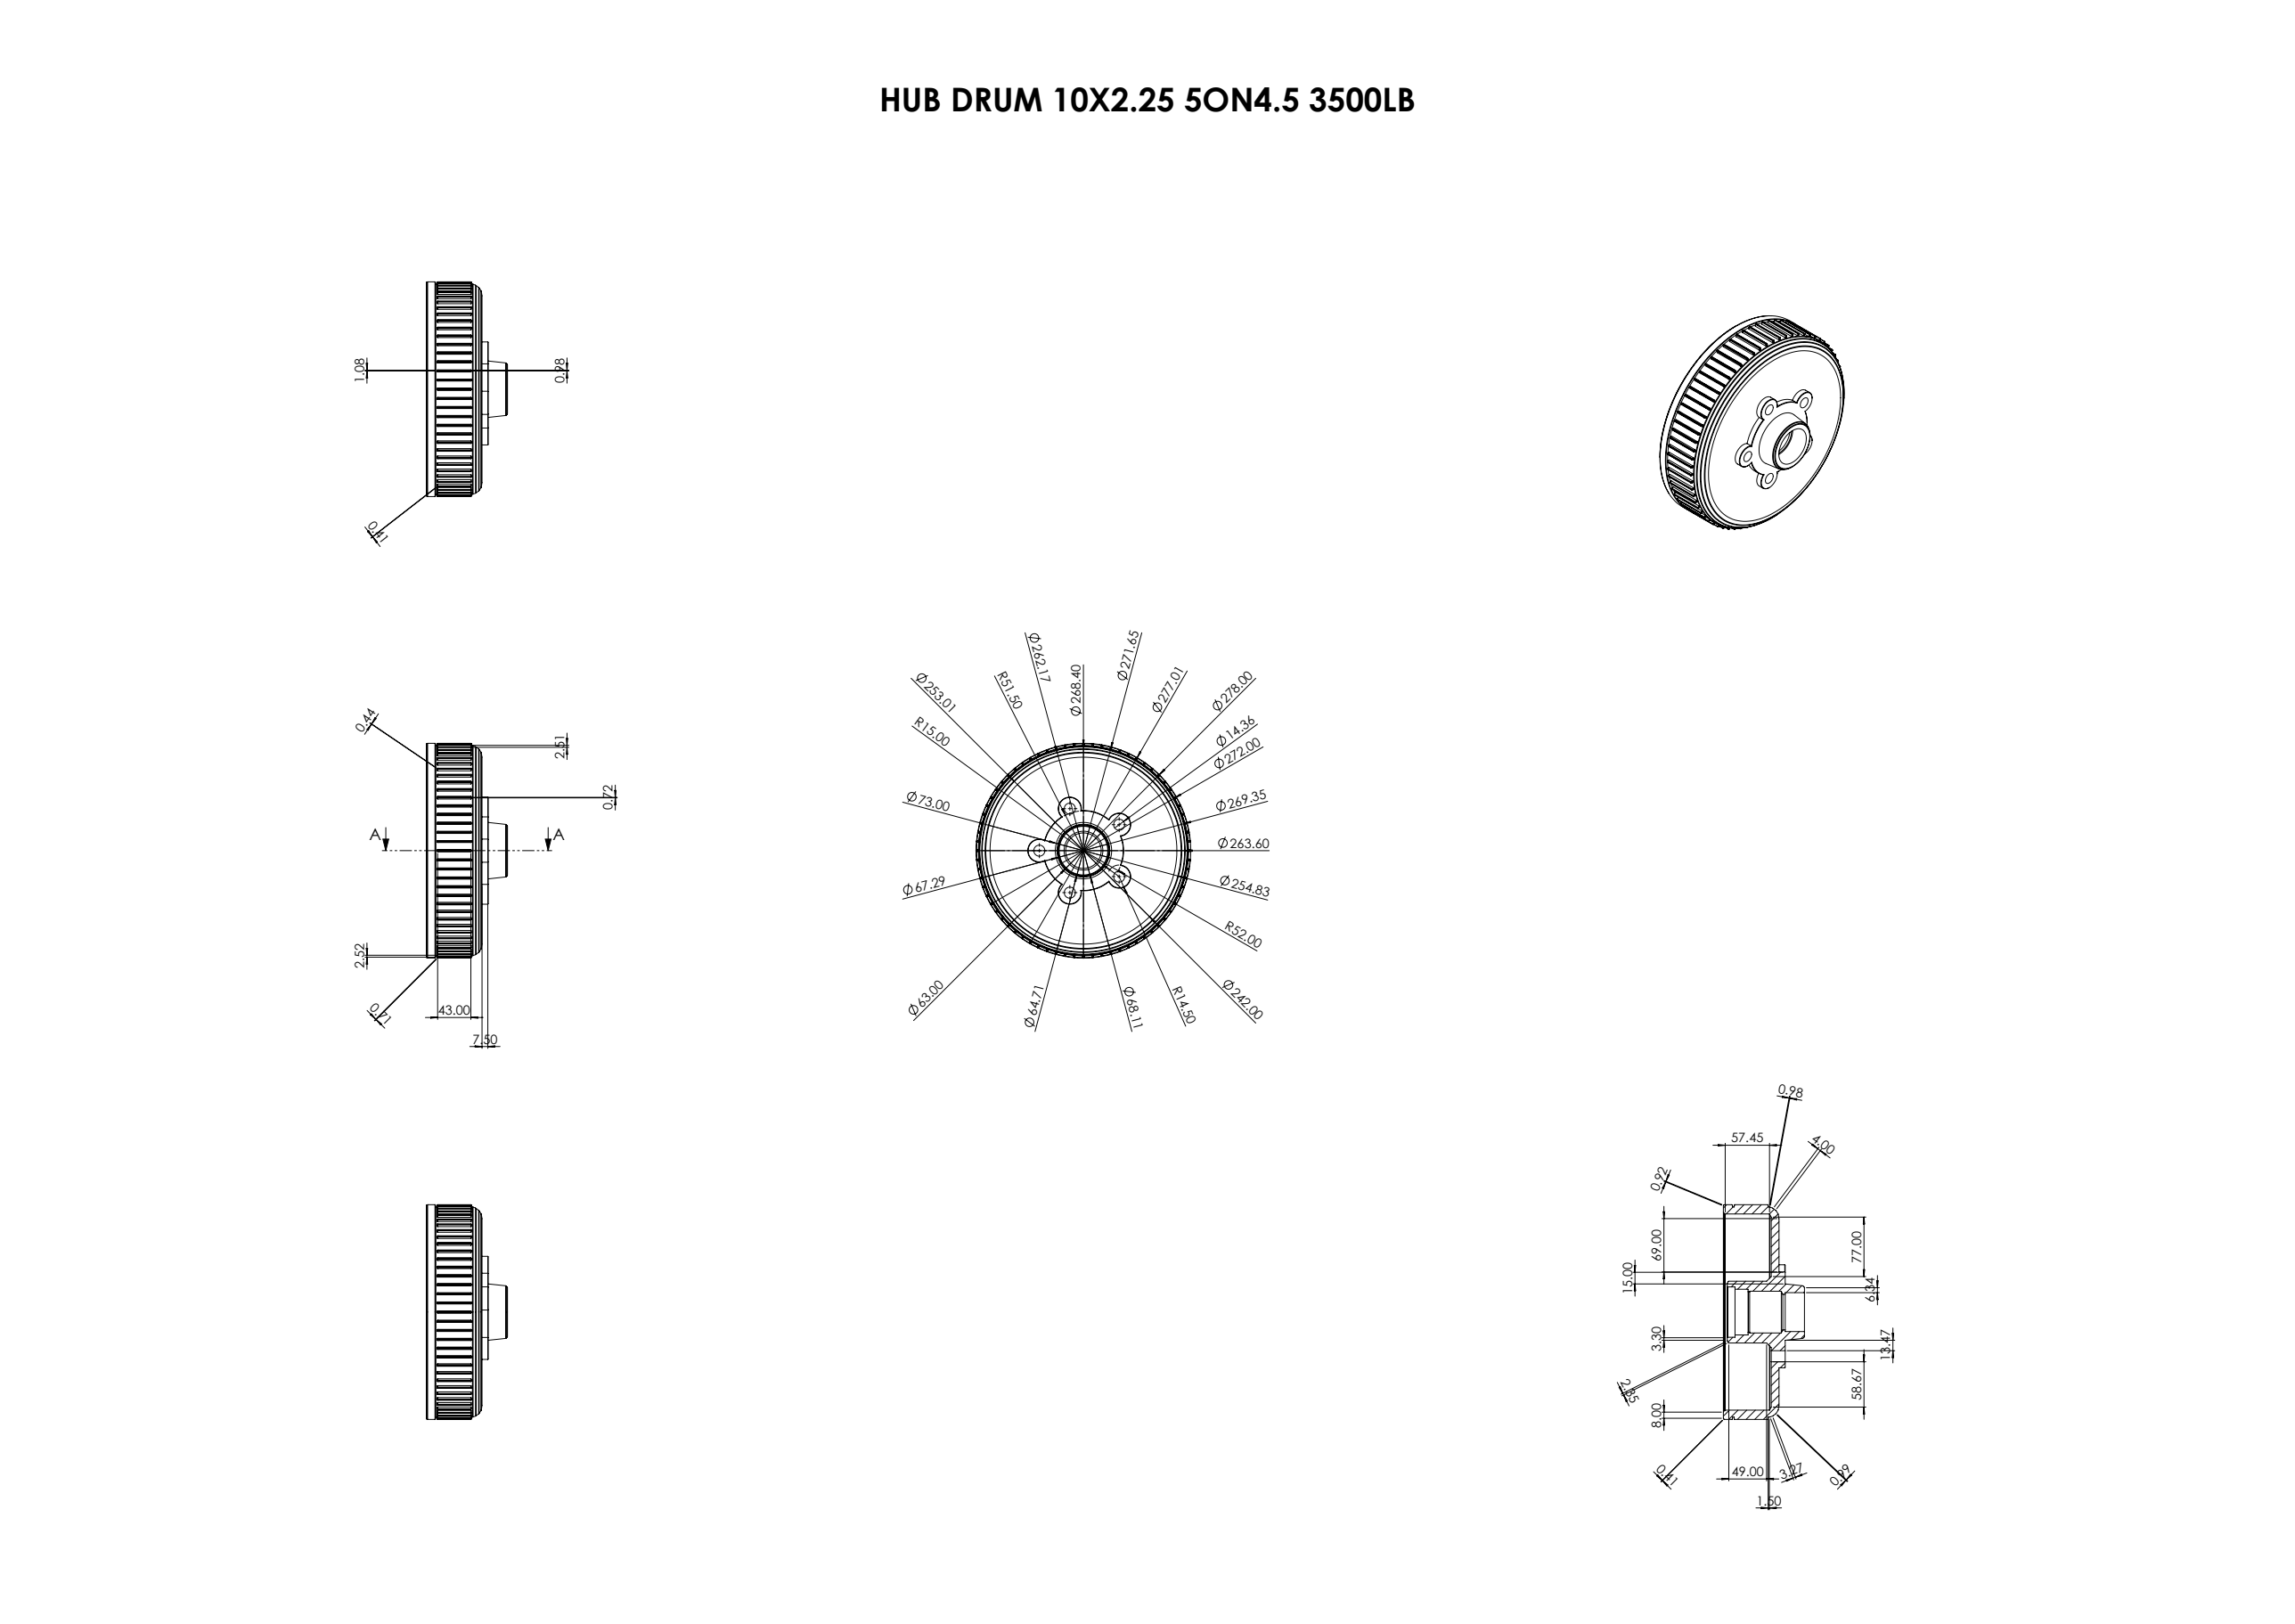
ISO-10303-21;
HEADER;
/* Generated by software containing ST-Developer
 * from STEP Tools, Inc. (www.steptools.com) 
 */

FILE_DESCRIPTION(
/* description */ (''),
/* implementation_level */ '2;1');

FILE_NAME(
/* name */ '01_Hub_Drum_10x2.25_5on4.5_3500lb.step',
/* time_stamp */ '2026-10-25T01:26:34-07:00',
/* author */ (''),
/* organization */ (''),
/* preprocessor_version */ 'ST-DEVELOPER v20.2',
/* originating_system */ 'Autodesk Translation Framework v15.15.0.0',
/* authorisation */ '');

FILE_SCHEMA (('AUTOMOTIVE_DESIGN { 1 0 10303 214 3 1 1 }'));
ENDSEC;

DATA;
#10=MECHANICAL_DESIGN_GEOMETRIC_PRESENTATION_REPRESENTATION('',(#321),#71628);
#295=SHAPE_REPRESENTATION_RELATIONSHIP('SRR','None',#71683,#308);
#308=ADVANCED_BREP_SHAPE_REPRESENTATION('',(#334),#71615);
#321=STYLED_ITEM('',(#71804),#334);
#334=MANIFOLD_SOLID_BREP('Body1',#34208);
#347=B_SPLINE_CURVE_WITH_KNOTS('',3,(#48590,#48591,#48592,#48593),
 .UNSPECIFIED.,.F.,.F.,(4,4),(-0.0954037219784117,0.),.UNSPECIFIED.);
#348=B_SPLINE_CURVE_WITH_KNOTS('',3,(#48596,#48597,#48598,#48599),
 .UNSPECIFIED.,.F.,.F.,(4,4),(-0.0954037219783748,0.),.UNSPECIFIED.);
#349=B_SPLINE_CURVE_WITH_KNOTS('',3,(#48604,#48605,#48606,#48607),
 .UNSPECIFIED.,.F.,.F.,(4,4),(-0.0954037219783863,0.),.UNSPECIFIED.);
#350=B_SPLINE_CURVE_WITH_KNOTS('',3,(#48613,#48614,#48615,#48616),
 .UNSPECIFIED.,.F.,.F.,(4,4),(-0.0954037219782671,0.),.UNSPECIFIED.);
#351=B_SPLINE_CURVE_WITH_KNOTS('',3,(#48622,#48623,#48624,#48625),
 .UNSPECIFIED.,.F.,.F.,(4,4),(-0.0954037219784872,0.),.UNSPECIFIED.);
#352=B_SPLINE_CURVE_WITH_KNOTS('',3,(#48631,#48632,#48633,#48634),
 .UNSPECIFIED.,.F.,.F.,(4,4),(-0.0954037219781768,0.),.UNSPECIFIED.);
#353=B_SPLINE_CURVE_WITH_KNOTS('',3,(#48640,#48641,#48642,#48643),
 .UNSPECIFIED.,.F.,.F.,(4,4),(-0.0954037219782904,0.),.UNSPECIFIED.);
#354=B_SPLINE_CURVE_WITH_KNOTS('',3,(#48650,#48651,#48652,#48653),
 .UNSPECIFIED.,.F.,.F.,(4,4),(-0.0954037219784109,0.),.UNSPECIFIED.);
#355=B_SPLINE_CURVE_WITH_KNOTS('',3,(#48659,#48660,#48661,#48662),
 .UNSPECIFIED.,.F.,.F.,(4,4),(-0.0954037219783438,0.),.UNSPECIFIED.);
#356=B_SPLINE_CURVE_WITH_KNOTS('',3,(#48668,#48669,#48670,#48671),
 .UNSPECIFIED.,.F.,.F.,(4,4),(-0.0954037219783345,0.),.UNSPECIFIED.);
#842=ELLIPSE('',#34430,192.333044482741,136.);
#843=ELLIPSE('',#34431,192.333044482741,136.);
#844=ELLIPSE('',#34435,192.333044482741,136.);
#845=ELLIPSE('',#34436,192.333044482741,136.);
#846=ELLIPSE('',#34438,192.333044482741,136.);
#847=ELLIPSE('',#34440,192.333044482741,136.);
#848=ELLIPSE('',#34441,192.333044482741,136.);
#849=ELLIPSE('',#34443,192.333044482741,136.);
#850=ELLIPSE('',#34444,192.333044482741,136.);
#851=ELLIPSE('',#34446,192.333044482741,136.);
#852=ELLIPSE('',#34447,192.33304448274,136.);
#853=ELLIPSE('',#34449,192.33304448274,136.);
#854=ELLIPSE('',#34450,192.333044482742,136.);
#855=ELLIPSE('',#34452,192.333044482743,136.);
#856=ELLIPSE('',#34453,192.333044482742,136.);
#857=ELLIPSE('',#34455,192.33304448274,136.);
#858=ELLIPSE('',#34456,192.33304448274,136.);
#859=ELLIPSE('',#34458,192.333044482743,136.);
#860=ELLIPSE('',#34459,192.333044482742,136.);
#861=ELLIPSE('',#34461,192.33304448274,136.);
#862=ELLIPSE('',#34462,192.333044482743,136.);
#863=ELLIPSE('',#34464,192.333044482739,136.);
#864=ELLIPSE('',#34465,192.333044482741,136.);
#865=ELLIPSE('',#34467,192.333044482745,136.);
#866=ELLIPSE('',#34468,192.333044482737,136.);
#867=ELLIPSE('',#34470,192.333044482741,136.);
#868=ELLIPSE('',#34471,192.333044482739,136.);
#869=ELLIPSE('',#34473,192.333044482738,136.);
#870=ELLIPSE('',#34474,192.333044482739,136.);
#871=ELLIPSE('',#34476,192.333044482743,136.);
#872=ELLIPSE('',#34477,192.333044482742,136.);
#873=ELLIPSE('',#34479,192.333044482738,136.);
#874=ELLIPSE('',#34480,192.333044482743,136.);
#875=ELLIPSE('',#34482,192.333044482741,136.);
#876=ELLIPSE('',#34483,192.333044482741,136.);
#877=ELLIPSE('',#34485,192.333044482741,136.);
#878=ELLIPSE('',#34486,192.333044482743,136.);
#879=ELLIPSE('',#34488,192.333044482743,136.);
#880=ELLIPSE('',#34489,192.33304448274,136.);
#881=ELLIPSE('',#34491,192.333044482743,136.);
#882=ELLIPSE('',#34492,192.33304448274,136.);
#883=ELLIPSE('',#34494,192.33304448274,136.);
#884=ELLIPSE('',#34495,192.33304448274,136.);
#885=ELLIPSE('',#34497,192.33304448274,136.);
#886=ELLIPSE('',#34498,192.333044482738,136.);
#887=ELLIPSE('',#34500,192.333044482741,136.);
#888=ELLIPSE('',#34501,192.333044482741,136.);
#889=ELLIPSE('',#34503,192.33304448274,136.);
#890=ELLIPSE('',#34504,192.33304448274,136.);
#891=ELLIPSE('',#34506,192.333044482742,136.);
#892=ELLIPSE('',#34507,192.333044482741,136.);
#893=ELLIPSE('',#34509,192.33304448274,136.);
#894=ELLIPSE('',#34510,192.333044482743,136.);
#895=ELLIPSE('',#34512,192.33304448274,136.);
#896=ELLIPSE('',#34513,192.33304448274,136.);
#897=ELLIPSE('',#34515,192.333044482739,136.);
#898=ELLIPSE('',#34516,192.33304448274,136.);
#899=ELLIPSE('',#34518,192.33304448274,136.);
#900=ELLIPSE('',#34519,192.33304448274,136.);
#901=ELLIPSE('',#34521,192.333044482739,136.);
#902=ELLIPSE('',#34522,192.333044482741,136.);
#903=ELLIPSE('',#34524,192.333044482743,136.);
#904=ELLIPSE('',#34525,192.333044482743,136.);
#905=ELLIPSE('',#34527,192.333044482741,136.);
#906=ELLIPSE('',#34528,192.333044482742,136.);
#907=ELLIPSE('',#34530,192.333044482741,136.);
#908=ELLIPSE('',#34531,192.333044482741,136.);
#909=ELLIPSE('',#34533,192.333044482742,136.);
#910=ELLIPSE('',#34534,192.333044482742,136.);
#911=ELLIPSE('',#34536,192.333044482742,136.);
#912=ELLIPSE('',#34537,192.333044482741,136.);
#913=ELLIPSE('',#34539,192.333044482741,136.);
#914=ELLIPSE('',#34540,192.333044482742,136.);
#915=ELLIPSE('',#34542,192.333044482741,136.);
#916=ELLIPSE('',#34543,192.33304448274,136.);
#917=ELLIPSE('',#34545,192.333044482742,136.);
#918=ELLIPSE('',#34546,192.333044482741,136.);
#919=ELLIPSE('',#34548,192.333044482741,136.);
#920=ELLIPSE('',#34549,192.33304448274,136.);
#921=ELLIPSE('',#34551,192.33304448274,136.);
#922=ELLIPSE('',#34552,192.333044482741,136.);
#923=ELLIPSE('',#34554,192.333044482743,136.);
#924=ELLIPSE('',#34555,192.333044482741,136.);
#925=ELLIPSE('',#34557,192.33304448274,136.);
#926=ELLIPSE('',#34558,192.33304448274,136.);
#927=ELLIPSE('',#34560,192.333044482742,136.);
#928=ELLIPSE('',#34561,192.333044482742,136.);
#929=ELLIPSE('',#34563,192.333044482742,136.);
#930=ELLIPSE('',#34564,192.333044482743,136.);
#931=ELLIPSE('',#34566,192.33304448274,136.);
#932=ELLIPSE('',#34567,192.333044482741,136.);
#933=ELLIPSE('',#34569,192.333044482745,136.);
#934=ELLIPSE('',#34570,192.33304448274,136.);
#935=ELLIPSE('',#34572,192.333044482743,136.);
#936=ELLIPSE('',#34573,192.333044482741,136.);
#937=ELLIPSE('',#34575,192.33304448274,136.);
#938=ELLIPSE('',#34576,192.33304448274,136.);
#939=ELLIPSE('',#34578,192.333044482743,136.);
#940=ELLIPSE('',#34579,192.333044482742,136.);
#941=ELLIPSE('',#34581,192.33304448274,136.);
#942=ELLIPSE('',#34582,192.333044482742,136.);
#943=ELLIPSE('',#34584,192.333044482741,136.);
#944=ELLIPSE('',#34585,192.333044482741,136.);
#945=ELLIPSE('',#34587,192.333044482741,136.);
#946=ELLIPSE('',#34588,192.333044482743,136.);
#947=ELLIPSE('',#34590,192.333044482741,136.);
#948=ELLIPSE('',#34591,192.33304448274,136.);
#949=ELLIPSE('',#34593,192.333044482743,136.);
#950=ELLIPSE('',#34594,192.33304448274,136.);
#951=ELLIPSE('',#34596,192.33304448274,136.);
#952=ELLIPSE('',#34597,192.33304448274,136.);
#953=ELLIPSE('',#34599,192.33304448274,136.);
#954=ELLIPSE('',#34600,192.333044482738,136.);
#955=ELLIPSE('',#34602,192.333044482741,136.);
#956=ELLIPSE('',#34603,192.333044482741,136.);
#957=ELLIPSE('',#34605,192.333044482738,136.);
#958=ELLIPSE('',#34606,192.333044482743,136.);
#959=ELLIPSE('',#34608,192.333044482742,136.);
#960=ELLIPSE('',#34609,192.333044482741,136.);
#961=ELLIPSE('',#34611,192.33304448274,136.);
#962=ELLIPSE('',#34612,192.333044482741,136.);
#963=ELLIPSE('',#34614,192.333044482739,136.);
#964=ELLIPSE('',#34615,192.33304448274,136.);
#965=ELLIPSE('',#34617,192.333044482741,136.);
#966=ELLIPSE('',#34618,192.333044482741,136.);
#967=ELLIPSE('',#34620,192.333044482739,136.);
#968=ELLIPSE('',#34621,192.333044482738,136.);
#969=ELLIPSE('',#34623,192.333044482741,136.);
#970=ELLIPSE('',#34624,192.333044482743,136.);
#971=ELLIPSE('',#34626,192.333044482743,136.);
#972=ELLIPSE('',#34627,192.333044482743,136.);
#973=ELLIPSE('',#34629,192.333044482741,136.);
#974=ELLIPSE('',#34630,192.333044482741,136.);
#975=ELLIPSE('',#34632,192.333044482741,136.);
#976=ELLIPSE('',#34633,192.333044482741,136.);
#977=ELLIPSE('',#34635,192.333044482742,136.);
#978=ELLIPSE('',#34636,192.333044482743,136.);
#979=ELLIPSE('',#34638,192.33304448274,136.);
#980=ELLIPSE('',#34639,192.333044482739,136.);
#981=ELLIPSE('',#34641,192.333044482742,136.);
#982=ELLIPSE('',#34642,192.333044482741,136.);
#983=ELLIPSE('',#34644,192.33304448274,136.);
#984=ELLIPSE('',#34645,192.33304448274,136.);
#985=ELLIPSE('',#34647,192.333044482741,136.);
#986=ELLIPSE('',#34648,192.333044482741,136.);
#987=ELLIPSE('',#34650,192.333044482741,136.);
#988=ELLIPSE('',#34651,192.33304448274,136.);
#989=ELLIPSE('',#34653,192.333044482741,136.);
#990=ELLIPSE('',#34654,192.333044482741,136.);
#991=ELLIPSE('',#34656,192.333044482741,136.);
#992=ELLIPSE('',#34657,192.33304448274,136.);
#993=ELLIPSE('',#34659,192.33304448274,136.);
#994=ELLIPSE('',#34660,192.333044482742,136.);
#995=ELLIPSE('',#34662,192.333044482743,136.);
#996=ELLIPSE('',#34663,192.333044482742,136.);
#997=ELLIPSE('',#34665,192.33304448274,136.);
#998=ELLIPSE('',#34666,192.333044482741,136.);
#999=ELLIPSE('',#34668,192.333044482742,136.);
#1000=ELLIPSE('',#34669,192.333044482742,136.);
#1001=ELLIPSE('',#34671,192.33304448274,136.);
#1002=ELLIPSE('',#34672,192.333044482745,136.);
#1003=ELLIPSE('',#34674,192.333044482739,136.);
#1004=ELLIPSE('',#34675,192.333044482741,136.);
#1005=ELLIPSE('',#34677,192.333044482745,136.);
#1006=ELLIPSE('',#34678,192.333044482739,136.);
#1007=ELLIPSE('',#34680,192.333044482741,136.);
#1008=ELLIPSE('',#34681,192.333044482741,136.);
#1009=ELLIPSE('',#34683,192.333044482738,136.);
#1010=ELLIPSE('',#34684,192.33304448274,136.);
#1011=ELLIPSE('',#34686,192.333044482743,136.);
#1012=ELLIPSE('',#34687,192.333044482742,136.);
#1013=ELLIPSE('',#34689,192.33304448274,136.);
#1014=ELLIPSE('',#34690,192.333044482742,136.);
#1015=ELLIPSE('',#34692,192.333044482741,136.);
#1016=ELLIPSE('',#34693,192.333044482741,136.);
#1017=ELLIPSE('',#34695,192.333044482741,136.);
#1018=ELLIPSE('',#34696,192.333044482743,136.);
#1019=ELLIPSE('',#34698,192.333044482743,136.);
#1020=ELLIPSE('',#34699,192.33304448274,136.);
#1021=ELLIPSE('',#34701,192.333044482743,136.);
#1022=ELLIPSE('',#34702,192.333044482738,136.);
#1023=ELLIPSE('',#34704,192.33304448274,136.);
#1024=ELLIPSE('',#34705,192.33304448274,136.);
#1025=ELLIPSE('',#34707,192.33304448274,136.);
#1026=ELLIPSE('',#34708,192.333044482738,136.);
#1027=ELLIPSE('',#34710,192.333044482741,136.);
#1028=ELLIPSE('',#34711,192.333044482741,136.);
#1029=ELLIPSE('',#34713,192.333044482738,136.);
#1030=ELLIPSE('',#34714,192.333044482743,136.);
#1031=ELLIPSE('',#34716,192.333044482742,136.);
#1032=ELLIPSE('',#34717,192.333044482741,136.);
#1033=ELLIPSE('',#34719,192.33304448274,136.);
#1034=ELLIPSE('',#34720,192.333044482744,136.);
#1035=ELLIPSE('',#34722,192.33304448274,136.);
#1036=ELLIPSE('',#34723,192.33304448274,136.);
#1037=ELLIPSE('',#34725,192.333044482741,136.);
#1038=ELLIPSE('',#34726,192.333044482741,136.);
#1039=ELLIPSE('',#34728,192.33304448274,136.);
#1040=ELLIPSE('',#34729,192.33304448274,136.);
#1041=ELLIPSE('',#34731,192.333044482741,136.);
#1042=ELLIPSE('',#34732,192.333044482741,136.);
#1043=ELLIPSE('',#34734,192.333044482742,136.);
#1044=ELLIPSE('',#34735,192.333044482741,136.);
#1045=ELLIPSE('',#34737,192.333044482741,136.);
#1046=ELLIPSE('',#34738,192.333044482741,136.);
#1047=ELLIPSE('',#34740,192.33304448274,136.);
#1048=ELLIPSE('',#34741,192.333044482742,136.);
#1049=ELLIPSE('',#34743,192.333044482742,136.);
#1050=ELLIPSE('',#34744,192.333044482743,136.);
#1051=ELLIPSE('',#34746,192.333044482742,136.);
#1052=ELLIPSE('',#34747,192.333044482741,136.);
#1053=ELLIPSE('',#34749,192.333044482741,136.);
#1054=ELLIPSE('',#34750,192.333044482742,136.);
#1055=ELLIPSE('',#34752,192.333044482741,136.);
#1056=ELLIPSE('',#34753,192.33304448274,136.);
#1057=ELLIPSE('',#34755,192.333044482741,136.);
#1058=ELLIPSE('',#34756,192.333044482741,136.);
#1059=ELLIPSE('',#34758,192.333044482741,136.);
#1060=ELLIPSE('',#34759,192.33304448274,136.);
#1061=ELLIPSE('',#34761,192.333044482741,136.);
#1062=ELLIPSE('',#34762,192.333044482741,136.);
#1063=ELLIPSE('',#34764,192.333044482741,136.);
#1064=ELLIPSE('',#34765,192.333044482741,136.);
#1065=ELLIPSE('',#34767,192.33304448274,136.);
#1066=ELLIPSE('',#34768,192.333044482742,136.);
#1067=ELLIPSE('',#34770,192.333044482742,136.);
#1068=ELLIPSE('',#34771,192.333044482741,136.);
#1069=ELLIPSE('',#34773,192.33304448274,136.);
#1070=ELLIPSE('',#34774,192.33304448274,136.);
#1071=ELLIPSE('',#34776,192.333044482742,136.);
#1072=ELLIPSE('',#34777,192.333044482742,136.);
#1073=ELLIPSE('',#34779,192.33304448274,136.);
#1074=ELLIPSE('',#34780,192.333044482742,136.);
#1075=ELLIPSE('',#34782,192.333044482741,136.);
#1076=ELLIPSE('',#34783,192.333044482741,136.);
#1077=ELLIPSE('',#34785,192.333044482743,136.);
#1078=ELLIPSE('',#34786,192.33304448274,136.);
#1079=ELLIPSE('',#34788,192.333044482743,136.);
#1080=ELLIPSE('',#34789,192.333044482742,136.);
#1081=ELLIPSE('',#34791,192.33304448274,136.);
#1082=ELLIPSE('',#34792,192.333044482739,136.);
#1083=ELLIPSE('',#34794,192.333044482741,136.);
#1084=ELLIPSE('',#34795,192.333044482741,136.);
#1085=ELLIPSE('',#34797,192.333044482738,136.);
#1086=ELLIPSE('',#34798,192.333044482743,136.);
#1087=ELLIPSE('',#34800,192.333044482741,136.);
#1088=ELLIPSE('',#34801,192.333044482741,136.);
#1089=ELLIPSE('',#34803,192.333044482741,136.);
#1090=ELLIPSE('',#34804,192.333044482743,136.);
#1091=ELLIPSE('',#34806,192.333044482741,136.);
#1092=ELLIPSE('',#34807,192.33304448274,136.);
#1093=ELLIPSE('',#34809,192.333044482743,136.);
#1094=ELLIPSE('',#34810,192.33304448274,136.);
#1095=ELLIPSE('',#34812,192.33304448274,136.);
#1096=ELLIPSE('',#34813,192.33304448274,136.);
#1097=ELLIPSE('',#34815,192.33304448274,136.);
#1098=ELLIPSE('',#34816,192.333044482738,136.);
#1099=ELLIPSE('',#34818,192.333044482738,136.);
#1100=ELLIPSE('',#34819,192.333044482743,136.);
#1101=ELLIPSE('',#34821,192.333044482738,136.);
#1102=ELLIPSE('',#34822,192.333044482743,136.);
#1103=ELLIPSE('',#34824,192.33304448274,136.);
#1104=ELLIPSE('',#34825,192.33304448274,136.);
#1105=ELLIPSE('',#34827,192.33304448274,136.);
#1106=ELLIPSE('',#34828,192.333044482744,136.);
#1107=ELLIPSE('',#34830,192.33304448274,136.);
#1108=ELLIPSE('',#34831,192.33304448274,136.);
#1109=ELLIPSE('',#34833,192.333044482741,136.);
#1110=ELLIPSE('',#34834,192.333044482741,136.);
#1111=ELLIPSE('',#34836,192.33304448274,136.);
#1112=ELLIPSE('',#34837,192.33304448274,136.);
#1113=ELLIPSE('',#34839,192.333044482741,136.);
#1114=ELLIPSE('',#34840,192.333044482743,136.);
#1115=ELLIPSE('',#34842,192.333044482743,136.);
#1116=ELLIPSE('',#34843,192.33304448274,136.);
#1117=ELLIPSE('',#34845,192.333044482742,136.);
#1118=ELLIPSE('',#34846,192.333044482742,136.);
#1119=ELLIPSE('',#34848,192.333044482741,136.);
#1120=ELLIPSE('',#34849,192.333044482741,136.);
#1121=ELLIPSE('',#34851,192.333044482742,136.);
#1122=ELLIPSE('',#34852,192.333044482743,136.);
#1123=ELLIPSE('',#34854,192.333044482742,136.);
#1124=ELLIPSE('',#34855,192.333044482741,136.);
#1125=ELLIPSE('',#34857,192.333044482741,136.);
#1126=ELLIPSE('',#34858,192.333044482742,136.);
#1127=ELLIPSE('',#34860,192.333044482741,136.);
#1128=ELLIPSE('',#34861,192.33304448274,136.);
#1129=ELLIPSE('',#34863,192.333044482741,136.);
#1130=FACE_BOUND('',#5239,.T.);
#1131=FACE_BOUND('',#5243,.T.);
#1132=FACE_BOUND('',#5247,.T.);
#1133=FACE_BOUND('',#5259,.T.);
#1134=FACE_BOUND('',#5260,.T.);
#1135=FACE_BOUND('',#5261,.T.);
#1136=FACE_BOUND('',#5262,.T.);
#1137=FACE_BOUND('',#5263,.T.);
#1138=FACE_BOUND('',#5264,.T.);
#1139=FACE_BOUND('',#5265,.T.);
#1140=FACE_BOUND('',#5266,.T.);
#1141=FACE_BOUND('',#5267,.T.);
#1142=FACE_BOUND('',#5268,.T.);
#1143=FACE_BOUND('',#5269,.T.);
#1144=FACE_BOUND('',#5270,.T.);
#1145=FACE_BOUND('',#5271,.T.);
#1146=FACE_BOUND('',#5272,.T.);
#1147=FACE_BOUND('',#5273,.T.);
#1148=FACE_BOUND('',#5274,.T.);
#1149=FACE_BOUND('',#5275,.T.);
#1150=FACE_BOUND('',#5276,.T.);
#1151=FACE_BOUND('',#5277,.T.);
#1152=FACE_BOUND('',#5278,.T.);
#1153=FACE_BOUND('',#5279,.T.);
#1154=FACE_BOUND('',#5280,.T.);
#1155=FACE_BOUND('',#5281,.T.);
#1156=FACE_BOUND('',#5282,.T.);
#1157=FACE_BOUND('',#5283,.T.);
#1158=FACE_BOUND('',#5284,.T.);
#1159=FACE_BOUND('',#5285,.T.);
#1160=FACE_BOUND('',#5286,.T.);
#1161=FACE_BOUND('',#5287,.T.);
#1162=FACE_BOUND('',#5288,.T.);
#1163=FACE_BOUND('',#5289,.T.);
#1164=FACE_BOUND('',#5290,.T.);
#1165=FACE_BOUND('',#5291,.T.);
#1166=FACE_BOUND('',#5292,.T.);
#1167=FACE_BOUND('',#5293,.T.);
#1168=FACE_BOUND('',#5294,.T.);
#1169=FACE_BOUND('',#5295,.T.);
#1170=FACE_BOUND('',#5296,.T.);
#1171=FACE_BOUND('',#5297,.T.);
#1172=FACE_BOUND('',#5298,.T.);
#1173=FACE_BOUND('',#5299,.T.);
#1174=FACE_BOUND('',#5300,.T.);
#1175=FACE_BOUND('',#5301,.T.);
#1176=FACE_BOUND('',#5302,.T.);
#1177=FACE_BOUND('',#5303,.T.);
#1178=FACE_BOUND('',#5304,.T.);
#1179=FACE_BOUND('',#5305,.T.);
#1180=FACE_BOUND('',#5306,.T.);
#1181=FACE_BOUND('',#5307,.T.);
#1182=FACE_BOUND('',#5308,.T.);
#1183=FACE_BOUND('',#5309,.T.);
#1184=FACE_BOUND('',#5310,.T.);
#1185=FACE_BOUND('',#5311,.T.);
#1186=FACE_BOUND('',#5312,.T.);
#1187=FACE_BOUND('',#5313,.T.);
#1188=FACE_BOUND('',#5314,.T.);
#1189=FACE_BOUND('',#5315,.T.);
#1190=FACE_BOUND('',#5316,.T.);
#1191=FACE_BOUND('',#5317,.T.);
#1192=FACE_BOUND('',#5318,.T.);
#1193=FACE_BOUND('',#5319,.T.);
#1194=FACE_BOUND('',#5320,.T.);
#1195=FACE_BOUND('',#5321,.T.);
#1196=FACE_BOUND('',#5322,.T.);
#1197=FACE_BOUND('',#5323,.T.);
#1198=FACE_BOUND('',#5324,.T.);
#1199=FACE_BOUND('',#5325,.T.);
#1200=FACE_BOUND('',#5326,.T.);
#1201=FACE_BOUND('',#5327,.T.);
#1202=FACE_BOUND('',#5328,.T.);
#1203=FACE_BOUND('',#5329,.T.);
#1204=FACE_BOUND('',#5347,.T.);
#1205=FACE_BOUND('',#5348,.T.);
#1206=FACE_BOUND('',#5349,.T.);
#1207=FACE_BOUND('',#5350,.T.);
#1208=FACE_BOUND('',#5351,.T.);
#1209=FACE_BOUND('',#5352,.T.);
#1210=FACE_BOUND('',#6399,.T.);
#1211=FACE_BOUND('',#6559,.T.);
#1212=FACE_BOUND('',#6562,.T.);
#1213=FACE_BOUND('',#6565,.T.);
#1214=FACE_BOUND('',#6568,.T.);
#1215=FACE_BOUND('',#6573,.T.);
#1216=FACE_BOUND('',#6574,.T.);
#1217=FACE_BOUND('',#6575,.T.);
#1218=FACE_BOUND('',#6576,.T.);
#1219=FACE_BOUND('',#6577,.T.);
#1220=FACE_BOUND('',#6578,.T.);
#1335=PLANE('',#34379);
#1336=PLANE('',#34387);
#1337=PLANE('',#34396);
#1338=PLANE('',#34906);
#1339=PLANE('',#34912);
#1340=PLANE('',#34913);
#1341=PLANE('',#34914);
#1342=PLANE('',#34915);
#1343=PLANE('',#34916);
#1344=PLANE('',#34917);
#1345=PLANE('',#34918);
#1346=PLANE('',#34919);
#1347=PLANE('',#34920);
#1348=PLANE('',#34921);
#1349=PLANE('',#34922);
#1350=PLANE('',#34923);
#1351=PLANE('',#34924);
#1352=PLANE('',#34925);
#1353=PLANE('',#34926);
#1354=PLANE('',#34927);
#1355=PLANE('',#34928);
#1356=PLANE('',#34929);
#1357=PLANE('',#34930);
#1358=PLANE('',#34931);
#1359=PLANE('',#34932);
#1360=PLANE('',#34933);
#1361=PLANE('',#34934);
#1362=PLANE('',#34935);
#1363=PLANE('',#34936);
#1364=PLANE('',#34937);
#1365=PLANE('',#34938);
#1366=PLANE('',#34939);
#1367=PLANE('',#34940);
#1368=PLANE('',#34941);
#1369=PLANE('',#34942);
#1370=PLANE('',#34943);
#1371=PLANE('',#34944);
#1372=PLANE('',#34945);
#1373=PLANE('',#34946);
#1374=PLANE('',#34947);
#1375=PLANE('',#34948);
#1376=PLANE('',#34949);
#1377=PLANE('',#34950);
#1378=PLANE('',#34951);
#1379=PLANE('',#34952);
#1380=PLANE('',#34953);
#1381=PLANE('',#34954);
#1382=PLANE('',#34955);
#1383=PLANE('',#34956);
#1384=PLANE('',#34957);
#1385=PLANE('',#34958);
#1386=PLANE('',#34959);
#1387=PLANE('',#34960);
#1388=PLANE('',#34961);
#1389=PLANE('',#34962);
#1390=PLANE('',#34963);
#1391=PLANE('',#34964);
#1392=PLANE('',#34965);
#1393=PLANE('',#34966);
#1394=PLANE('',#34967);
#1395=PLANE('',#34968);
#1396=PLANE('',#34969);
#1397=PLANE('',#34970);
#1398=PLANE('',#34971);
#1399=PLANE('',#34972);
#1400=PLANE('',#34973);
#1401=PLANE('',#34974);
#1402=PLANE('',#34975);
#1403=PLANE('',#34976);
#1404=PLANE('',#34977);
#1405=PLANE('',#34978);
#1406=PLANE('',#34979);
#1407=PLANE('',#34980);
#1408=PLANE('',#34981);
#1409=PLANE('',#34982);
#1410=PLANE('',#34983);
#1411=PLANE('',#34984);
#1412=PLANE('',#34985);
#1413=PLANE('',#34986);
#1414=PLANE('',#34987);
#1415=PLANE('',#34988);
#1416=PLANE('',#34989);
#1417=PLANE('',#34990);
#1418=PLANE('',#34991);
#1419=PLANE('',#34992);
#1420=PLANE('',#34993);
#1421=PLANE('',#34994);
#1422=PLANE('',#34995);
#1423=PLANE('',#34996);
#1424=PLANE('',#34997);
#1425=PLANE('',#34998);
#1426=PLANE('',#34999);
#1427=PLANE('',#35000);
#1428=PLANE('',#35001);
#1429=PLANE('',#35002);
#1430=PLANE('',#35003);
#1431=PLANE('',#35004);
#1432=PLANE('',#35005);
#1433=PLANE('',#35006);
#1434=PLANE('',#35007);
#1435=PLANE('',#35008);
#1436=PLANE('',#35009);
#1437=PLANE('',#35010);
#1438=PLANE('',#35011);
#1439=PLANE('',#35012);
#1440=PLANE('',#35013);
#1441=PLANE('',#35014);
#1442=PLANE('',#35015);
#1443=PLANE('',#35016);
#1444=PLANE('',#35017);
#1445=PLANE('',#35018);
#1446=PLANE('',#35019);
#1447=PLANE('',#35020);
#1448=PLANE('',#35021);
#1449=PLANE('',#35022);
#1450=PLANE('',#35023);
#1451=PLANE('',#35024);
#1452=PLANE('',#35025);
#1453=PLANE('',#35026);
#1454=PLANE('',#35027);
#1455=PLANE('',#35028);
#1456=PLANE('',#35029);
#1457=PLANE('',#35030);
#1458=PLANE('',#35031);
#1459=PLANE('',#35032);
#1460=PLANE('',#35033);
#1461=PLANE('',#35034);
#1462=PLANE('',#35035);
#1463=PLANE('',#35036);
#1464=PLANE('',#35037);
#1465=PLANE('',#35038);
#1466=PLANE('',#35039);
#1467=PLANE('',#35040);
#1468=PLANE('',#35041);
#1469=PLANE('',#35042);
#1470=PLANE('',#35043);
#1471=PLANE('',#35044);
#1472=PLANE('',#35045);
#1473=PLANE('',#35046);
#1474=PLANE('',#35047);
#1475=PLANE('',#35048);
#1476=PLANE('',#35049);
#1477=PLANE('',#35050);
#1478=PLANE('',#35051);
#1479=PLANE('',#35052);
#1480=PLANE('',#35053);
#1481=PLANE('',#35054);
#1482=PLANE('',#35055);
#1483=PLANE('',#35056);
#1484=PLANE('',#35057);
#1485=PLANE('',#35058);
#1486=PLANE('',#35059);
#1487=PLANE('',#35060);
#1488=PLANE('',#35061);
#1489=PLANE('',#35062);
#1490=PLANE('',#35063);
#1491=PLANE('',#35064);
#1492=PLANE('',#35065);
#1493=PLANE('',#35066);
#1494=PLANE('',#35067);
#1495=PLANE('',#35068);
#1496=PLANE('',#35069);
#1497=PLANE('',#35070);
#1498=PLANE('',#35071);
#1499=PLANE('',#35072);
#1500=PLANE('',#35073);
#1501=PLANE('',#35074);
#1502=PLANE('',#35075);
#1503=PLANE('',#35076);
#1504=PLANE('',#35077);
#1505=PLANE('',#35078);
#1506=PLANE('',#35079);
#1507=PLANE('',#35080);
#1508=PLANE('',#35081);
#1509=PLANE('',#35082);
#1510=PLANE('',#35083);
#1511=PLANE('',#35084);
#1512=PLANE('',#35085);
#1513=PLANE('',#35086);
#1514=PLANE('',#35087);
#1515=PLANE('',#35088);
#1516=PLANE('',#35089);
#1517=PLANE('',#35090);
#1518=PLANE('',#35091);
#1519=PLANE('',#35092);
#1520=PLANE('',#35093);
#1521=PLANE('',#35094);
#1522=PLANE('',#35095);
#1523=PLANE('',#35096);
#1524=PLANE('',#35097);
#1525=PLANE('',#35098);
#1526=PLANE('',#35099);
#1527=PLANE('',#35100);
#1528=PLANE('',#35101);
#1529=PLANE('',#35102);
#1530=PLANE('',#35103);
#1531=PLANE('',#35104);
#1532=PLANE('',#35105);
#1533=PLANE('',#35106);
#1534=PLANE('',#35107);
#1535=PLANE('',#35108);
#1536=PLANE('',#35109);
#1537=PLANE('',#35110);
#1538=PLANE('',#35111);
#1539=PLANE('',#35112);
#1540=PLANE('',#35113);
#1541=PLANE('',#35114);
#1542=PLANE('',#35115);
#1543=PLANE('',#35116);
#1544=PLANE('',#35117);
#1545=PLANE('',#35118);
#1546=PLANE('',#35119);
#1547=PLANE('',#35120);
#1548=PLANE('',#35121);
#1549=PLANE('',#35122);
#1550=PLANE('',#35123);
#1551=PLANE('',#35124);
#1552=PLANE('',#35125);
#1553=PLANE('',#35126);
#1554=PLANE('',#35127);
#1555=PLANE('',#35128);
#1556=PLANE('',#35129);
#1557=PLANE('',#35130);
#1558=PLANE('',#35131);
#1559=PLANE('',#35132);
#1560=PLANE('',#35133);
#1561=PLANE('',#35134);
#1562=PLANE('',#35135);
#1563=PLANE('',#35136);
#1564=PLANE('',#35137);
#1565=PLANE('',#35138);
#1566=PLANE('',#35139);
#1567=PLANE('',#35140);
#1568=PLANE('',#35141);
#1569=PLANE('',#35142);
#1570=PLANE('',#35143);
#1571=PLANE('',#35144);
#1572=PLANE('',#35145);
#1573=PLANE('',#35146);
#1574=PLANE('',#35147);
#1575=PLANE('',#35148);
#1576=PLANE('',#35149);
#1577=PLANE('',#35150);
#1578=PLANE('',#35151);
#1579=PLANE('',#35152);
#1580=PLANE('',#35153);
#1581=PLANE('',#35154);
#1582=PLANE('',#35155);
#1583=PLANE('',#35156);
#1584=PLANE('',#35157);
#1585=PLANE('',#35158);
#1586=PLANE('',#35159);
#1587=PLANE('',#35160);
#1588=PLANE('',#35161);
#1589=PLANE('',#35162);
#1590=PLANE('',#35163);
#1591=PLANE('',#35164);
#1592=PLANE('',#35165);
#1593=PLANE('',#35166);
#1594=PLANE('',#35167);
#1595=PLANE('',#35168);
#1596=PLANE('',#35169);
#1597=PLANE('',#35170);
#1598=PLANE('',#35171);
#1599=PLANE('',#35172);
#1600=PLANE('',#35173);
#1601=PLANE('',#35174);
#1602=PLANE('',#35175);
#1603=PLANE('',#35176);
#1604=PLANE('',#35177);
#1605=PLANE('',#35178);
#1606=PLANE('',#35179);
#1607=PLANE('',#35180);
#1608=PLANE('',#35181);
#1609=PLANE('',#35182);
#1610=PLANE('',#35183);
#1611=PLANE('',#35184);
#1612=PLANE('',#35185);
#1613=PLANE('',#35186);
#1614=PLANE('',#35187);
#1615=PLANE('',#35188);
#1616=PLANE('',#35189);
#1617=PLANE('',#35190);
#1618=PLANE('',#35191);
#1619=PLANE('',#35192);
#1620=PLANE('',#35193);
#1621=PLANE('',#35194);
#1622=PLANE('',#35195);
#1623=PLANE('',#35196);
#1624=PLANE('',#35197);
#1625=PLANE('',#35198);
#1626=PLANE('',#35199);
#1627=PLANE('',#35200);
#1628=PLANE('',#35201);
#1629=PLANE('',#35202);
#1630=PLANE('',#35203);
#1631=PLANE('',#35204);
#1632=PLANE('',#35205);
#1633=PLANE('',#35206);
#1634=PLANE('',#35207);
#1635=PLANE('',#35208);
#1636=PLANE('',#35209);
#1637=PLANE('',#35210);
#1638=PLANE('',#35211);
#1639=PLANE('',#35212);
#1640=PLANE('',#35213);
#1641=PLANE('',#35214);
#1642=PLANE('',#35215);
#1643=PLANE('',#35216);
#1644=PLANE('',#35217);
#1645=PLANE('',#35218);
#1646=PLANE('',#35219);
#1647=PLANE('',#35220);
#1648=PLANE('',#35221);
#1649=PLANE('',#35222);
#1650=PLANE('',#35223);
#1651=PLANE('',#35224);
#1652=PLANE('',#35225);
#1653=PLANE('',#35226);
#1654=PLANE('',#35227);
#1655=PLANE('',#35228);
#1656=PLANE('',#35229);
#1657=PLANE('',#35230);
#1658=PLANE('',#35231);
#1659=PLANE('',#35232);
#1660=PLANE('',#35233);
#1661=PLANE('',#35234);
#1662=PLANE('',#35235);
#1663=PLANE('',#35236);
#1664=PLANE('',#35237);
#1665=PLANE('',#35238);
#1666=PLANE('',#35239);
#1667=PLANE('',#35240);
#1668=PLANE('',#35241);
#1669=PLANE('',#35242);
#1670=PLANE('',#35243);
#1671=PLANE('',#35244);
#1672=PLANE('',#35245);
#1673=PLANE('',#35246);
#1674=PLANE('',#35247);
#1675=PLANE('',#35248);
#1676=PLANE('',#35249);
#1677=PLANE('',#35250);
#1678=PLANE('',#35251);
#1679=PLANE('',#35252);
#1680=PLANE('',#35253);
#1681=PLANE('',#35254);
#1682=PLANE('',#35255);
#1683=PLANE('',#35256);
#1684=PLANE('',#35257);
#1685=PLANE('',#35258);
#1686=PLANE('',#35259);
#1687=PLANE('',#35260);
#1688=PLANE('',#35261);
#1689=PLANE('',#35262);
#1690=PLANE('',#35263);
#1691=PLANE('',#35264);
#1692=PLANE('',#35265);
#1693=PLANE('',#35266);
#1694=PLANE('',#35267);
#1695=PLANE('',#35268);
#1696=PLANE('',#35269);
#1697=PLANE('',#35270);
#1698=PLANE('',#35271);
#1699=PLANE('',#35272);
#1700=PLANE('',#35273);
#1701=PLANE('',#35274);
#1702=PLANE('',#35275);
#1703=PLANE('',#35276);
#1704=PLANE('',#35277);
#1705=PLANE('',#35278);
#1706=PLANE('',#35279);
#1707=PLANE('',#35280);
#1708=PLANE('',#35281);
#1709=PLANE('',#35282);
#1710=PLANE('',#35283);
#1711=PLANE('',#35284);
#1712=PLANE('',#35285);
#1713=PLANE('',#35286);
#1714=PLANE('',#35287);
#1715=PLANE('',#35288);
#1716=PLANE('',#35289);
#1717=PLANE('',#35290);
#1718=PLANE('',#35291);
#1719=PLANE('',#35292);
#1720=PLANE('',#35293);
#1721=PLANE('',#35294);
#1722=PLANE('',#35295);
#1723=PLANE('',#35296);
#1724=PLANE('',#35297);
#1725=PLANE('',#35298);
#1726=PLANE('',#35299);
#1727=PLANE('',#35300);
#1728=PLANE('',#35301);
#1729=PLANE('',#35302);
#1730=PLANE('',#35303);
#1731=PLANE('',#35304);
#1732=PLANE('',#35305);
#1733=PLANE('',#35306);
#1734=PLANE('',#35307);
#1735=PLANE('',#35308);
#1736=PLANE('',#35309);
#1737=PLANE('',#35310);
#1738=PLANE('',#35311);
#1739=PLANE('',#35312);
#1740=PLANE('',#35313);
#1741=PLANE('',#35314);
#1742=PLANE('',#35315);
#1743=PLANE('',#35316);
#1744=PLANE('',#35317);
#1745=PLANE('',#35318);
#1746=PLANE('',#35319);
#1747=PLANE('',#35320);
#1748=PLANE('',#35321);
#1749=PLANE('',#35322);
#1750=PLANE('',#35323);
#1751=PLANE('',#35324);
#1752=PLANE('',#35325);
#1753=PLANE('',#35326);
#1754=PLANE('',#35327);
#1755=PLANE('',#35328);
#1756=PLANE('',#35329);
#1757=PLANE('',#35330);
#1758=PLANE('',#35331);
#1759=PLANE('',#35332);
#1760=PLANE('',#35333);
#1761=PLANE('',#35334);
#1762=PLANE('',#35335);
#1763=PLANE('',#35336);
#1764=PLANE('',#35337);
#1765=PLANE('',#35338);
#1766=PLANE('',#35339);
#1767=PLANE('',#35340);
#1768=PLANE('',#35341);
#1769=PLANE('',#35342);
#1770=PLANE('',#35343);
#1771=PLANE('',#35344);
#1772=PLANE('',#35345);
#1773=PLANE('',#35346);
#1774=PLANE('',#35347);
#1775=PLANE('',#35348);
#1776=PLANE('',#35349);
#1777=PLANE('',#35350);
#1778=PLANE('',#35351);
#1779=PLANE('',#35352);
#1780=PLANE('',#35353);
#1781=PLANE('',#35354);
#1782=PLANE('',#35355);
#1783=PLANE('',#35356);
#1784=PLANE('',#35357);
#1785=PLANE('',#35358);
#1786=PLANE('',#35359);
#1787=PLANE('',#35360);
#1788=PLANE('',#35361);
#1789=PLANE('',#35362);
#1790=PLANE('',#35363);
#1791=PLANE('',#35364);
#1792=PLANE('',#35365);
#1793=PLANE('',#35366);
#1794=PLANE('',#35367);
#1795=PLANE('',#35368);
#1796=PLANE('',#35369);
#1797=PLANE('',#35370);
#1798=PLANE('',#35371);
#1799=PLANE('',#35372);
#1800=PLANE('',#35373);
#1801=PLANE('',#35374);
#1802=PLANE('',#35375);
#1803=PLANE('',#35376);
#1804=PLANE('',#35377);
#1805=PLANE('',#35378);
#1806=PLANE('',#35379);
#1807=PLANE('',#35380);
#1808=PLANE('',#35381);
#1809=PLANE('',#35382);
#1810=PLANE('',#35383);
#1811=PLANE('',#35384);
#1812=PLANE('',#35385);
#1813=PLANE('',#35386);
#1814=PLANE('',#35387);
#1815=PLANE('',#35388);
#1816=PLANE('',#35389);
#1817=PLANE('',#35390);
#1818=PLANE('',#35391);
#1819=PLANE('',#35392);
#1820=PLANE('',#35393);
#1821=PLANE('',#35394);
#1822=PLANE('',#35395);
#1823=PLANE('',#35396);
#1824=PLANE('',#35397);
#1825=PLANE('',#35398);
#1826=PLANE('',#35399);
#1827=PLANE('',#35400);
#1828=PLANE('',#35401);
#1829=PLANE('',#35402);
#1830=PLANE('',#35403);
#1831=PLANE('',#35404);
#1832=PLANE('',#35405);
#1833=PLANE('',#35406);
#1834=PLANE('',#35407);
#1835=PLANE('',#35408);
#1836=PLANE('',#35409);
#1837=PLANE('',#35410);
#1838=PLANE('',#35411);
#1839=PLANE('',#35412);
#1840=PLANE('',#35413);
#1841=PLANE('',#35414);
#1842=PLANE('',#35415);
#1843=PLANE('',#35416);
#1844=PLANE('',#35417);
#1845=PLANE('',#35418);
#1846=PLANE('',#35419);
#1847=PLANE('',#35420);
#1848=PLANE('',#35421);
#1849=PLANE('',#35422);
#1850=PLANE('',#35423);
#1851=PLANE('',#35424);
#1852=PLANE('',#35425);
#1853=PLANE('',#35426);
#1854=PLANE('',#35427);
#1855=PLANE('',#35428);
#1856=PLANE('',#35429);
#1857=PLANE('',#35430);
#1858=PLANE('',#35431);
#1859=PLANE('',#35432);
#1860=PLANE('',#35433);
#1861=PLANE('',#35434);
#1862=PLANE('',#35435);
#1863=PLANE('',#35436);
#1864=PLANE('',#35437);
#1865=PLANE('',#35438);
#1866=PLANE('',#35439);
#1867=PLANE('',#35440);
#1868=PLANE('',#35441);
#1869=PLANE('',#35442);
#1870=PLANE('',#35443);
#1871=PLANE('',#35444);
#1872=PLANE('',#35445);
#1873=PLANE('',#35446);
#1874=PLANE('',#35447);
#1875=PLANE('',#35448);
#1876=PLANE('',#35449);
#1877=PLANE('',#35450);
#1878=PLANE('',#35451);
#1879=PLANE('',#35452);
#1880=PLANE('',#35453);
#1881=PLANE('',#35454);
#1882=PLANE('',#35455);
#1883=PLANE('',#35456);
#1884=PLANE('',#35457);
#1885=PLANE('',#35458);
#1886=PLANE('',#35459);
#1887=PLANE('',#35460);
#1888=PLANE('',#35461);
#1889=PLANE('',#35462);
#1890=PLANE('',#35463);
#1891=PLANE('',#35464);
#1892=PLANE('',#35465);
#1893=PLANE('',#35466);
#1894=PLANE('',#35467);
#1895=PLANE('',#35468);
#1896=PLANE('',#35469);
#1897=PLANE('',#35470);
#1898=PLANE('',#35471);
#1899=PLANE('',#35472);
#1900=PLANE('',#35473);
#1901=PLANE('',#35474);
#1902=PLANE('',#35475);
#1903=PLANE('',#35476);
#1904=PLANE('',#35477);
#1905=PLANE('',#35478);
#1906=PLANE('',#35479);
#1907=PLANE('',#35480);
#1908=PLANE('',#35481);
#1909=PLANE('',#35482);
#1910=PLANE('',#35483);
#1911=PLANE('',#35484);
#1912=PLANE('',#35485);
#1913=PLANE('',#35486);
#1914=PLANE('',#35487);
#1915=PLANE('',#35488);
#1916=PLANE('',#35489);
#1917=PLANE('',#35490);
#1918=PLANE('',#35491);
#1919=PLANE('',#35492);
#1920=PLANE('',#35493);
#1921=PLANE('',#35494);
#1922=PLANE('',#35495);
#1923=PLANE('',#35496);
#1924=PLANE('',#35497);
#1925=PLANE('',#35498);
#1926=PLANE('',#35499);
#1927=PLANE('',#35500);
#1928=PLANE('',#35501);
#1929=PLANE('',#35502);
#1930=PLANE('',#35503);
#1931=PLANE('',#35504);
#1932=PLANE('',#35505);
#1933=PLANE('',#35506);
#1934=PLANE('',#35507);
#1935=PLANE('',#35508);
#1936=PLANE('',#35509);
#1937=PLANE('',#35510);
#1938=PLANE('',#35511);
#1939=PLANE('',#35512);
#1940=PLANE('',#35513);
#1941=PLANE('',#35514);
#1942=PLANE('',#35515);
#1943=PLANE('',#35516);
#1944=PLANE('',#35517);
#1945=PLANE('',#35518);
#1946=PLANE('',#35519);
#1947=PLANE('',#35520);
#1948=PLANE('',#35521);
#1949=PLANE('',#35522);
#1950=PLANE('',#35523);
#1951=PLANE('',#35524);
#1952=PLANE('',#35525);
#1953=PLANE('',#35526);
#1954=PLANE('',#35527);
#1955=PLANE('',#35528);
#1956=PLANE('',#35529);
#1957=PLANE('',#35530);
#1958=PLANE('',#35531);
#1959=PLANE('',#35532);
#1960=PLANE('',#35533);
#1961=PLANE('',#35534);
#1962=PLANE('',#35535);
#1963=PLANE('',#35536);
#1964=PLANE('',#35537);
#1965=PLANE('',#35538);
#1966=PLANE('',#35539);
#1967=PLANE('',#35540);
#1968=PLANE('',#35541);
#1969=PLANE('',#35542);
#1970=PLANE('',#35543);
#1971=PLANE('',#35544);
#1972=PLANE('',#35545);
#1973=PLANE('',#35546);
#1974=PLANE('',#35547);
#1975=PLANE('',#35548);
#1976=PLANE('',#35549);
#1977=PLANE('',#35550);
#1978=PLANE('',#35551);
#1979=PLANE('',#35552);
#1980=PLANE('',#35553);
#1981=PLANE('',#35554);
#1982=PLANE('',#35555);
#1983=PLANE('',#35556);
#1984=PLANE('',#35557);
#1985=PLANE('',#35558);
#1986=PLANE('',#35559);
#1987=PLANE('',#35560);
#1988=PLANE('',#35561);
#1989=PLANE('',#35562);
#1990=PLANE('',#35563);
#1991=PLANE('',#35564);
#1992=PLANE('',#35565);
#1993=PLANE('',#35566);
#1994=PLANE('',#35567);
#1995=PLANE('',#35568);
#1996=PLANE('',#35569);
#1997=PLANE('',#35570);
#1998=PLANE('',#35571);
#1999=PLANE('',#35572);
#2000=PLANE('',#35573);
#2001=PLANE('',#35574);
#2002=PLANE('',#35575);
#2003=PLANE('',#35576);
#2004=PLANE('',#35577);
#2005=PLANE('',#35578);
#2006=PLANE('',#35579);
#2007=PLANE('',#35580);
#2008=PLANE('',#35581);
#2009=PLANE('',#35582);
#2010=PLANE('',#35583);
#2011=PLANE('',#35584);
#2012=PLANE('',#35585);
#2013=PLANE('',#35586);
#2014=PLANE('',#35587);
#2015=PLANE('',#35588);
#2016=PLANE('',#35589);
#2017=PLANE('',#35590);
#2018=PLANE('',#35591);
#2019=PLANE('',#35592);
#2020=PLANE('',#35593);
#2021=PLANE('',#35594);
#2022=PLANE('',#35595);
#2023=PLANE('',#35596);
#2024=PLANE('',#35597);
#2025=PLANE('',#35598);
#2026=PLANE('',#35599);
#2027=PLANE('',#35600);
#2028=PLANE('',#35601);
#2029=PLANE('',#35602);
#2030=PLANE('',#35603);
#2031=PLANE('',#35604);
#2032=PLANE('',#35605);
#2033=PLANE('',#35606);
#2034=PLANE('',#35607);
#2035=PLANE('',#35608);
#2036=PLANE('',#35609);
#2037=PLANE('',#35610);
#2038=PLANE('',#35611);
#2039=PLANE('',#35612);
#2040=PLANE('',#35613);
#2041=PLANE('',#35614);
#2042=PLANE('',#35615);
#2043=PLANE('',#35616);
#2044=PLANE('',#35617);
#2045=PLANE('',#35618);
#2046=PLANE('',#35619);
#2047=PLANE('',#35620);
#2048=PLANE('',#35621);
#2049=PLANE('',#35622);
#2050=PLANE('',#35623);
#2051=PLANE('',#35624);
#2052=PLANE('',#35625);
#2053=PLANE('',#35626);
#2054=PLANE('',#35627);
#2055=PLANE('',#35628);
#2056=PLANE('',#35629);
#2057=PLANE('',#35630);
#2058=PLANE('',#35631);
#2059=PLANE('',#35632);
#2060=PLANE('',#35633);
#2061=PLANE('',#35634);
#2062=PLANE('',#35635);
#2063=PLANE('',#35636);
#2064=PLANE('',#35637);
#2065=PLANE('',#35638);
#2066=PLANE('',#35639);
#2067=PLANE('',#35640);
#2068=PLANE('',#35641);
#2069=PLANE('',#35642);
#2070=PLANE('',#35643);
#2071=PLANE('',#35644);
#2072=PLANE('',#35645);
#2073=PLANE('',#35646);
#2074=PLANE('',#35647);
#2075=PLANE('',#35648);
#2076=PLANE('',#35649);
#2077=PLANE('',#35650);
#2078=PLANE('',#35651);
#2079=PLANE('',#35652);
#2080=PLANE('',#35653);
#2081=PLANE('',#35654);
#2082=PLANE('',#35655);
#2083=PLANE('',#35656);
#2084=PLANE('',#35657);
#2085=PLANE('',#35658);
#2086=PLANE('',#35659);
#2087=PLANE('',#35660);
#2088=PLANE('',#35661);
#2089=PLANE('',#35662);
#2090=PLANE('',#35663);
#2091=PLANE('',#35664);
#2092=PLANE('',#35665);
#2093=PLANE('',#35666);
#2094=PLANE('',#35667);
#2095=PLANE('',#35668);
#2096=PLANE('',#35669);
#2097=PLANE('',#35670);
#2098=PLANE('',#35671);
#2099=PLANE('',#35672);
#2100=PLANE('',#35673);
#2101=PLANE('',#35674);
#2102=PLANE('',#35675);
#2103=PLANE('',#35676);
#2104=PLANE('',#35677);
#2105=PLANE('',#35678);
#2106=PLANE('',#35679);
#2107=PLANE('',#35680);
#2108=PLANE('',#35681);
#2109=PLANE('',#35682);
#2110=PLANE('',#35683);
#2111=PLANE('',#35684);
#2112=PLANE('',#35685);
#2113=PLANE('',#35686);
#2114=PLANE('',#35687);
#2115=PLANE('',#35688);
#2116=PLANE('',#35689);
#2117=PLANE('',#35690);
#2118=PLANE('',#35691);
#2119=PLANE('',#35692);
#2120=PLANE('',#35693);
#2121=PLANE('',#35694);
#2122=PLANE('',#35695);
#2123=PLANE('',#35696);
#2124=PLANE('',#35697);
#2125=PLANE('',#35698);
#2126=PLANE('',#35699);
#2127=PLANE('',#35700);
#2128=PLANE('',#35701);
#2129=PLANE('',#35702);
#2130=PLANE('',#35703);
#2131=PLANE('',#35704);
#2132=PLANE('',#35705);
#2133=PLANE('',#35706);
#2134=PLANE('',#35707);
#2135=PLANE('',#35708);
#2136=PLANE('',#35709);
#2137=PLANE('',#35710);
#2138=PLANE('',#35711);
#2139=PLANE('',#35712);
#2140=PLANE('',#35713);
#2141=PLANE('',#35714);
#2142=PLANE('',#35715);
#2143=PLANE('',#35716);
#2144=PLANE('',#35717);
#2145=PLANE('',#35718);
#2146=PLANE('',#35719);
#2147=PLANE('',#35720);
#2148=PLANE('',#35721);
#2149=PLANE('',#35722);
#2150=PLANE('',#35723);
#2151=PLANE('',#35724);
#2152=PLANE('',#35725);
#2153=PLANE('',#35726);
#2154=PLANE('',#35727);
#2155=PLANE('',#35728);
#2156=PLANE('',#35729);
#2157=PLANE('',#35730);
#2158=PLANE('',#35731);
#2159=PLANE('',#35732);
#2160=PLANE('',#35733);
#2161=PLANE('',#35734);
#2162=PLANE('',#35735);
#2163=PLANE('',#35736);
#2164=PLANE('',#35737);
#2165=PLANE('',#35738);
#2166=PLANE('',#35739);
#2167=PLANE('',#35740);
#2168=PLANE('',#35741);
#2169=PLANE('',#35742);
#2170=PLANE('',#35743);
#2171=PLANE('',#35744);
#2172=PLANE('',#35745);
#2173=PLANE('',#35746);
#2174=PLANE('',#35747);
#2175=PLANE('',#35748);
#2176=PLANE('',#35749);
#2177=PLANE('',#35750);
#2178=PLANE('',#35751);
#2179=PLANE('',#35752);
#2180=PLANE('',#35753);
#2181=PLANE('',#35754);
#2182=PLANE('',#35755);
#2183=PLANE('',#35756);
#2184=PLANE('',#35757);
#2185=PLANE('',#35758);
#2186=PLANE('',#35759);
#2187=PLANE('',#35760);
#2188=PLANE('',#35761);
#2189=PLANE('',#35762);
#2190=PLANE('',#35763);
#2191=PLANE('',#35764);
#2192=PLANE('',#35765);
#2193=PLANE('',#35766);
#2194=PLANE('',#35767);
#2195=PLANE('',#35768);
#2196=PLANE('',#35769);
#2197=PLANE('',#35770);
#2198=PLANE('',#35771);
#2199=PLANE('',#35772);
#2200=PLANE('',#35773);
#2201=PLANE('',#35774);
#2202=PLANE('',#35775);
#2203=PLANE('',#35776);
#2204=PLANE('',#35777);
#2205=PLANE('',#35778);
#2206=PLANE('',#35779);
#2207=PLANE('',#35780);
#2208=PLANE('',#35781);
#2209=PLANE('',#35782);
#2210=PLANE('',#35783);
#2211=PLANE('',#35784);
#2212=PLANE('',#35785);
#2213=PLANE('',#35786);
#2214=PLANE('',#35787);
#2215=PLANE('',#35788);
#2216=PLANE('',#35789);
#2217=PLANE('',#35790);
#2218=PLANE('',#35791);
#2219=PLANE('',#35792);
#2220=PLANE('',#35793);
#2221=PLANE('',#35794);
#2222=PLANE('',#35795);
#2223=PLANE('',#35796);
#2224=PLANE('',#35797);
#2225=PLANE('',#35798);
#2226=PLANE('',#35799);
#2227=PLANE('',#35800);
#2228=PLANE('',#35801);
#2229=PLANE('',#35802);
#2230=PLANE('',#35803);
#2231=PLANE('',#35804);
#2232=PLANE('',#35805);
#2233=PLANE('',#35806);
#2234=PLANE('',#35807);
#2235=PLANE('',#35808);
#2236=PLANE('',#35809);
#2237=PLANE('',#35810);
#2238=PLANE('',#35811);
#2239=PLANE('',#35812);
#2240=PLANE('',#35813);
#2241=PLANE('',#35814);
#2242=PLANE('',#35815);
#2243=PLANE('',#35816);
#2244=PLANE('',#35817);
#2245=PLANE('',#35818);
#2246=PLANE('',#35819);
#2247=PLANE('',#35820);
#2248=PLANE('',#35821);
#2249=PLANE('',#35822);
#2250=PLANE('',#35823);
#2251=PLANE('',#35824);
#2252=PLANE('',#35825);
#2253=PLANE('',#35826);
#2254=PLANE('',#35827);
#2255=PLANE('',#35828);
#2256=PLANE('',#35829);
#2257=PLANE('',#35830);
#2258=PLANE('',#35831);
#2259=PLANE('',#35832);
#2260=PLANE('',#35833);
#2261=PLANE('',#35834);
#2262=PLANE('',#35835);
#2263=PLANE('',#35836);
#2264=PLANE('',#35837);
#2265=PLANE('',#35838);
#2266=PLANE('',#35839);
#2267=PLANE('',#35840);
#2268=PLANE('',#35841);
#2269=PLANE('',#35842);
#2270=PLANE('',#35843);
#2271=PLANE('',#35844);
#2272=PLANE('',#35845);
#2273=PLANE('',#35846);
#2274=PLANE('',#35847);
#2275=PLANE('',#35848);
#2276=PLANE('',#35849);
#2277=PLANE('',#35850);
#2278=PLANE('',#35851);
#2279=PLANE('',#35852);
#2280=PLANE('',#35853);
#2281=PLANE('',#35854);
#2282=PLANE('',#35855);
#2283=PLANE('',#35856);
#2284=PLANE('',#35857);
#2285=PLANE('',#35858);
#2286=PLANE('',#35859);
#2287=PLANE('',#35860);
#2288=PLANE('',#35861);
#2289=PLANE('',#35862);
#2290=PLANE('',#35863);
#2291=PLANE('',#35864);
#2292=PLANE('',#35865);
#2293=PLANE('',#35866);
#2294=PLANE('',#35867);
#2295=PLANE('',#35868);
#2296=PLANE('',#35869);
#2297=PLANE('',#35870);
#2298=PLANE('',#35871);
#2299=PLANE('',#35872);
#2300=PLANE('',#35873);
#2301=PLANE('',#35874);
#2302=PLANE('',#35875);
#2303=PLANE('',#35876);
#2304=PLANE('',#35877);
#2305=PLANE('',#35878);
#2306=PLANE('',#35879);
#2307=PLANE('',#35880);
#2308=PLANE('',#35881);
#2309=PLANE('',#35882);
#2310=PLANE('',#35883);
#2311=PLANE('',#35884);
#2312=PLANE('',#35885);
#2313=PLANE('',#35886);
#2314=PLANE('',#35887);
#2315=PLANE('',#35888);
#2316=PLANE('',#35889);
#2317=PLANE('',#35890);
#2318=PLANE('',#35891);
#2319=PLANE('',#35892);
#2320=PLANE('',#35893);
#2321=PLANE('',#35894);
#2322=PLANE('',#35895);
#2323=PLANE('',#35896);
#2324=PLANE('',#35897);
#2325=PLANE('',#35898);
#2326=PLANE('',#35899);
#2327=PLANE('',#35900);
#2328=PLANE('',#35901);
#2329=PLANE('',#35902);
#2330=PLANE('',#35903);
#2331=PLANE('',#35904);
#2332=PLANE('',#35905);
#2333=PLANE('',#35906);
#2334=PLANE('',#35907);
#2335=PLANE('',#35908);
#2336=PLANE('',#35909);
#2337=PLANE('',#35910);
#2338=PLANE('',#35911);
#2339=PLANE('',#35912);
#2340=PLANE('',#35913);
#2341=PLANE('',#35914);
#2342=PLANE('',#35915);
#2343=PLANE('',#35916);
#2344=PLANE('',#35917);
#2345=PLANE('',#35918);
#2346=PLANE('',#35919);
#2347=PLANE('',#35930);
#2348=PLANE('',#35931);
#2349=PLANE('',#35932);
#2350=PLANE('',#35933);
#2351=PLANE('',#35934);
#2352=PLANE('',#35935);
#2353=PLANE('',#35936);
#2354=PLANE('',#35937);
#2355=PLANE('',#35938);
#2356=PLANE('',#35939);
#2357=PLANE('',#35940);
#2358=PLANE('',#35941);
#2359=PLANE('',#35942);
#2360=PLANE('',#35943);
#2361=PLANE('',#35944);
#2362=PLANE('',#35945);
#2363=PLANE('',#35946);
#2364=PLANE('',#35947);
#2365=PLANE('',#35948);
#2366=PLANE('',#35949);
#2367=PLANE('',#35950);
#2368=PLANE('',#35951);
#2369=PLANE('',#35952);
#2370=PLANE('',#35953);
#2371=PLANE('',#35954);
#2372=PLANE('',#35955);
#2373=PLANE('',#35956);
#2374=PLANE('',#35957);
#2375=PLANE('',#35958);
#2376=PLANE('',#35959);
#2377=PLANE('',#35971);
#2378=PLANE('',#35978);
#2379=PLANE('',#35979);
#2380=PLANE('',#35980);
#2381=PLANE('',#35981);
#2382=PLANE('',#35982);
#2383=PLANE('',#35983);
#2384=PLANE('',#35984);
#2385=PLANE('',#35985);
#2386=PLANE('',#35986);
#2387=PLANE('',#35987);
#2388=PLANE('',#35988);
#2389=PLANE('',#35989);
#2390=PLANE('',#35990);
#2391=PLANE('',#35991);
#2392=PLANE('',#35992);
#2393=PLANE('',#35993);
#2394=PLANE('',#35994);
#2395=PLANE('',#35995);
#2396=PLANE('',#35996);
#2397=PLANE('',#35997);
#2398=PLANE('',#35998);
#2399=PLANE('',#35999);
#2400=PLANE('',#36000);
#2401=PLANE('',#36001);
#2402=PLANE('',#36002);
#2403=PLANE('',#36003);
#2404=PLANE('',#36004);
#2405=PLANE('',#36005);
#2406=PLANE('',#36006);
#2407=PLANE('',#36007);
#2408=PLANE('',#36008);
#2409=PLANE('',#36009);
#2410=PLANE('',#36010);
#2411=PLANE('',#36011);
#2412=PLANE('',#36012);
#2413=PLANE('',#36013);
#2414=PLANE('',#36014);
#2415=PLANE('',#36015);
#2416=PLANE('',#36016);
#2417=PLANE('',#36017);
#2418=PLANE('',#36018);
#2419=PLANE('',#36019);
#2420=PLANE('',#36020);
#2421=PLANE('',#36021);
#2422=PLANE('',#36022);
#2423=PLANE('',#36023);
#2424=PLANE('',#36024);
#2425=PLANE('',#36025);
#2426=PLANE('',#36026);
#2427=PLANE('',#36027);
#2428=PLANE('',#36028);
#2429=PLANE('',#36029);
#2430=PLANE('',#36030);
#2431=PLANE('',#36031);
#2432=PLANE('',#36032);
#2433=PLANE('',#36033);
#2434=PLANE('',#36034);
#2435=PLANE('',#36035);
#2436=PLANE('',#36036);
#2437=PLANE('',#36037);
#2438=PLANE('',#36038);
#2439=PLANE('',#36039);
#2440=PLANE('',#36040);
#2441=PLANE('',#36041);
#2442=PLANE('',#36042);
#2443=PLANE('',#36043);
#2444=PLANE('',#36044);
#2445=PLANE('',#36045);
#2446=PLANE('',#36046);
#2447=PLANE('',#36047);
#2448=PLANE('',#36048);
#2449=PLANE('',#36049);
#2450=PLANE('',#36050);
#2451=PLANE('',#36051);
#2452=PLANE('',#36052);
#2453=PLANE('',#36053);
#2454=PLANE('',#36054);
#2455=PLANE('',#36055);
#2456=PLANE('',#36056);
#2457=PLANE('',#36057);
#2458=PLANE('',#36058);
#2459=PLANE('',#36059);
#2460=PLANE('',#36060);
#2461=PLANE('',#36061);
#2462=PLANE('',#36062);
#2463=PLANE('',#36063);
#2464=PLANE('',#36064);
#2465=PLANE('',#36065);
#2466=PLANE('',#36066);
#2467=PLANE('',#36067);
#2468=PLANE('',#36068);
#2469=PLANE('',#36069);
#2470=PLANE('',#36070);
#2471=PLANE('',#36071);
#2472=PLANE('',#36072);
#2473=PLANE('',#36073);
#2474=PLANE('',#36074);
#2475=PLANE('',#36075);
#2476=PLANE('',#36076);
#2477=PLANE('',#36077);
#2478=PLANE('',#36078);
#2479=PLANE('',#36079);
#2480=PLANE('',#36080);
#2481=PLANE('',#36081);
#2482=PLANE('',#36082);
#2483=PLANE('',#36083);
#2484=PLANE('',#36084);
#2485=PLANE('',#36085);
#2486=PLANE('',#36086);
#2487=PLANE('',#36087);
#2488=PLANE('',#36088);
#2489=PLANE('',#36089);
#2490=PLANE('',#36090);
#2491=PLANE('',#36091);
#2492=PLANE('',#36092);
#2493=PLANE('',#36093);
#2494=PLANE('',#36094);
#2495=PLANE('',#36095);
#2496=PLANE('',#36096);
#2497=PLANE('',#36097);
#2498=PLANE('',#36098);
#2499=PLANE('',#36099);
#2500=PLANE('',#36100);
#2501=PLANE('',#36101);
#2502=PLANE('',#36102);
#2503=PLANE('',#36103);
#2504=PLANE('',#36104);
#2505=PLANE('',#36105);
#2506=PLANE('',#36106);
#2507=PLANE('',#36107);
#2508=PLANE('',#36108);
#2509=PLANE('',#36109);
#2510=PLANE('',#36110);
#2511=PLANE('',#36111);
#2512=PLANE('',#36112);
#2513=PLANE('',#36113);
#2514=PLANE('',#36114);
#2515=PLANE('',#36115);
#2516=PLANE('',#36116);
#2517=PLANE('',#36117);
#2518=PLANE('',#36118);
#2519=PLANE('',#36119);
#2520=PLANE('',#36120);
#2521=PLANE('',#36121);
#2522=PLANE('',#36145);
#2523=PLANE('',#36148);
#2524=PLANE('',#36151);
#2525=PLANE('',#36154);
#2526=PLANE('',#36161);
#2992=CYLINDRICAL_SURFACE('',#34375,40.);
#2993=CYLINDRICAL_SURFACE('',#34385,26.);
#2994=CYLINDRICAL_SURFACE('',#34428,136.);
#2995=CYLINDRICAL_SURFACE('',#34894,15.);
#2996=CYLINDRICAL_SURFACE('',#34896,52.);
#2997=CYLINDRICAL_SURFACE('',#34898,15.);
#2998=CYLINDRICAL_SURFACE('',#34900,52.);
#2999=CYLINDRICAL_SURFACE('',#34902,15.);
#3000=CYLINDRICAL_SURFACE('',#34904,52.);
#3001=CYLINDRICAL_SURFACE('',#35928,127.);
#3002=CYLINDRICAL_SURFACE('',#35965,139.);
#3003=CYLINDRICAL_SURFACE('',#36122,7.18);
#3004=CYLINDRICAL_SURFACE('',#36124,7.18);
#3005=CYLINDRICAL_SURFACE('',#36126,7.18);
#3006=CYLINDRICAL_SURFACE('',#36128,7.18);
#3007=CYLINDRICAL_SURFACE('',#36130,7.18);
#3008=CYLINDRICAL_SURFACE('',#36135,23.);
#3009=CYLINDRICAL_SURFACE('',#36137,15.);
#3010=CYLINDRICAL_SURFACE('',#36139,52.);
#3011=CYLINDRICAL_SURFACE('',#36141,15.);
#3012=CYLINDRICAL_SURFACE('',#36143,52.);
#3013=CYLINDRICAL_SURFACE('',#36146,25.16);
#3014=CYLINDRICAL_SURFACE('',#36149,27.);
#3015=CYLINDRICAL_SURFACE('',#36152,29.58);
#3016=CYLINDRICAL_SURFACE('',#36156,32.6);
#3139=FACE_OUTER_BOUND('',#5234,.T.);
#3140=FACE_OUTER_BOUND('',#5235,.T.);
#3141=FACE_OUTER_BOUND('',#5236,.T.);
#3142=FACE_OUTER_BOUND('',#5237,.T.);
#3143=FACE_OUTER_BOUND('',#5238,.T.);
#3144=FACE_OUTER_BOUND('',#5240,.T.);
#3145=FACE_OUTER_BOUND('',#5241,.T.);
#3146=FACE_OUTER_BOUND('',#5242,.T.);
#3147=FACE_OUTER_BOUND('',#5244,.T.);
#3148=FACE_OUTER_BOUND('',#5245,.T.);
#3149=FACE_OUTER_BOUND('',#5246,.T.);
#3150=FACE_OUTER_BOUND('',#5248,.T.);
#3151=FACE_OUTER_BOUND('',#5249,.T.);
#3152=FACE_OUTER_BOUND('',#5250,.T.);
#3153=FACE_OUTER_BOUND('',#5251,.T.);
#3154=FACE_OUTER_BOUND('',#5252,.T.);
#3155=FACE_OUTER_BOUND('',#5253,.T.);
#3156=FACE_OUTER_BOUND('',#5254,.T.);
#3157=FACE_OUTER_BOUND('',#5255,.T.);
#3158=FACE_OUTER_BOUND('',#5256,.T.);
#3159=FACE_OUTER_BOUND('',#5257,.T.);
#3160=FACE_OUTER_BOUND('',#5258,.T.);
#3161=FACE_OUTER_BOUND('',#5330,.T.);
#3162=FACE_OUTER_BOUND('',#5331,.T.);
#3163=FACE_OUTER_BOUND('',#5332,.T.);
#3164=FACE_OUTER_BOUND('',#5333,.T.);
#3165=FACE_OUTER_BOUND('',#5334,.T.);
#3166=FACE_OUTER_BOUND('',#5335,.T.);
#3167=FACE_OUTER_BOUND('',#5336,.T.);
#3168=FACE_OUTER_BOUND('',#5337,.T.);
#3169=FACE_OUTER_BOUND('',#5338,.T.);
#3170=FACE_OUTER_BOUND('',#5339,.T.);
#3171=FACE_OUTER_BOUND('',#5340,.T.);
#3172=FACE_OUTER_BOUND('',#5341,.T.);
#3173=FACE_OUTER_BOUND('',#5342,.T.);
#3174=FACE_OUTER_BOUND('',#5343,.T.);
#3175=FACE_OUTER_BOUND('',#5344,.T.);
#3176=FACE_OUTER_BOUND('',#5345,.T.);
#3177=FACE_OUTER_BOUND('',#5346,.T.);
#3178=FACE_OUTER_BOUND('',#5353,.T.);
#3179=FACE_OUTER_BOUND('',#5354,.T.);
#3180=FACE_OUTER_BOUND('',#5355,.T.);
#3181=FACE_OUTER_BOUND('',#5356,.T.);
#3182=FACE_OUTER_BOUND('',#5357,.T.);
#3183=FACE_OUTER_BOUND('',#5358,.T.);
#3184=FACE_OUTER_BOUND('',#5359,.T.);
#3185=FACE_OUTER_BOUND('',#5360,.T.);
#3186=FACE_OUTER_BOUND('',#5361,.T.);
#3187=FACE_OUTER_BOUND('',#5362,.T.);
#3188=FACE_OUTER_BOUND('',#5363,.T.);
#3189=FACE_OUTER_BOUND('',#5364,.T.);
#3190=FACE_OUTER_BOUND('',#5365,.T.);
#3191=FACE_OUTER_BOUND('',#5366,.T.);
#3192=FACE_OUTER_BOUND('',#5367,.T.);
#3193=FACE_OUTER_BOUND('',#5368,.T.);
#3194=FACE_OUTER_BOUND('',#5369,.T.);
#3195=FACE_OUTER_BOUND('',#5370,.T.);
#3196=FACE_OUTER_BOUND('',#5371,.T.);
#3197=FACE_OUTER_BOUND('',#5372,.T.);
#3198=FACE_OUTER_BOUND('',#5373,.T.);
#3199=FACE_OUTER_BOUND('',#5374,.T.);
#3200=FACE_OUTER_BOUND('',#5375,.T.);
#3201=FACE_OUTER_BOUND('',#5376,.T.);
#3202=FACE_OUTER_BOUND('',#5377,.T.);
#3203=FACE_OUTER_BOUND('',#5378,.T.);
#3204=FACE_OUTER_BOUND('',#5379,.T.);
#3205=FACE_OUTER_BOUND('',#5380,.T.);
#3206=FACE_OUTER_BOUND('',#5381,.T.);
#3207=FACE_OUTER_BOUND('',#5382,.T.);
#3208=FACE_OUTER_BOUND('',#5383,.T.);
#3209=FACE_OUTER_BOUND('',#5384,.T.);
#3210=FACE_OUTER_BOUND('',#5385,.T.);
#3211=FACE_OUTER_BOUND('',#5386,.T.);
#3212=FACE_OUTER_BOUND('',#5387,.T.);
#3213=FACE_OUTER_BOUND('',#5388,.T.);
#3214=FACE_OUTER_BOUND('',#5389,.T.);
#3215=FACE_OUTER_BOUND('',#5390,.T.);
#3216=FACE_OUTER_BOUND('',#5391,.T.);
#3217=FACE_OUTER_BOUND('',#5392,.T.);
#3218=FACE_OUTER_BOUND('',#5393,.T.);
#3219=FACE_OUTER_BOUND('',#5394,.T.);
#3220=FACE_OUTER_BOUND('',#5395,.T.);
#3221=FACE_OUTER_BOUND('',#5396,.T.);
#3222=FACE_OUTER_BOUND('',#5397,.T.);
#3223=FACE_OUTER_BOUND('',#5398,.T.);
#3224=FACE_OUTER_BOUND('',#5399,.T.);
#3225=FACE_OUTER_BOUND('',#5400,.T.);
#3226=FACE_OUTER_BOUND('',#5401,.T.);
#3227=FACE_OUTER_BOUND('',#5402,.T.);
#3228=FACE_OUTER_BOUND('',#5403,.T.);
#3229=FACE_OUTER_BOUND('',#5404,.T.);
#3230=FACE_OUTER_BOUND('',#5405,.T.);
#3231=FACE_OUTER_BOUND('',#5406,.T.);
#3232=FACE_OUTER_BOUND('',#5407,.T.);
#3233=FACE_OUTER_BOUND('',#5408,.T.);
#3234=FACE_OUTER_BOUND('',#5409,.T.);
#3235=FACE_OUTER_BOUND('',#5410,.T.);
#3236=FACE_OUTER_BOUND('',#5411,.T.);
#3237=FACE_OUTER_BOUND('',#5412,.T.);
#3238=FACE_OUTER_BOUND('',#5413,.T.);
#3239=FACE_OUTER_BOUND('',#5414,.T.);
#3240=FACE_OUTER_BOUND('',#5415,.T.);
#3241=FACE_OUTER_BOUND('',#5416,.T.);
#3242=FACE_OUTER_BOUND('',#5417,.T.);
#3243=FACE_OUTER_BOUND('',#5418,.T.);
#3244=FACE_OUTER_BOUND('',#5419,.T.);
#3245=FACE_OUTER_BOUND('',#5420,.T.);
#3246=FACE_OUTER_BOUND('',#5421,.T.);
#3247=FACE_OUTER_BOUND('',#5422,.T.);
#3248=FACE_OUTER_BOUND('',#5423,.T.);
#3249=FACE_OUTER_BOUND('',#5424,.T.);
#3250=FACE_OUTER_BOUND('',#5425,.T.);
#3251=FACE_OUTER_BOUND('',#5426,.T.);
#3252=FACE_OUTER_BOUND('',#5427,.T.);
#3253=FACE_OUTER_BOUND('',#5428,.T.);
#3254=FACE_OUTER_BOUND('',#5429,.T.);
#3255=FACE_OUTER_BOUND('',#5430,.T.);
#3256=FACE_OUTER_BOUND('',#5431,.T.);
#3257=FACE_OUTER_BOUND('',#5432,.T.);
#3258=FACE_OUTER_BOUND('',#5433,.T.);
#3259=FACE_OUTER_BOUND('',#5434,.T.);
#3260=FACE_OUTER_BOUND('',#5435,.T.);
#3261=FACE_OUTER_BOUND('',#5436,.T.);
#3262=FACE_OUTER_BOUND('',#5437,.T.);
#3263=FACE_OUTER_BOUND('',#5438,.T.);
#3264=FACE_OUTER_BOUND('',#5439,.T.);
#3265=FACE_OUTER_BOUND('',#5440,.T.);
#3266=FACE_OUTER_BOUND('',#5441,.T.);
#3267=FACE_OUTER_BOUND('',#5442,.T.);
#3268=FACE_OUTER_BOUND('',#5443,.T.);
#3269=FACE_OUTER_BOUND('',#5444,.T.);
#3270=FACE_OUTER_BOUND('',#5445,.T.);
#3271=FACE_OUTER_BOUND('',#5446,.T.);
#3272=FACE_OUTER_BOUND('',#5447,.T.);
#3273=FACE_OUTER_BOUND('',#5448,.T.);
#3274=FACE_OUTER_BOUND('',#5449,.T.);
#3275=FACE_OUTER_BOUND('',#5450,.T.);
#3276=FACE_OUTER_BOUND('',#5451,.T.);
#3277=FACE_OUTER_BOUND('',#5452,.T.);
#3278=FACE_OUTER_BOUND('',#5453,.T.);
#3279=FACE_OUTER_BOUND('',#5454,.T.);
#3280=FACE_OUTER_BOUND('',#5455,.T.);
#3281=FACE_OUTER_BOUND('',#5456,.T.);
#3282=FACE_OUTER_BOUND('',#5457,.T.);
#3283=FACE_OUTER_BOUND('',#5458,.T.);
#3284=FACE_OUTER_BOUND('',#5459,.T.);
#3285=FACE_OUTER_BOUND('',#5460,.T.);
#3286=FACE_OUTER_BOUND('',#5461,.T.);
#3287=FACE_OUTER_BOUND('',#5462,.T.);
#3288=FACE_OUTER_BOUND('',#5463,.T.);
#3289=FACE_OUTER_BOUND('',#5464,.T.);
#3290=FACE_OUTER_BOUND('',#5465,.T.);
#3291=FACE_OUTER_BOUND('',#5466,.T.);
#3292=FACE_OUTER_BOUND('',#5467,.T.);
#3293=FACE_OUTER_BOUND('',#5468,.T.);
#3294=FACE_OUTER_BOUND('',#5469,.T.);
#3295=FACE_OUTER_BOUND('',#5470,.T.);
#3296=FACE_OUTER_BOUND('',#5471,.T.);
#3297=FACE_OUTER_BOUND('',#5472,.T.);
#3298=FACE_OUTER_BOUND('',#5473,.T.);
#3299=FACE_OUTER_BOUND('',#5474,.T.);
#3300=FACE_OUTER_BOUND('',#5475,.T.);
#3301=FACE_OUTER_BOUND('',#5476,.T.);
#3302=FACE_OUTER_BOUND('',#5477,.T.);
#3303=FACE_OUTER_BOUND('',#5478,.T.);
#3304=FACE_OUTER_BOUND('',#5479,.T.);
#3305=FACE_OUTER_BOUND('',#5480,.T.);
#3306=FACE_OUTER_BOUND('',#5481,.T.);
#3307=FACE_OUTER_BOUND('',#5482,.T.);
#3308=FACE_OUTER_BOUND('',#5483,.T.);
#3309=FACE_OUTER_BOUND('',#5484,.T.);
#3310=FACE_OUTER_BOUND('',#5485,.T.);
#3311=FACE_OUTER_BOUND('',#5486,.T.);
#3312=FACE_OUTER_BOUND('',#5487,.T.);
#3313=FACE_OUTER_BOUND('',#5488,.T.);
#3314=FACE_OUTER_BOUND('',#5489,.T.);
#3315=FACE_OUTER_BOUND('',#5490,.T.);
#3316=FACE_OUTER_BOUND('',#5491,.T.);
#3317=FACE_OUTER_BOUND('',#5492,.T.);
#3318=FACE_OUTER_BOUND('',#5493,.T.);
#3319=FACE_OUTER_BOUND('',#5494,.T.);
#3320=FACE_OUTER_BOUND('',#5495,.T.);
#3321=FACE_OUTER_BOUND('',#5496,.T.);
#3322=FACE_OUTER_BOUND('',#5497,.T.);
#3323=FACE_OUTER_BOUND('',#5498,.T.);
#3324=FACE_OUTER_BOUND('',#5499,.T.);
#3325=FACE_OUTER_BOUND('',#5500,.T.);
#3326=FACE_OUTER_BOUND('',#5501,.T.);
#3327=FACE_OUTER_BOUND('',#5502,.T.);
#3328=FACE_OUTER_BOUND('',#5503,.T.);
#3329=FACE_OUTER_BOUND('',#5504,.T.);
#3330=FACE_OUTER_BOUND('',#5505,.T.);
#3331=FACE_OUTER_BOUND('',#5506,.T.);
#3332=FACE_OUTER_BOUND('',#5507,.T.);
#3333=FACE_OUTER_BOUND('',#5508,.T.);
#3334=FACE_OUTER_BOUND('',#5509,.T.);
#3335=FACE_OUTER_BOUND('',#5510,.T.);
#3336=FACE_OUTER_BOUND('',#5511,.T.);
#3337=FACE_OUTER_BOUND('',#5512,.T.);
#3338=FACE_OUTER_BOUND('',#5513,.T.);
#3339=FACE_OUTER_BOUND('',#5514,.T.);
#3340=FACE_OUTER_BOUND('',#5515,.T.);
#3341=FACE_OUTER_BOUND('',#5516,.T.);
#3342=FACE_OUTER_BOUND('',#5517,.T.);
#3343=FACE_OUTER_BOUND('',#5518,.T.);
#3344=FACE_OUTER_BOUND('',#5519,.T.);
#3345=FACE_OUTER_BOUND('',#5520,.T.);
#3346=FACE_OUTER_BOUND('',#5521,.T.);
#3347=FACE_OUTER_BOUND('',#5522,.T.);
#3348=FACE_OUTER_BOUND('',#5523,.T.);
#3349=FACE_OUTER_BOUND('',#5524,.T.);
#3350=FACE_OUTER_BOUND('',#5525,.T.);
#3351=FACE_OUTER_BOUND('',#5526,.T.);
#3352=FACE_OUTER_BOUND('',#5527,.T.);
#3353=FACE_OUTER_BOUND('',#5528,.T.);
#3354=FACE_OUTER_BOUND('',#5529,.T.);
#3355=FACE_OUTER_BOUND('',#5530,.T.);
#3356=FACE_OUTER_BOUND('',#5531,.T.);
#3357=FACE_OUTER_BOUND('',#5532,.T.);
#3358=FACE_OUTER_BOUND('',#5533,.T.);
#3359=FACE_OUTER_BOUND('',#5534,.T.);
#3360=FACE_OUTER_BOUND('',#5535,.T.);
#3361=FACE_OUTER_BOUND('',#5536,.T.);
#3362=FACE_OUTER_BOUND('',#5537,.T.);
#3363=FACE_OUTER_BOUND('',#5538,.T.);
#3364=FACE_OUTER_BOUND('',#5539,.T.);
#3365=FACE_OUTER_BOUND('',#5540,.T.);
#3366=FACE_OUTER_BOUND('',#5541,.T.);
#3367=FACE_OUTER_BOUND('',#5542,.T.);
#3368=FACE_OUTER_BOUND('',#5543,.T.);
#3369=FACE_OUTER_BOUND('',#5544,.T.);
#3370=FACE_OUTER_BOUND('',#5545,.T.);
#3371=FACE_OUTER_BOUND('',#5546,.T.);
#3372=FACE_OUTER_BOUND('',#5547,.T.);
#3373=FACE_OUTER_BOUND('',#5548,.T.);
#3374=FACE_OUTER_BOUND('',#5549,.T.);
#3375=FACE_OUTER_BOUND('',#5550,.T.);
#3376=FACE_OUTER_BOUND('',#5551,.T.);
#3377=FACE_OUTER_BOUND('',#5552,.T.);
#3378=FACE_OUTER_BOUND('',#5553,.T.);
#3379=FACE_OUTER_BOUND('',#5554,.T.);
#3380=FACE_OUTER_BOUND('',#5555,.T.);
#3381=FACE_OUTER_BOUND('',#5556,.T.);
#3382=FACE_OUTER_BOUND('',#5557,.T.);
#3383=FACE_OUTER_BOUND('',#5558,.T.);
#3384=FACE_OUTER_BOUND('',#5559,.T.);
#3385=FACE_OUTER_BOUND('',#5560,.T.);
#3386=FACE_OUTER_BOUND('',#5561,.T.);
#3387=FACE_OUTER_BOUND('',#5562,.T.);
#3388=FACE_OUTER_BOUND('',#5563,.T.);
#3389=FACE_OUTER_BOUND('',#5564,.T.);
#3390=FACE_OUTER_BOUND('',#5565,.T.);
#3391=FACE_OUTER_BOUND('',#5566,.T.);
#3392=FACE_OUTER_BOUND('',#5567,.T.);
#3393=FACE_OUTER_BOUND('',#5568,.T.);
#3394=FACE_OUTER_BOUND('',#5569,.T.);
#3395=FACE_OUTER_BOUND('',#5570,.T.);
#3396=FACE_OUTER_BOUND('',#5571,.T.);
#3397=FACE_OUTER_BOUND('',#5572,.T.);
#3398=FACE_OUTER_BOUND('',#5573,.T.);
#3399=FACE_OUTER_BOUND('',#5574,.T.);
#3400=FACE_OUTER_BOUND('',#5575,.T.);
#3401=FACE_OUTER_BOUND('',#5576,.T.);
#3402=FACE_OUTER_BOUND('',#5577,.T.);
#3403=FACE_OUTER_BOUND('',#5578,.T.);
#3404=FACE_OUTER_BOUND('',#5579,.T.);
#3405=FACE_OUTER_BOUND('',#5580,.T.);
#3406=FACE_OUTER_BOUND('',#5581,.T.);
#3407=FACE_OUTER_BOUND('',#5582,.T.);
#3408=FACE_OUTER_BOUND('',#5583,.T.);
#3409=FACE_OUTER_BOUND('',#5584,.T.);
#3410=FACE_OUTER_BOUND('',#5585,.T.);
#3411=FACE_OUTER_BOUND('',#5586,.T.);
#3412=FACE_OUTER_BOUND('',#5587,.T.);
#3413=FACE_OUTER_BOUND('',#5588,.T.);
#3414=FACE_OUTER_BOUND('',#5589,.T.);
#3415=FACE_OUTER_BOUND('',#5590,.T.);
#3416=FACE_OUTER_BOUND('',#5591,.T.);
#3417=FACE_OUTER_BOUND('',#5592,.T.);
#3418=FACE_OUTER_BOUND('',#5593,.T.);
#3419=FACE_OUTER_BOUND('',#5594,.T.);
#3420=FACE_OUTER_BOUND('',#5595,.T.);
#3421=FACE_OUTER_BOUND('',#5596,.T.);
#3422=FACE_OUTER_BOUND('',#5597,.T.);
#3423=FACE_OUTER_BOUND('',#5598,.T.);
#3424=FACE_OUTER_BOUND('',#5599,.T.);
#3425=FACE_OUTER_BOUND('',#5600,.T.);
#3426=FACE_OUTER_BOUND('',#5601,.T.);
#3427=FACE_OUTER_BOUND('',#5602,.T.);
#3428=FACE_OUTER_BOUND('',#5603,.T.);
#3429=FACE_OUTER_BOUND('',#5604,.T.);
#3430=FACE_OUTER_BOUND('',#5605,.T.);
#3431=FACE_OUTER_BOUND('',#5606,.T.);
#3432=FACE_OUTER_BOUND('',#5607,.T.);
#3433=FACE_OUTER_BOUND('',#5608,.T.);
#3434=FACE_OUTER_BOUND('',#5609,.T.);
#3435=FACE_OUTER_BOUND('',#5610,.T.);
#3436=FACE_OUTER_BOUND('',#5611,.T.);
#3437=FACE_OUTER_BOUND('',#5612,.T.);
#3438=FACE_OUTER_BOUND('',#5613,.T.);
#3439=FACE_OUTER_BOUND('',#5614,.T.);
#3440=FACE_OUTER_BOUND('',#5615,.T.);
#3441=FACE_OUTER_BOUND('',#5616,.T.);
#3442=FACE_OUTER_BOUND('',#5617,.T.);
#3443=FACE_OUTER_BOUND('',#5618,.T.);
#3444=FACE_OUTER_BOUND('',#5619,.T.);
#3445=FACE_OUTER_BOUND('',#5620,.T.);
#3446=FACE_OUTER_BOUND('',#5621,.T.);
#3447=FACE_OUTER_BOUND('',#5622,.T.);
#3448=FACE_OUTER_BOUND('',#5623,.T.);
#3449=FACE_OUTER_BOUND('',#5624,.T.);
#3450=FACE_OUTER_BOUND('',#5625,.T.);
#3451=FACE_OUTER_BOUND('',#5626,.T.);
#3452=FACE_OUTER_BOUND('',#5627,.T.);
#3453=FACE_OUTER_BOUND('',#5628,.T.);
#3454=FACE_OUTER_BOUND('',#5629,.T.);
#3455=FACE_OUTER_BOUND('',#5630,.T.);
#3456=FACE_OUTER_BOUND('',#5631,.T.);
#3457=FACE_OUTER_BOUND('',#5632,.T.);
#3458=FACE_OUTER_BOUND('',#5633,.T.);
#3459=FACE_OUTER_BOUND('',#5634,.T.);
#3460=FACE_OUTER_BOUND('',#5635,.T.);
#3461=FACE_OUTER_BOUND('',#5636,.T.);
#3462=FACE_OUTER_BOUND('',#5637,.T.);
#3463=FACE_OUTER_BOUND('',#5638,.T.);
#3464=FACE_OUTER_BOUND('',#5639,.T.);
#3465=FACE_OUTER_BOUND('',#5640,.T.);
#3466=FACE_OUTER_BOUND('',#5641,.T.);
#3467=FACE_OUTER_BOUND('',#5642,.T.);
#3468=FACE_OUTER_BOUND('',#5643,.T.);
#3469=FACE_OUTER_BOUND('',#5644,.T.);
#3470=FACE_OUTER_BOUND('',#5645,.T.);
#3471=FACE_OUTER_BOUND('',#5646,.T.);
#3472=FACE_OUTER_BOUND('',#5647,.T.);
#3473=FACE_OUTER_BOUND('',#5648,.T.);
#3474=FACE_OUTER_BOUND('',#5649,.T.);
#3475=FACE_OUTER_BOUND('',#5650,.T.);
#3476=FACE_OUTER_BOUND('',#5651,.T.);
#3477=FACE_OUTER_BOUND('',#5652,.T.);
#3478=FACE_OUTER_BOUND('',#5653,.T.);
#3479=FACE_OUTER_BOUND('',#5654,.T.);
#3480=FACE_OUTER_BOUND('',#5655,.T.);
#3481=FACE_OUTER_BOUND('',#5656,.T.);
#3482=FACE_OUTER_BOUND('',#5657,.T.);
#3483=FACE_OUTER_BOUND('',#5658,.T.);
#3484=FACE_OUTER_BOUND('',#5659,.T.);
#3485=FACE_OUTER_BOUND('',#5660,.T.);
#3486=FACE_OUTER_BOUND('',#5661,.T.);
#3487=FACE_OUTER_BOUND('',#5662,.T.);
#3488=FACE_OUTER_BOUND('',#5663,.T.);
#3489=FACE_OUTER_BOUND('',#5664,.T.);
#3490=FACE_OUTER_BOUND('',#5665,.T.);
#3491=FACE_OUTER_BOUND('',#5666,.T.);
#3492=FACE_OUTER_BOUND('',#5667,.T.);
#3493=FACE_OUTER_BOUND('',#5668,.T.);
#3494=FACE_OUTER_BOUND('',#5669,.T.);
#3495=FACE_OUTER_BOUND('',#5670,.T.);
#3496=FACE_OUTER_BOUND('',#5671,.T.);
#3497=FACE_OUTER_BOUND('',#5672,.T.);
#3498=FACE_OUTER_BOUND('',#5673,.T.);
#3499=FACE_OUTER_BOUND('',#5674,.T.);
#3500=FACE_OUTER_BOUND('',#5675,.T.);
#3501=FACE_OUTER_BOUND('',#5676,.T.);
#3502=FACE_OUTER_BOUND('',#5677,.T.);
#3503=FACE_OUTER_BOUND('',#5678,.T.);
#3504=FACE_OUTER_BOUND('',#5679,.T.);
#3505=FACE_OUTER_BOUND('',#5680,.T.);
#3506=FACE_OUTER_BOUND('',#5681,.T.);
#3507=FACE_OUTER_BOUND('',#5682,.T.);
#3508=FACE_OUTER_BOUND('',#5683,.T.);
#3509=FACE_OUTER_BOUND('',#5684,.T.);
#3510=FACE_OUTER_BOUND('',#5685,.T.);
#3511=FACE_OUTER_BOUND('',#5686,.T.);
#3512=FACE_OUTER_BOUND('',#5687,.T.);
#3513=FACE_OUTER_BOUND('',#5688,.T.);
#3514=FACE_OUTER_BOUND('',#5689,.T.);
#3515=FACE_OUTER_BOUND('',#5690,.T.);
#3516=FACE_OUTER_BOUND('',#5691,.T.);
#3517=FACE_OUTER_BOUND('',#5692,.T.);
#3518=FACE_OUTER_BOUND('',#5693,.T.);
#3519=FACE_OUTER_BOUND('',#5694,.T.);
#3520=FACE_OUTER_BOUND('',#5695,.T.);
#3521=FACE_OUTER_BOUND('',#5696,.T.);
#3522=FACE_OUTER_BOUND('',#5697,.T.);
#3523=FACE_OUTER_BOUND('',#5698,.T.);
#3524=FACE_OUTER_BOUND('',#5699,.T.);
#3525=FACE_OUTER_BOUND('',#5700,.T.);
#3526=FACE_OUTER_BOUND('',#5701,.T.);
#3527=FACE_OUTER_BOUND('',#5702,.T.);
#3528=FACE_OUTER_BOUND('',#5703,.T.);
#3529=FACE_OUTER_BOUND('',#5704,.T.);
#3530=FACE_OUTER_BOUND('',#5705,.T.);
#3531=FACE_OUTER_BOUND('',#5706,.T.);
#3532=FACE_OUTER_BOUND('',#5707,.T.);
#3533=FACE_OUTER_BOUND('',#5708,.T.);
#3534=FACE_OUTER_BOUND('',#5709,.T.);
#3535=FACE_OUTER_BOUND('',#5710,.T.);
#3536=FACE_OUTER_BOUND('',#5711,.T.);
#3537=FACE_OUTER_BOUND('',#5712,.T.);
#3538=FACE_OUTER_BOUND('',#5713,.T.);
#3539=FACE_OUTER_BOUND('',#5714,.T.);
#3540=FACE_OUTER_BOUND('',#5715,.T.);
#3541=FACE_OUTER_BOUND('',#5716,.T.);
#3542=FACE_OUTER_BOUND('',#5717,.T.);
#3543=FACE_OUTER_BOUND('',#5718,.T.);
#3544=FACE_OUTER_BOUND('',#5719,.T.);
#3545=FACE_OUTER_BOUND('',#5720,.T.);
#3546=FACE_OUTER_BOUND('',#5721,.T.);
#3547=FACE_OUTER_BOUND('',#5722,.T.);
#3548=FACE_OUTER_BOUND('',#5723,.T.);
#3549=FACE_OUTER_BOUND('',#5724,.T.);
#3550=FACE_OUTER_BOUND('',#5725,.T.);
#3551=FACE_OUTER_BOUND('',#5726,.T.);
#3552=FACE_OUTER_BOUND('',#5727,.T.);
#3553=FACE_OUTER_BOUND('',#5728,.T.);
#3554=FACE_OUTER_BOUND('',#5729,.T.);
#3555=FACE_OUTER_BOUND('',#5730,.T.);
#3556=FACE_OUTER_BOUND('',#5731,.T.);
#3557=FACE_OUTER_BOUND('',#5732,.T.);
#3558=FACE_OUTER_BOUND('',#5733,.T.);
#3559=FACE_OUTER_BOUND('',#5734,.T.);
#3560=FACE_OUTER_BOUND('',#5735,.T.);
#3561=FACE_OUTER_BOUND('',#5736,.T.);
#3562=FACE_OUTER_BOUND('',#5737,.T.);
#3563=FACE_OUTER_BOUND('',#5738,.T.);
#3564=FACE_OUTER_BOUND('',#5739,.T.);
#3565=FACE_OUTER_BOUND('',#5740,.T.);
#3566=FACE_OUTER_BOUND('',#5741,.T.);
#3567=FACE_OUTER_BOUND('',#5742,.T.);
#3568=FACE_OUTER_BOUND('',#5743,.T.);
#3569=FACE_OUTER_BOUND('',#5744,.T.);
#3570=FACE_OUTER_BOUND('',#5745,.T.);
#3571=FACE_OUTER_BOUND('',#5746,.T.);
#3572=FACE_OUTER_BOUND('',#5747,.T.);
#3573=FACE_OUTER_BOUND('',#5748,.T.);
#3574=FACE_OUTER_BOUND('',#5749,.T.);
#3575=FACE_OUTER_BOUND('',#5750,.T.);
#3576=FACE_OUTER_BOUND('',#5751,.T.);
#3577=FACE_OUTER_BOUND('',#5752,.T.);
#3578=FACE_OUTER_BOUND('',#5753,.T.);
#3579=FACE_OUTER_BOUND('',#5754,.T.);
#3580=FACE_OUTER_BOUND('',#5755,.T.);
#3581=FACE_OUTER_BOUND('',#5756,.T.);
#3582=FACE_OUTER_BOUND('',#5757,.T.);
#3583=FACE_OUTER_BOUND('',#5758,.T.);
#3584=FACE_OUTER_BOUND('',#5759,.T.);
#3585=FACE_OUTER_BOUND('',#5760,.T.);
#3586=FACE_OUTER_BOUND('',#5761,.T.);
#3587=FACE_OUTER_BOUND('',#5762,.T.);
#3588=FACE_OUTER_BOUND('',#5763,.T.);
#3589=FACE_OUTER_BOUND('',#5764,.T.);
#3590=FACE_OUTER_BOUND('',#5765,.T.);
#3591=FACE_OUTER_BOUND('',#5766,.T.);
#3592=FACE_OUTER_BOUND('',#5767,.T.);
#3593=FACE_OUTER_BOUND('',#5768,.T.);
#3594=FACE_OUTER_BOUND('',#5769,.T.);
#3595=FACE_OUTER_BOUND('',#5770,.T.);
#3596=FACE_OUTER_BOUND('',#5771,.T.);
#3597=FACE_OUTER_BOUND('',#5772,.T.);
#3598=FACE_OUTER_BOUND('',#5773,.T.);
#3599=FACE_OUTER_BOUND('',#5774,.T.);
#3600=FACE_OUTER_BOUND('',#5775,.T.);
#3601=FACE_OUTER_BOUND('',#5776,.T.);
#3602=FACE_OUTER_BOUND('',#5777,.T.);
#3603=FACE_OUTER_BOUND('',#5778,.T.);
#3604=FACE_OUTER_BOUND('',#5779,.T.);
#3605=FACE_OUTER_BOUND('',#5780,.T.);
#3606=FACE_OUTER_BOUND('',#5781,.T.);
#3607=FACE_OUTER_BOUND('',#5782,.T.);
#3608=FACE_OUTER_BOUND('',#5783,.T.);
#3609=FACE_OUTER_BOUND('',#5784,.T.);
#3610=FACE_OUTER_BOUND('',#5785,.T.);
#3611=FACE_OUTER_BOUND('',#5786,.T.);
#3612=FACE_OUTER_BOUND('',#5787,.T.);
#3613=FACE_OUTER_BOUND('',#5788,.T.);
#3614=FACE_OUTER_BOUND('',#5789,.T.);
#3615=FACE_OUTER_BOUND('',#5790,.T.);
#3616=FACE_OUTER_BOUND('',#5791,.T.);
#3617=FACE_OUTER_BOUND('',#5792,.T.);
#3618=FACE_OUTER_BOUND('',#5793,.T.);
#3619=FACE_OUTER_BOUND('',#5794,.T.);
#3620=FACE_OUTER_BOUND('',#5795,.T.);
#3621=FACE_OUTER_BOUND('',#5796,.T.);
#3622=FACE_OUTER_BOUND('',#5797,.T.);
#3623=FACE_OUTER_BOUND('',#5798,.T.);
#3624=FACE_OUTER_BOUND('',#5799,.T.);
#3625=FACE_OUTER_BOUND('',#5800,.T.);
#3626=FACE_OUTER_BOUND('',#5801,.T.);
#3627=FACE_OUTER_BOUND('',#5802,.T.);
#3628=FACE_OUTER_BOUND('',#5803,.T.);
#3629=FACE_OUTER_BOUND('',#5804,.T.);
#3630=FACE_OUTER_BOUND('',#5805,.T.);
#3631=FACE_OUTER_BOUND('',#5806,.T.);
#3632=FACE_OUTER_BOUND('',#5807,.T.);
#3633=FACE_OUTER_BOUND('',#5808,.T.);
#3634=FACE_OUTER_BOUND('',#5809,.T.);
#3635=FACE_OUTER_BOUND('',#5810,.T.);
#3636=FACE_OUTER_BOUND('',#5811,.T.);
#3637=FACE_OUTER_BOUND('',#5812,.T.);
#3638=FACE_OUTER_BOUND('',#5813,.T.);
#3639=FACE_OUTER_BOUND('',#5814,.T.);
#3640=FACE_OUTER_BOUND('',#5815,.T.);
#3641=FACE_OUTER_BOUND('',#5816,.T.);
#3642=FACE_OUTER_BOUND('',#5817,.T.);
#3643=FACE_OUTER_BOUND('',#5818,.T.);
#3644=FACE_OUTER_BOUND('',#5819,.T.);
#3645=FACE_OUTER_BOUND('',#5820,.T.);
#3646=FACE_OUTER_BOUND('',#5821,.T.);
#3647=FACE_OUTER_BOUND('',#5822,.T.);
#3648=FACE_OUTER_BOUND('',#5823,.T.);
#3649=FACE_OUTER_BOUND('',#5824,.T.);
#3650=FACE_OUTER_BOUND('',#5825,.T.);
#3651=FACE_OUTER_BOUND('',#5826,.T.);
#3652=FACE_OUTER_BOUND('',#5827,.T.);
#3653=FACE_OUTER_BOUND('',#5828,.T.);
#3654=FACE_OUTER_BOUND('',#5829,.T.);
#3655=FACE_OUTER_BOUND('',#5830,.T.);
#3656=FACE_OUTER_BOUND('',#5831,.T.);
#3657=FACE_OUTER_BOUND('',#5832,.T.);
#3658=FACE_OUTER_BOUND('',#5833,.T.);
#3659=FACE_OUTER_BOUND('',#5834,.T.);
#3660=FACE_OUTER_BOUND('',#5835,.T.);
#3661=FACE_OUTER_BOUND('',#5836,.T.);
#3662=FACE_OUTER_BOUND('',#5837,.T.);
#3663=FACE_OUTER_BOUND('',#5838,.T.);
#3664=FACE_OUTER_BOUND('',#5839,.T.);
#3665=FACE_OUTER_BOUND('',#5840,.T.);
#3666=FACE_OUTER_BOUND('',#5841,.T.);
#3667=FACE_OUTER_BOUND('',#5842,.T.);
#3668=FACE_OUTER_BOUND('',#5843,.T.);
#3669=FACE_OUTER_BOUND('',#5844,.T.);
#3670=FACE_OUTER_BOUND('',#5845,.T.);
#3671=FACE_OUTER_BOUND('',#5846,.T.);
#3672=FACE_OUTER_BOUND('',#5847,.T.);
#3673=FACE_OUTER_BOUND('',#5848,.T.);
#3674=FACE_OUTER_BOUND('',#5849,.T.);
#3675=FACE_OUTER_BOUND('',#5850,.T.);
#3676=FACE_OUTER_BOUND('',#5851,.T.);
#3677=FACE_OUTER_BOUND('',#5852,.T.);
#3678=FACE_OUTER_BOUND('',#5853,.T.);
#3679=FACE_OUTER_BOUND('',#5854,.T.);
#3680=FACE_OUTER_BOUND('',#5855,.T.);
#3681=FACE_OUTER_BOUND('',#5856,.T.);
#3682=FACE_OUTER_BOUND('',#5857,.T.);
#3683=FACE_OUTER_BOUND('',#5858,.T.);
#3684=FACE_OUTER_BOUND('',#5859,.T.);
#3685=FACE_OUTER_BOUND('',#5860,.T.);
#3686=FACE_OUTER_BOUND('',#5861,.T.);
#3687=FACE_OUTER_BOUND('',#5862,.T.);
#3688=FACE_OUTER_BOUND('',#5863,.T.);
#3689=FACE_OUTER_BOUND('',#5864,.T.);
#3690=FACE_OUTER_BOUND('',#5865,.T.);
#3691=FACE_OUTER_BOUND('',#5866,.T.);
#3692=FACE_OUTER_BOUND('',#5867,.T.);
#3693=FACE_OUTER_BOUND('',#5868,.T.);
#3694=FACE_OUTER_BOUND('',#5869,.T.);
#3695=FACE_OUTER_BOUND('',#5870,.T.);
#3696=FACE_OUTER_BOUND('',#5871,.T.);
#3697=FACE_OUTER_BOUND('',#5872,.T.);
#3698=FACE_OUTER_BOUND('',#5873,.T.);
#3699=FACE_OUTER_BOUND('',#5874,.T.);
#3700=FACE_OUTER_BOUND('',#5875,.T.);
#3701=FACE_OUTER_BOUND('',#5876,.T.);
#3702=FACE_OUTER_BOUND('',#5877,.T.);
#3703=FACE_OUTER_BOUND('',#5878,.T.);
#3704=FACE_OUTER_BOUND('',#5879,.T.);
#3705=FACE_OUTER_BOUND('',#5880,.T.);
#3706=FACE_OUTER_BOUND('',#5881,.T.);
#3707=FACE_OUTER_BOUND('',#5882,.T.);
#3708=FACE_OUTER_BOUND('',#5883,.T.);
#3709=FACE_OUTER_BOUND('',#5884,.T.);
#3710=FACE_OUTER_BOUND('',#5885,.T.);
#3711=FACE_OUTER_BOUND('',#5886,.T.);
#3712=FACE_OUTER_BOUND('',#5887,.T.);
#3713=FACE_OUTER_BOUND('',#5888,.T.);
#3714=FACE_OUTER_BOUND('',#5889,.T.);
#3715=FACE_OUTER_BOUND('',#5890,.T.);
#3716=FACE_OUTER_BOUND('',#5891,.T.);
#3717=FACE_OUTER_BOUND('',#5892,.T.);
#3718=FACE_OUTER_BOUND('',#5893,.T.);
#3719=FACE_OUTER_BOUND('',#5894,.T.);
#3720=FACE_OUTER_BOUND('',#5895,.T.);
#3721=FACE_OUTER_BOUND('',#5896,.T.);
#3722=FACE_OUTER_BOUND('',#5897,.T.);
#3723=FACE_OUTER_BOUND('',#5898,.T.);
#3724=FACE_OUTER_BOUND('',#5899,.T.);
#3725=FACE_OUTER_BOUND('',#5900,.T.);
#3726=FACE_OUTER_BOUND('',#5901,.T.);
#3727=FACE_OUTER_BOUND('',#5902,.T.);
#3728=FACE_OUTER_BOUND('',#5903,.T.);
#3729=FACE_OUTER_BOUND('',#5904,.T.);
#3730=FACE_OUTER_BOUND('',#5905,.T.);
#3731=FACE_OUTER_BOUND('',#5906,.T.);
#3732=FACE_OUTER_BOUND('',#5907,.T.);
#3733=FACE_OUTER_BOUND('',#5908,.T.);
#3734=FACE_OUTER_BOUND('',#5909,.T.);
#3735=FACE_OUTER_BOUND('',#5910,.T.);
#3736=FACE_OUTER_BOUND('',#5911,.T.);
#3737=FACE_OUTER_BOUND('',#5912,.T.);
#3738=FACE_OUTER_BOUND('',#5913,.T.);
#3739=FACE_OUTER_BOUND('',#5914,.T.);
#3740=FACE_OUTER_BOUND('',#5915,.T.);
#3741=FACE_OUTER_BOUND('',#5916,.T.);
#3742=FACE_OUTER_BOUND('',#5917,.T.);
#3743=FACE_OUTER_BOUND('',#5918,.T.);
#3744=FACE_OUTER_BOUND('',#5919,.T.);
#3745=FACE_OUTER_BOUND('',#5920,.T.);
#3746=FACE_OUTER_BOUND('',#5921,.T.);
#3747=FACE_OUTER_BOUND('',#5922,.T.);
#3748=FACE_OUTER_BOUND('',#5923,.T.);
#3749=FACE_OUTER_BOUND('',#5924,.T.);
#3750=FACE_OUTER_BOUND('',#5925,.T.);
#3751=FACE_OUTER_BOUND('',#5926,.T.);
#3752=FACE_OUTER_BOUND('',#5927,.T.);
#3753=FACE_OUTER_BOUND('',#5928,.T.);
#3754=FACE_OUTER_BOUND('',#5929,.T.);
#3755=FACE_OUTER_BOUND('',#5930,.T.);
#3756=FACE_OUTER_BOUND('',#5931,.T.);
#3757=FACE_OUTER_BOUND('',#5932,.T.);
#3758=FACE_OUTER_BOUND('',#5933,.T.);
#3759=FACE_OUTER_BOUND('',#5934,.T.);
#3760=FACE_OUTER_BOUND('',#5935,.T.);
#3761=FACE_OUTER_BOUND('',#5936,.T.);
#3762=FACE_OUTER_BOUND('',#5937,.T.);
#3763=FACE_OUTER_BOUND('',#5938,.T.);
#3764=FACE_OUTER_BOUND('',#5939,.T.);
#3765=FACE_OUTER_BOUND('',#5940,.T.);
#3766=FACE_OUTER_BOUND('',#5941,.T.);
#3767=FACE_OUTER_BOUND('',#5942,.T.);
#3768=FACE_OUTER_BOUND('',#5943,.T.);
#3769=FACE_OUTER_BOUND('',#5944,.T.);
#3770=FACE_OUTER_BOUND('',#5945,.T.);
#3771=FACE_OUTER_BOUND('',#5946,.T.);
#3772=FACE_OUTER_BOUND('',#5947,.T.);
#3773=FACE_OUTER_BOUND('',#5948,.T.);
#3774=FACE_OUTER_BOUND('',#5949,.T.);
#3775=FACE_OUTER_BOUND('',#5950,.T.);
#3776=FACE_OUTER_BOUND('',#5951,.T.);
#3777=FACE_OUTER_BOUND('',#5952,.T.);
#3778=FACE_OUTER_BOUND('',#5953,.T.);
#3779=FACE_OUTER_BOUND('',#5954,.T.);
#3780=FACE_OUTER_BOUND('',#5955,.T.);
#3781=FACE_OUTER_BOUND('',#5956,.T.);
#3782=FACE_OUTER_BOUND('',#5957,.T.);
#3783=FACE_OUTER_BOUND('',#5958,.T.);
#3784=FACE_OUTER_BOUND('',#5959,.T.);
#3785=FACE_OUTER_BOUND('',#5960,.T.);
#3786=FACE_OUTER_BOUND('',#5961,.T.);
#3787=FACE_OUTER_BOUND('',#5962,.T.);
#3788=FACE_OUTER_BOUND('',#5963,.T.);
#3789=FACE_OUTER_BOUND('',#5964,.T.);
#3790=FACE_OUTER_BOUND('',#5965,.T.);
#3791=FACE_OUTER_BOUND('',#5966,.T.);
#3792=FACE_OUTER_BOUND('',#5967,.T.);
#3793=FACE_OUTER_BOUND('',#5968,.T.);
#3794=FACE_OUTER_BOUND('',#5969,.T.);
#3795=FACE_OUTER_BOUND('',#5970,.T.);
#3796=FACE_OUTER_BOUND('',#5971,.T.);
#3797=FACE_OUTER_BOUND('',#5972,.T.);
#3798=FACE_OUTER_BOUND('',#5973,.T.);
#3799=FACE_OUTER_BOUND('',#5974,.T.);
#3800=FACE_OUTER_BOUND('',#5975,.T.);
#3801=FACE_OUTER_BOUND('',#5976,.T.);
#3802=FACE_OUTER_BOUND('',#5977,.T.);
#3803=FACE_OUTER_BOUND('',#5978,.T.);
#3804=FACE_OUTER_BOUND('',#5979,.T.);
#3805=FACE_OUTER_BOUND('',#5980,.T.);
#3806=FACE_OUTER_BOUND('',#5981,.T.);
#3807=FACE_OUTER_BOUND('',#5982,.T.);
#3808=FACE_OUTER_BOUND('',#5983,.T.);
#3809=FACE_OUTER_BOUND('',#5984,.T.);
#3810=FACE_OUTER_BOUND('',#5985,.T.);
#3811=FACE_OUTER_BOUND('',#5986,.T.);
#3812=FACE_OUTER_BOUND('',#5987,.T.);
#3813=FACE_OUTER_BOUND('',#5988,.T.);
#3814=FACE_OUTER_BOUND('',#5989,.T.);
#3815=FACE_OUTER_BOUND('',#5990,.T.);
#3816=FACE_OUTER_BOUND('',#5991,.T.);
#3817=FACE_OUTER_BOUND('',#5992,.T.);
#3818=FACE_OUTER_BOUND('',#5993,.T.);
#3819=FACE_OUTER_BOUND('',#5994,.T.);
#3820=FACE_OUTER_BOUND('',#5995,.T.);
#3821=FACE_OUTER_BOUND('',#5996,.T.);
#3822=FACE_OUTER_BOUND('',#5997,.T.);
#3823=FACE_OUTER_BOUND('',#5998,.T.);
#3824=FACE_OUTER_BOUND('',#5999,.T.);
#3825=FACE_OUTER_BOUND('',#6000,.T.);
#3826=FACE_OUTER_BOUND('',#6001,.T.);
#3827=FACE_OUTER_BOUND('',#6002,.T.);
#3828=FACE_OUTER_BOUND('',#6003,.T.);
#3829=FACE_OUTER_BOUND('',#6004,.T.);
#3830=FACE_OUTER_BOUND('',#6005,.T.);
#3831=FACE_OUTER_BOUND('',#6006,.T.);
#3832=FACE_OUTER_BOUND('',#6007,.T.);
#3833=FACE_OUTER_BOUND('',#6008,.T.);
#3834=FACE_OUTER_BOUND('',#6009,.T.);
#3835=FACE_OUTER_BOUND('',#6010,.T.);
#3836=FACE_OUTER_BOUND('',#6011,.T.);
#3837=FACE_OUTER_BOUND('',#6012,.T.);
#3838=FACE_OUTER_BOUND('',#6013,.T.);
#3839=FACE_OUTER_BOUND('',#6014,.T.);
#3840=FACE_OUTER_BOUND('',#6015,.T.);
#3841=FACE_OUTER_BOUND('',#6016,.T.);
#3842=FACE_OUTER_BOUND('',#6017,.T.);
#3843=FACE_OUTER_BOUND('',#6018,.T.);
#3844=FACE_OUTER_BOUND('',#6019,.T.);
#3845=FACE_OUTER_BOUND('',#6020,.T.);
#3846=FACE_OUTER_BOUND('',#6021,.T.);
#3847=FACE_OUTER_BOUND('',#6022,.T.);
#3848=FACE_OUTER_BOUND('',#6023,.T.);
#3849=FACE_OUTER_BOUND('',#6024,.T.);
#3850=FACE_OUTER_BOUND('',#6025,.T.);
#3851=FACE_OUTER_BOUND('',#6026,.T.);
#3852=FACE_OUTER_BOUND('',#6027,.T.);
#3853=FACE_OUTER_BOUND('',#6028,.T.);
#3854=FACE_OUTER_BOUND('',#6029,.T.);
#3855=FACE_OUTER_BOUND('',#6030,.T.);
#3856=FACE_OUTER_BOUND('',#6031,.T.);
#3857=FACE_OUTER_BOUND('',#6032,.T.);
#3858=FACE_OUTER_BOUND('',#6033,.T.);
#3859=FACE_OUTER_BOUND('',#6034,.T.);
#3860=FACE_OUTER_BOUND('',#6035,.T.);
#3861=FACE_OUTER_BOUND('',#6036,.T.);
#3862=FACE_OUTER_BOUND('',#6037,.T.);
#3863=FACE_OUTER_BOUND('',#6038,.T.);
#3864=FACE_OUTER_BOUND('',#6039,.T.);
#3865=FACE_OUTER_BOUND('',#6040,.T.);
#3866=FACE_OUTER_BOUND('',#6041,.T.);
#3867=FACE_OUTER_BOUND('',#6042,.T.);
#3868=FACE_OUTER_BOUND('',#6043,.T.);
#3869=FACE_OUTER_BOUND('',#6044,.T.);
#3870=FACE_OUTER_BOUND('',#6045,.T.);
#3871=FACE_OUTER_BOUND('',#6046,.T.);
#3872=FACE_OUTER_BOUND('',#6047,.T.);
#3873=FACE_OUTER_BOUND('',#6048,.T.);
#3874=FACE_OUTER_BOUND('',#6049,.T.);
#3875=FACE_OUTER_BOUND('',#6050,.T.);
#3876=FACE_OUTER_BOUND('',#6051,.T.);
#3877=FACE_OUTER_BOUND('',#6052,.T.);
#3878=FACE_OUTER_BOUND('',#6053,.T.);
#3879=FACE_OUTER_BOUND('',#6054,.T.);
#3880=FACE_OUTER_BOUND('',#6055,.T.);
#3881=FACE_OUTER_BOUND('',#6056,.T.);
#3882=FACE_OUTER_BOUND('',#6057,.T.);
#3883=FACE_OUTER_BOUND('',#6058,.T.);
#3884=FACE_OUTER_BOUND('',#6059,.T.);
#3885=FACE_OUTER_BOUND('',#6060,.T.);
#3886=FACE_OUTER_BOUND('',#6061,.T.);
#3887=FACE_OUTER_BOUND('',#6062,.T.);
#3888=FACE_OUTER_BOUND('',#6063,.T.);
#3889=FACE_OUTER_BOUND('',#6064,.T.);
#3890=FACE_OUTER_BOUND('',#6065,.T.);
#3891=FACE_OUTER_BOUND('',#6066,.T.);
#3892=FACE_OUTER_BOUND('',#6067,.T.);
#3893=FACE_OUTER_BOUND('',#6068,.T.);
#3894=FACE_OUTER_BOUND('',#6069,.T.);
#3895=FACE_OUTER_BOUND('',#6070,.T.);
#3896=FACE_OUTER_BOUND('',#6071,.T.);
#3897=FACE_OUTER_BOUND('',#6072,.T.);
#3898=FACE_OUTER_BOUND('',#6073,.T.);
#3899=FACE_OUTER_BOUND('',#6074,.T.);
#3900=FACE_OUTER_BOUND('',#6075,.T.);
#3901=FACE_OUTER_BOUND('',#6076,.T.);
#3902=FACE_OUTER_BOUND('',#6077,.T.);
#3903=FACE_OUTER_BOUND('',#6078,.T.);
#3904=FACE_OUTER_BOUND('',#6079,.T.);
#3905=FACE_OUTER_BOUND('',#6080,.T.);
#3906=FACE_OUTER_BOUND('',#6081,.T.);
#3907=FACE_OUTER_BOUND('',#6082,.T.);
#3908=FACE_OUTER_BOUND('',#6083,.T.);
#3909=FACE_OUTER_BOUND('',#6084,.T.);
#3910=FACE_OUTER_BOUND('',#6085,.T.);
#3911=FACE_OUTER_BOUND('',#6086,.T.);
#3912=FACE_OUTER_BOUND('',#6087,.T.);
#3913=FACE_OUTER_BOUND('',#6088,.T.);
#3914=FACE_OUTER_BOUND('',#6089,.T.);
#3915=FACE_OUTER_BOUND('',#6090,.T.);
#3916=FACE_OUTER_BOUND('',#6091,.T.);
#3917=FACE_OUTER_BOUND('',#6092,.T.);
#3918=FACE_OUTER_BOUND('',#6093,.T.);
#3919=FACE_OUTER_BOUND('',#6094,.T.);
#3920=FACE_OUTER_BOUND('',#6095,.T.);
#3921=FACE_OUTER_BOUND('',#6096,.T.);
#3922=FACE_OUTER_BOUND('',#6097,.T.);
#3923=FACE_OUTER_BOUND('',#6098,.T.);
#3924=FACE_OUTER_BOUND('',#6099,.T.);
#3925=FACE_OUTER_BOUND('',#6100,.T.);
#3926=FACE_OUTER_BOUND('',#6101,.T.);
#3927=FACE_OUTER_BOUND('',#6102,.T.);
#3928=FACE_OUTER_BOUND('',#6103,.T.);
#3929=FACE_OUTER_BOUND('',#6104,.T.);
#3930=FACE_OUTER_BOUND('',#6105,.T.);
#3931=FACE_OUTER_BOUND('',#6106,.T.);
#3932=FACE_OUTER_BOUND('',#6107,.T.);
#3933=FACE_OUTER_BOUND('',#6108,.T.);
#3934=FACE_OUTER_BOUND('',#6109,.T.);
#3935=FACE_OUTER_BOUND('',#6110,.T.);
#3936=FACE_OUTER_BOUND('',#6111,.T.);
#3937=FACE_OUTER_BOUND('',#6112,.T.);
#3938=FACE_OUTER_BOUND('',#6113,.T.);
#3939=FACE_OUTER_BOUND('',#6114,.T.);
#3940=FACE_OUTER_BOUND('',#6115,.T.);
#3941=FACE_OUTER_BOUND('',#6116,.T.);
#3942=FACE_OUTER_BOUND('',#6117,.T.);
#3943=FACE_OUTER_BOUND('',#6118,.T.);
#3944=FACE_OUTER_BOUND('',#6119,.T.);
#3945=FACE_OUTER_BOUND('',#6120,.T.);
#3946=FACE_OUTER_BOUND('',#6121,.T.);
#3947=FACE_OUTER_BOUND('',#6122,.T.);
#3948=FACE_OUTER_BOUND('',#6123,.T.);
#3949=FACE_OUTER_BOUND('',#6124,.T.);
#3950=FACE_OUTER_BOUND('',#6125,.T.);
#3951=FACE_OUTER_BOUND('',#6126,.T.);
#3952=FACE_OUTER_BOUND('',#6127,.T.);
#3953=FACE_OUTER_BOUND('',#6128,.T.);
#3954=FACE_OUTER_BOUND('',#6129,.T.);
#3955=FACE_OUTER_BOUND('',#6130,.T.);
#3956=FACE_OUTER_BOUND('',#6131,.T.);
#3957=FACE_OUTER_BOUND('',#6132,.T.);
#3958=FACE_OUTER_BOUND('',#6133,.T.);
#3959=FACE_OUTER_BOUND('',#6134,.T.);
#3960=FACE_OUTER_BOUND('',#6135,.T.);
#3961=FACE_OUTER_BOUND('',#6136,.T.);
#3962=FACE_OUTER_BOUND('',#6137,.T.);
#3963=FACE_OUTER_BOUND('',#6138,.T.);
#3964=FACE_OUTER_BOUND('',#6139,.T.);
#3965=FACE_OUTER_BOUND('',#6140,.T.);
#3966=FACE_OUTER_BOUND('',#6141,.T.);
#3967=FACE_OUTER_BOUND('',#6142,.T.);
#3968=FACE_OUTER_BOUND('',#6143,.T.);
#3969=FACE_OUTER_BOUND('',#6144,.T.);
#3970=FACE_OUTER_BOUND('',#6145,.T.);
#3971=FACE_OUTER_BOUND('',#6146,.T.);
#3972=FACE_OUTER_BOUND('',#6147,.T.);
#3973=FACE_OUTER_BOUND('',#6148,.T.);
#3974=FACE_OUTER_BOUND('',#6149,.T.);
#3975=FACE_OUTER_BOUND('',#6150,.T.);
#3976=FACE_OUTER_BOUND('',#6151,.T.);
#3977=FACE_OUTER_BOUND('',#6152,.T.);
#3978=FACE_OUTER_BOUND('',#6153,.T.);
#3979=FACE_OUTER_BOUND('',#6154,.T.);
#3980=FACE_OUTER_BOUND('',#6155,.T.);
#3981=FACE_OUTER_BOUND('',#6156,.T.);
#3982=FACE_OUTER_BOUND('',#6157,.T.);
#3983=FACE_OUTER_BOUND('',#6158,.T.);
#3984=FACE_OUTER_BOUND('',#6159,.T.);
#3985=FACE_OUTER_BOUND('',#6160,.T.);
#3986=FACE_OUTER_BOUND('',#6161,.T.);
#3987=FACE_OUTER_BOUND('',#6162,.T.);
#3988=FACE_OUTER_BOUND('',#6163,.T.);
#3989=FACE_OUTER_BOUND('',#6164,.T.);
#3990=FACE_OUTER_BOUND('',#6165,.T.);
#3991=FACE_OUTER_BOUND('',#6166,.T.);
#3992=FACE_OUTER_BOUND('',#6167,.T.);
#3993=FACE_OUTER_BOUND('',#6168,.T.);
#3994=FACE_OUTER_BOUND('',#6169,.T.);
#3995=FACE_OUTER_BOUND('',#6170,.T.);
#3996=FACE_OUTER_BOUND('',#6171,.T.);
#3997=FACE_OUTER_BOUND('',#6172,.T.);
#3998=FACE_OUTER_BOUND('',#6173,.T.);
#3999=FACE_OUTER_BOUND('',#6174,.T.);
#4000=FACE_OUTER_BOUND('',#6175,.T.);
#4001=FACE_OUTER_BOUND('',#6176,.T.);
#4002=FACE_OUTER_BOUND('',#6177,.T.);
#4003=FACE_OUTER_BOUND('',#6178,.T.);
#4004=FACE_OUTER_BOUND('',#6179,.T.);
#4005=FACE_OUTER_BOUND('',#6180,.T.);
#4006=FACE_OUTER_BOUND('',#6181,.T.);
#4007=FACE_OUTER_BOUND('',#6182,.T.);
#4008=FACE_OUTER_BOUND('',#6183,.T.);
#4009=FACE_OUTER_BOUND('',#6184,.T.);
#4010=FACE_OUTER_BOUND('',#6185,.T.);
#4011=FACE_OUTER_BOUND('',#6186,.T.);
#4012=FACE_OUTER_BOUND('',#6187,.T.);
#4013=FACE_OUTER_BOUND('',#6188,.T.);
#4014=FACE_OUTER_BOUND('',#6189,.T.);
#4015=FACE_OUTER_BOUND('',#6190,.T.);
#4016=FACE_OUTER_BOUND('',#6191,.T.);
#4017=FACE_OUTER_BOUND('',#6192,.T.);
#4018=FACE_OUTER_BOUND('',#6193,.T.);
#4019=FACE_OUTER_BOUND('',#6194,.T.);
#4020=FACE_OUTER_BOUND('',#6195,.T.);
#4021=FACE_OUTER_BOUND('',#6196,.T.);
#4022=FACE_OUTER_BOUND('',#6197,.T.);
#4023=FACE_OUTER_BOUND('',#6198,.T.);
#4024=FACE_OUTER_BOUND('',#6199,.T.);
#4025=FACE_OUTER_BOUND('',#6200,.T.);
#4026=FACE_OUTER_BOUND('',#6201,.T.);
#4027=FACE_OUTER_BOUND('',#6202,.T.);
#4028=FACE_OUTER_BOUND('',#6203,.T.);
#4029=FACE_OUTER_BOUND('',#6204,.T.);
#4030=FACE_OUTER_BOUND('',#6205,.T.);
#4031=FACE_OUTER_BOUND('',#6206,.T.);
#4032=FACE_OUTER_BOUND('',#6207,.T.);
#4033=FACE_OUTER_BOUND('',#6208,.T.);
#4034=FACE_OUTER_BOUND('',#6209,.T.);
#4035=FACE_OUTER_BOUND('',#6210,.T.);
#4036=FACE_OUTER_BOUND('',#6211,.T.);
#4037=FACE_OUTER_BOUND('',#6212,.T.);
#4038=FACE_OUTER_BOUND('',#6213,.T.);
#4039=FACE_OUTER_BOUND('',#6214,.T.);
#4040=FACE_OUTER_BOUND('',#6215,.T.);
#4041=FACE_OUTER_BOUND('',#6216,.T.);
#4042=FACE_OUTER_BOUND('',#6217,.T.);
#4043=FACE_OUTER_BOUND('',#6218,.T.);
#4044=FACE_OUTER_BOUND('',#6219,.T.);
#4045=FACE_OUTER_BOUND('',#6220,.T.);
#4046=FACE_OUTER_BOUND('',#6221,.T.);
#4047=FACE_OUTER_BOUND('',#6222,.T.);
#4048=FACE_OUTER_BOUND('',#6223,.T.);
#4049=FACE_OUTER_BOUND('',#6224,.T.);
#4050=FACE_OUTER_BOUND('',#6225,.T.);
#4051=FACE_OUTER_BOUND('',#6226,.T.);
#4052=FACE_OUTER_BOUND('',#6227,.T.);
#4053=FACE_OUTER_BOUND('',#6228,.T.);
#4054=FACE_OUTER_BOUND('',#6229,.T.);
#4055=FACE_OUTER_BOUND('',#6230,.T.);
#4056=FACE_OUTER_BOUND('',#6231,.T.);
#4057=FACE_OUTER_BOUND('',#6232,.T.);
#4058=FACE_OUTER_BOUND('',#6233,.T.);
#4059=FACE_OUTER_BOUND('',#6234,.T.);
#4060=FACE_OUTER_BOUND('',#6235,.T.);
#4061=FACE_OUTER_BOUND('',#6236,.T.);
#4062=FACE_OUTER_BOUND('',#6237,.T.);
#4063=FACE_OUTER_BOUND('',#6238,.T.);
#4064=FACE_OUTER_BOUND('',#6239,.T.);
#4065=FACE_OUTER_BOUND('',#6240,.T.);
#4066=FACE_OUTER_BOUND('',#6241,.T.);
#4067=FACE_OUTER_BOUND('',#6242,.T.);
#4068=FACE_OUTER_BOUND('',#6243,.T.);
#4069=FACE_OUTER_BOUND('',#6244,.T.);
#4070=FACE_OUTER_BOUND('',#6245,.T.);
#4071=FACE_OUTER_BOUND('',#6246,.T.);
#4072=FACE_OUTER_BOUND('',#6247,.T.);
#4073=FACE_OUTER_BOUND('',#6248,.T.);
#4074=FACE_OUTER_BOUND('',#6249,.T.);
#4075=FACE_OUTER_BOUND('',#6250,.T.);
#4076=FACE_OUTER_BOUND('',#6251,.T.);
#4077=FACE_OUTER_BOUND('',#6252,.T.);
#4078=FACE_OUTER_BOUND('',#6253,.T.);
#4079=FACE_OUTER_BOUND('',#6254,.T.);
#4080=FACE_OUTER_BOUND('',#6255,.T.);
#4081=FACE_OUTER_BOUND('',#6256,.T.);
#4082=FACE_OUTER_BOUND('',#6257,.T.);
#4083=FACE_OUTER_BOUND('',#6258,.T.);
#4084=FACE_OUTER_BOUND('',#6259,.T.);
#4085=FACE_OUTER_BOUND('',#6260,.T.);
#4086=FACE_OUTER_BOUND('',#6261,.T.);
#4087=FACE_OUTER_BOUND('',#6262,.T.);
#4088=FACE_OUTER_BOUND('',#6263,.T.);
#4089=FACE_OUTER_BOUND('',#6264,.T.);
#4090=FACE_OUTER_BOUND('',#6265,.T.);
#4091=FACE_OUTER_BOUND('',#6266,.T.);
#4092=FACE_OUTER_BOUND('',#6267,.T.);
#4093=FACE_OUTER_BOUND('',#6268,.T.);
#4094=FACE_OUTER_BOUND('',#6269,.T.);
#4095=FACE_OUTER_BOUND('',#6270,.T.);
#4096=FACE_OUTER_BOUND('',#6271,.T.);
#4097=FACE_OUTER_BOUND('',#6272,.T.);
#4098=FACE_OUTER_BOUND('',#6273,.T.);
#4099=FACE_OUTER_BOUND('',#6274,.T.);
#4100=FACE_OUTER_BOUND('',#6275,.T.);
#4101=FACE_OUTER_BOUND('',#6276,.T.);
#4102=FACE_OUTER_BOUND('',#6277,.T.);
#4103=FACE_OUTER_BOUND('',#6278,.T.);
#4104=FACE_OUTER_BOUND('',#6279,.T.);
#4105=FACE_OUTER_BOUND('',#6280,.T.);
#4106=FACE_OUTER_BOUND('',#6281,.T.);
#4107=FACE_OUTER_BOUND('',#6282,.T.);
#4108=FACE_OUTER_BOUND('',#6283,.T.);
#4109=FACE_OUTER_BOUND('',#6284,.T.);
#4110=FACE_OUTER_BOUND('',#6285,.T.);
#4111=FACE_OUTER_BOUND('',#6286,.T.);
#4112=FACE_OUTER_BOUND('',#6287,.T.);
#4113=FACE_OUTER_BOUND('',#6288,.T.);
#4114=FACE_OUTER_BOUND('',#6289,.T.);
#4115=FACE_OUTER_BOUND('',#6290,.T.);
#4116=FACE_OUTER_BOUND('',#6291,.T.);
#4117=FACE_OUTER_BOUND('',#6292,.T.);
#4118=FACE_OUTER_BOUND('',#6293,.T.);
#4119=FACE_OUTER_BOUND('',#6294,.T.);
#4120=FACE_OUTER_BOUND('',#6295,.T.);
#4121=FACE_OUTER_BOUND('',#6296,.T.);
#4122=FACE_OUTER_BOUND('',#6297,.T.);
#4123=FACE_OUTER_BOUND('',#6298,.T.);
#4124=FACE_OUTER_BOUND('',#6299,.T.);
#4125=FACE_OUTER_BOUND('',#6300,.T.);
#4126=FACE_OUTER_BOUND('',#6301,.T.);
#4127=FACE_OUTER_BOUND('',#6302,.T.);
#4128=FACE_OUTER_BOUND('',#6303,.T.);
#4129=FACE_OUTER_BOUND('',#6304,.T.);
#4130=FACE_OUTER_BOUND('',#6305,.T.);
#4131=FACE_OUTER_BOUND('',#6306,.T.);
#4132=FACE_OUTER_BOUND('',#6307,.T.);
#4133=FACE_OUTER_BOUND('',#6308,.T.);
#4134=FACE_OUTER_BOUND('',#6309,.T.);
#4135=FACE_OUTER_BOUND('',#6310,.T.);
#4136=FACE_OUTER_BOUND('',#6311,.T.);
#4137=FACE_OUTER_BOUND('',#6312,.T.);
#4138=FACE_OUTER_BOUND('',#6313,.T.);
#4139=FACE_OUTER_BOUND('',#6314,.T.);
#4140=FACE_OUTER_BOUND('',#6315,.T.);
#4141=FACE_OUTER_BOUND('',#6316,.T.);
#4142=FACE_OUTER_BOUND('',#6317,.T.);
#4143=FACE_OUTER_BOUND('',#6318,.T.);
#4144=FACE_OUTER_BOUND('',#6319,.T.);
#4145=FACE_OUTER_BOUND('',#6320,.T.);
#4146=FACE_OUTER_BOUND('',#6321,.T.);
#4147=FACE_OUTER_BOUND('',#6322,.T.);
#4148=FACE_OUTER_BOUND('',#6323,.T.);
#4149=FACE_OUTER_BOUND('',#6324,.T.);
#4150=FACE_OUTER_BOUND('',#6325,.T.);
#4151=FACE_OUTER_BOUND('',#6326,.T.);
#4152=FACE_OUTER_BOUND('',#6327,.T.);
#4153=FACE_OUTER_BOUND('',#6328,.T.);
#4154=FACE_OUTER_BOUND('',#6329,.T.);
#4155=FACE_OUTER_BOUND('',#6330,.T.);
#4156=FACE_OUTER_BOUND('',#6331,.T.);
#4157=FACE_OUTER_BOUND('',#6332,.T.);
#4158=FACE_OUTER_BOUND('',#6333,.T.);
#4159=FACE_OUTER_BOUND('',#6334,.T.);
#4160=FACE_OUTER_BOUND('',#6335,.T.);
#4161=FACE_OUTER_BOUND('',#6336,.T.);
#4162=FACE_OUTER_BOUND('',#6337,.T.);
#4163=FACE_OUTER_BOUND('',#6338,.T.);
#4164=FACE_OUTER_BOUND('',#6339,.T.);
#4165=FACE_OUTER_BOUND('',#6340,.T.);
#4166=FACE_OUTER_BOUND('',#6341,.T.);
#4167=FACE_OUTER_BOUND('',#6342,.T.);
#4168=FACE_OUTER_BOUND('',#6343,.T.);
#4169=FACE_OUTER_BOUND('',#6344,.T.);
#4170=FACE_OUTER_BOUND('',#6345,.T.);
#4171=FACE_OUTER_BOUND('',#6346,.T.);
#4172=FACE_OUTER_BOUND('',#6347,.T.);
#4173=FACE_OUTER_BOUND('',#6348,.T.);
#4174=FACE_OUTER_BOUND('',#6349,.T.);
#4175=FACE_OUTER_BOUND('',#6350,.T.);
#4176=FACE_OUTER_BOUND('',#6351,.T.);
#4177=FACE_OUTER_BOUND('',#6352,.T.);
#4178=FACE_OUTER_BOUND('',#6353,.T.);
#4179=FACE_OUTER_BOUND('',#6354,.T.);
#4180=FACE_OUTER_BOUND('',#6355,.T.);
#4181=FACE_OUTER_BOUND('',#6356,.T.);
#4182=FACE_OUTER_BOUND('',#6357,.T.);
#4183=FACE_OUTER_BOUND('',#6358,.T.);
#4184=FACE_OUTER_BOUND('',#6359,.T.);
#4185=FACE_OUTER_BOUND('',#6360,.T.);
#4186=FACE_OUTER_BOUND('',#6361,.T.);
#4187=FACE_OUTER_BOUND('',#6362,.T.);
#4188=FACE_OUTER_BOUND('',#6363,.T.);
#4189=FACE_OUTER_BOUND('',#6364,.T.);
#4190=FACE_OUTER_BOUND('',#6365,.T.);
#4191=FACE_OUTER_BOUND('',#6366,.T.);
#4192=FACE_OUTER_BOUND('',#6367,.T.);
#4193=FACE_OUTER_BOUND('',#6368,.T.);
#4194=FACE_OUTER_BOUND('',#6369,.T.);
#4195=FACE_OUTER_BOUND('',#6370,.T.);
#4196=FACE_OUTER_BOUND('',#6371,.T.);
#4197=FACE_OUTER_BOUND('',#6372,.T.);
#4198=FACE_OUTER_BOUND('',#6373,.T.);
#4199=FACE_OUTER_BOUND('',#6374,.T.);
#4200=FACE_OUTER_BOUND('',#6375,.T.);
#4201=FACE_OUTER_BOUND('',#6376,.T.);
#4202=FACE_OUTER_BOUND('',#6377,.T.);
#4203=FACE_OUTER_BOUND('',#6378,.T.);
#4204=FACE_OUTER_BOUND('',#6379,.T.);
#4205=FACE_OUTER_BOUND('',#6380,.T.);
#4206=FACE_OUTER_BOUND('',#6381,.T.);
#4207=FACE_OUTER_BOUND('',#6382,.T.);
#4208=FACE_OUTER_BOUND('',#6383,.T.);
#4209=FACE_OUTER_BOUND('',#6384,.T.);
#4210=FACE_OUTER_BOUND('',#6385,.T.);
#4211=FACE_OUTER_BOUND('',#6386,.T.);
#4212=FACE_OUTER_BOUND('',#6387,.T.);
#4213=FACE_OUTER_BOUND('',#6388,.T.);
#4214=FACE_OUTER_BOUND('',#6389,.T.);
#4215=FACE_OUTER_BOUND('',#6390,.T.);
#4216=FACE_OUTER_BOUND('',#6391,.T.);
#4217=FACE_OUTER_BOUND('',#6392,.T.);
#4218=FACE_OUTER_BOUND('',#6393,.T.);
#4219=FACE_OUTER_BOUND('',#6394,.T.);
#4220=FACE_OUTER_BOUND('',#6395,.T.);
#4221=FACE_OUTER_BOUND('',#6396,.T.);
#4222=FACE_OUTER_BOUND('',#6397,.T.);
#4223=FACE_OUTER_BOUND('',#6398,.T.);
#4224=FACE_OUTER_BOUND('',#6400,.T.);
#4225=FACE_OUTER_BOUND('',#6401,.T.);
#4226=FACE_OUTER_BOUND('',#6402,.T.);
#4227=FACE_OUTER_BOUND('',#6403,.T.);
#4228=FACE_OUTER_BOUND('',#6404,.T.);
#4229=FACE_OUTER_BOUND('',#6405,.T.);
#4230=FACE_OUTER_BOUND('',#6406,.T.);
#4231=FACE_OUTER_BOUND('',#6407,.T.);
#4232=FACE_OUTER_BOUND('',#6408,.T.);
#4233=FACE_OUTER_BOUND('',#6409,.T.);
#4234=FACE_OUTER_BOUND('',#6410,.T.);
#4235=FACE_OUTER_BOUND('',#6411,.T.);
#4236=FACE_OUTER_BOUND('',#6412,.T.);
#4237=FACE_OUTER_BOUND('',#6413,.T.);
#4238=FACE_OUTER_BOUND('',#6414,.T.);
#4239=FACE_OUTER_BOUND('',#6415,.T.);
#4240=FACE_OUTER_BOUND('',#6416,.T.);
#4241=FACE_OUTER_BOUND('',#6417,.T.);
#4242=FACE_OUTER_BOUND('',#6418,.T.);
#4243=FACE_OUTER_BOUND('',#6419,.T.);
#4244=FACE_OUTER_BOUND('',#6420,.T.);
#4245=FACE_OUTER_BOUND('',#6421,.T.);
#4246=FACE_OUTER_BOUND('',#6422,.T.);
#4247=FACE_OUTER_BOUND('',#6423,.T.);
#4248=FACE_OUTER_BOUND('',#6424,.T.);
#4249=FACE_OUTER_BOUND('',#6425,.T.);
#4250=FACE_OUTER_BOUND('',#6426,.T.);
#4251=FACE_OUTER_BOUND('',#6427,.T.);
#4252=FACE_OUTER_BOUND('',#6428,.T.);
#4253=FACE_OUTER_BOUND('',#6429,.T.);
#4254=FACE_OUTER_BOUND('',#6430,.T.);
#4255=FACE_OUTER_BOUND('',#6431,.T.);
#4256=FACE_OUTER_BOUND('',#6432,.T.);
#4257=FACE_OUTER_BOUND('',#6433,.T.);
#4258=FACE_OUTER_BOUND('',#6434,.T.);
#4259=FACE_OUTER_BOUND('',#6435,.T.);
#4260=FACE_OUTER_BOUND('',#6436,.T.);
#4261=FACE_OUTER_BOUND('',#6437,.T.);
#4262=FACE_OUTER_BOUND('',#6438,.T.);
#4263=FACE_OUTER_BOUND('',#6439,.T.);
#4264=FACE_OUTER_BOUND('',#6440,.T.);
#4265=FACE_OUTER_BOUND('',#6441,.T.);
#4266=FACE_OUTER_BOUND('',#6442,.T.);
#4267=FACE_OUTER_BOUND('',#6443,.T.);
#4268=FACE_OUTER_BOUND('',#6444,.T.);
#4269=FACE_OUTER_BOUND('',#6445,.T.);
#4270=FACE_OUTER_BOUND('',#6446,.T.);
#4271=FACE_OUTER_BOUND('',#6447,.T.);
#4272=FACE_OUTER_BOUND('',#6448,.T.);
#4273=FACE_OUTER_BOUND('',#6449,.T.);
#4274=FACE_OUTER_BOUND('',#6450,.T.);
#4275=FACE_OUTER_BOUND('',#6451,.T.);
#4276=FACE_OUTER_BOUND('',#6452,.T.);
#4277=FACE_OUTER_BOUND('',#6453,.T.);
#4278=FACE_OUTER_BOUND('',#6454,.T.);
#4279=FACE_OUTER_BOUND('',#6455,.T.);
#4280=FACE_OUTER_BOUND('',#6456,.T.);
#4281=FACE_OUTER_BOUND('',#6457,.T.);
#4282=FACE_OUTER_BOUND('',#6458,.T.);
#4283=FACE_OUTER_BOUND('',#6459,.T.);
#4284=FACE_OUTER_BOUND('',#6460,.T.);
#4285=FACE_OUTER_BOUND('',#6461,.T.);
#4286=FACE_OUTER_BOUND('',#6462,.T.);
#4287=FACE_OUTER_BOUND('',#6463,.T.);
#4288=FACE_OUTER_BOUND('',#6464,.T.);
#4289=FACE_OUTER_BOUND('',#6465,.T.);
#4290=FACE_OUTER_BOUND('',#6466,.T.);
#4291=FACE_OUTER_BOUND('',#6467,.T.);
#4292=FACE_OUTER_BOUND('',#6468,.T.);
#4293=FACE_OUTER_BOUND('',#6469,.T.);
#4294=FACE_OUTER_BOUND('',#6470,.T.);
#4295=FACE_OUTER_BOUND('',#6471,.T.);
#4296=FACE_OUTER_BOUND('',#6472,.T.);
#4297=FACE_OUTER_BOUND('',#6473,.T.);
#4298=FACE_OUTER_BOUND('',#6474,.T.);
#4299=FACE_OUTER_BOUND('',#6475,.T.);
#4300=FACE_OUTER_BOUND('',#6476,.T.);
#4301=FACE_OUTER_BOUND('',#6477,.T.);
#4302=FACE_OUTER_BOUND('',#6478,.T.);
#4303=FACE_OUTER_BOUND('',#6479,.T.);
#4304=FACE_OUTER_BOUND('',#6480,.T.);
#4305=FACE_OUTER_BOUND('',#6481,.T.);
#4306=FACE_OUTER_BOUND('',#6482,.T.);
#4307=FACE_OUTER_BOUND('',#6483,.T.);
#4308=FACE_OUTER_BOUND('',#6484,.T.);
#4309=FACE_OUTER_BOUND('',#6485,.T.);
#4310=FACE_OUTER_BOUND('',#6486,.T.);
#4311=FACE_OUTER_BOUND('',#6487,.T.);
#4312=FACE_OUTER_BOUND('',#6488,.T.);
#4313=FACE_OUTER_BOUND('',#6489,.T.);
#4314=FACE_OUTER_BOUND('',#6490,.T.);
#4315=FACE_OUTER_BOUND('',#6491,.T.);
#4316=FACE_OUTER_BOUND('',#6492,.T.);
#4317=FACE_OUTER_BOUND('',#6493,.T.);
#4318=FACE_OUTER_BOUND('',#6494,.T.);
#4319=FACE_OUTER_BOUND('',#6495,.T.);
#4320=FACE_OUTER_BOUND('',#6496,.T.);
#4321=FACE_OUTER_BOUND('',#6497,.T.);
#4322=FACE_OUTER_BOUND('',#6498,.T.);
#4323=FACE_OUTER_BOUND('',#6499,.T.);
#4324=FACE_OUTER_BOUND('',#6500,.T.);
#4325=FACE_OUTER_BOUND('',#6501,.T.);
#4326=FACE_OUTER_BOUND('',#6502,.T.);
#4327=FACE_OUTER_BOUND('',#6503,.T.);
#4328=FACE_OUTER_BOUND('',#6504,.T.);
#4329=FACE_OUTER_BOUND('',#6505,.T.);
#4330=FACE_OUTER_BOUND('',#6506,.T.);
#4331=FACE_OUTER_BOUND('',#6507,.T.);
#4332=FACE_OUTER_BOUND('',#6508,.T.);
#4333=FACE_OUTER_BOUND('',#6509,.T.);
#4334=FACE_OUTER_BOUND('',#6510,.T.);
#4335=FACE_OUTER_BOUND('',#6511,.T.);
#4336=FACE_OUTER_BOUND('',#6512,.T.);
#4337=FACE_OUTER_BOUND('',#6513,.T.);
#4338=FACE_OUTER_BOUND('',#6514,.T.);
#4339=FACE_OUTER_BOUND('',#6515,.T.);
#4340=FACE_OUTER_BOUND('',#6516,.T.);
#4341=FACE_OUTER_BOUND('',#6517,.T.);
#4342=FACE_OUTER_BOUND('',#6518,.T.);
#4343=FACE_OUTER_BOUND('',#6519,.T.);
#4344=FACE_OUTER_BOUND('',#6520,.T.);
#4345=FACE_OUTER_BOUND('',#6521,.T.);
#4346=FACE_OUTER_BOUND('',#6522,.T.);
#4347=FACE_OUTER_BOUND('',#6523,.T.);
#4348=FACE_OUTER_BOUND('',#6524,.T.);
#4349=FACE_OUTER_BOUND('',#6525,.T.);
#4350=FACE_OUTER_BOUND('',#6526,.T.);
#4351=FACE_OUTER_BOUND('',#6527,.T.);
#4352=FACE_OUTER_BOUND('',#6528,.T.);
#4353=FACE_OUTER_BOUND('',#6529,.T.);
#4354=FACE_OUTER_BOUND('',#6530,.T.);
#4355=FACE_OUTER_BOUND('',#6531,.T.);
#4356=FACE_OUTER_BOUND('',#6532,.T.);
#4357=FACE_OUTER_BOUND('',#6533,.T.);
#4358=FACE_OUTER_BOUND('',#6534,.T.);
#4359=FACE_OUTER_BOUND('',#6535,.T.);
#4360=FACE_OUTER_BOUND('',#6536,.T.);
#4361=FACE_OUTER_BOUND('',#6537,.T.);
#4362=FACE_OUTER_BOUND('',#6538,.T.);
#4363=FACE_OUTER_BOUND('',#6539,.T.);
#4364=FACE_OUTER_BOUND('',#6540,.T.);
#4365=FACE_OUTER_BOUND('',#6541,.T.);
#4366=FACE_OUTER_BOUND('',#6542,.T.);
#4367=FACE_OUTER_BOUND('',#6543,.T.);
#4368=FACE_OUTER_BOUND('',#6544,.T.);
#4369=FACE_OUTER_BOUND('',#6545,.T.);
#4370=FACE_OUTER_BOUND('',#6546,.T.);
#4371=FACE_OUTER_BOUND('',#6547,.T.);
#4372=FACE_OUTER_BOUND('',#6548,.T.);
#4373=FACE_OUTER_BOUND('',#6549,.T.);
#4374=FACE_OUTER_BOUND('',#6550,.T.);
#4375=FACE_OUTER_BOUND('',#6551,.T.);
#4376=FACE_OUTER_BOUND('',#6552,.T.);
#4377=FACE_OUTER_BOUND('',#6553,.T.);
#4378=FACE_OUTER_BOUND('',#6554,.T.);
#4379=FACE_OUTER_BOUND('',#6555,.T.);
#4380=FACE_OUTER_BOUND('',#6556,.T.);
#4381=FACE_OUTER_BOUND('',#6557,.T.);
#4382=FACE_OUTER_BOUND('',#6558,.T.);
#4383=FACE_OUTER_BOUND('',#6560,.T.);
#4384=FACE_OUTER_BOUND('',#6561,.T.);
#4385=FACE_OUTER_BOUND('',#6563,.T.);
#4386=FACE_OUTER_BOUND('',#6564,.T.);
#4387=FACE_OUTER_BOUND('',#6566,.T.);
#4388=FACE_OUTER_BOUND('',#6567,.T.);
#4389=FACE_OUTER_BOUND('',#6569,.T.);
#4390=FACE_OUTER_BOUND('',#6570,.T.);
#4391=FACE_OUTER_BOUND('',#6571,.T.);
#4392=FACE_OUTER_BOUND('',#6572,.T.);
#4393=FACE_OUTER_BOUND('',#6579,.T.);
#4394=FACE_OUTER_BOUND('',#6580,.T.);
#5234=EDGE_LOOP('',(#22278,#22279,#22280,#22281,#22282,#22283));
#5235=EDGE_LOOP('',(#22284,#22285,#22286,#22287,#22288,#22289));
#5236=EDGE_LOOP('',(#22290,#22291,#22292,#22293,#22294));
#5237=EDGE_LOOP('',(#22295,#22296,#22297,#22298,#22299));
#5238=EDGE_LOOP('',(#22300));
#5239=EDGE_LOOP('',(#22301));
#5240=EDGE_LOOP('',(#22302,#22303,#22304,#22305,#22306));
#5241=EDGE_LOOP('',(#22307,#22308,#22309,#22310,#22311));
#5242=EDGE_LOOP('',(#22312));
#5243=EDGE_LOOP('',(#22313));
#5244=EDGE_LOOP('',(#22314,#22315,#22316,#22317,#22318));
#5245=EDGE_LOOP('',(#22319,#22320,#22321,#22322,#22323,#22324));
#5246=EDGE_LOOP('',(#22325));
#5247=EDGE_LOOP('',(#22326));
#5248=EDGE_LOOP('',(#22327,#22328,#22329,#22330,#22331,#22332));
#5249=EDGE_LOOP('',(#22333,#22334,#22335,#22336,#22337));
#5250=EDGE_LOOP('',(#22338,#22339,#22340,#22341,#22342,#22343));
#5251=EDGE_LOOP('',(#22344,#22345,#22346,#22347,#22348,#22349));
#5252=EDGE_LOOP('',(#22350,#22351,#22352,#22353,#22354));
#5253=EDGE_LOOP('',(#22355,#22356,#22357,#22358,#22359,#22360));
#5254=EDGE_LOOP('',(#22361,#22362,#22363,#22364,#22365,#22366));
#5255=EDGE_LOOP('',(#22367,#22368,#22369,#22370,#22371,#22372));
#5256=EDGE_LOOP('',(#22373,#22374,#22375,#22376,#22377,#22378));
#5257=EDGE_LOOP('',(#22379,#22380,#22381,#22382,#22383,#22384));
#5258=EDGE_LOOP('',(#22385,#22386,#22387,#22388,#22389,#22390,#22391,#22392,
#22393,#22394,#22395,#22396,#22397,#22398,#22399,#22400,#22401));
#5259=EDGE_LOOP('',(#22402,#22403,#22404,#22405,#22406,#22407,#22408,#22409));
#5260=EDGE_LOOP('',(#22410,#22411,#22412,#22413,#22414,#22415,#22416,#22417));
#5261=EDGE_LOOP('',(#22418,#22419,#22420,#22421,#22422,#22423,#22424,#22425));
#5262=EDGE_LOOP('',(#22426,#22427,#22428,#22429,#22430,#22431,#22432,#22433));
#5263=EDGE_LOOP('',(#22434,#22435,#22436,#22437,#22438,#22439,#22440,#22441));
#5264=EDGE_LOOP('',(#22442,#22443,#22444,#22445,#22446,#22447,#22448,#22449));
#5265=EDGE_LOOP('',(#22450,#22451,#22452,#22453,#22454,#22455,#22456,#22457));
#5266=EDGE_LOOP('',(#22458,#22459,#22460,#22461,#22462,#22463,#22464,#22465));
#5267=EDGE_LOOP('',(#22466,#22467,#22468,#22469,#22470,#22471,#22472,#22473));
#5268=EDGE_LOOP('',(#22474,#22475,#22476,#22477,#22478,#22479,#22480,#22481));
#5269=EDGE_LOOP('',(#22482,#22483,#22484,#22485,#22486,#22487,#22488,#22489));
#5270=EDGE_LOOP('',(#22490,#22491,#22492,#22493,#22494,#22495,#22496,#22497));
#5271=EDGE_LOOP('',(#22498,#22499,#22500,#22501,#22502,#22503,#22504,#22505));
#5272=EDGE_LOOP('',(#22506,#22507,#22508,#22509,#22510,#22511,#22512,#22513));
#5273=EDGE_LOOP('',(#22514,#22515,#22516,#22517,#22518,#22519,#22520,#22521));
#5274=EDGE_LOOP('',(#22522,#22523,#22524,#22525,#22526,#22527,#22528,#22529));
#5275=EDGE_LOOP('',(#22530,#22531,#22532,#22533,#22534,#22535,#22536,#22537));
#5276=EDGE_LOOP('',(#22538,#22539,#22540,#22541,#22542,#22543,#22544,#22545));
#5277=EDGE_LOOP('',(#22546,#22547,#22548,#22549,#22550,#22551,#22552,#22553));
#5278=EDGE_LOOP('',(#22554,#22555,#22556,#22557,#22558,#22559,#22560,#22561));
#5279=EDGE_LOOP('',(#22562,#22563,#22564,#22565,#22566,#22567,#22568,#22569));
#5280=EDGE_LOOP('',(#22570,#22571,#22572,#22573,#22574,#22575,#22576,#22577));
#5281=EDGE_LOOP('',(#22578,#22579,#22580,#22581,#22582,#22583,#22584,#22585));
#5282=EDGE_LOOP('',(#22586,#22587,#22588,#22589,#22590,#22591,#22592,#22593));
#5283=EDGE_LOOP('',(#22594,#22595,#22596,#22597,#22598,#22599,#22600,#22601));
#5284=EDGE_LOOP('',(#22602,#22603,#22604,#22605,#22606,#22607,#22608,#22609));
#5285=EDGE_LOOP('',(#22610,#22611,#22612,#22613,#22614,#22615,#22616,#22617));
#5286=EDGE_LOOP('',(#22618,#22619,#22620,#22621,#22622,#22623,#22624,#22625));
#5287=EDGE_LOOP('',(#22626,#22627,#22628,#22629,#22630,#22631,#22632,#22633));
#5288=EDGE_LOOP('',(#22634,#22635,#22636,#22637,#22638,#22639,#22640,#22641));
#5289=EDGE_LOOP('',(#22642,#22643,#22644,#22645,#22646,#22647,#22648,#22649));
#5290=EDGE_LOOP('',(#22650,#22651,#22652,#22653,#22654,#22655,#22656,#22657));
#5291=EDGE_LOOP('',(#22658,#22659,#22660,#22661,#22662,#22663,#22664,#22665));
#5292=EDGE_LOOP('',(#22666,#22667,#22668,#22669,#22670,#22671,#22672,#22673));
#5293=EDGE_LOOP('',(#22674,#22675,#22676,#22677,#22678,#22679,#22680,#22681));
#5294=EDGE_LOOP('',(#22682,#22683,#22684,#22685,#22686,#22687,#22688,#22689));
#5295=EDGE_LOOP('',(#22690,#22691,#22692,#22693,#22694,#22695,#22696,#22697));
#5296=EDGE_LOOP('',(#22698,#22699,#22700,#22701,#22702,#22703,#22704,#22705));
#5297=EDGE_LOOP('',(#22706,#22707,#22708,#22709,#22710,#22711,#22712,#22713));
#5298=EDGE_LOOP('',(#22714,#22715,#22716,#22717,#22718,#22719,#22720,#22721));
#5299=EDGE_LOOP('',(#22722,#22723,#22724,#22725,#22726,#22727,#22728,#22729));
#5300=EDGE_LOOP('',(#22730,#22731,#22732,#22733,#22734,#22735,#22736,#22737));
#5301=EDGE_LOOP('',(#22738,#22739,#22740,#22741,#22742,#22743,#22744,#22745));
#5302=EDGE_LOOP('',(#22746,#22747,#22748,#22749,#22750,#22751,#22752,#22753));
#5303=EDGE_LOOP('',(#22754,#22755,#22756,#22757,#22758,#22759,#22760,#22761));
#5304=EDGE_LOOP('',(#22762,#22763,#22764,#22765,#22766,#22767,#22768,#22769));
#5305=EDGE_LOOP('',(#22770,#22771,#22772,#22773,#22774,#22775,#22776,#22777));
#5306=EDGE_LOOP('',(#22778,#22779,#22780,#22781,#22782,#22783,#22784,#22785));
#5307=EDGE_LOOP('',(#22786,#22787,#22788,#22789,#22790,#22791,#22792,#22793));
#5308=EDGE_LOOP('',(#22794,#22795,#22796,#22797,#22798,#22799,#22800,#22801));
#5309=EDGE_LOOP('',(#22802,#22803,#22804,#22805,#22806,#22807,#22808,#22809));
#5310=EDGE_LOOP('',(#22810,#22811,#22812,#22813,#22814,#22815,#22816,#22817));
#5311=EDGE_LOOP('',(#22818,#22819,#22820,#22821,#22822,#22823,#22824,#22825));
#5312=EDGE_LOOP('',(#22826,#22827,#22828,#22829,#22830,#22831,#22832,#22833));
#5313=EDGE_LOOP('',(#22834,#22835,#22836,#22837,#22838,#22839,#22840,#22841));
#5314=EDGE_LOOP('',(#22842,#22843,#22844,#22845,#22846,#22847,#22848,#22849));
#5315=EDGE_LOOP('',(#22850,#22851,#22852,#22853,#22854,#22855,#22856,#22857));
#5316=EDGE_LOOP('',(#22858,#22859,#22860,#22861,#22862,#22863,#22864,#22865));
#5317=EDGE_LOOP('',(#22866,#22867,#22868,#22869,#22870,#22871,#22872,#22873));
#5318=EDGE_LOOP('',(#22874,#22875,#22876,#22877,#22878,#22879,#22880,#22881));
#5319=EDGE_LOOP('',(#22882,#22883,#22884,#22885,#22886,#22887,#22888,#22889));
#5320=EDGE_LOOP('',(#22890,#22891,#22892,#22893,#22894,#22895,#22896,#22897));
#5321=EDGE_LOOP('',(#22898,#22899,#22900,#22901,#22902,#22903,#22904,#22905));
#5322=EDGE_LOOP('',(#22906,#22907,#22908,#22909,#22910,#22911,#22912,#22913));
#5323=EDGE_LOOP('',(#22914,#22915,#22916,#22917,#22918,#22919,#22920,#22921));
#5324=EDGE_LOOP('',(#22922,#22923,#22924,#22925,#22926,#22927,#22928,#22929));
#5325=EDGE_LOOP('',(#22930,#22931,#22932,#22933,#22934,#22935,#22936,#22937));
#5326=EDGE_LOOP('',(#22938,#22939,#22940,#22941,#22942,#22943,#22944,#22945));
#5327=EDGE_LOOP('',(#22946,#22947,#22948,#22949,#22950,#22951,#22952,#22953));
#5328=EDGE_LOOP('',(#22954,#22955,#22956,#22957,#22958,#22959,#22960,#22961));
#5329=EDGE_LOOP('',(#22962,#22963,#22964,#22965,#22966,#22967,#22968,#22969));
#5330=EDGE_LOOP('',(#22970,#22971,#22972,#22973));
#5331=EDGE_LOOP('',(#22974,#22975,#22976,#22977));
#5332=EDGE_LOOP('',(#22978,#22979,#22980,#22981));
#5333=EDGE_LOOP('',(#22982,#22983,#22984,#22985));
#5334=EDGE_LOOP('',(#22986,#22987,#22988,#22989));
#5335=EDGE_LOOP('',(#22990,#22991,#22992,#22993));
#5336=EDGE_LOOP('',(#22994,#22995,#22996,#22997));
#5337=EDGE_LOOP('',(#22998,#22999,#23000,#23001));
#5338=EDGE_LOOP('',(#23002,#23003,#23004,#23005));
#5339=EDGE_LOOP('',(#23006,#23007,#23008,#23009));
#5340=EDGE_LOOP('',(#23010,#23011,#23012,#23013));
#5341=EDGE_LOOP('',(#23014,#23015,#23016,#23017));
#5342=EDGE_LOOP('',(#23018,#23019,#23020,#23021));
#5343=EDGE_LOOP('',(#23022,#23023,#23024,#23025));
#5344=EDGE_LOOP('',(#23026,#23027,#23028,#23029));
#5345=EDGE_LOOP('',(#23030,#23031,#23032,#23033));
#5346=EDGE_LOOP('',(#23034,#23035,#23036,#23037,#23038,#23039,#23040,#23041,
#23042,#23043));
#5347=EDGE_LOOP('',(#23044));
#5348=EDGE_LOOP('',(#23045));
#5349=EDGE_LOOP('',(#23046));
#5350=EDGE_LOOP('',(#23047));
#5351=EDGE_LOOP('',(#23048));
#5352=EDGE_LOOP('',(#23049));
#5353=EDGE_LOOP('',(#23050,#23051,#23052,#23053,#23054));
#5354=EDGE_LOOP('',(#23055,#23056,#23057,#23058));
#5355=EDGE_LOOP('',(#23059,#23060,#23061,#23062,#23063));
#5356=EDGE_LOOP('',(#23064,#23065,#23066,#23067,#23068));
#5357=EDGE_LOOP('',(#23069,#23070,#23071));
#5358=EDGE_LOOP('',(#23072,#23073,#23074));
#5359=EDGE_LOOP('',(#23075,#23076,#23077,#23078));
#5360=EDGE_LOOP('',(#23079,#23080,#23081));
#5361=EDGE_LOOP('',(#23082,#23083,#23084,#23085));
#5362=EDGE_LOOP('',(#23086,#23087,#23088,#23089));
#5363=EDGE_LOOP('',(#23090,#23091,#23092,#23093));
#5364=EDGE_LOOP('',(#23094,#23095,#23096,#23097));
#5365=EDGE_LOOP('',(#23098,#23099,#23100,#23101));
#5366=EDGE_LOOP('',(#23102,#23103,#23104,#23105));
#5367=EDGE_LOOP('',(#23106,#23107,#23108));
#5368=EDGE_LOOP('',(#23109,#23110,#23111));
#5369=EDGE_LOOP('',(#23112,#23113,#23114));
#5370=EDGE_LOOP('',(#23115,#23116,#23117,#23118));
#5371=EDGE_LOOP('',(#23119,#23120,#23121));
#5372=EDGE_LOOP('',(#23122,#23123,#23124,#23125));
#5373=EDGE_LOOP('',(#23126,#23127,#23128,#23129));
#5374=EDGE_LOOP('',(#23130,#23131,#23132,#23133));
#5375=EDGE_LOOP('',(#23134,#23135,#23136,#23137));
#5376=EDGE_LOOP('',(#23138,#23139,#23140,#23141));
#5377=EDGE_LOOP('',(#23142,#23143,#23144,#23145));
#5378=EDGE_LOOP('',(#23146,#23147,#23148,#23149));
#5379=EDGE_LOOP('',(#23150,#23151,#23152,#23153));
#5380=EDGE_LOOP('',(#23154,#23155,#23156,#23157));
#5381=EDGE_LOOP('',(#23158,#23159,#23160,#23161));
#5382=EDGE_LOOP('',(#23162,#23163,#23164));
#5383=EDGE_LOOP('',(#23165,#23166,#23167,#23168,#23169));
#5384=EDGE_LOOP('',(#23170,#23171,#23172,#23173));
#5385=EDGE_LOOP('',(#23174,#23175,#23176));
#5386=EDGE_LOOP('',(#23177,#23178,#23179,#23180,#23181));
#5387=EDGE_LOOP('',(#23182,#23183,#23184,#23185));
#5388=EDGE_LOOP('',(#23186,#23187,#23188,#23189));
#5389=EDGE_LOOP('',(#23190,#23191,#23192,#23193,#23194));
#5390=EDGE_LOOP('',(#23195,#23196,#23197,#23198));
#5391=EDGE_LOOP('',(#23199,#23200,#23201,#23202,#23203,#23204));
#5392=EDGE_LOOP('',(#23205,#23206,#23207,#23208,#23209));
#5393=EDGE_LOOP('',(#23210,#23211,#23212,#23213));
#5394=EDGE_LOOP('',(#23214,#23215,#23216,#23217));
#5395=EDGE_LOOP('',(#23218,#23219,#23220));
#5396=EDGE_LOOP('',(#23221,#23222,#23223));
#5397=EDGE_LOOP('',(#23224,#23225,#23226));
#5398=EDGE_LOOP('',(#23227,#23228,#23229,#23230));
#5399=EDGE_LOOP('',(#23231,#23232,#23233));
#5400=EDGE_LOOP('',(#23234,#23235,#23236,#23237));
#5401=EDGE_LOOP('',(#23238,#23239,#23240,#23241));
#5402=EDGE_LOOP('',(#23242,#23243,#23244,#23245));
#5403=EDGE_LOOP('',(#23246,#23247,#23248,#23249));
#5404=EDGE_LOOP('',(#23250,#23251,#23252,#23253));
#5405=EDGE_LOOP('',(#23254,#23255,#23256,#23257));
#5406=EDGE_LOOP('',(#23258,#23259,#23260,#23261));
#5407=EDGE_LOOP('',(#23262,#23263,#23264,#23265));
#5408=EDGE_LOOP('',(#23266,#23267,#23268,#23269));
#5409=EDGE_LOOP('',(#23270,#23271,#23272,#23273));
#5410=EDGE_LOOP('',(#23274,#23275,#23276));
#5411=EDGE_LOOP('',(#23277,#23278,#23279));
#5412=EDGE_LOOP('',(#23280,#23281,#23282));
#5413=EDGE_LOOP('',(#23283,#23284,#23285,#23286));
#5414=EDGE_LOOP('',(#23287,#23288,#23289));
#5415=EDGE_LOOP('',(#23290,#23291,#23292,#23293));
#5416=EDGE_LOOP('',(#23294,#23295,#23296,#23297));
#5417=EDGE_LOOP('',(#23298,#23299,#23300,#23301));
#5418=EDGE_LOOP('',(#23302,#23303,#23304,#23305));
#5419=EDGE_LOOP('',(#23306,#23307,#23308,#23309));
#5420=EDGE_LOOP('',(#23310,#23311,#23312,#23313));
#5421=EDGE_LOOP('',(#23314,#23315,#23316,#23317));
#5422=EDGE_LOOP('',(#23318,#23319,#23320,#23321));
#5423=EDGE_LOOP('',(#23322,#23323,#23324,#23325));
#5424=EDGE_LOOP('',(#23326,#23327,#23328,#23329));
#5425=EDGE_LOOP('',(#23330,#23331,#23332,#23333,#23334));
#5426=EDGE_LOOP('',(#23335,#23336,#23337,#23338));
#5427=EDGE_LOOP('',(#23339,#23340,#23341,#23342,#23343));
#5428=EDGE_LOOP('',(#23344,#23345,#23346,#23347,#23348));
#5429=EDGE_LOOP('',(#23349,#23350,#23351));
#5430=EDGE_LOOP('',(#23352,#23353,#23354));
#5431=EDGE_LOOP('',(#23355,#23356,#23357,#23358));
#5432=EDGE_LOOP('',(#23359,#23360,#23361));
#5433=EDGE_LOOP('',(#23362,#23363,#23364,#23365));
#5434=EDGE_LOOP('',(#23366,#23367,#23368,#23369));
#5435=EDGE_LOOP('',(#23370,#23371,#23372,#23373));
#5436=EDGE_LOOP('',(#23374,#23375,#23376,#23377));
#5437=EDGE_LOOP('',(#23378,#23379,#23380,#23381));
#5438=EDGE_LOOP('',(#23382,#23383,#23384,#23385));
#5439=EDGE_LOOP('',(#23386,#23387,#23388));
#5440=EDGE_LOOP('',(#23389,#23390,#23391));
#5441=EDGE_LOOP('',(#23392,#23393,#23394));
#5442=EDGE_LOOP('',(#23395,#23396,#23397,#23398));
#5443=EDGE_LOOP('',(#23399,#23400,#23401));
#5444=EDGE_LOOP('',(#23402,#23403,#23404,#23405));
#5445=EDGE_LOOP('',(#23406,#23407,#23408,#23409));
#5446=EDGE_LOOP('',(#23410,#23411,#23412,#23413));
#5447=EDGE_LOOP('',(#23414,#23415,#23416,#23417));
#5448=EDGE_LOOP('',(#23418,#23419,#23420,#23421));
#5449=EDGE_LOOP('',(#23422,#23423,#23424,#23425));
#5450=EDGE_LOOP('',(#23426,#23427,#23428,#23429));
#5451=EDGE_LOOP('',(#23430,#23431,#23432,#23433));
#5452=EDGE_LOOP('',(#23434,#23435,#23436,#23437));
#5453=EDGE_LOOP('',(#23438,#23439,#23440,#23441));
#5454=EDGE_LOOP('',(#23442,#23443,#23444));
#5455=EDGE_LOOP('',(#23445,#23446,#23447,#23448,#23449));
#5456=EDGE_LOOP('',(#23450,#23451,#23452,#23453));
#5457=EDGE_LOOP('',(#23454,#23455,#23456));
#5458=EDGE_LOOP('',(#23457,#23458,#23459,#23460,#23461));
#5459=EDGE_LOOP('',(#23462,#23463,#23464,#23465));
#5460=EDGE_LOOP('',(#23466,#23467,#23468,#23469));
#5461=EDGE_LOOP('',(#23470,#23471,#23472,#23473,#23474));
#5462=EDGE_LOOP('',(#23475,#23476,#23477,#23478));
#5463=EDGE_LOOP('',(#23479,#23480,#23481,#23482,#23483,#23484));
#5464=EDGE_LOOP('',(#23485,#23486,#23487,#23488,#23489));
#5465=EDGE_LOOP('',(#23490,#23491,#23492,#23493));
#5466=EDGE_LOOP('',(#23494,#23495,#23496,#23497));
#5467=EDGE_LOOP('',(#23498,#23499,#23500));
#5468=EDGE_LOOP('',(#23501,#23502,#23503));
#5469=EDGE_LOOP('',(#23504,#23505,#23506));
#5470=EDGE_LOOP('',(#23507,#23508,#23509,#23510));
#5471=EDGE_LOOP('',(#23511,#23512,#23513));
#5472=EDGE_LOOP('',(#23514,#23515,#23516,#23517));
#5473=EDGE_LOOP('',(#23518,#23519,#23520,#23521));
#5474=EDGE_LOOP('',(#23522,#23523,#23524,#23525));
#5475=EDGE_LOOP('',(#23526,#23527,#23528,#23529));
#5476=EDGE_LOOP('',(#23530,#23531,#23532,#23533));
#5477=EDGE_LOOP('',(#23534,#23535,#23536,#23537));
#5478=EDGE_LOOP('',(#23538,#23539,#23540,#23541));
#5479=EDGE_LOOP('',(#23542,#23543,#23544,#23545));
#5480=EDGE_LOOP('',(#23546,#23547,#23548,#23549));
#5481=EDGE_LOOP('',(#23550,#23551,#23552,#23553));
#5482=EDGE_LOOP('',(#23554,#23555,#23556));
#5483=EDGE_LOOP('',(#23557,#23558,#23559));
#5484=EDGE_LOOP('',(#23560,#23561,#23562));
#5485=EDGE_LOOP('',(#23563,#23564,#23565,#23566));
#5486=EDGE_LOOP('',(#23567,#23568,#23569));
#5487=EDGE_LOOP('',(#23570,#23571,#23572,#23573));
#5488=EDGE_LOOP('',(#23574,#23575,#23576,#23577));
#5489=EDGE_LOOP('',(#23578,#23579,#23580,#23581));
#5490=EDGE_LOOP('',(#23582,#23583,#23584,#23585));
#5491=EDGE_LOOP('',(#23586,#23587,#23588,#23589));
#5492=EDGE_LOOP('',(#23590,#23591,#23592,#23593));
#5493=EDGE_LOOP('',(#23594,#23595,#23596,#23597));
#5494=EDGE_LOOP('',(#23598,#23599,#23600,#23601));
#5495=EDGE_LOOP('',(#23602,#23603,#23604,#23605));
#5496=EDGE_LOOP('',(#23606,#23607,#23608,#23609));
#5497=EDGE_LOOP('',(#23610,#23611,#23612,#23613,#23614));
#5498=EDGE_LOOP('',(#23615,#23616,#23617,#23618));
#5499=EDGE_LOOP('',(#23619,#23620,#23621,#23622,#23623));
#5500=EDGE_LOOP('',(#23624,#23625,#23626,#23627,#23628));
#5501=EDGE_LOOP('',(#23629,#23630,#23631));
#5502=EDGE_LOOP('',(#23632,#23633,#23634));
#5503=EDGE_LOOP('',(#23635,#23636,#23637,#23638));
#5504=EDGE_LOOP('',(#23639,#23640,#23641));
#5505=EDGE_LOOP('',(#23642,#23643,#23644,#23645));
#5506=EDGE_LOOP('',(#23646,#23647,#23648,#23649));
#5507=EDGE_LOOP('',(#23650,#23651,#23652,#23653));
#5508=EDGE_LOOP('',(#23654,#23655,#23656,#23657));
#5509=EDGE_LOOP('',(#23658,#23659,#23660,#23661));
#5510=EDGE_LOOP('',(#23662,#23663,#23664,#23665));
#5511=EDGE_LOOP('',(#23666,#23667,#23668));
#5512=EDGE_LOOP('',(#23669,#23670,#23671));
#5513=EDGE_LOOP('',(#23672,#23673,#23674));
#5514=EDGE_LOOP('',(#23675,#23676,#23677,#23678));
#5515=EDGE_LOOP('',(#23679,#23680,#23681));
#5516=EDGE_LOOP('',(#23682,#23683,#23684,#23685));
#5517=EDGE_LOOP('',(#23686,#23687,#23688,#23689));
#5518=EDGE_LOOP('',(#23690,#23691,#23692,#23693));
#5519=EDGE_LOOP('',(#23694,#23695,#23696,#23697));
#5520=EDGE_LOOP('',(#23698,#23699,#23700,#23701));
#5521=EDGE_LOOP('',(#23702,#23703,#23704,#23705));
#5522=EDGE_LOOP('',(#23706,#23707,#23708,#23709));
#5523=EDGE_LOOP('',(#23710,#23711,#23712,#23713));
#5524=EDGE_LOOP('',(#23714,#23715,#23716,#23717));
#5525=EDGE_LOOP('',(#23718,#23719,#23720,#23721));
#5526=EDGE_LOOP('',(#23722,#23723,#23724));
#5527=EDGE_LOOP('',(#23725,#23726,#23727,#23728,#23729));
#5528=EDGE_LOOP('',(#23730,#23731,#23732,#23733));
#5529=EDGE_LOOP('',(#23734,#23735,#23736));
#5530=EDGE_LOOP('',(#23737,#23738,#23739,#23740,#23741));
#5531=EDGE_LOOP('',(#23742,#23743,#23744,#23745));
#5532=EDGE_LOOP('',(#23746,#23747,#23748,#23749));
#5533=EDGE_LOOP('',(#23750,#23751,#23752,#23753,#23754));
#5534=EDGE_LOOP('',(#23755,#23756,#23757,#23758));
#5535=EDGE_LOOP('',(#23759,#23760,#23761,#23762,#23763,#23764));
#5536=EDGE_LOOP('',(#23765,#23766,#23767,#23768,#23769));
#5537=EDGE_LOOP('',(#23770,#23771,#23772,#23773));
#5538=EDGE_LOOP('',(#23774,#23775,#23776,#23777));
#5539=EDGE_LOOP('',(#23778,#23779,#23780));
#5540=EDGE_LOOP('',(#23781,#23782,#23783));
#5541=EDGE_LOOP('',(#23784,#23785,#23786));
#5542=EDGE_LOOP('',(#23787,#23788,#23789,#23790));
#5543=EDGE_LOOP('',(#23791,#23792,#23793));
#5544=EDGE_LOOP('',(#23794,#23795,#23796,#23797));
#5545=EDGE_LOOP('',(#23798,#23799,#23800,#23801));
#5546=EDGE_LOOP('',(#23802,#23803,#23804,#23805));
#5547=EDGE_LOOP('',(#23806,#23807,#23808,#23809));
#5548=EDGE_LOOP('',(#23810,#23811,#23812,#23813));
#5549=EDGE_LOOP('',(#23814,#23815,#23816,#23817));
#5550=EDGE_LOOP('',(#23818,#23819,#23820,#23821));
#5551=EDGE_LOOP('',(#23822,#23823,#23824,#23825));
#5552=EDGE_LOOP('',(#23826,#23827,#23828,#23829));
#5553=EDGE_LOOP('',(#23830,#23831,#23832,#23833));
#5554=EDGE_LOOP('',(#23834,#23835,#23836));
#5555=EDGE_LOOP('',(#23837,#23838,#23839));
#5556=EDGE_LOOP('',(#23840,#23841,#23842));
#5557=EDGE_LOOP('',(#23843,#23844,#23845,#23846));
#5558=EDGE_LOOP('',(#23847,#23848,#23849));
#5559=EDGE_LOOP('',(#23850,#23851,#23852,#23853));
#5560=EDGE_LOOP('',(#23854,#23855,#23856,#23857));
#5561=EDGE_LOOP('',(#23858,#23859,#23860,#23861));
#5562=EDGE_LOOP('',(#23862,#23863,#23864,#23865));
#5563=EDGE_LOOP('',(#23866,#23867,#23868,#23869));
#5564=EDGE_LOOP('',(#23870,#23871,#23872,#23873));
#5565=EDGE_LOOP('',(#23874,#23875,#23876,#23877));
#5566=EDGE_LOOP('',(#23878,#23879,#23880,#23881));
#5567=EDGE_LOOP('',(#23882,#23883,#23884,#23885));
#5568=EDGE_LOOP('',(#23886,#23887,#23888,#23889));
#5569=EDGE_LOOP('',(#23890,#23891,#23892,#23893,#23894));
#5570=EDGE_LOOP('',(#23895,#23896,#23897,#23898));
#5571=EDGE_LOOP('',(#23899,#23900,#23901,#23902,#23903));
#5572=EDGE_LOOP('',(#23904,#23905,#23906,#23907,#23908));
#5573=EDGE_LOOP('',(#23909,#23910,#23911));
#5574=EDGE_LOOP('',(#23912,#23913,#23914));
#5575=EDGE_LOOP('',(#23915,#23916,#23917,#23918));
#5576=EDGE_LOOP('',(#23919,#23920,#23921));
#5577=EDGE_LOOP('',(#23922,#23923,#23924,#23925));
#5578=EDGE_LOOP('',(#23926,#23927,#23928,#23929));
#5579=EDGE_LOOP('',(#23930,#23931,#23932,#23933));
#5580=EDGE_LOOP('',(#23934,#23935,#23936,#23937));
#5581=EDGE_LOOP('',(#23938,#23939,#23940,#23941));
#5582=EDGE_LOOP('',(#23942,#23943,#23944,#23945));
#5583=EDGE_LOOP('',(#23946,#23947,#23948));
#5584=EDGE_LOOP('',(#23949,#23950,#23951));
#5585=EDGE_LOOP('',(#23952,#23953,#23954));
#5586=EDGE_LOOP('',(#23955,#23956,#23957,#23958));
#5587=EDGE_LOOP('',(#23959,#23960,#23961));
#5588=EDGE_LOOP('',(#23962,#23963,#23964,#23965));
#5589=EDGE_LOOP('',(#23966,#23967,#23968,#23969));
#5590=EDGE_LOOP('',(#23970,#23971,#23972,#23973));
#5591=EDGE_LOOP('',(#23974,#23975,#23976,#23977));
#5592=EDGE_LOOP('',(#23978,#23979,#23980,#23981));
#5593=EDGE_LOOP('',(#23982,#23983,#23984,#23985));
#5594=EDGE_LOOP('',(#23986,#23987,#23988,#23989));
#5595=EDGE_LOOP('',(#23990,#23991,#23992,#23993));
#5596=EDGE_LOOP('',(#23994,#23995,#23996,#23997));
#5597=EDGE_LOOP('',(#23998,#23999,#24000,#24001));
#5598=EDGE_LOOP('',(#24002,#24003,#24004));
#5599=EDGE_LOOP('',(#24005,#24006,#24007,#24008,#24009));
#5600=EDGE_LOOP('',(#24010,#24011,#24012,#24013));
#5601=EDGE_LOOP('',(#24014,#24015,#24016));
#5602=EDGE_LOOP('',(#24017,#24018,#24019,#24020,#24021));
#5603=EDGE_LOOP('',(#24022,#24023,#24024,#24025));
#5604=EDGE_LOOP('',(#24026,#24027,#24028,#24029));
#5605=EDGE_LOOP('',(#24030,#24031,#24032,#24033,#24034));
#5606=EDGE_LOOP('',(#24035,#24036,#24037,#24038));
#5607=EDGE_LOOP('',(#24039,#24040,#24041,#24042,#24043,#24044));
#5608=EDGE_LOOP('',(#24045,#24046,#24047,#24048,#24049));
#5609=EDGE_LOOP('',(#24050,#24051,#24052,#24053));
#5610=EDGE_LOOP('',(#24054,#24055,#24056,#24057));
#5611=EDGE_LOOP('',(#24058,#24059,#24060));
#5612=EDGE_LOOP('',(#24061,#24062,#24063));
#5613=EDGE_LOOP('',(#24064,#24065,#24066));
#5614=EDGE_LOOP('',(#24067,#24068,#24069,#24070));
#5615=EDGE_LOOP('',(#24071,#24072,#24073));
#5616=EDGE_LOOP('',(#24074,#24075,#24076,#24077));
#5617=EDGE_LOOP('',(#24078,#24079,#24080,#24081));
#5618=EDGE_LOOP('',(#24082,#24083,#24084,#24085));
#5619=EDGE_LOOP('',(#24086,#24087,#24088,#24089));
#5620=EDGE_LOOP('',(#24090,#24091,#24092,#24093));
#5621=EDGE_LOOP('',(#24094,#24095,#24096,#24097));
#5622=EDGE_LOOP('',(#24098,#24099,#24100,#24101));
#5623=EDGE_LOOP('',(#24102,#24103,#24104,#24105,#24106));
#5624=EDGE_LOOP('',(#24107,#24108,#24109,#24110));
#5625=EDGE_LOOP('',(#24111,#24112,#24113,#24114));
#5626=EDGE_LOOP('',(#24115,#24116,#24117));
#5627=EDGE_LOOP('',(#24118,#24119,#24120));
#5628=EDGE_LOOP('',(#24121,#24122,#24123));
#5629=EDGE_LOOP('',(#24124,#24125,#24126,#24127));
#5630=EDGE_LOOP('',(#24128,#24129,#24130));
#5631=EDGE_LOOP('',(#24131,#24132,#24133,#24134));
#5632=EDGE_LOOP('',(#24135,#24136,#24137,#24138));
#5633=EDGE_LOOP('',(#24139,#24140,#24141,#24142));
#5634=EDGE_LOOP('',(#24143,#24144,#24145,#24146));
#5635=EDGE_LOOP('',(#24147,#24148,#24149,#24150));
#5636=EDGE_LOOP('',(#24151,#24152,#24153,#24154));
#5637=EDGE_LOOP('',(#24155,#24156,#24157,#24158));
#5638=EDGE_LOOP('',(#24159,#24160,#24161,#24162));
#5639=EDGE_LOOP('',(#24163,#24164,#24165,#24166));
#5640=EDGE_LOOP('',(#24167,#24168,#24169,#24170));
#5641=EDGE_LOOP('',(#24171,#24172,#24173,#24174,#24175));
#5642=EDGE_LOOP('',(#24176,#24177,#24178,#24179));
#5643=EDGE_LOOP('',(#24180,#24181,#24182,#24183,#24184));
#5644=EDGE_LOOP('',(#24185,#24186,#24187,#24188,#24189));
#5645=EDGE_LOOP('',(#24190,#24191,#24192));
#5646=EDGE_LOOP('',(#24193,#24194,#24195));
#5647=EDGE_LOOP('',(#24196,#24197,#24198,#24199));
#5648=EDGE_LOOP('',(#24200,#24201,#24202));
#5649=EDGE_LOOP('',(#24203,#24204,#24205,#24206));
#5650=EDGE_LOOP('',(#24207,#24208,#24209,#24210));
#5651=EDGE_LOOP('',(#24211,#24212,#24213,#24214));
#5652=EDGE_LOOP('',(#24215,#24216,#24217,#24218));
#5653=EDGE_LOOP('',(#24219,#24220,#24221,#24222));
#5654=EDGE_LOOP('',(#24223,#24224,#24225,#24226));
#5655=EDGE_LOOP('',(#24227,#24228,#24229));
#5656=EDGE_LOOP('',(#24230,#24231,#24232));
#5657=EDGE_LOOP('',(#24233,#24234,#24235));
#5658=EDGE_LOOP('',(#24236,#24237,#24238,#24239));
#5659=EDGE_LOOP('',(#24240,#24241,#24242));
#5660=EDGE_LOOP('',(#24243,#24244,#24245,#24246));
#5661=EDGE_LOOP('',(#24247,#24248,#24249,#24250));
#5662=EDGE_LOOP('',(#24251,#24252,#24253,#24254));
#5663=EDGE_LOOP('',(#24255,#24256,#24257,#24258));
#5664=EDGE_LOOP('',(#24259,#24260,#24261,#24262));
#5665=EDGE_LOOP('',(#24263,#24264,#24265,#24266));
#5666=EDGE_LOOP('',(#24267,#24268,#24269,#24270));
#5667=EDGE_LOOP('',(#24271,#24272,#24273,#24274));
#5668=EDGE_LOOP('',(#24275,#24276,#24277,#24278));
#5669=EDGE_LOOP('',(#24279,#24280,#24281,#24282));
#5670=EDGE_LOOP('',(#24283,#24284,#24285));
#5671=EDGE_LOOP('',(#24286,#24287,#24288,#24289,#24290));
#5672=EDGE_LOOP('',(#24291,#24292,#24293,#24294));
#5673=EDGE_LOOP('',(#24295,#24296,#24297));
#5674=EDGE_LOOP('',(#24298,#24299,#24300,#24301,#24302));
#5675=EDGE_LOOP('',(#24303,#24304,#24305,#24306));
#5676=EDGE_LOOP('',(#24307,#24308,#24309,#24310));
#5677=EDGE_LOOP('',(#24311,#24312,#24313,#24314,#24315));
#5678=EDGE_LOOP('',(#24316,#24317,#24318,#24319));
#5679=EDGE_LOOP('',(#24320,#24321,#24322,#24323,#24324,#24325));
#5680=EDGE_LOOP('',(#24326,#24327,#24328,#24329,#24330));
#5681=EDGE_LOOP('',(#24331,#24332,#24333,#24334));
#5682=EDGE_LOOP('',(#24335,#24336,#24337,#24338));
#5683=EDGE_LOOP('',(#24339,#24340,#24341));
#5684=EDGE_LOOP('',(#24342,#24343,#24344));
#5685=EDGE_LOOP('',(#24345,#24346,#24347));
#5686=EDGE_LOOP('',(#24348,#24349,#24350,#24351));
#5687=EDGE_LOOP('',(#24352,#24353,#24354));
#5688=EDGE_LOOP('',(#24355,#24356,#24357,#24358));
#5689=EDGE_LOOP('',(#24359,#24360,#24361,#24362));
#5690=EDGE_LOOP('',(#24363,#24364,#24365,#24366));
#5691=EDGE_LOOP('',(#24367,#24368,#24369,#24370));
#5692=EDGE_LOOP('',(#24371,#24372,#24373,#24374));
#5693=EDGE_LOOP('',(#24375,#24376,#24377,#24378));
#5694=EDGE_LOOP('',(#24379,#24380,#24381,#24382));
#5695=EDGE_LOOP('',(#24383,#24384,#24385,#24386));
#5696=EDGE_LOOP('',(#24387,#24388,#24389,#24390));
#5697=EDGE_LOOP('',(#24391,#24392,#24393,#24394));
#5698=EDGE_LOOP('',(#24395,#24396,#24397));
#5699=EDGE_LOOP('',(#24398,#24399,#24400));
#5700=EDGE_LOOP('',(#24401,#24402,#24403));
#5701=EDGE_LOOP('',(#24404,#24405,#24406,#24407));
#5702=EDGE_LOOP('',(#24408,#24409,#24410));
#5703=EDGE_LOOP('',(#24411,#24412,#24413,#24414));
#5704=EDGE_LOOP('',(#24415,#24416,#24417,#24418));
#5705=EDGE_LOOP('',(#24419,#24420,#24421,#24422));
#5706=EDGE_LOOP('',(#24423,#24424,#24425,#24426));
#5707=EDGE_LOOP('',(#24427,#24428,#24429,#24430));
#5708=EDGE_LOOP('',(#24431,#24432,#24433,#24434));
#5709=EDGE_LOOP('',(#24435,#24436,#24437,#24438));
#5710=EDGE_LOOP('',(#24439,#24440,#24441,#24442));
#5711=EDGE_LOOP('',(#24443,#24444,#24445,#24446));
#5712=EDGE_LOOP('',(#24447,#24448,#24449,#24450));
#5713=EDGE_LOOP('',(#24451,#24452,#24453,#24454,#24455));
#5714=EDGE_LOOP('',(#24456,#24457,#24458,#24459));
#5715=EDGE_LOOP('',(#24460,#24461,#24462,#24463,#24464));
#5716=EDGE_LOOP('',(#24465,#24466,#24467,#24468,#24469));
#5717=EDGE_LOOP('',(#24470,#24471,#24472));
#5718=EDGE_LOOP('',(#24473,#24474,#24475));
#5719=EDGE_LOOP('',(#24476,#24477,#24478,#24479));
#5720=EDGE_LOOP('',(#24480,#24481,#24482));
#5721=EDGE_LOOP('',(#24483,#24484,#24485,#24486));
#5722=EDGE_LOOP('',(#24487,#24488,#24489,#24490));
#5723=EDGE_LOOP('',(#24491,#24492,#24493,#24494));
#5724=EDGE_LOOP('',(#24495,#24496,#24497,#24498));
#5725=EDGE_LOOP('',(#24499,#24500,#24501,#24502));
#5726=EDGE_LOOP('',(#24503,#24504,#24505,#24506));
#5727=EDGE_LOOP('',(#24507,#24508,#24509));
#5728=EDGE_LOOP('',(#24510,#24511,#24512));
#5729=EDGE_LOOP('',(#24513,#24514,#24515));
#5730=EDGE_LOOP('',(#24516,#24517,#24518,#24519));
#5731=EDGE_LOOP('',(#24520,#24521,#24522));
#5732=EDGE_LOOP('',(#24523,#24524,#24525,#24526));
#5733=EDGE_LOOP('',(#24527,#24528,#24529,#24530));
#5734=EDGE_LOOP('',(#24531,#24532,#24533,#24534));
#5735=EDGE_LOOP('',(#24535,#24536,#24537,#24538));
#5736=EDGE_LOOP('',(#24539,#24540,#24541,#24542));
#5737=EDGE_LOOP('',(#24543,#24544,#24545,#24546));
#5738=EDGE_LOOP('',(#24547,#24548,#24549,#24550));
#5739=EDGE_LOOP('',(#24551,#24552,#24553,#24554));
#5740=EDGE_LOOP('',(#24555,#24556,#24557,#24558));
#5741=EDGE_LOOP('',(#24559,#24560,#24561,#24562));
#5742=EDGE_LOOP('',(#24563,#24564,#24565));
#5743=EDGE_LOOP('',(#24566,#24567,#24568,#24569,#24570));
#5744=EDGE_LOOP('',(#24571,#24572,#24573,#24574));
#5745=EDGE_LOOP('',(#24575,#24576,#24577));
#5746=EDGE_LOOP('',(#24578,#24579,#24580,#24581,#24582));
#5747=EDGE_LOOP('',(#24583,#24584,#24585,#24586));
#5748=EDGE_LOOP('',(#24587,#24588,#24589,#24590));
#5749=EDGE_LOOP('',(#24591,#24592,#24593,#24594,#24595));
#5750=EDGE_LOOP('',(#24596,#24597,#24598,#24599));
#5751=EDGE_LOOP('',(#24600,#24601,#24602,#24603,#24604,#24605));
#5752=EDGE_LOOP('',(#24606,#24607,#24608,#24609,#24610));
#5753=EDGE_LOOP('',(#24611,#24612,#24613,#24614));
#5754=EDGE_LOOP('',(#24615,#24616,#24617,#24618));
#5755=EDGE_LOOP('',(#24619,#24620,#24621));
#5756=EDGE_LOOP('',(#24622,#24623,#24624));
#5757=EDGE_LOOP('',(#24625,#24626,#24627));
#5758=EDGE_LOOP('',(#24628,#24629,#24630,#24631));
#5759=EDGE_LOOP('',(#24632,#24633,#24634));
#5760=EDGE_LOOP('',(#24635,#24636,#24637,#24638));
#5761=EDGE_LOOP('',(#24639,#24640,#24641,#24642));
#5762=EDGE_LOOP('',(#24643,#24644,#24645,#24646));
#5763=EDGE_LOOP('',(#24647,#24648,#24649,#24650));
#5764=EDGE_LOOP('',(#24651,#24652,#24653,#24654));
#5765=EDGE_LOOP('',(#24655,#24656,#24657,#24658));
#5766=EDGE_LOOP('',(#24659,#24660,#24661,#24662));
#5767=EDGE_LOOP('',(#24663,#24664,#24665,#24666));
#5768=EDGE_LOOP('',(#24667,#24668,#24669,#24670));
#5769=EDGE_LOOP('',(#24671,#24672,#24673,#24674));
#5770=EDGE_LOOP('',(#24675,#24676,#24677));
#5771=EDGE_LOOP('',(#24678,#24679,#24680));
#5772=EDGE_LOOP('',(#24681,#24682,#24683));
#5773=EDGE_LOOP('',(#24684,#24685,#24686,#24687));
#5774=EDGE_LOOP('',(#24688,#24689,#24690));
#5775=EDGE_LOOP('',(#24691,#24692,#24693,#24694));
#5776=EDGE_LOOP('',(#24695,#24696,#24697,#24698));
#5777=EDGE_LOOP('',(#24699,#24700,#24701,#24702));
#5778=EDGE_LOOP('',(#24703,#24704,#24705,#24706));
#5779=EDGE_LOOP('',(#24707,#24708,#24709,#24710));
#5780=EDGE_LOOP('',(#24711,#24712,#24713,#24714));
#5781=EDGE_LOOP('',(#24715,#24716,#24717,#24718));
#5782=EDGE_LOOP('',(#24719,#24720,#24721,#24722));
#5783=EDGE_LOOP('',(#24723,#24724,#24725,#24726));
#5784=EDGE_LOOP('',(#24727,#24728,#24729,#24730));
#5785=EDGE_LOOP('',(#24731,#24732,#24733,#24734,#24735));
#5786=EDGE_LOOP('',(#24736,#24737,#24738,#24739));
#5787=EDGE_LOOP('',(#24740,#24741,#24742,#24743,#24744));
#5788=EDGE_LOOP('',(#24745,#24746,#24747,#24748,#24749));
#5789=EDGE_LOOP('',(#24750,#24751,#24752));
#5790=EDGE_LOOP('',(#24753,#24754,#24755));
#5791=EDGE_LOOP('',(#24756,#24757,#24758,#24759));
#5792=EDGE_LOOP('',(#24760,#24761,#24762));
#5793=EDGE_LOOP('',(#24763,#24764,#24765,#24766));
#5794=EDGE_LOOP('',(#24767,#24768,#24769,#24770));
#5795=EDGE_LOOP('',(#24771,#24772,#24773,#24774));
#5796=EDGE_LOOP('',(#24775,#24776,#24777,#24778));
#5797=EDGE_LOOP('',(#24779,#24780,#24781,#24782));
#5798=EDGE_LOOP('',(#24783,#24784,#24785,#24786));
#5799=EDGE_LOOP('',(#24787,#24788,#24789));
#5800=EDGE_LOOP('',(#24790,#24791,#24792));
#5801=EDGE_LOOP('',(#24793,#24794,#24795));
#5802=EDGE_LOOP('',(#24796,#24797,#24798,#24799));
#5803=EDGE_LOOP('',(#24800,#24801,#24802));
#5804=EDGE_LOOP('',(#24803,#24804,#24805,#24806));
#5805=EDGE_LOOP('',(#24807,#24808,#24809,#24810));
#5806=EDGE_LOOP('',(#24811,#24812,#24813,#24814));
#5807=EDGE_LOOP('',(#24815,#24816,#24817,#24818));
#5808=EDGE_LOOP('',(#24819,#24820,#24821,#24822));
#5809=EDGE_LOOP('',(#24823,#24824,#24825,#24826));
#5810=EDGE_LOOP('',(#24827,#24828,#24829,#24830));
#5811=EDGE_LOOP('',(#24831,#24832,#24833,#24834));
#5812=EDGE_LOOP('',(#24835,#24836,#24837,#24838));
#5813=EDGE_LOOP('',(#24839,#24840,#24841,#24842));
#5814=EDGE_LOOP('',(#24843,#24844,#24845));
#5815=EDGE_LOOP('',(#24846,#24847,#24848,#24849,#24850));
#5816=EDGE_LOOP('',(#24851,#24852,#24853,#24854));
#5817=EDGE_LOOP('',(#24855,#24856,#24857));
#5818=EDGE_LOOP('',(#24858,#24859,#24860,#24861,#24862));
#5819=EDGE_LOOP('',(#24863,#24864,#24865,#24866));
#5820=EDGE_LOOP('',(#24867,#24868,#24869,#24870));
#5821=EDGE_LOOP('',(#24871,#24872,#24873,#24874,#24875));
#5822=EDGE_LOOP('',(#24876,#24877,#24878,#24879));
#5823=EDGE_LOOP('',(#24880,#24881,#24882,#24883,#24884,#24885));
#5824=EDGE_LOOP('',(#24886,#24887,#24888,#24889,#24890));
#5825=EDGE_LOOP('',(#24891,#24892,#24893,#24894));
#5826=EDGE_LOOP('',(#24895,#24896,#24897,#24898));
#5827=EDGE_LOOP('',(#24899,#24900,#24901));
#5828=EDGE_LOOP('',(#24902,#24903,#24904));
#5829=EDGE_LOOP('',(#24905,#24906,#24907));
#5830=EDGE_LOOP('',(#24908,#24909,#24910,#24911));
#5831=EDGE_LOOP('',(#24912,#24913,#24914));
#5832=EDGE_LOOP('',(#24915,#24916,#24917,#24918));
#5833=EDGE_LOOP('',(#24919,#24920,#24921,#24922));
#5834=EDGE_LOOP('',(#24923,#24924,#24925,#24926));
#5835=EDGE_LOOP('',(#24927,#24928,#24929,#24930));
#5836=EDGE_LOOP('',(#24931,#24932,#24933,#24934));
#5837=EDGE_LOOP('',(#24935,#24936,#24937,#24938));
#5838=EDGE_LOOP('',(#24939,#24940,#24941,#24942));
#5839=EDGE_LOOP('',(#24943,#24944,#24945,#24946));
#5840=EDGE_LOOP('',(#24947,#24948,#24949,#24950));
#5841=EDGE_LOOP('',(#24951,#24952,#24953,#24954));
#5842=EDGE_LOOP('',(#24955,#24956,#24957));
#5843=EDGE_LOOP('',(#24958,#24959,#24960));
#5844=EDGE_LOOP('',(#24961,#24962,#24963));
#5845=EDGE_LOOP('',(#24964,#24965,#24966,#24967));
#5846=EDGE_LOOP('',(#24968,#24969,#24970));
#5847=EDGE_LOOP('',(#24971,#24972,#24973,#24974));
#5848=EDGE_LOOP('',(#24975,#24976,#24977,#24978));
#5849=EDGE_LOOP('',(#24979,#24980,#24981,#24982));
#5850=EDGE_LOOP('',(#24983,#24984,#24985,#24986));
#5851=EDGE_LOOP('',(#24987,#24988,#24989,#24990));
#5852=EDGE_LOOP('',(#24991,#24992,#24993,#24994));
#5853=EDGE_LOOP('',(#24995,#24996,#24997,#24998));
#5854=EDGE_LOOP('',(#24999,#25000,#25001,#25002));
#5855=EDGE_LOOP('',(#25003,#25004,#25005,#25006));
#5856=EDGE_LOOP('',(#25007,#25008,#25009,#25010));
#5857=EDGE_LOOP('',(#25011,#25012,#25013,#25014,#25015));
#5858=EDGE_LOOP('',(#25016,#25017,#25018,#25019));
#5859=EDGE_LOOP('',(#25020,#25021,#25022,#25023,#25024));
#5860=EDGE_LOOP('',(#25025,#25026,#25027,#25028,#25029));
#5861=EDGE_LOOP('',(#25030,#25031,#25032));
#5862=EDGE_LOOP('',(#25033,#25034,#25035));
#5863=EDGE_LOOP('',(#25036,#25037,#25038,#25039));
#5864=EDGE_LOOP('',(#25040,#25041,#25042));
#5865=EDGE_LOOP('',(#25043,#25044,#25045,#25046));
#5866=EDGE_LOOP('',(#25047,#25048,#25049,#25050));
#5867=EDGE_LOOP('',(#25051,#25052,#25053,#25054));
#5868=EDGE_LOOP('',(#25055,#25056,#25057,#25058));
#5869=EDGE_LOOP('',(#25059,#25060,#25061,#25062));
#5870=EDGE_LOOP('',(#25063,#25064,#25065,#25066));
#5871=EDGE_LOOP('',(#25067,#25068,#25069));
#5872=EDGE_LOOP('',(#25070,#25071,#25072));
#5873=EDGE_LOOP('',(#25073,#25074,#25075));
#5874=EDGE_LOOP('',(#25076,#25077,#25078,#25079));
#5875=EDGE_LOOP('',(#25080,#25081,#25082));
#5876=EDGE_LOOP('',(#25083,#25084,#25085,#25086));
#5877=EDGE_LOOP('',(#25087,#25088,#25089,#25090));
#5878=EDGE_LOOP('',(#25091,#25092,#25093,#25094));
#5879=EDGE_LOOP('',(#25095,#25096,#25097,#25098));
#5880=EDGE_LOOP('',(#25099,#25100,#25101,#25102));
#5881=EDGE_LOOP('',(#25103,#25104,#25105,#25106));
#5882=EDGE_LOOP('',(#25107,#25108,#25109,#25110));
#5883=EDGE_LOOP('',(#25111,#25112,#25113,#25114));
#5884=EDGE_LOOP('',(#25115,#25116,#25117,#25118));
#5885=EDGE_LOOP('',(#25119,#25120,#25121,#25122));
#5886=EDGE_LOOP('',(#25123,#25124,#25125));
#5887=EDGE_LOOP('',(#25126,#25127,#25128,#25129,#25130));
#5888=EDGE_LOOP('',(#25131,#25132,#25133,#25134));
#5889=EDGE_LOOP('',(#25135,#25136,#25137));
#5890=EDGE_LOOP('',(#25138,#25139,#25140,#25141,#25142));
#5891=EDGE_LOOP('',(#25143,#25144,#25145,#25146));
#5892=EDGE_LOOP('',(#25147,#25148,#25149,#25150));
#5893=EDGE_LOOP('',(#25151,#25152,#25153,#25154,#25155));
#5894=EDGE_LOOP('',(#25156,#25157,#25158,#25159));
#5895=EDGE_LOOP('',(#25160,#25161,#25162,#25163,#25164,#25165));
#5896=EDGE_LOOP('',(#25166,#25167,#25168,#25169,#25170));
#5897=EDGE_LOOP('',(#25171,#25172,#25173,#25174));
#5898=EDGE_LOOP('',(#25175,#25176,#25177,#25178));
#5899=EDGE_LOOP('',(#25179,#25180,#25181));
#5900=EDGE_LOOP('',(#25182,#25183,#25184));
#5901=EDGE_LOOP('',(#25185,#25186,#25187));
#5902=EDGE_LOOP('',(#25188,#25189,#25190,#25191));
#5903=EDGE_LOOP('',(#25192,#25193,#25194));
#5904=EDGE_LOOP('',(#25195,#25196,#25197,#25198));
#5905=EDGE_LOOP('',(#25199,#25200,#25201,#25202));
#5906=EDGE_LOOP('',(#25203,#25204,#25205,#25206));
#5907=EDGE_LOOP('',(#25207,#25208,#25209,#25210));
#5908=EDGE_LOOP('',(#25211,#25212,#25213,#25214));
#5909=EDGE_LOOP('',(#25215,#25216,#25217,#25218));
#5910=EDGE_LOOP('',(#25219,#25220,#25221,#25222));
#5911=EDGE_LOOP('',(#25223,#25224,#25225,#25226));
#5912=EDGE_LOOP('',(#25227,#25228,#25229,#25230));
#5913=EDGE_LOOP('',(#25231,#25232,#25233,#25234));
#5914=EDGE_LOOP('',(#25235,#25236,#25237));
#5915=EDGE_LOOP('',(#25238,#25239,#25240));
#5916=EDGE_LOOP('',(#25241,#25242,#25243));
#5917=EDGE_LOOP('',(#25244,#25245,#25246,#25247));
#5918=EDGE_LOOP('',(#25248,#25249,#25250));
#5919=EDGE_LOOP('',(#25251,#25252,#25253,#25254));
#5920=EDGE_LOOP('',(#25255,#25256,#25257,#25258));
#5921=EDGE_LOOP('',(#25259,#25260,#25261,#25262));
#5922=EDGE_LOOP('',(#25263,#25264,#25265,#25266));
#5923=EDGE_LOOP('',(#25267,#25268,#25269,#25270));
#5924=EDGE_LOOP('',(#25271,#25272,#25273,#25274));
#5925=EDGE_LOOP('',(#25275,#25276,#25277,#25278));
#5926=EDGE_LOOP('',(#25279,#25280,#25281,#25282));
#5927=EDGE_LOOP('',(#25283,#25284,#25285,#25286));
#5928=EDGE_LOOP('',(#25287,#25288,#25289,#25290));
#5929=EDGE_LOOP('',(#25291,#25292,#25293,#25294,#25295));
#5930=EDGE_LOOP('',(#25296,#25297,#25298,#25299));
#5931=EDGE_LOOP('',(#25300,#25301,#25302,#25303,#25304));
#5932=EDGE_LOOP('',(#25305,#25306,#25307,#25308,#25309));
#5933=EDGE_LOOP('',(#25310,#25311,#25312));
#5934=EDGE_LOOP('',(#25313,#25314,#25315));
#5935=EDGE_LOOP('',(#25316,#25317,#25318,#25319));
#5936=EDGE_LOOP('',(#25320,#25321,#25322));
#5937=EDGE_LOOP('',(#25323,#25324,#25325,#25326));
#5938=EDGE_LOOP('',(#25327,#25328,#25329,#25330));
#5939=EDGE_LOOP('',(#25331,#25332,#25333,#25334));
#5940=EDGE_LOOP('',(#25335,#25336,#25337,#25338));
#5941=EDGE_LOOP('',(#25339,#25340,#25341,#25342));
#5942=EDGE_LOOP('',(#25343,#25344,#25345,#25346));
#5943=EDGE_LOOP('',(#25347,#25348,#25349));
#5944=EDGE_LOOP('',(#25350,#25351,#25352));
#5945=EDGE_LOOP('',(#25353,#25354,#25355));
#5946=EDGE_LOOP('',(#25356,#25357,#25358,#25359));
#5947=EDGE_LOOP('',(#25360,#25361,#25362));
#5948=EDGE_LOOP('',(#25363,#25364,#25365,#25366));
#5949=EDGE_LOOP('',(#25367,#25368,#25369,#25370));
#5950=EDGE_LOOP('',(#25371,#25372,#25373,#25374));
#5951=EDGE_LOOP('',(#25375,#25376,#25377,#25378));
#5952=EDGE_LOOP('',(#25379,#25380,#25381,#25382));
#5953=EDGE_LOOP('',(#25383,#25384,#25385,#25386));
#5954=EDGE_LOOP('',(#25387,#25388,#25389,#25390));
#5955=EDGE_LOOP('',(#25391,#25392,#25393,#25394));
#5956=EDGE_LOOP('',(#25395,#25396,#25397,#25398));
#5957=EDGE_LOOP('',(#25399,#25400,#25401,#25402));
#5958=EDGE_LOOP('',(#25403,#25404,#25405));
#5959=EDGE_LOOP('',(#25406,#25407,#25408,#25409,#25410));
#5960=EDGE_LOOP('',(#25411,#25412,#25413,#25414));
#5961=EDGE_LOOP('',(#25415,#25416,#25417));
#5962=EDGE_LOOP('',(#25418,#25419,#25420,#25421,#25422));
#5963=EDGE_LOOP('',(#25423,#25424,#25425,#25426));
#5964=EDGE_LOOP('',(#25427,#25428,#25429,#25430));
#5965=EDGE_LOOP('',(#25431,#25432,#25433,#25434,#25435));
#5966=EDGE_LOOP('',(#25436,#25437,#25438,#25439));
#5967=EDGE_LOOP('',(#25440,#25441,#25442,#25443,#25444,#25445));
#5968=EDGE_LOOP('',(#25446,#25447,#25448,#25449,#25450));
#5969=EDGE_LOOP('',(#25451,#25452,#25453,#25454));
#5970=EDGE_LOOP('',(#25455,#25456,#25457,#25458));
#5971=EDGE_LOOP('',(#25459,#25460,#25461));
#5972=EDGE_LOOP('',(#25462,#25463,#25464));
#5973=EDGE_LOOP('',(#25465,#25466,#25467));
#5974=EDGE_LOOP('',(#25468,#25469,#25470,#25471));
#5975=EDGE_LOOP('',(#25472,#25473,#25474));
#5976=EDGE_LOOP('',(#25475,#25476,#25477,#25478));
#5977=EDGE_LOOP('',(#25479,#25480,#25481,#25482));
#5978=EDGE_LOOP('',(#25483,#25484,#25485,#25486));
#5979=EDGE_LOOP('',(#25487,#25488,#25489,#25490));
#5980=EDGE_LOOP('',(#25491,#25492,#25493,#25494));
#5981=EDGE_LOOP('',(#25495,#25496,#25497,#25498));
#5982=EDGE_LOOP('',(#25499,#25500,#25501,#25502));
#5983=EDGE_LOOP('',(#25503,#25504,#25505,#25506));
#5984=EDGE_LOOP('',(#25507,#25508,#25509,#25510));
#5985=EDGE_LOOP('',(#25511,#25512,#25513,#25514));
#5986=EDGE_LOOP('',(#25515,#25516,#25517));
#5987=EDGE_LOOP('',(#25518,#25519,#25520));
#5988=EDGE_LOOP('',(#25521,#25522,#25523));
#5989=EDGE_LOOP('',(#25524,#25525,#25526,#25527));
#5990=EDGE_LOOP('',(#25528,#25529,#25530));
#5991=EDGE_LOOP('',(#25531,#25532,#25533,#25534));
#5992=EDGE_LOOP('',(#25535,#25536,#25537,#25538));
#5993=EDGE_LOOP('',(#25539,#25540,#25541,#25542));
#5994=EDGE_LOOP('',(#25543,#25544,#25545,#25546));
#5995=EDGE_LOOP('',(#25547,#25548,#25549,#25550));
#5996=EDGE_LOOP('',(#25551,#25552,#25553,#25554));
#5997=EDGE_LOOP('',(#25555,#25556,#25557,#25558));
#5998=EDGE_LOOP('',(#25559,#25560,#25561,#25562));
#5999=EDGE_LOOP('',(#25563,#25564,#25565,#25566));
#6000=EDGE_LOOP('',(#25567,#25568,#25569,#25570));
#6001=EDGE_LOOP('',(#25571,#25572,#25573,#25574,#25575));
#6002=EDGE_LOOP('',(#25576,#25577,#25578,#25579));
#6003=EDGE_LOOP('',(#25580,#25581,#25582,#25583,#25584));
#6004=EDGE_LOOP('',(#25585,#25586,#25587,#25588,#25589));
#6005=EDGE_LOOP('',(#25590,#25591,#25592));
#6006=EDGE_LOOP('',(#25593,#25594,#25595));
#6007=EDGE_LOOP('',(#25596,#25597,#25598,#25599));
#6008=EDGE_LOOP('',(#25600,#25601,#25602));
#6009=EDGE_LOOP('',(#25603,#25604,#25605,#25606));
#6010=EDGE_LOOP('',(#25607,#25608,#25609,#25610));
#6011=EDGE_LOOP('',(#25611,#25612,#25613,#25614));
#6012=EDGE_LOOP('',(#25615,#25616,#25617,#25618));
#6013=EDGE_LOOP('',(#25619,#25620,#25621,#25622));
#6014=EDGE_LOOP('',(#25623,#25624,#25625,#25626));
#6015=EDGE_LOOP('',(#25627,#25628,#25629));
#6016=EDGE_LOOP('',(#25630,#25631,#25632));
#6017=EDGE_LOOP('',(#25633,#25634,#25635));
#6018=EDGE_LOOP('',(#25636,#25637,#25638,#25639));
#6019=EDGE_LOOP('',(#25640,#25641,#25642));
#6020=EDGE_LOOP('',(#25643,#25644,#25645,#25646));
#6021=EDGE_LOOP('',(#25647,#25648,#25649,#25650));
#6022=EDGE_LOOP('',(#25651,#25652,#25653,#25654));
#6023=EDGE_LOOP('',(#25655,#25656,#25657,#25658));
#6024=EDGE_LOOP('',(#25659,#25660,#25661,#25662));
#6025=EDGE_LOOP('',(#25663,#25664,#25665,#25666));
#6026=EDGE_LOOP('',(#25667,#25668,#25669,#25670));
#6027=EDGE_LOOP('',(#25671,#25672,#25673,#25674));
#6028=EDGE_LOOP('',(#25675,#25676,#25677,#25678));
#6029=EDGE_LOOP('',(#25679,#25680,#25681,#25682));
#6030=EDGE_LOOP('',(#25683,#25684,#25685));
#6031=EDGE_LOOP('',(#25686,#25687,#25688,#25689,#25690));
#6032=EDGE_LOOP('',(#25691,#25692,#25693,#25694));
#6033=EDGE_LOOP('',(#25695,#25696,#25697));
#6034=EDGE_LOOP('',(#25698,#25699,#25700,#25701,#25702));
#6035=EDGE_LOOP('',(#25703,#25704,#25705,#25706));
#6036=EDGE_LOOP('',(#25707,#25708,#25709,#25710));
#6037=EDGE_LOOP('',(#25711,#25712,#25713,#25714,#25715));
#6038=EDGE_LOOP('',(#25716,#25717,#25718,#25719));
#6039=EDGE_LOOP('',(#25720,#25721,#25722,#25723,#25724,#25725));
#6040=EDGE_LOOP('',(#25726,#25727,#25728,#25729,#25730));
#6041=EDGE_LOOP('',(#25731,#25732,#25733,#25734));
#6042=EDGE_LOOP('',(#25735,#25736,#25737,#25738));
#6043=EDGE_LOOP('',(#25739,#25740,#25741));
#6044=EDGE_LOOP('',(#25742,#25743,#25744));
#6045=EDGE_LOOP('',(#25745,#25746,#25747));
#6046=EDGE_LOOP('',(#25748,#25749,#25750,#25751));
#6047=EDGE_LOOP('',(#25752,#25753,#25754));
#6048=EDGE_LOOP('',(#25755,#25756,#25757,#25758));
#6049=EDGE_LOOP('',(#25759,#25760,#25761,#25762));
#6050=EDGE_LOOP('',(#25763,#25764,#25765,#25766));
#6051=EDGE_LOOP('',(#25767,#25768,#25769,#25770));
#6052=EDGE_LOOP('',(#25771,#25772,#25773,#25774));
#6053=EDGE_LOOP('',(#25775,#25776,#25777,#25778));
#6054=EDGE_LOOP('',(#25779,#25780,#25781,#25782));
#6055=EDGE_LOOP('',(#25783,#25784,#25785,#25786));
#6056=EDGE_LOOP('',(#25787,#25788,#25789,#25790));
#6057=EDGE_LOOP('',(#25791,#25792,#25793,#25794));
#6058=EDGE_LOOP('',(#25795,#25796,#25797));
#6059=EDGE_LOOP('',(#25798,#25799,#25800));
#6060=EDGE_LOOP('',(#25801,#25802,#25803));
#6061=EDGE_LOOP('',(#25804,#25805,#25806,#25807));
#6062=EDGE_LOOP('',(#25808,#25809,#25810));
#6063=EDGE_LOOP('',(#25811,#25812,#25813,#25814));
#6064=EDGE_LOOP('',(#25815,#25816,#25817,#25818));
#6065=EDGE_LOOP('',(#25819,#25820,#25821,#25822));
#6066=EDGE_LOOP('',(#25823,#25824,#25825,#25826));
#6067=EDGE_LOOP('',(#25827,#25828,#25829,#25830));
#6068=EDGE_LOOP('',(#25831,#25832,#25833,#25834));
#6069=EDGE_LOOP('',(#25835,#25836,#25837,#25838));
#6070=EDGE_LOOP('',(#25839,#25840,#25841,#25842));
#6071=EDGE_LOOP('',(#25843,#25844,#25845,#25846));
#6072=EDGE_LOOP('',(#25847,#25848,#25849,#25850));
#6073=EDGE_LOOP('',(#25851,#25852,#25853,#25854,#25855));
#6074=EDGE_LOOP('',(#25856,#25857,#25858,#25859));
#6075=EDGE_LOOP('',(#25860,#25861,#25862,#25863,#25864));
#6076=EDGE_LOOP('',(#25865,#25866,#25867,#25868,#25869));
#6077=EDGE_LOOP('',(#25870,#25871,#25872));
#6078=EDGE_LOOP('',(#25873,#25874,#25875));
#6079=EDGE_LOOP('',(#25876,#25877,#25878,#25879));
#6080=EDGE_LOOP('',(#25880,#25881,#25882));
#6081=EDGE_LOOP('',(#25883,#25884,#25885,#25886));
#6082=EDGE_LOOP('',(#25887,#25888,#25889,#25890));
#6083=EDGE_LOOP('',(#25891,#25892,#25893,#25894));
#6084=EDGE_LOOP('',(#25895,#25896,#25897,#25898));
#6085=EDGE_LOOP('',(#25899,#25900,#25901,#25902));
#6086=EDGE_LOOP('',(#25903,#25904,#25905,#25906));
#6087=EDGE_LOOP('',(#25907,#25908,#25909));
#6088=EDGE_LOOP('',(#25910,#25911,#25912));
#6089=EDGE_LOOP('',(#25913,#25914,#25915));
#6090=EDGE_LOOP('',(#25916,#25917,#25918,#25919));
#6091=EDGE_LOOP('',(#25920,#25921,#25922));
#6092=EDGE_LOOP('',(#25923,#25924,#25925,#25926));
#6093=EDGE_LOOP('',(#25927,#25928,#25929,#25930));
#6094=EDGE_LOOP('',(#25931,#25932,#25933,#25934));
#6095=EDGE_LOOP('',(#25935,#25936,#25937,#25938));
#6096=EDGE_LOOP('',(#25939,#25940,#25941,#25942));
#6097=EDGE_LOOP('',(#25943,#25944,#25945,#25946));
#6098=EDGE_LOOP('',(#25947,#25948,#25949,#25950));
#6099=EDGE_LOOP('',(#25951,#25952,#25953,#25954));
#6100=EDGE_LOOP('',(#25955,#25956,#25957,#25958));
#6101=EDGE_LOOP('',(#25959,#25960,#25961,#25962));
#6102=EDGE_LOOP('',(#25963,#25964,#25965));
#6103=EDGE_LOOP('',(#25966,#25967,#25968,#25969,#25970));
#6104=EDGE_LOOP('',(#25971,#25972,#25973,#25974));
#6105=EDGE_LOOP('',(#25975,#25976,#25977));
#6106=EDGE_LOOP('',(#25978,#25979,#25980,#25981,#25982));
#6107=EDGE_LOOP('',(#25983,#25984,#25985,#25986));
#6108=EDGE_LOOP('',(#25987,#25988,#25989,#25990));
#6109=EDGE_LOOP('',(#25991,#25992,#25993,#25994,#25995));
#6110=EDGE_LOOP('',(#25996,#25997,#25998,#25999));
#6111=EDGE_LOOP('',(#26000,#26001,#26002,#26003,#26004,#26005));
#6112=EDGE_LOOP('',(#26006,#26007,#26008,#26009,#26010));
#6113=EDGE_LOOP('',(#26011,#26012,#26013,#26014));
#6114=EDGE_LOOP('',(#26015,#26016,#26017,#26018));
#6115=EDGE_LOOP('',(#26019,#26020,#26021));
#6116=EDGE_LOOP('',(#26022,#26023,#26024));
#6117=EDGE_LOOP('',(#26025,#26026,#26027));
#6118=EDGE_LOOP('',(#26028,#26029,#26030,#26031));
#6119=EDGE_LOOP('',(#26032,#26033,#26034));
#6120=EDGE_LOOP('',(#26035,#26036,#26037,#26038));
#6121=EDGE_LOOP('',(#26039,#26040,#26041,#26042));
#6122=EDGE_LOOP('',(#26043,#26044,#26045,#26046));
#6123=EDGE_LOOP('',(#26047,#26048,#26049,#26050));
#6124=EDGE_LOOP('',(#26051,#26052,#26053,#26054));
#6125=EDGE_LOOP('',(#26055,#26056,#26057,#26058));
#6126=EDGE_LOOP('',(#26059,#26060,#26061,#26062));
#6127=EDGE_LOOP('',(#26063,#26064,#26065,#26066));
#6128=EDGE_LOOP('',(#26067,#26068,#26069,#26070));
#6129=EDGE_LOOP('',(#26071,#26072,#26073,#26074));
#6130=EDGE_LOOP('',(#26075,#26076,#26077));
#6131=EDGE_LOOP('',(#26078,#26079,#26080));
#6132=EDGE_LOOP('',(#26081,#26082,#26083));
#6133=EDGE_LOOP('',(#26084,#26085,#26086,#26087));
#6134=EDGE_LOOP('',(#26088,#26089,#26090));
#6135=EDGE_LOOP('',(#26091,#26092,#26093,#26094));
#6136=EDGE_LOOP('',(#26095,#26096,#26097,#26098));
#6137=EDGE_LOOP('',(#26099,#26100,#26101,#26102));
#6138=EDGE_LOOP('',(#26103,#26104,#26105,#26106));
#6139=EDGE_LOOP('',(#26107,#26108,#26109,#26110));
#6140=EDGE_LOOP('',(#26111,#26112,#26113,#26114));
#6141=EDGE_LOOP('',(#26115,#26116,#26117,#26118));
#6142=EDGE_LOOP('',(#26119,#26120,#26121,#26122));
#6143=EDGE_LOOP('',(#26123,#26124,#26125,#26126));
#6144=EDGE_LOOP('',(#26127,#26128,#26129,#26130));
#6145=EDGE_LOOP('',(#26131,#26132,#26133,#26134,#26135));
#6146=EDGE_LOOP('',(#26136,#26137,#26138,#26139));
#6147=EDGE_LOOP('',(#26140,#26141,#26142,#26143,#26144));
#6148=EDGE_LOOP('',(#26145,#26146,#26147,#26148,#26149));
#6149=EDGE_LOOP('',(#26150,#26151,#26152));
#6150=EDGE_LOOP('',(#26153,#26154,#26155));
#6151=EDGE_LOOP('',(#26156,#26157,#26158,#26159));
#6152=EDGE_LOOP('',(#26160,#26161,#26162));
#6153=EDGE_LOOP('',(#26163,#26164,#26165,#26166));
#6154=EDGE_LOOP('',(#26167,#26168,#26169,#26170));
#6155=EDGE_LOOP('',(#26171,#26172,#26173,#26174));
#6156=EDGE_LOOP('',(#26175,#26176,#26177,#26178));
#6157=EDGE_LOOP('',(#26179,#26180,#26181,#26182));
#6158=EDGE_LOOP('',(#26183,#26184,#26185,#26186));
#6159=EDGE_LOOP('',(#26187,#26188,#26189));
#6160=EDGE_LOOP('',(#26190,#26191,#26192));
#6161=EDGE_LOOP('',(#26193,#26194,#26195));
#6162=EDGE_LOOP('',(#26196,#26197,#26198,#26199));
#6163=EDGE_LOOP('',(#26200,#26201,#26202));
#6164=EDGE_LOOP('',(#26203,#26204,#26205,#26206));
#6165=EDGE_LOOP('',(#26207,#26208,#26209,#26210));
#6166=EDGE_LOOP('',(#26211,#26212,#26213,#26214));
#6167=EDGE_LOOP('',(#26215,#26216,#26217,#26218));
#6168=EDGE_LOOP('',(#26219,#26220,#26221,#26222));
#6169=EDGE_LOOP('',(#26223,#26224,#26225,#26226));
#6170=EDGE_LOOP('',(#26227,#26228,#26229,#26230));
#6171=EDGE_LOOP('',(#26231,#26232,#26233,#26234));
#6172=EDGE_LOOP('',(#26235,#26236,#26237,#26238));
#6173=EDGE_LOOP('',(#26239,#26240,#26241,#26242));
#6174=EDGE_LOOP('',(#26243,#26244,#26245));
#6175=EDGE_LOOP('',(#26246,#26247,#26248,#26249,#26250));
#6176=EDGE_LOOP('',(#26251,#26252,#26253,#26254));
#6177=EDGE_LOOP('',(#26255,#26256,#26257));
#6178=EDGE_LOOP('',(#26258,#26259,#26260,#26261,#26262));
#6179=EDGE_LOOP('',(#26263,#26264,#26265,#26266));
#6180=EDGE_LOOP('',(#26267,#26268,#26269,#26270));
#6181=EDGE_LOOP('',(#26271,#26272,#26273,#26274,#26275));
#6182=EDGE_LOOP('',(#26276,#26277,#26278,#26279));
#6183=EDGE_LOOP('',(#26280,#26281,#26282,#26283,#26284,#26285));
#6184=EDGE_LOOP('',(#26286,#26287,#26288,#26289,#26290));
#6185=EDGE_LOOP('',(#26291,#26292,#26293,#26294));
#6186=EDGE_LOOP('',(#26295,#26296,#26297,#26298));
#6187=EDGE_LOOP('',(#26299,#26300,#26301));
#6188=EDGE_LOOP('',(#26302,#26303,#26304));
#6189=EDGE_LOOP('',(#26305,#26306,#26307));
#6190=EDGE_LOOP('',(#26308,#26309,#26310,#26311));
#6191=EDGE_LOOP('',(#26312,#26313,#26314));
#6192=EDGE_LOOP('',(#26315,#26316,#26317,#26318));
#6193=EDGE_LOOP('',(#26319,#26320,#26321,#26322));
#6194=EDGE_LOOP('',(#26323,#26324,#26325,#26326));
#6195=EDGE_LOOP('',(#26327,#26328,#26329,#26330));
#6196=EDGE_LOOP('',(#26331,#26332,#26333,#26334));
#6197=EDGE_LOOP('',(#26335,#26336,#26337,#26338));
#6198=EDGE_LOOP('',(#26339,#26340,#26341,#26342));
#6199=EDGE_LOOP('',(#26343,#26344,#26345,#26346));
#6200=EDGE_LOOP('',(#26347,#26348,#26349,#26350));
#6201=EDGE_LOOP('',(#26351,#26352,#26353,#26354));
#6202=EDGE_LOOP('',(#26355,#26356,#26357));
#6203=EDGE_LOOP('',(#26358,#26359,#26360));
#6204=EDGE_LOOP('',(#26361,#26362,#26363));
#6205=EDGE_LOOP('',(#26364,#26365,#26366,#26367));
#6206=EDGE_LOOP('',(#26368,#26369,#26370));
#6207=EDGE_LOOP('',(#26371,#26372,#26373,#26374));
#6208=EDGE_LOOP('',(#26375,#26376,#26377,#26378));
#6209=EDGE_LOOP('',(#26379,#26380,#26381,#26382));
#6210=EDGE_LOOP('',(#26383,#26384,#26385,#26386));
#6211=EDGE_LOOP('',(#26387,#26388,#26389,#26390));
#6212=EDGE_LOOP('',(#26391,#26392,#26393,#26394));
#6213=EDGE_LOOP('',(#26395,#26396,#26397,#26398));
#6214=EDGE_LOOP('',(#26399,#26400,#26401,#26402));
#6215=EDGE_LOOP('',(#26403,#26404,#26405,#26406));
#6216=EDGE_LOOP('',(#26407,#26408,#26409,#26410));
#6217=EDGE_LOOP('',(#26411,#26412,#26413,#26414,#26415));
#6218=EDGE_LOOP('',(#26416,#26417,#26418,#26419));
#6219=EDGE_LOOP('',(#26420,#26421,#26422,#26423,#26424));
#6220=EDGE_LOOP('',(#26425,#26426,#26427,#26428,#26429));
#6221=EDGE_LOOP('',(#26430,#26431,#26432));
#6222=EDGE_LOOP('',(#26433,#26434,#26435));
#6223=EDGE_LOOP('',(#26436,#26437,#26438,#26439));
#6224=EDGE_LOOP('',(#26440,#26441,#26442));
#6225=EDGE_LOOP('',(#26443,#26444,#26445,#26446));
#6226=EDGE_LOOP('',(#26447,#26448,#26449,#26450));
#6227=EDGE_LOOP('',(#26451,#26452,#26453,#26454));
#6228=EDGE_LOOP('',(#26455,#26456,#26457,#26458));
#6229=EDGE_LOOP('',(#26459,#26460,#26461,#26462));
#6230=EDGE_LOOP('',(#26463,#26464,#26465,#26466));
#6231=EDGE_LOOP('',(#26467,#26468,#26469));
#6232=EDGE_LOOP('',(#26470,#26471,#26472));
#6233=EDGE_LOOP('',(#26473,#26474,#26475));
#6234=EDGE_LOOP('',(#26476,#26477,#26478,#26479));
#6235=EDGE_LOOP('',(#26480,#26481,#26482));
#6236=EDGE_LOOP('',(#26483,#26484,#26485,#26486));
#6237=EDGE_LOOP('',(#26487,#26488,#26489,#26490));
#6238=EDGE_LOOP('',(#26491,#26492,#26493,#26494));
#6239=EDGE_LOOP('',(#26495,#26496,#26497,#26498));
#6240=EDGE_LOOP('',(#26499,#26500,#26501,#26502));
#6241=EDGE_LOOP('',(#26503,#26504,#26505,#26506));
#6242=EDGE_LOOP('',(#26507,#26508,#26509,#26510));
#6243=EDGE_LOOP('',(#26511,#26512,#26513,#26514));
#6244=EDGE_LOOP('',(#26515,#26516,#26517,#26518));
#6245=EDGE_LOOP('',(#26519,#26520,#26521,#26522));
#6246=EDGE_LOOP('',(#26523,#26524,#26525));
#6247=EDGE_LOOP('',(#26526,#26527,#26528,#26529,#26530));
#6248=EDGE_LOOP('',(#26531,#26532,#26533,#26534));
#6249=EDGE_LOOP('',(#26535,#26536,#26537));
#6250=EDGE_LOOP('',(#26538,#26539,#26540,#26541,#26542));
#6251=EDGE_LOOP('',(#26543,#26544,#26545,#26546));
#6252=EDGE_LOOP('',(#26547,#26548,#26549,#26550));
#6253=EDGE_LOOP('',(#26551,#26552,#26553,#26554,#26555));
#6254=EDGE_LOOP('',(#26556,#26557,#26558,#26559));
#6255=EDGE_LOOP('',(#26560,#26561,#26562,#26563,#26564,#26565));
#6256=EDGE_LOOP('',(#26566,#26567,#26568,#26569,#26570));
#6257=EDGE_LOOP('',(#26571,#26572,#26573,#26574));
#6258=EDGE_LOOP('',(#26575,#26576,#26577,#26578));
#6259=EDGE_LOOP('',(#26579,#26580,#26581));
#6260=EDGE_LOOP('',(#26582,#26583,#26584));
#6261=EDGE_LOOP('',(#26585,#26586,#26587));
#6262=EDGE_LOOP('',(#26588,#26589,#26590,#26591));
#6263=EDGE_LOOP('',(#26592,#26593,#26594));
#6264=EDGE_LOOP('',(#26595,#26596,#26597,#26598));
#6265=EDGE_LOOP('',(#26599,#26600,#26601,#26602));
#6266=EDGE_LOOP('',(#26603,#26604,#26605,#26606));
#6267=EDGE_LOOP('',(#26607,#26608,#26609,#26610));
#6268=EDGE_LOOP('',(#26611,#26612,#26613,#26614));
#6269=EDGE_LOOP('',(#26615,#26616,#26617,#26618));
#6270=EDGE_LOOP('',(#26619,#26620,#26621,#26622));
#6271=EDGE_LOOP('',(#26623,#26624,#26625,#26626));
#6272=EDGE_LOOP('',(#26627,#26628,#26629,#26630));
#6273=EDGE_LOOP('',(#26631,#26632,#26633,#26634));
#6274=EDGE_LOOP('',(#26635,#26636,#26637));
#6275=EDGE_LOOP('',(#26638,#26639,#26640));
#6276=EDGE_LOOP('',(#26641,#26642,#26643));
#6277=EDGE_LOOP('',(#26644,#26645,#26646,#26647));
#6278=EDGE_LOOP('',(#26648,#26649,#26650));
#6279=EDGE_LOOP('',(#26651,#26652,#26653,#26654));
#6280=EDGE_LOOP('',(#26655,#26656,#26657,#26658));
#6281=EDGE_LOOP('',(#26659,#26660,#26661,#26662));
#6282=EDGE_LOOP('',(#26663,#26664,#26665,#26666));
#6283=EDGE_LOOP('',(#26667,#26668,#26669,#26670));
#6284=EDGE_LOOP('',(#26671,#26672,#26673,#26674));
#6285=EDGE_LOOP('',(#26675,#26676,#26677,#26678));
#6286=EDGE_LOOP('',(#26679,#26680,#26681,#26682));
#6287=EDGE_LOOP('',(#26683,#26684,#26685,#26686));
#6288=EDGE_LOOP('',(#26687,#26688,#26689,#26690));
#6289=EDGE_LOOP('',(#26691,#26692,#26693,#26694,#26695));
#6290=EDGE_LOOP('',(#26696,#26697,#26698,#26699));
#6291=EDGE_LOOP('',(#26700,#26701,#26702,#26703,#26704));
#6292=EDGE_LOOP('',(#26705,#26706,#26707,#26708,#26709));
#6293=EDGE_LOOP('',(#26710,#26711,#26712));
#6294=EDGE_LOOP('',(#26713,#26714,#26715));
#6295=EDGE_LOOP('',(#26716,#26717,#26718,#26719));
#6296=EDGE_LOOP('',(#26720,#26721,#26722));
#6297=EDGE_LOOP('',(#26723,#26724,#26725,#26726));
#6298=EDGE_LOOP('',(#26727,#26728,#26729,#26730));
#6299=EDGE_LOOP('',(#26731,#26732,#26733,#26734));
#6300=EDGE_LOOP('',(#26735,#26736,#26737,#26738));
#6301=EDGE_LOOP('',(#26739,#26740,#26741,#26742));
#6302=EDGE_LOOP('',(#26743,#26744,#26745,#26746));
#6303=EDGE_LOOP('',(#26747,#26748,#26749));
#6304=EDGE_LOOP('',(#26750,#26751,#26752));
#6305=EDGE_LOOP('',(#26753,#26754,#26755));
#6306=EDGE_LOOP('',(#26756,#26757,#26758,#26759));
#6307=EDGE_LOOP('',(#26760,#26761,#26762));
#6308=EDGE_LOOP('',(#26763,#26764,#26765,#26766));
#6309=EDGE_LOOP('',(#26767,#26768,#26769,#26770));
#6310=EDGE_LOOP('',(#26771,#26772,#26773,#26774));
#6311=EDGE_LOOP('',(#26775,#26776,#26777,#26778));
#6312=EDGE_LOOP('',(#26779,#26780,#26781,#26782));
#6313=EDGE_LOOP('',(#26783,#26784,#26785,#26786));
#6314=EDGE_LOOP('',(#26787,#26788,#26789,#26790));
#6315=EDGE_LOOP('',(#26791,#26792,#26793,#26794));
#6316=EDGE_LOOP('',(#26795,#26796,#26797,#26798));
#6317=EDGE_LOOP('',(#26799,#26800,#26801,#26802));
#6318=EDGE_LOOP('',(#26803,#26804,#26805));
#6319=EDGE_LOOP('',(#26806,#26807,#26808,#26809,#26810));
#6320=EDGE_LOOP('',(#26811,#26812,#26813,#26814));
#6321=EDGE_LOOP('',(#26815,#26816,#26817));
#6322=EDGE_LOOP('',(#26818,#26819,#26820,#26821,#26822));
#6323=EDGE_LOOP('',(#26823,#26824,#26825,#26826));
#6324=EDGE_LOOP('',(#26827,#26828,#26829,#26830));
#6325=EDGE_LOOP('',(#26831,#26832,#26833,#26834,#26835));
#6326=EDGE_LOOP('',(#26836,#26837,#26838,#26839));
#6327=EDGE_LOOP('',(#26840,#26841,#26842,#26843,#26844,#26845));
#6328=EDGE_LOOP('',(#26846,#26847,#26848,#26849,#26850));
#6329=EDGE_LOOP('',(#26851,#26852,#26853,#26854));
#6330=EDGE_LOOP('',(#26855,#26856,#26857,#26858));
#6331=EDGE_LOOP('',(#26859,#26860,#26861));
#6332=EDGE_LOOP('',(#26862,#26863,#26864));
#6333=EDGE_LOOP('',(#26865,#26866,#26867));
#6334=EDGE_LOOP('',(#26868,#26869,#26870,#26871));
#6335=EDGE_LOOP('',(#26872,#26873,#26874));
#6336=EDGE_LOOP('',(#26875,#26876,#26877,#26878));
#6337=EDGE_LOOP('',(#26879,#26880,#26881,#26882));
#6338=EDGE_LOOP('',(#26883,#26884,#26885,#26886));
#6339=EDGE_LOOP('',(#26887,#26888,#26889,#26890));
#6340=EDGE_LOOP('',(#26891,#26892,#26893,#26894));
#6341=EDGE_LOOP('',(#26895,#26896,#26897,#26898));
#6342=EDGE_LOOP('',(#26899,#26900,#26901,#26902));
#6343=EDGE_LOOP('',(#26903,#26904,#26905,#26906));
#6344=EDGE_LOOP('',(#26907,#26908,#26909,#26910));
#6345=EDGE_LOOP('',(#26911,#26912,#26913,#26914));
#6346=EDGE_LOOP('',(#26915,#26916,#26917));
#6347=EDGE_LOOP('',(#26918,#26919,#26920));
#6348=EDGE_LOOP('',(#26921,#26922,#26923));
#6349=EDGE_LOOP('',(#26924,#26925,#26926,#26927));
#6350=EDGE_LOOP('',(#26928,#26929,#26930));
#6351=EDGE_LOOP('',(#26931,#26932,#26933,#26934));
#6352=EDGE_LOOP('',(#26935,#26936,#26937,#26938));
#6353=EDGE_LOOP('',(#26939,#26940,#26941,#26942));
#6354=EDGE_LOOP('',(#26943,#26944,#26945,#26946));
#6355=EDGE_LOOP('',(#26947,#26948,#26949,#26950));
#6356=EDGE_LOOP('',(#26951,#26952,#26953,#26954));
#6357=EDGE_LOOP('',(#26955,#26956,#26957,#26958));
#6358=EDGE_LOOP('',(#26959,#26960,#26961,#26962));
#6359=EDGE_LOOP('',(#26963,#26964,#26965,#26966));
#6360=EDGE_LOOP('',(#26967,#26968,#26969,#26970));
#6361=EDGE_LOOP('',(#26971,#26972,#26973,#26974,#26975,#26976));
#6362=EDGE_LOOP('',(#26977,#26978,#26979,#26980,#26981,#26982));
#6363=EDGE_LOOP('',(#26983,#26984,#26985,#26986,#26987));
#6364=EDGE_LOOP('',(#26988,#26989,#26990));
#6365=EDGE_LOOP('',(#26991,#26992,#26993));
#6366=EDGE_LOOP('',(#26994,#26995,#26996));
#6367=EDGE_LOOP('',(#26997,#26998,#26999,#27000));
#6368=EDGE_LOOP('',(#27001,#27002,#27003));
#6369=EDGE_LOOP('',(#27004,#27005,#27006,#27007));
#6370=EDGE_LOOP('',(#27008,#27009,#27010,#27011));
#6371=EDGE_LOOP('',(#27012,#27013,#27014,#27015));
#6372=EDGE_LOOP('',(#27016,#27017,#27018,#27019));
#6373=EDGE_LOOP('',(#27020,#27021,#27022,#27023));
#6374=EDGE_LOOP('',(#27024,#27025,#27026,#27027));
#6375=EDGE_LOOP('',(#27028,#27029,#27030,#27031));
#6376=EDGE_LOOP('',(#27032,#27033,#27034,#27035));
#6377=EDGE_LOOP('',(#27036,#27037,#27038,#27039));
#6378=EDGE_LOOP('',(#27040,#27041,#27042,#27043));
#6379=EDGE_LOOP('',(#27044,#27045,#27046));
#6380=EDGE_LOOP('',(#27047,#27048,#27049));
#6381=EDGE_LOOP('',(#27050,#27051,#27052));
#6382=EDGE_LOOP('',(#27053,#27054,#27055,#27056));
#6383=EDGE_LOOP('',(#27057,#27058,#27059));
#6384=EDGE_LOOP('',(#27060,#27061,#27062,#27063));
#6385=EDGE_LOOP('',(#27064,#27065,#27066,#27067));
#6386=EDGE_LOOP('',(#27068,#27069,#27070,#27071));
#6387=EDGE_LOOP('',(#27072,#27073,#27074,#27075));
#6388=EDGE_LOOP('',(#27076,#27077,#27078,#27079));
#6389=EDGE_LOOP('',(#27080,#27081,#27082,#27083));
#6390=EDGE_LOOP('',(#27084,#27085,#27086,#27087));
#6391=EDGE_LOOP('',(#27088,#27089,#27090,#27091));
#6392=EDGE_LOOP('',(#27092,#27093,#27094,#27095));
#6393=EDGE_LOOP('',(#27096,#27097,#27098,#27099));
#6394=EDGE_LOOP('',(#27100,#27101,#27102,#27103,#27104,#27105));
#6395=EDGE_LOOP('',(#27106,#27107,#27108,#27109,#27110,#27111));
#6396=EDGE_LOOP('',(#27112,#27113,#27114,#27115,#27116));
#6397=EDGE_LOOP('',(#27117,#27118,#27119,#27120,#27121));
#6398=EDGE_LOOP('',(#27122));
#6399=EDGE_LOOP('',(#27123));
#6400=EDGE_LOOP('',(#27124,#27125,#27126,#27127,#27128));
#6401=EDGE_LOOP('',(#27129,#27130,#27131,#27132));
#6402=EDGE_LOOP('',(#27133,#27134,#27135,#27136));
#6403=EDGE_LOOP('',(#27137,#27138,#27139,#27140));
#6404=EDGE_LOOP('',(#27141,#27142,#27143,#27144));
#6405=EDGE_LOOP('',(#27145,#27146,#27147,#27148));
#6406=EDGE_LOOP('',(#27149,#27150,#27151,#27152));
#6407=EDGE_LOOP('',(#27153,#27154,#27155,#27156));
#6408=EDGE_LOOP('',(#27157,#27158,#27159,#27160));
#6409=EDGE_LOOP('',(#27161,#27162,#27163,#27164));
#6410=EDGE_LOOP('',(#27165,#27166,#27167,#27168));
#6411=EDGE_LOOP('',(#27169,#27170,#27171,#27172));
#6412=EDGE_LOOP('',(#27173,#27174,#27175,#27176));
#6413=EDGE_LOOP('',(#27177,#27178,#27179,#27180));
#6414=EDGE_LOOP('',(#27181,#27182,#27183,#27184));
#6415=EDGE_LOOP('',(#27185,#27186,#27187,#27188));
#6416=EDGE_LOOP('',(#27189,#27190,#27191,#27192));
#6417=EDGE_LOOP('',(#27193,#27194,#27195,#27196));
#6418=EDGE_LOOP('',(#27197,#27198,#27199,#27200));
#6419=EDGE_LOOP('',(#27201,#27202,#27203,#27204));
#6420=EDGE_LOOP('',(#27205,#27206,#27207,#27208));
#6421=EDGE_LOOP('',(#27209,#27210,#27211,#27212));
#6422=EDGE_LOOP('',(#27213,#27214,#27215,#27216));
#6423=EDGE_LOOP('',(#27217,#27218,#27219,#27220));
#6424=EDGE_LOOP('',(#27221,#27222,#27223,#27224));
#6425=EDGE_LOOP('',(#27225,#27226,#27227,#27228));
#6426=EDGE_LOOP('',(#27229,#27230,#27231,#27232));
#6427=EDGE_LOOP('',(#27233,#27234,#27235,#27236));
#6428=EDGE_LOOP('',(#27237,#27238,#27239,#27240));
#6429=EDGE_LOOP('',(#27241,#27242,#27243,#27244));
#6430=EDGE_LOOP('',(#27245,#27246,#27247,#27248));
#6431=EDGE_LOOP('',(#27249,#27250,#27251,#27252));
#6432=EDGE_LOOP('',(#27253,#27254,#27255,#27256));
#6433=EDGE_LOOP('',(#27257,#27258,#27259,#27260));
#6434=EDGE_LOOP('',(#27261,#27262,#27263,#27264));
#6435=EDGE_LOOP('',(#27265,#27266,#27267,#27268));
#6436=EDGE_LOOP('',(#27269,#27270,#27271,#27272));
#6437=EDGE_LOOP('',(#27273,#27274,#27275,#27276));
#6438=EDGE_LOOP('',(#27277,#27278,#27279,#27280));
#6439=EDGE_LOOP('',(#27281,#27282,#27283,#27284));
#6440=EDGE_LOOP('',(#27285,#27286,#27287,#27288));
#6441=EDGE_LOOP('',(#27289,#27290,#27291,#27292));
#6442=EDGE_LOOP('',(#27293,#27294,#27295,#27296));
#6443=EDGE_LOOP('',(#27297,#27298,#27299,#27300));
#6444=EDGE_LOOP('',(#27301,#27302,#27303,#27304));
#6445=EDGE_LOOP('',(#27305,#27306,#27307,#27308));
#6446=EDGE_LOOP('',(#27309,#27310,#27311,#27312));
#6447=EDGE_LOOP('',(#27313,#27314,#27315,#27316));
#6448=EDGE_LOOP('',(#27317,#27318,#27319,#27320));
#6449=EDGE_LOOP('',(#27321,#27322,#27323,#27324));
#6450=EDGE_LOOP('',(#27325,#27326,#27327,#27328));
#6451=EDGE_LOOP('',(#27329,#27330,#27331,#27332));
#6452=EDGE_LOOP('',(#27333,#27334,#27335,#27336));
#6453=EDGE_LOOP('',(#27337,#27338,#27339,#27340));
#6454=EDGE_LOOP('',(#27341,#27342,#27343,#27344));
#6455=EDGE_LOOP('',(#27345,#27346,#27347,#27348));
#6456=EDGE_LOOP('',(#27349,#27350,#27351,#27352));
#6457=EDGE_LOOP('',(#27353,#27354,#27355,#27356));
#6458=EDGE_LOOP('',(#27357,#27358,#27359,#27360));
#6459=EDGE_LOOP('',(#27361,#27362,#27363,#27364));
#6460=EDGE_LOOP('',(#27365,#27366,#27367,#27368));
#6461=EDGE_LOOP('',(#27369,#27370,#27371,#27372));
#6462=EDGE_LOOP('',(#27373,#27374,#27375,#27376));
#6463=EDGE_LOOP('',(#27377,#27378,#27379,#27380));
#6464=EDGE_LOOP('',(#27381,#27382,#27383,#27384));
#6465=EDGE_LOOP('',(#27385,#27386,#27387,#27388));
#6466=EDGE_LOOP('',(#27389,#27390,#27391,#27392));
#6467=EDGE_LOOP('',(#27393,#27394,#27395,#27396));
#6468=EDGE_LOOP('',(#27397,#27398,#27399,#27400));
#6469=EDGE_LOOP('',(#27401,#27402,#27403,#27404));
#6470=EDGE_LOOP('',(#27405,#27406,#27407,#27408));
#6471=EDGE_LOOP('',(#27409,#27410,#27411,#27412));
#6472=EDGE_LOOP('',(#27413,#27414,#27415,#27416));
#6473=EDGE_LOOP('',(#27417,#27418,#27419,#27420));
#6474=EDGE_LOOP('',(#27421,#27422,#27423,#27424));
#6475=EDGE_LOOP('',(#27425,#27426,#27427,#27428));
#6476=EDGE_LOOP('',(#27429,#27430,#27431,#27432));
#6477=EDGE_LOOP('',(#27433,#27434,#27435,#27436));
#6478=EDGE_LOOP('',(#27437,#27438,#27439,#27440));
#6479=EDGE_LOOP('',(#27441,#27442,#27443,#27444));
#6480=EDGE_LOOP('',(#27445,#27446,#27447,#27448));
#6481=EDGE_LOOP('',(#27449,#27450,#27451,#27452));
#6482=EDGE_LOOP('',(#27453,#27454,#27455,#27456));
#6483=EDGE_LOOP('',(#27457,#27458,#27459,#27460));
#6484=EDGE_LOOP('',(#27461,#27462,#27463,#27464));
#6485=EDGE_LOOP('',(#27465,#27466,#27467,#27468));
#6486=EDGE_LOOP('',(#27469,#27470,#27471,#27472));
#6487=EDGE_LOOP('',(#27473,#27474,#27475,#27476));
#6488=EDGE_LOOP('',(#27477,#27478,#27479,#27480));
#6489=EDGE_LOOP('',(#27481,#27482,#27483,#27484));
#6490=EDGE_LOOP('',(#27485,#27486,#27487,#27488));
#6491=EDGE_LOOP('',(#27489,#27490,#27491,#27492));
#6492=EDGE_LOOP('',(#27493,#27494,#27495,#27496));
#6493=EDGE_LOOP('',(#27497,#27498,#27499,#27500));
#6494=EDGE_LOOP('',(#27501,#27502,#27503,#27504));
#6495=EDGE_LOOP('',(#27505,#27506,#27507,#27508));
#6496=EDGE_LOOP('',(#27509,#27510,#27511,#27512));
#6497=EDGE_LOOP('',(#27513,#27514,#27515,#27516));
#6498=EDGE_LOOP('',(#27517,#27518,#27519,#27520));
#6499=EDGE_LOOP('',(#27521,#27522,#27523,#27524));
#6500=EDGE_LOOP('',(#27525,#27526,#27527,#27528));
#6501=EDGE_LOOP('',(#27529,#27530,#27531,#27532));
#6502=EDGE_LOOP('',(#27533,#27534,#27535,#27536));
#6503=EDGE_LOOP('',(#27537,#27538,#27539,#27540));
#6504=EDGE_LOOP('',(#27541,#27542,#27543,#27544));
#6505=EDGE_LOOP('',(#27545,#27546,#27547,#27548));
#6506=EDGE_LOOP('',(#27549,#27550,#27551,#27552));
#6507=EDGE_LOOP('',(#27553,#27554,#27555,#27556));
#6508=EDGE_LOOP('',(#27557,#27558,#27559,#27560));
#6509=EDGE_LOOP('',(#27561,#27562,#27563,#27564));
#6510=EDGE_LOOP('',(#27565,#27566,#27567,#27568,#27569));
#6511=EDGE_LOOP('',(#27570,#27571,#27572,#27573));
#6512=EDGE_LOOP('',(#27574,#27575,#27576,#27577));
#6513=EDGE_LOOP('',(#27578,#27579,#27580,#27581));
#6514=EDGE_LOOP('',(#27582,#27583,#27584,#27585));
#6515=EDGE_LOOP('',(#27586,#27587,#27588,#27589));
#6516=EDGE_LOOP('',(#27590,#27591,#27592,#27593));
#6517=EDGE_LOOP('',(#27594,#27595,#27596,#27597));
#6518=EDGE_LOOP('',(#27598,#27599,#27600,#27601));
#6519=EDGE_LOOP('',(#27602,#27603,#27604,#27605));
#6520=EDGE_LOOP('',(#27606,#27607,#27608,#27609));
#6521=EDGE_LOOP('',(#27610,#27611,#27612,#27613));
#6522=EDGE_LOOP('',(#27614,#27615,#27616,#27617));
#6523=EDGE_LOOP('',(#27618,#27619,#27620,#27621));
#6524=EDGE_LOOP('',(#27622,#27623,#27624,#27625));
#6525=EDGE_LOOP('',(#27626,#27627,#27628,#27629));
#6526=EDGE_LOOP('',(#27630,#27631,#27632,#27633));
#6527=EDGE_LOOP('',(#27634,#27635,#27636,#27637));
#6528=EDGE_LOOP('',(#27638,#27639,#27640,#27641));
#6529=EDGE_LOOP('',(#27642,#27643,#27644,#27645));
#6530=EDGE_LOOP('',(#27646,#27647,#27648,#27649));
#6531=EDGE_LOOP('',(#27650,#27651,#27652,#27653));
#6532=EDGE_LOOP('',(#27654,#27655,#27656,#27657));
#6533=EDGE_LOOP('',(#27658,#27659,#27660,#27661));
#6534=EDGE_LOOP('',(#27662,#27663,#27664,#27665));
#6535=EDGE_LOOP('',(#27666,#27667,#27668,#27669));
#6536=EDGE_LOOP('',(#27670,#27671,#27672,#27673));
#6537=EDGE_LOOP('',(#27674,#27675,#27676,#27677));
#6538=EDGE_LOOP('',(#27678,#27679,#27680,#27681));
#6539=EDGE_LOOP('',(#27682,#27683,#27684,#27685));
#6540=EDGE_LOOP('',(#27686,#27687,#27688,#27689));
#6541=EDGE_LOOP('',(#27690,#27691,#27692,#27693));
#6542=EDGE_LOOP('',(#27694,#27695,#27696,#27697));
#6543=EDGE_LOOP('',(#27698,#27699,#27700,#27701));
#6544=EDGE_LOOP('',(#27702,#27703,#27704,#27705));
#6545=EDGE_LOOP('',(#27706,#27707,#27708,#27709));
#6546=EDGE_LOOP('',(#27710,#27711,#27712,#27713));
#6547=EDGE_LOOP('',(#27714,#27715,#27716,#27717));
#6548=EDGE_LOOP('',(#27718,#27719,#27720,#27721));
#6549=EDGE_LOOP('',(#27722,#27723,#27724,#27725));
#6550=EDGE_LOOP('',(#27726,#27727,#27728,#27729));
#6551=EDGE_LOOP('',(#27730,#27731,#27732,#27733));
#6552=EDGE_LOOP('',(#27734,#27735,#27736,#27737));
#6553=EDGE_LOOP('',(#27738,#27739,#27740,#27741));
#6554=EDGE_LOOP('',(#27742,#27743,#27744,#27745));
#6555=EDGE_LOOP('',(#27746,#27747,#27748,#27749));
#6556=EDGE_LOOP('',(#27750,#27751,#27752,#27753));
#6557=EDGE_LOOP('',(#27754,#27755,#27756,#27757));
#6558=EDGE_LOOP('',(#27758));
#6559=EDGE_LOOP('',(#27759,#27760,#27761,#27762,#27763,#27764,#27765,#27766,
#27767,#27768));
#6560=EDGE_LOOP('',(#27769,#27770,#27771,#27772));
#6561=EDGE_LOOP('',(#27773));
#6562=EDGE_LOOP('',(#27774));
#6563=EDGE_LOOP('',(#27775,#27776,#27777,#27778));
#6564=EDGE_LOOP('',(#27779));
#6565=EDGE_LOOP('',(#27780));
#6566=EDGE_LOOP('',(#27781,#27782,#27783,#27784));
#6567=EDGE_LOOP('',(#27785));
#6568=EDGE_LOOP('',(#27786));
#6569=EDGE_LOOP('',(#27787,#27788,#27789,#27790));
#6570=EDGE_LOOP('',(#27791,#27792,#27793,#27794));
#6571=EDGE_LOOP('',(#27795,#27796,#27797,#27798));
#6572=EDGE_LOOP('',(#27799));
#6573=EDGE_LOOP('',(#27800));
#6574=EDGE_LOOP('',(#27801));
#6575=EDGE_LOOP('',(#27802));
#6576=EDGE_LOOP('',(#27803));
#6577=EDGE_LOOP('',(#27804));
#6578=EDGE_LOOP('',(#27805));
#6579=EDGE_LOOP('',(#27806,#27807,#27808,#27809));
#6580=EDGE_LOOP('',(#27810,#27811,#27812,#27813));
#7534=LINE('',#47311,#10584);
#7535=LINE('',#47317,#10585);
#7536=LINE('',#47324,#10586);
#7537=LINE('',#47327,#10587);
#7538=LINE('',#47336,#10588);
#7539=LINE('',#47343,#10589);
#7540=LINE('',#47351,#10590);
#7541=LINE('',#47357,#10591);
#7542=LINE('',#47366,#10592);
#7543=LINE('',#47372,#10593);
#7544=LINE('',#47380,#10594);
#7545=LINE('',#47386,#10595);
#7546=LINE('',#47393,#10596);
#7547=LINE('',#47396,#10597);
#7548=LINE('',#47402,#10598);
#7549=LINE('',#47408,#10599);
#7550=LINE('',#47414,#10600);
#7551=LINE('',#47420,#10601);
#7552=LINE('',#47426,#10602);
#7553=LINE('',#47432,#10603);
#7554=LINE('',#47438,#10604);
#7555=LINE('',#47445,#10605);
#7556=LINE('',#47451,#10606);
#7557=LINE('',#47459,#10607);
#7558=LINE('',#47467,#10608);
#7559=LINE('',#47475,#10609);
#7560=LINE('',#47483,#10610);
#7561=LINE('',#47491,#10611);
#7562=LINE('',#47499,#10612);
#7563=LINE('',#47507,#10613);
#7564=LINE('',#47515,#10614);
#7565=LINE('',#47523,#10615);
#7566=LINE('',#47531,#10616);
#7567=LINE('',#47539,#10617);
#7568=LINE('',#47547,#10618);
#7569=LINE('',#47555,#10619);
#7570=LINE('',#47563,#10620);
#7571=LINE('',#47571,#10621);
#7572=LINE('',#47579,#10622);
#7573=LINE('',#47587,#10623);
#7574=LINE('',#47595,#10624);
#7575=LINE('',#47603,#10625);
#7576=LINE('',#47611,#10626);
#7577=LINE('',#47619,#10627);
#7578=LINE('',#47627,#10628);
#7579=LINE('',#47635,#10629);
#7580=LINE('',#47643,#10630);
#7581=LINE('',#47651,#10631);
#7582=LINE('',#47659,#10632);
#7583=LINE('',#47667,#10633);
#7584=LINE('',#47675,#10634);
#7585=LINE('',#47683,#10635);
#7586=LINE('',#47691,#10636);
#7587=LINE('',#47699,#10637);
#7588=LINE('',#47707,#10638);
#7589=LINE('',#47715,#10639);
#7590=LINE('',#47723,#10640);
#7591=LINE('',#47731,#10641);
#7592=LINE('',#47739,#10642);
#7593=LINE('',#47747,#10643);
#7594=LINE('',#47755,#10644);
#7595=LINE('',#47763,#10645);
#7596=LINE('',#47771,#10646);
#7597=LINE('',#47779,#10647);
#7598=LINE('',#47787,#10648);
#7599=LINE('',#47795,#10649);
#7600=LINE('',#47803,#10650);
#7601=LINE('',#47811,#10651);
#7602=LINE('',#47819,#10652);
#7603=LINE('',#47827,#10653);
#7604=LINE('',#47835,#10654);
#7605=LINE('',#47843,#10655);
#7606=LINE('',#47851,#10656);
#7607=LINE('',#47859,#10657);
#7608=LINE('',#47867,#10658);
#7609=LINE('',#47875,#10659);
#7610=LINE('',#47883,#10660);
#7611=LINE('',#47891,#10661);
#7612=LINE('',#47899,#10662);
#7613=LINE('',#47907,#10663);
#7614=LINE('',#47915,#10664);
#7615=LINE('',#47923,#10665);
#7616=LINE('',#47931,#10666);
#7617=LINE('',#47939,#10667);
#7618=LINE('',#47947,#10668);
#7619=LINE('',#47955,#10669);
#7620=LINE('',#47963,#10670);
#7621=LINE('',#47971,#10671);
#7622=LINE('',#47979,#10672);
#7623=LINE('',#47987,#10673);
#7624=LINE('',#47995,#10674);
#7625=LINE('',#48003,#10675);
#7626=LINE('',#48011,#10676);
#7627=LINE('',#48019,#10677);
#7628=LINE('',#48027,#10678);
#7629=LINE('',#48035,#10679);
#7630=LINE('',#48043,#10680);
#7631=LINE('',#48051,#10681);
#7632=LINE('',#48059,#10682);
#7633=LINE('',#48067,#10683);
#7634=LINE('',#48075,#10684);
#7635=LINE('',#48083,#10685);
#7636=LINE('',#48091,#10686);
#7637=LINE('',#48099,#10687);
#7638=LINE('',#48107,#10688);
#7639=LINE('',#48115,#10689);
#7640=LINE('',#48123,#10690);
#7641=LINE('',#48131,#10691);
#7642=LINE('',#48139,#10692);
#7643=LINE('',#48147,#10693);
#7644=LINE('',#48155,#10694);
#7645=LINE('',#48163,#10695);
#7646=LINE('',#48171,#10696);
#7647=LINE('',#48179,#10697);
#7648=LINE('',#48187,#10698);
#7649=LINE('',#48195,#10699);
#7650=LINE('',#48203,#10700);
#7651=LINE('',#48211,#10701);
#7652=LINE('',#48219,#10702);
#7653=LINE('',#48227,#10703);
#7654=LINE('',#48235,#10704);
#7655=LINE('',#48243,#10705);
#7656=LINE('',#48251,#10706);
#7657=LINE('',#48259,#10707);
#7658=LINE('',#48267,#10708);
#7659=LINE('',#48275,#10709);
#7660=LINE('',#48283,#10710);
#7661=LINE('',#48291,#10711);
#7662=LINE('',#48299,#10712);
#7663=LINE('',#48307,#10713);
#7664=LINE('',#48315,#10714);
#7665=LINE('',#48323,#10715);
#7666=LINE('',#48331,#10716);
#7667=LINE('',#48339,#10717);
#7668=LINE('',#48347,#10718);
#7669=LINE('',#48355,#10719);
#7670=LINE('',#48363,#10720);
#7671=LINE('',#48371,#10721);
#7672=LINE('',#48379,#10722);
#7673=LINE('',#48387,#10723);
#7674=LINE('',#48395,#10724);
#7675=LINE('',#48403,#10725);
#7676=LINE('',#48411,#10726);
#7677=LINE('',#48419,#10727);
#7678=LINE('',#48427,#10728);
#7679=LINE('',#48435,#10729);
#7680=LINE('',#48443,#10730);
#7681=LINE('',#48451,#10731);
#7682=LINE('',#48459,#10732);
#7683=LINE('',#48467,#10733);
#7684=LINE('',#48475,#10734);
#7685=LINE('',#48483,#10735);
#7686=LINE('',#48491,#10736);
#7687=LINE('',#48499,#10737);
#7688=LINE('',#48507,#10738);
#7689=LINE('',#48515,#10739);
#7690=LINE('',#48523,#10740);
#7691=LINE('',#48531,#10741);
#7692=LINE('',#48539,#10742);
#7693=LINE('',#48547,#10743);
#7694=LINE('',#48555,#10744);
#7695=LINE('',#48563,#10745);
#7696=LINE('',#48571,#10746);
#7697=LINE('',#48579,#10747);
#7698=LINE('',#48677,#10748);
#7699=LINE('',#48680,#10749);
#7700=LINE('',#48683,#10750);
#7701=LINE('',#48687,#10751);
#7702=LINE('',#48691,#10752);
#7703=LINE('',#48695,#10753);
#7704=LINE('',#48699,#10754);
#7705=LINE('',#48715,#10755);
#7706=LINE('',#48716,#10756);
#7707=LINE('',#48718,#10757);
#7708=LINE('',#48719,#10758);
#7709=LINE('',#48722,#10759);
#7710=LINE('',#48723,#10760);
#7711=LINE('',#48726,#10761);
#7712=LINE('',#48728,#10762);
#7713=LINE('',#48729,#10763);
#7714=LINE('',#48732,#10764);
#7715=LINE('',#48734,#10765);
#7716=LINE('',#48735,#10766);
#7717=LINE('',#48738,#10767);
#7718=LINE('',#48739,#10768);
#7719=LINE('',#48742,#10769);
#7720=LINE('',#48743,#10770);
#7721=LINE('',#48745,#10771);
#7722=LINE('',#48746,#10772);
#7723=LINE('',#48750,#10773);
#7724=LINE('',#48752,#10774);
#7725=LINE('',#48753,#10775);
#7726=LINE('',#48755,#10776);
#7727=LINE('',#48756,#10777);
#7728=LINE('',#48758,#10778);
#7729=LINE('',#48759,#10779);
#7730=LINE('',#48761,#10780);
#7731=LINE('',#48762,#10781);
#7732=LINE('',#48764,#10782);
#7733=LINE('',#48770,#10783);
#7734=LINE('',#48772,#10784);
#7735=LINE('',#48773,#10785);
#7736=LINE('',#48777,#10786);
#7737=LINE('',#48779,#10787);
#7738=LINE('',#48780,#10788);
#7739=LINE('',#48784,#10789);
#7740=LINE('',#48786,#10790);
#7741=LINE('',#48787,#10791);
#7742=LINE('',#48789,#10792);
#7743=LINE('',#48790,#10793);
#7744=LINE('',#48794,#10794);
#7745=LINE('',#48796,#10795);
#7746=LINE('',#48797,#10796);
#7747=LINE('',#48799,#10797);
#7748=LINE('',#48800,#10798);
#7749=LINE('',#48802,#10799);
#7750=LINE('',#48803,#10800);
#7751=LINE('',#48805,#10801);
#7752=LINE('',#48806,#10802);
#7753=LINE('',#48808,#10803);
#7754=LINE('',#48809,#10804);
#7755=LINE('',#48811,#10805);
#7756=LINE('',#48812,#10806);
#7757=LINE('',#48814,#10807);
#7758=LINE('',#48815,#10808);
#7759=LINE('',#48817,#10809);
#7760=LINE('',#48818,#10810);
#7761=LINE('',#48825,#10811);
#7762=LINE('',#48827,#10812);
#7763=LINE('',#48828,#10813);
#7764=LINE('',#48832,#10814);
#7765=LINE('',#48833,#10815);
#7766=LINE('',#48835,#10816);
#7767=LINE('',#48836,#10817);
#7768=LINE('',#48838,#10818);
#7769=LINE('',#48839,#10819);
#7770=LINE('',#48843,#10820);
#7771=LINE('',#48845,#10821);
#7772=LINE('',#48846,#10822);
#7773=LINE('',#48850,#10823);
#7774=LINE('',#48851,#10824);
#7775=LINE('',#48853,#10825);
#7776=LINE('',#48854,#10826);
#7777=LINE('',#48856,#10827);
#7778=LINE('',#48857,#10828);
#7779=LINE('',#48859,#10829);
#7780=LINE('',#48860,#10830);
#7781=LINE('',#48863,#10831);
#7782=LINE('',#48864,#10832);
#7783=LINE('',#48865,#10833);
#7784=LINE('',#48867,#10834);
#7785=LINE('',#48870,#10835);
#7786=LINE('',#48871,#10836);
#7787=LINE('',#48873,#10837);
#7788=LINE('',#48874,#10838);
#7789=LINE('',#48880,#10839);
#7790=LINE('',#48882,#10840);
#7791=LINE('',#48883,#10841);
#7792=LINE('',#48887,#10842);
#7793=LINE('',#48889,#10843);
#7794=LINE('',#48890,#10844);
#7795=LINE('',#48894,#10845);
#7796=LINE('',#48896,#10846);
#7797=LINE('',#48897,#10847);
#7798=LINE('',#48899,#10848);
#7799=LINE('',#48900,#10849);
#7800=LINE('',#48904,#10850);
#7801=LINE('',#48906,#10851);
#7802=LINE('',#48907,#10852);
#7803=LINE('',#48909,#10853);
#7804=LINE('',#48910,#10854);
#7805=LINE('',#48912,#10855);
#7806=LINE('',#48913,#10856);
#7807=LINE('',#48915,#10857);
#7808=LINE('',#48916,#10858);
#7809=LINE('',#48918,#10859);
#7810=LINE('',#48919,#10860);
#7811=LINE('',#48921,#10861);
#7812=LINE('',#48922,#10862);
#7813=LINE('',#48924,#10863);
#7814=LINE('',#48925,#10864);
#7815=LINE('',#48927,#10865);
#7816=LINE('',#48928,#10866);
#7817=LINE('',#48935,#10867);
#7818=LINE('',#48937,#10868);
#7819=LINE('',#48938,#10869);
#7820=LINE('',#48942,#10870);
#7821=LINE('',#48944,#10871);
#7822=LINE('',#48945,#10872);
#7823=LINE('',#48949,#10873);
#7824=LINE('',#48951,#10874);
#7825=LINE('',#48952,#10875);
#7826=LINE('',#48954,#10876);
#7827=LINE('',#48955,#10877);
#7828=LINE('',#48959,#10878);
#7829=LINE('',#48961,#10879);
#7830=LINE('',#48962,#10880);
#7831=LINE('',#48964,#10881);
#7832=LINE('',#48965,#10882);
#7833=LINE('',#48967,#10883);
#7834=LINE('',#48968,#10884);
#7835=LINE('',#48970,#10885);
#7836=LINE('',#48971,#10886);
#7837=LINE('',#48973,#10887);
#7838=LINE('',#48974,#10888);
#7839=LINE('',#48976,#10889);
#7840=LINE('',#48977,#10890);
#7841=LINE('',#48979,#10891);
#7842=LINE('',#48980,#10892);
#7843=LINE('',#48982,#10893);
#7844=LINE('',#48983,#10894);
#7845=LINE('',#48990,#10895);
#7846=LINE('',#48991,#10896);
#7847=LINE('',#48993,#10897);
#7848=LINE('',#48994,#10898);
#7849=LINE('',#48997,#10899);
#7850=LINE('',#48998,#10900);
#7851=LINE('',#49001,#10901);
#7852=LINE('',#49003,#10902);
#7853=LINE('',#49004,#10903);
#7854=LINE('',#49007,#10904);
#7855=LINE('',#49009,#10905);
#7856=LINE('',#49010,#10906);
#7857=LINE('',#49013,#10907);
#7858=LINE('',#49014,#10908);
#7859=LINE('',#49017,#10909);
#7860=LINE('',#49018,#10910);
#7861=LINE('',#49020,#10911);
#7862=LINE('',#49021,#10912);
#7863=LINE('',#49025,#10913);
#7864=LINE('',#49027,#10914);
#7865=LINE('',#49028,#10915);
#7866=LINE('',#49030,#10916);
#7867=LINE('',#49031,#10917);
#7868=LINE('',#49033,#10918);
#7869=LINE('',#49034,#10919);
#7870=LINE('',#49036,#10920);
#7871=LINE('',#49037,#10921);
#7872=LINE('',#49039,#10922);
#7873=LINE('',#49045,#10923);
#7874=LINE('',#49047,#10924);
#7875=LINE('',#49048,#10925);
#7876=LINE('',#49052,#10926);
#7877=LINE('',#49054,#10927);
#7878=LINE('',#49055,#10928);
#7879=LINE('',#49059,#10929);
#7880=LINE('',#49061,#10930);
#7881=LINE('',#49062,#10931);
#7882=LINE('',#49064,#10932);
#7883=LINE('',#49065,#10933);
#7884=LINE('',#49069,#10934);
#7885=LINE('',#49071,#10935);
#7886=LINE('',#49072,#10936);
#7887=LINE('',#49074,#10937);
#7888=LINE('',#49075,#10938);
#7889=LINE('',#49077,#10939);
#7890=LINE('',#49078,#10940);
#7891=LINE('',#49080,#10941);
#7892=LINE('',#49081,#10942);
#7893=LINE('',#49083,#10943);
#7894=LINE('',#49084,#10944);
#7895=LINE('',#49086,#10945);
#7896=LINE('',#49087,#10946);
#7897=LINE('',#49089,#10947);
#7898=LINE('',#49090,#10948);
#7899=LINE('',#49092,#10949);
#7900=LINE('',#49093,#10950);
#7901=LINE('',#49100,#10951);
#7902=LINE('',#49102,#10952);
#7903=LINE('',#49103,#10953);
#7904=LINE('',#49107,#10954);
#7905=LINE('',#49108,#10955);
#7906=LINE('',#49110,#10956);
#7907=LINE('',#49111,#10957);
#7908=LINE('',#49113,#10958);
#7909=LINE('',#49114,#10959);
#7910=LINE('',#49118,#10960);
#7911=LINE('',#49120,#10961);
#7912=LINE('',#49121,#10962);
#7913=LINE('',#49125,#10963);
#7914=LINE('',#49126,#10964);
#7915=LINE('',#49128,#10965);
#7916=LINE('',#49129,#10966);
#7917=LINE('',#49131,#10967);
#7918=LINE('',#49132,#10968);
#7919=LINE('',#49134,#10969);
#7920=LINE('',#49135,#10970);
#7921=LINE('',#49138,#10971);
#7922=LINE('',#49139,#10972);
#7923=LINE('',#49140,#10973);
#7924=LINE('',#49142,#10974);
#7925=LINE('',#49145,#10975);
#7926=LINE('',#49146,#10976);
#7927=LINE('',#49148,#10977);
#7928=LINE('',#49149,#10978);
#7929=LINE('',#49155,#10979);
#7930=LINE('',#49157,#10980);
#7931=LINE('',#49158,#10981);
#7932=LINE('',#49162,#10982);
#7933=LINE('',#49164,#10983);
#7934=LINE('',#49165,#10984);
#7935=LINE('',#49169,#10985);
#7936=LINE('',#49171,#10986);
#7937=LINE('',#49172,#10987);
#7938=LINE('',#49174,#10988);
#7939=LINE('',#49175,#10989);
#7940=LINE('',#49179,#10990);
#7941=LINE('',#49181,#10991);
#7942=LINE('',#49182,#10992);
#7943=LINE('',#49184,#10993);
#7944=LINE('',#49185,#10994);
#7945=LINE('',#49187,#10995);
#7946=LINE('',#49188,#10996);
#7947=LINE('',#49190,#10997);
#7948=LINE('',#49191,#10998);
#7949=LINE('',#49193,#10999);
#7950=LINE('',#49194,#11000);
#7951=LINE('',#49196,#11001);
#7952=LINE('',#49197,#11002);
#7953=LINE('',#49199,#11003);
#7954=LINE('',#49200,#11004);
#7955=LINE('',#49202,#11005);
#7956=LINE('',#49203,#11006);
#7957=LINE('',#49210,#11007);
#7958=LINE('',#49212,#11008);
#7959=LINE('',#49213,#11009);
#7960=LINE('',#49217,#11010);
#7961=LINE('',#49219,#11011);
#7962=LINE('',#49220,#11012);
#7963=LINE('',#49224,#11013);
#7964=LINE('',#49226,#11014);
#7965=LINE('',#49227,#11015);
#7966=LINE('',#49229,#11016);
#7967=LINE('',#49230,#11017);
#7968=LINE('',#49234,#11018);
#7969=LINE('',#49236,#11019);
#7970=LINE('',#49237,#11020);
#7971=LINE('',#49239,#11021);
#7972=LINE('',#49240,#11022);
#7973=LINE('',#49242,#11023);
#7974=LINE('',#49243,#11024);
#7975=LINE('',#49245,#11025);
#7976=LINE('',#49246,#11026);
#7977=LINE('',#49248,#11027);
#7978=LINE('',#49249,#11028);
#7979=LINE('',#49251,#11029);
#7980=LINE('',#49252,#11030);
#7981=LINE('',#49254,#11031);
#7982=LINE('',#49255,#11032);
#7983=LINE('',#49257,#11033);
#7984=LINE('',#49258,#11034);
#7985=LINE('',#49265,#11035);
#7986=LINE('',#49266,#11036);
#7987=LINE('',#49268,#11037);
#7988=LINE('',#49269,#11038);
#7989=LINE('',#49272,#11039);
#7990=LINE('',#49273,#11040);
#7991=LINE('',#49276,#11041);
#7992=LINE('',#49278,#11042);
#7993=LINE('',#49279,#11043);
#7994=LINE('',#49282,#11044);
#7995=LINE('',#49284,#11045);
#7996=LINE('',#49285,#11046);
#7997=LINE('',#49288,#11047);
#7998=LINE('',#49289,#11048);
#7999=LINE('',#49292,#11049);
#8000=LINE('',#49293,#11050);
#8001=LINE('',#49295,#11051);
#8002=LINE('',#49296,#11052);
#8003=LINE('',#49300,#11053);
#8004=LINE('',#49302,#11054);
#8005=LINE('',#49303,#11055);
#8006=LINE('',#49305,#11056);
#8007=LINE('',#49306,#11057);
#8008=LINE('',#49308,#11058);
#8009=LINE('',#49309,#11059);
#8010=LINE('',#49311,#11060);
#8011=LINE('',#49312,#11061);
#8012=LINE('',#49314,#11062);
#8013=LINE('',#49320,#11063);
#8014=LINE('',#49322,#11064);
#8015=LINE('',#49323,#11065);
#8016=LINE('',#49327,#11066);
#8017=LINE('',#49329,#11067);
#8018=LINE('',#49330,#11068);
#8019=LINE('',#49334,#11069);
#8020=LINE('',#49336,#11070);
#8021=LINE('',#49337,#11071);
#8022=LINE('',#49339,#11072);
#8023=LINE('',#49340,#11073);
#8024=LINE('',#49344,#11074);
#8025=LINE('',#49346,#11075);
#8026=LINE('',#49347,#11076);
#8027=LINE('',#49349,#11077);
#8028=LINE('',#49350,#11078);
#8029=LINE('',#49352,#11079);
#8030=LINE('',#49353,#11080);
#8031=LINE('',#49355,#11081);
#8032=LINE('',#49356,#11082);
#8033=LINE('',#49358,#11083);
#8034=LINE('',#49359,#11084);
#8035=LINE('',#49361,#11085);
#8036=LINE('',#49362,#11086);
#8037=LINE('',#49364,#11087);
#8038=LINE('',#49365,#11088);
#8039=LINE('',#49367,#11089);
#8040=LINE('',#49368,#11090);
#8041=LINE('',#49375,#11091);
#8042=LINE('',#49377,#11092);
#8043=LINE('',#49378,#11093);
#8044=LINE('',#49382,#11094);
#8045=LINE('',#49383,#11095);
#8046=LINE('',#49385,#11096);
#8047=LINE('',#49386,#11097);
#8048=LINE('',#49388,#11098);
#8049=LINE('',#49389,#11099);
#8050=LINE('',#49393,#11100);
#8051=LINE('',#49395,#11101);
#8052=LINE('',#49396,#11102);
#8053=LINE('',#49400,#11103);
#8054=LINE('',#49401,#11104);
#8055=LINE('',#49403,#11105);
#8056=LINE('',#49404,#11106);
#8057=LINE('',#49406,#11107);
#8058=LINE('',#49407,#11108);
#8059=LINE('',#49409,#11109);
#8060=LINE('',#49410,#11110);
#8061=LINE('',#49413,#11111);
#8062=LINE('',#49414,#11112);
#8063=LINE('',#49415,#11113);
#8064=LINE('',#49417,#11114);
#8065=LINE('',#49420,#11115);
#8066=LINE('',#49421,#11116);
#8067=LINE('',#49423,#11117);
#8068=LINE('',#49424,#11118);
#8069=LINE('',#49430,#11119);
#8070=LINE('',#49432,#11120);
#8071=LINE('',#49433,#11121);
#8072=LINE('',#49437,#11122);
#8073=LINE('',#49439,#11123);
#8074=LINE('',#49440,#11124);
#8075=LINE('',#49444,#11125);
#8076=LINE('',#49446,#11126);
#8077=LINE('',#49447,#11127);
#8078=LINE('',#49449,#11128);
#8079=LINE('',#49450,#11129);
#8080=LINE('',#49454,#11130);
#8081=LINE('',#49456,#11131);
#8082=LINE('',#49457,#11132);
#8083=LINE('',#49459,#11133);
#8084=LINE('',#49460,#11134);
#8085=LINE('',#49462,#11135);
#8086=LINE('',#49463,#11136);
#8087=LINE('',#49465,#11137);
#8088=LINE('',#49466,#11138);
#8089=LINE('',#49468,#11139);
#8090=LINE('',#49469,#11140);
#8091=LINE('',#49471,#11141);
#8092=LINE('',#49472,#11142);
#8093=LINE('',#49474,#11143);
#8094=LINE('',#49475,#11144);
#8095=LINE('',#49477,#11145);
#8096=LINE('',#49478,#11146);
#8097=LINE('',#49485,#11147);
#8098=LINE('',#49487,#11148);
#8099=LINE('',#49488,#11149);
#8100=LINE('',#49492,#11150);
#8101=LINE('',#49494,#11151);
#8102=LINE('',#49495,#11152);
#8103=LINE('',#49499,#11153);
#8104=LINE('',#49501,#11154);
#8105=LINE('',#49502,#11155);
#8106=LINE('',#49504,#11156);
#8107=LINE('',#49505,#11157);
#8108=LINE('',#49509,#11158);
#8109=LINE('',#49511,#11159);
#8110=LINE('',#49512,#11160);
#8111=LINE('',#49514,#11161);
#8112=LINE('',#49515,#11162);
#8113=LINE('',#49517,#11163);
#8114=LINE('',#49518,#11164);
#8115=LINE('',#49520,#11165);
#8116=LINE('',#49521,#11166);
#8117=LINE('',#49523,#11167);
#8118=LINE('',#49524,#11168);
#8119=LINE('',#49526,#11169);
#8120=LINE('',#49527,#11170);
#8121=LINE('',#49529,#11171);
#8122=LINE('',#49530,#11172);
#8123=LINE('',#49532,#11173);
#8124=LINE('',#49533,#11174);
#8125=LINE('',#49540,#11175);
#8126=LINE('',#49541,#11176);
#8127=LINE('',#49543,#11177);
#8128=LINE('',#49544,#11178);
#8129=LINE('',#49547,#11179);
#8130=LINE('',#49548,#11180);
#8131=LINE('',#49551,#11181);
#8132=LINE('',#49553,#11182);
#8133=LINE('',#49554,#11183);
#8134=LINE('',#49557,#11184);
#8135=LINE('',#49559,#11185);
#8136=LINE('',#49560,#11186);
#8137=LINE('',#49563,#11187);
#8138=LINE('',#49564,#11188);
#8139=LINE('',#49567,#11189);
#8140=LINE('',#49568,#11190);
#8141=LINE('',#49570,#11191);
#8142=LINE('',#49571,#11192);
#8143=LINE('',#49575,#11193);
#8144=LINE('',#49577,#11194);
#8145=LINE('',#49578,#11195);
#8146=LINE('',#49580,#11196);
#8147=LINE('',#49581,#11197);
#8148=LINE('',#49583,#11198);
#8149=LINE('',#49584,#11199);
#8150=LINE('',#49586,#11200);
#8151=LINE('',#49587,#11201);
#8152=LINE('',#49589,#11202);
#8153=LINE('',#49595,#11203);
#8154=LINE('',#49597,#11204);
#8155=LINE('',#49598,#11205);
#8156=LINE('',#49602,#11206);
#8157=LINE('',#49604,#11207);
#8158=LINE('',#49605,#11208);
#8159=LINE('',#49609,#11209);
#8160=LINE('',#49611,#11210);
#8161=LINE('',#49612,#11211);
#8162=LINE('',#49614,#11212);
#8163=LINE('',#49615,#11213);
#8164=LINE('',#49619,#11214);
#8165=LINE('',#49621,#11215);
#8166=LINE('',#49622,#11216);
#8167=LINE('',#49624,#11217);
#8168=LINE('',#49625,#11218);
#8169=LINE('',#49627,#11219);
#8170=LINE('',#49628,#11220);
#8171=LINE('',#49630,#11221);
#8172=LINE('',#49631,#11222);
#8173=LINE('',#49633,#11223);
#8174=LINE('',#49634,#11224);
#8175=LINE('',#49636,#11225);
#8176=LINE('',#49637,#11226);
#8177=LINE('',#49639,#11227);
#8178=LINE('',#49640,#11228);
#8179=LINE('',#49642,#11229);
#8180=LINE('',#49643,#11230);
#8181=LINE('',#49650,#11231);
#8182=LINE('',#49652,#11232);
#8183=LINE('',#49653,#11233);
#8184=LINE('',#49657,#11234);
#8185=LINE('',#49658,#11235);
#8186=LINE('',#49660,#11236);
#8187=LINE('',#49661,#11237);
#8188=LINE('',#49663,#11238);
#8189=LINE('',#49664,#11239);
#8190=LINE('',#49668,#11240);
#8191=LINE('',#49670,#11241);
#8192=LINE('',#49671,#11242);
#8193=LINE('',#49675,#11243);
#8194=LINE('',#49676,#11244);
#8195=LINE('',#49678,#11245);
#8196=LINE('',#49679,#11246);
#8197=LINE('',#49681,#11247);
#8198=LINE('',#49682,#11248);
#8199=LINE('',#49684,#11249);
#8200=LINE('',#49685,#11250);
#8201=LINE('',#49688,#11251);
#8202=LINE('',#49689,#11252);
#8203=LINE('',#49690,#11253);
#8204=LINE('',#49692,#11254);
#8205=LINE('',#49695,#11255);
#8206=LINE('',#49696,#11256);
#8207=LINE('',#49698,#11257);
#8208=LINE('',#49699,#11258);
#8209=LINE('',#49705,#11259);
#8210=LINE('',#49707,#11260);
#8211=LINE('',#49708,#11261);
#8212=LINE('',#49712,#11262);
#8213=LINE('',#49714,#11263);
#8214=LINE('',#49715,#11264);
#8215=LINE('',#49719,#11265);
#8216=LINE('',#49721,#11266);
#8217=LINE('',#49722,#11267);
#8218=LINE('',#49724,#11268);
#8219=LINE('',#49725,#11269);
#8220=LINE('',#49729,#11270);
#8221=LINE('',#49731,#11271);
#8222=LINE('',#49732,#11272);
#8223=LINE('',#49734,#11273);
#8224=LINE('',#49735,#11274);
#8225=LINE('',#49737,#11275);
#8226=LINE('',#49738,#11276);
#8227=LINE('',#49740,#11277);
#8228=LINE('',#49741,#11278);
#8229=LINE('',#49743,#11279);
#8230=LINE('',#49744,#11280);
#8231=LINE('',#49746,#11281);
#8232=LINE('',#49747,#11282);
#8233=LINE('',#49749,#11283);
#8234=LINE('',#49750,#11284);
#8235=LINE('',#49752,#11285);
#8236=LINE('',#49753,#11286);
#8237=LINE('',#49760,#11287);
#8238=LINE('',#49762,#11288);
#8239=LINE('',#49763,#11289);
#8240=LINE('',#49767,#11290);
#8241=LINE('',#49769,#11291);
#8242=LINE('',#49770,#11292);
#8243=LINE('',#49774,#11293);
#8244=LINE('',#49776,#11294);
#8245=LINE('',#49777,#11295);
#8246=LINE('',#49779,#11296);
#8247=LINE('',#49780,#11297);
#8248=LINE('',#49784,#11298);
#8249=LINE('',#49786,#11299);
#8250=LINE('',#49787,#11300);
#8251=LINE('',#49789,#11301);
#8252=LINE('',#49790,#11302);
#8253=LINE('',#49792,#11303);
#8254=LINE('',#49793,#11304);
#8255=LINE('',#49795,#11305);
#8256=LINE('',#49796,#11306);
#8257=LINE('',#49798,#11307);
#8258=LINE('',#49799,#11308);
#8259=LINE('',#49801,#11309);
#8260=LINE('',#49802,#11310);
#8261=LINE('',#49804,#11311);
#8262=LINE('',#49805,#11312);
#8263=LINE('',#49807,#11313);
#8264=LINE('',#49808,#11314);
#8265=LINE('',#49815,#11315);
#8266=LINE('',#49816,#11316);
#8267=LINE('',#49818,#11317);
#8268=LINE('',#49819,#11318);
#8269=LINE('',#49822,#11319);
#8270=LINE('',#49823,#11320);
#8271=LINE('',#49826,#11321);
#8272=LINE('',#49828,#11322);
#8273=LINE('',#49829,#11323);
#8274=LINE('',#49832,#11324);
#8275=LINE('',#49834,#11325);
#8276=LINE('',#49835,#11326);
#8277=LINE('',#49838,#11327);
#8278=LINE('',#49839,#11328);
#8279=LINE('',#49842,#11329);
#8280=LINE('',#49843,#11330);
#8281=LINE('',#49845,#11331);
#8282=LINE('',#49846,#11332);
#8283=LINE('',#49850,#11333);
#8284=LINE('',#49852,#11334);
#8285=LINE('',#49853,#11335);
#8286=LINE('',#49855,#11336);
#8287=LINE('',#49856,#11337);
#8288=LINE('',#49858,#11338);
#8289=LINE('',#49859,#11339);
#8290=LINE('',#49861,#11340);
#8291=LINE('',#49862,#11341);
#8292=LINE('',#49864,#11342);
#8293=LINE('',#49870,#11343);
#8294=LINE('',#49872,#11344);
#8295=LINE('',#49873,#11345);
#8296=LINE('',#49877,#11346);
#8297=LINE('',#49879,#11347);
#8298=LINE('',#49880,#11348);
#8299=LINE('',#49884,#11349);
#8300=LINE('',#49886,#11350);
#8301=LINE('',#49887,#11351);
#8302=LINE('',#49889,#11352);
#8303=LINE('',#49890,#11353);
#8304=LINE('',#49894,#11354);
#8305=LINE('',#49896,#11355);
#8306=LINE('',#49897,#11356);
#8307=LINE('',#49899,#11357);
#8308=LINE('',#49900,#11358);
#8309=LINE('',#49902,#11359);
#8310=LINE('',#49903,#11360);
#8311=LINE('',#49905,#11361);
#8312=LINE('',#49906,#11362);
#8313=LINE('',#49908,#11363);
#8314=LINE('',#49909,#11364);
#8315=LINE('',#49911,#11365);
#8316=LINE('',#49912,#11366);
#8317=LINE('',#49914,#11367);
#8318=LINE('',#49915,#11368);
#8319=LINE('',#49917,#11369);
#8320=LINE('',#49918,#11370);
#8321=LINE('',#49925,#11371);
#8322=LINE('',#49927,#11372);
#8323=LINE('',#49928,#11373);
#8324=LINE('',#49932,#11374);
#8325=LINE('',#49933,#11375);
#8326=LINE('',#49935,#11376);
#8327=LINE('',#49936,#11377);
#8328=LINE('',#49938,#11378);
#8329=LINE('',#49939,#11379);
#8330=LINE('',#49943,#11380);
#8331=LINE('',#49945,#11381);
#8332=LINE('',#49946,#11382);
#8333=LINE('',#49950,#11383);
#8334=LINE('',#49951,#11384);
#8335=LINE('',#49953,#11385);
#8336=LINE('',#49954,#11386);
#8337=LINE('',#49956,#11387);
#8338=LINE('',#49957,#11388);
#8339=LINE('',#49959,#11389);
#8340=LINE('',#49960,#11390);
#8341=LINE('',#49963,#11391);
#8342=LINE('',#49964,#11392);
#8343=LINE('',#49965,#11393);
#8344=LINE('',#49967,#11394);
#8345=LINE('',#49970,#11395);
#8346=LINE('',#49971,#11396);
#8347=LINE('',#49973,#11397);
#8348=LINE('',#49974,#11398);
#8349=LINE('',#49980,#11399);
#8350=LINE('',#49982,#11400);
#8351=LINE('',#49983,#11401);
#8352=LINE('',#49987,#11402);
#8353=LINE('',#49989,#11403);
#8354=LINE('',#49990,#11404);
#8355=LINE('',#49994,#11405);
#8356=LINE('',#49996,#11406);
#8357=LINE('',#49997,#11407);
#8358=LINE('',#49999,#11408);
#8359=LINE('',#50000,#11409);
#8360=LINE('',#50004,#11410);
#8361=LINE('',#50006,#11411);
#8362=LINE('',#50007,#11412);
#8363=LINE('',#50009,#11413);
#8364=LINE('',#50010,#11414);
#8365=LINE('',#50012,#11415);
#8366=LINE('',#50013,#11416);
#8367=LINE('',#50015,#11417);
#8368=LINE('',#50016,#11418);
#8369=LINE('',#50018,#11419);
#8370=LINE('',#50019,#11420);
#8371=LINE('',#50021,#11421);
#8372=LINE('',#50022,#11422);
#8373=LINE('',#50024,#11423);
#8374=LINE('',#50025,#11424);
#8375=LINE('',#50027,#11425);
#8376=LINE('',#50028,#11426);
#8377=LINE('',#50035,#11427);
#8378=LINE('',#50037,#11428);
#8379=LINE('',#50038,#11429);
#8380=LINE('',#50042,#11430);
#8381=LINE('',#50044,#11431);
#8382=LINE('',#50045,#11432);
#8383=LINE('',#50049,#11433);
#8384=LINE('',#50051,#11434);
#8385=LINE('',#50052,#11435);
#8386=LINE('',#50054,#11436);
#8387=LINE('',#50055,#11437);
#8388=LINE('',#50059,#11438);
#8389=LINE('',#50061,#11439);
#8390=LINE('',#50062,#11440);
#8391=LINE('',#50064,#11441);
#8392=LINE('',#50065,#11442);
#8393=LINE('',#50067,#11443);
#8394=LINE('',#50068,#11444);
#8395=LINE('',#50070,#11445);
#8396=LINE('',#50071,#11446);
#8397=LINE('',#50073,#11447);
#8398=LINE('',#50074,#11448);
#8399=LINE('',#50076,#11449);
#8400=LINE('',#50077,#11450);
#8401=LINE('',#50079,#11451);
#8402=LINE('',#50080,#11452);
#8403=LINE('',#50082,#11453);
#8404=LINE('',#50083,#11454);
#8405=LINE('',#50090,#11455);
#8406=LINE('',#50091,#11456);
#8407=LINE('',#50093,#11457);
#8408=LINE('',#50094,#11458);
#8409=LINE('',#50097,#11459);
#8410=LINE('',#50098,#11460);
#8411=LINE('',#50101,#11461);
#8412=LINE('',#50103,#11462);
#8413=LINE('',#50104,#11463);
#8414=LINE('',#50107,#11464);
#8415=LINE('',#50109,#11465);
#8416=LINE('',#50110,#11466);
#8417=LINE('',#50113,#11467);
#8418=LINE('',#50114,#11468);
#8419=LINE('',#50117,#11469);
#8420=LINE('',#50118,#11470);
#8421=LINE('',#50120,#11471);
#8422=LINE('',#50121,#11472);
#8423=LINE('',#50125,#11473);
#8424=LINE('',#50127,#11474);
#8425=LINE('',#50128,#11475);
#8426=LINE('',#50130,#11476);
#8427=LINE('',#50131,#11477);
#8428=LINE('',#50133,#11478);
#8429=LINE('',#50134,#11479);
#8430=LINE('',#50136,#11480);
#8431=LINE('',#50137,#11481);
#8432=LINE('',#50139,#11482);
#8433=LINE('',#50145,#11483);
#8434=LINE('',#50147,#11484);
#8435=LINE('',#50148,#11485);
#8436=LINE('',#50152,#11486);
#8437=LINE('',#50154,#11487);
#8438=LINE('',#50155,#11488);
#8439=LINE('',#50159,#11489);
#8440=LINE('',#50161,#11490);
#8441=LINE('',#50162,#11491);
#8442=LINE('',#50164,#11492);
#8443=LINE('',#50165,#11493);
#8444=LINE('',#50169,#11494);
#8445=LINE('',#50171,#11495);
#8446=LINE('',#50172,#11496);
#8447=LINE('',#50174,#11497);
#8448=LINE('',#50175,#11498);
#8449=LINE('',#50177,#11499);
#8450=LINE('',#50178,#11500);
#8451=LINE('',#50180,#11501);
#8452=LINE('',#50181,#11502);
#8453=LINE('',#50183,#11503);
#8454=LINE('',#50184,#11504);
#8455=LINE('',#50186,#11505);
#8456=LINE('',#50187,#11506);
#8457=LINE('',#50189,#11507);
#8458=LINE('',#50190,#11508);
#8459=LINE('',#50192,#11509);
#8460=LINE('',#50193,#11510);
#8461=LINE('',#50200,#11511);
#8462=LINE('',#50202,#11512);
#8463=LINE('',#50203,#11513);
#8464=LINE('',#50207,#11514);
#8465=LINE('',#50208,#11515);
#8466=LINE('',#50210,#11516);
#8467=LINE('',#50211,#11517);
#8468=LINE('',#50213,#11518);
#8469=LINE('',#50214,#11519);
#8470=LINE('',#50218,#11520);
#8471=LINE('',#50220,#11521);
#8472=LINE('',#50221,#11522);
#8473=LINE('',#50225,#11523);
#8474=LINE('',#50226,#11524);
#8475=LINE('',#50228,#11525);
#8476=LINE('',#50229,#11526);
#8477=LINE('',#50231,#11527);
#8478=LINE('',#50232,#11528);
#8479=LINE('',#50234,#11529);
#8480=LINE('',#50235,#11530);
#8481=LINE('',#50238,#11531);
#8482=LINE('',#50239,#11532);
#8483=LINE('',#50240,#11533);
#8484=LINE('',#50242,#11534);
#8485=LINE('',#50245,#11535);
#8486=LINE('',#50246,#11536);
#8487=LINE('',#50248,#11537);
#8488=LINE('',#50249,#11538);
#8489=LINE('',#50255,#11539);
#8490=LINE('',#50257,#11540);
#8491=LINE('',#50258,#11541);
#8492=LINE('',#50262,#11542);
#8493=LINE('',#50264,#11543);
#8494=LINE('',#50265,#11544);
#8495=LINE('',#50269,#11545);
#8496=LINE('',#50271,#11546);
#8497=LINE('',#50272,#11547);
#8498=LINE('',#50274,#11548);
#8499=LINE('',#50275,#11549);
#8500=LINE('',#50279,#11550);
#8501=LINE('',#50281,#11551);
#8502=LINE('',#50282,#11552);
#8503=LINE('',#50284,#11553);
#8504=LINE('',#50285,#11554);
#8505=LINE('',#50287,#11555);
#8506=LINE('',#50288,#11556);
#8507=LINE('',#50290,#11557);
#8508=LINE('',#50291,#11558);
#8509=LINE('',#50293,#11559);
#8510=LINE('',#50294,#11560);
#8511=LINE('',#50296,#11561);
#8512=LINE('',#50297,#11562);
#8513=LINE('',#50299,#11563);
#8514=LINE('',#50300,#11564);
#8515=LINE('',#50302,#11565);
#8516=LINE('',#50303,#11566);
#8517=LINE('',#50310,#11567);
#8518=LINE('',#50312,#11568);
#8519=LINE('',#50313,#11569);
#8520=LINE('',#50317,#11570);
#8521=LINE('',#50319,#11571);
#8522=LINE('',#50320,#11572);
#8523=LINE('',#50324,#11573);
#8524=LINE('',#50326,#11574);
#8525=LINE('',#50327,#11575);
#8526=LINE('',#50329,#11576);
#8527=LINE('',#50330,#11577);
#8528=LINE('',#50334,#11578);
#8529=LINE('',#50336,#11579);
#8530=LINE('',#50337,#11580);
#8531=LINE('',#50339,#11581);
#8532=LINE('',#50340,#11582);
#8533=LINE('',#50342,#11583);
#8534=LINE('',#50343,#11584);
#8535=LINE('',#50345,#11585);
#8536=LINE('',#50346,#11586);
#8537=LINE('',#50348,#11587);
#8538=LINE('',#50349,#11588);
#8539=LINE('',#50351,#11589);
#8540=LINE('',#50352,#11590);
#8541=LINE('',#50354,#11591);
#8542=LINE('',#50355,#11592);
#8543=LINE('',#50357,#11593);
#8544=LINE('',#50358,#11594);
#8545=LINE('',#50365,#11595);
#8546=LINE('',#50366,#11596);
#8547=LINE('',#50368,#11597);
#8548=LINE('',#50369,#11598);
#8549=LINE('',#50372,#11599);
#8550=LINE('',#50373,#11600);
#8551=LINE('',#50376,#11601);
#8552=LINE('',#50378,#11602);
#8553=LINE('',#50379,#11603);
#8554=LINE('',#50382,#11604);
#8555=LINE('',#50384,#11605);
#8556=LINE('',#50385,#11606);
#8557=LINE('',#50388,#11607);
#8558=LINE('',#50389,#11608);
#8559=LINE('',#50392,#11609);
#8560=LINE('',#50393,#11610);
#8561=LINE('',#50395,#11611);
#8562=LINE('',#50396,#11612);
#8563=LINE('',#50400,#11613);
#8564=LINE('',#50402,#11614);
#8565=LINE('',#50403,#11615);
#8566=LINE('',#50405,#11616);
#8567=LINE('',#50406,#11617);
#8568=LINE('',#50408,#11618);
#8569=LINE('',#50409,#11619);
#8570=LINE('',#50411,#11620);
#8571=LINE('',#50412,#11621);
#8572=LINE('',#50414,#11622);
#8573=LINE('',#50420,#11623);
#8574=LINE('',#50422,#11624);
#8575=LINE('',#50423,#11625);
#8576=LINE('',#50427,#11626);
#8577=LINE('',#50429,#11627);
#8578=LINE('',#50430,#11628);
#8579=LINE('',#50434,#11629);
#8580=LINE('',#50436,#11630);
#8581=LINE('',#50437,#11631);
#8582=LINE('',#50439,#11632);
#8583=LINE('',#50440,#11633);
#8584=LINE('',#50444,#11634);
#8585=LINE('',#50446,#11635);
#8586=LINE('',#50447,#11636);
#8587=LINE('',#50449,#11637);
#8588=LINE('',#50450,#11638);
#8589=LINE('',#50452,#11639);
#8590=LINE('',#50453,#11640);
#8591=LINE('',#50455,#11641);
#8592=LINE('',#50456,#11642);
#8593=LINE('',#50458,#11643);
#8594=LINE('',#50459,#11644);
#8595=LINE('',#50461,#11645);
#8596=LINE('',#50462,#11646);
#8597=LINE('',#50464,#11647);
#8598=LINE('',#50465,#11648);
#8599=LINE('',#50467,#11649);
#8600=LINE('',#50468,#11650);
#8601=LINE('',#50475,#11651);
#8602=LINE('',#50477,#11652);
#8603=LINE('',#50478,#11653);
#8604=LINE('',#50482,#11654);
#8605=LINE('',#50483,#11655);
#8606=LINE('',#50485,#11656);
#8607=LINE('',#50486,#11657);
#8608=LINE('',#50488,#11658);
#8609=LINE('',#50489,#11659);
#8610=LINE('',#50493,#11660);
#8611=LINE('',#50495,#11661);
#8612=LINE('',#50496,#11662);
#8613=LINE('',#50500,#11663);
#8614=LINE('',#50501,#11664);
#8615=LINE('',#50503,#11665);
#8616=LINE('',#50504,#11666);
#8617=LINE('',#50506,#11667);
#8618=LINE('',#50507,#11668);
#8619=LINE('',#50509,#11669);
#8620=LINE('',#50510,#11670);
#8621=LINE('',#50513,#11671);
#8622=LINE('',#50514,#11672);
#8623=LINE('',#50515,#11673);
#8624=LINE('',#50517,#11674);
#8625=LINE('',#50520,#11675);
#8626=LINE('',#50521,#11676);
#8627=LINE('',#50523,#11677);
#8628=LINE('',#50524,#11678);
#8629=LINE('',#50530,#11679);
#8630=LINE('',#50532,#11680);
#8631=LINE('',#50533,#11681);
#8632=LINE('',#50537,#11682);
#8633=LINE('',#50539,#11683);
#8634=LINE('',#50540,#11684);
#8635=LINE('',#50544,#11685);
#8636=LINE('',#50546,#11686);
#8637=LINE('',#50547,#11687);
#8638=LINE('',#50549,#11688);
#8639=LINE('',#50550,#11689);
#8640=LINE('',#50554,#11690);
#8641=LINE('',#50556,#11691);
#8642=LINE('',#50557,#11692);
#8643=LINE('',#50559,#11693);
#8644=LINE('',#50560,#11694);
#8645=LINE('',#50562,#11695);
#8646=LINE('',#50563,#11696);
#8647=LINE('',#50565,#11697);
#8648=LINE('',#50566,#11698);
#8649=LINE('',#50568,#11699);
#8650=LINE('',#50569,#11700);
#8651=LINE('',#50571,#11701);
#8652=LINE('',#50572,#11702);
#8653=LINE('',#50574,#11703);
#8654=LINE('',#50575,#11704);
#8655=LINE('',#50577,#11705);
#8656=LINE('',#50578,#11706);
#8657=LINE('',#50585,#11707);
#8658=LINE('',#50587,#11708);
#8659=LINE('',#50588,#11709);
#8660=LINE('',#50592,#11710);
#8661=LINE('',#50594,#11711);
#8662=LINE('',#50595,#11712);
#8663=LINE('',#50599,#11713);
#8664=LINE('',#50601,#11714);
#8665=LINE('',#50602,#11715);
#8666=LINE('',#50604,#11716);
#8667=LINE('',#50605,#11717);
#8668=LINE('',#50609,#11718);
#8669=LINE('',#50611,#11719);
#8670=LINE('',#50612,#11720);
#8671=LINE('',#50614,#11721);
#8672=LINE('',#50615,#11722);
#8673=LINE('',#50617,#11723);
#8674=LINE('',#50618,#11724);
#8675=LINE('',#50620,#11725);
#8676=LINE('',#50621,#11726);
#8677=LINE('',#50623,#11727);
#8678=LINE('',#50624,#11728);
#8679=LINE('',#50626,#11729);
#8680=LINE('',#50627,#11730);
#8681=LINE('',#50629,#11731);
#8682=LINE('',#50630,#11732);
#8683=LINE('',#50632,#11733);
#8684=LINE('',#50633,#11734);
#8685=LINE('',#50640,#11735);
#8686=LINE('',#50641,#11736);
#8687=LINE('',#50643,#11737);
#8688=LINE('',#50644,#11738);
#8689=LINE('',#50647,#11739);
#8690=LINE('',#50648,#11740);
#8691=LINE('',#50651,#11741);
#8692=LINE('',#50653,#11742);
#8693=LINE('',#50654,#11743);
#8694=LINE('',#50657,#11744);
#8695=LINE('',#50659,#11745);
#8696=LINE('',#50660,#11746);
#8697=LINE('',#50663,#11747);
#8698=LINE('',#50664,#11748);
#8699=LINE('',#50667,#11749);
#8700=LINE('',#50668,#11750);
#8701=LINE('',#50670,#11751);
#8702=LINE('',#50671,#11752);
#8703=LINE('',#50675,#11753);
#8704=LINE('',#50677,#11754);
#8705=LINE('',#50678,#11755);
#8706=LINE('',#50680,#11756);
#8707=LINE('',#50681,#11757);
#8708=LINE('',#50683,#11758);
#8709=LINE('',#50684,#11759);
#8710=LINE('',#50686,#11760);
#8711=LINE('',#50687,#11761);
#8712=LINE('',#50689,#11762);
#8713=LINE('',#50695,#11763);
#8714=LINE('',#50697,#11764);
#8715=LINE('',#50698,#11765);
#8716=LINE('',#50702,#11766);
#8717=LINE('',#50704,#11767);
#8718=LINE('',#50705,#11768);
#8719=LINE('',#50709,#11769);
#8720=LINE('',#50711,#11770);
#8721=LINE('',#50712,#11771);
#8722=LINE('',#50714,#11772);
#8723=LINE('',#50715,#11773);
#8724=LINE('',#50719,#11774);
#8725=LINE('',#50721,#11775);
#8726=LINE('',#50722,#11776);
#8727=LINE('',#50724,#11777);
#8728=LINE('',#50725,#11778);
#8729=LINE('',#50727,#11779);
#8730=LINE('',#50728,#11780);
#8731=LINE('',#50730,#11781);
#8732=LINE('',#50731,#11782);
#8733=LINE('',#50733,#11783);
#8734=LINE('',#50734,#11784);
#8735=LINE('',#50736,#11785);
#8736=LINE('',#50737,#11786);
#8737=LINE('',#50739,#11787);
#8738=LINE('',#50740,#11788);
#8739=LINE('',#50742,#11789);
#8740=LINE('',#50743,#11790);
#8741=LINE('',#50750,#11791);
#8742=LINE('',#50752,#11792);
#8743=LINE('',#50753,#11793);
#8744=LINE('',#50757,#11794);
#8745=LINE('',#50758,#11795);
#8746=LINE('',#50760,#11796);
#8747=LINE('',#50761,#11797);
#8748=LINE('',#50763,#11798);
#8749=LINE('',#50764,#11799);
#8750=LINE('',#50768,#11800);
#8751=LINE('',#50770,#11801);
#8752=LINE('',#50771,#11802);
#8753=LINE('',#50775,#11803);
#8754=LINE('',#50776,#11804);
#8755=LINE('',#50778,#11805);
#8756=LINE('',#50779,#11806);
#8757=LINE('',#50781,#11807);
#8758=LINE('',#50782,#11808);
#8759=LINE('',#50784,#11809);
#8760=LINE('',#50785,#11810);
#8761=LINE('',#50788,#11811);
#8762=LINE('',#50789,#11812);
#8763=LINE('',#50790,#11813);
#8764=LINE('',#50792,#11814);
#8765=LINE('',#50795,#11815);
#8766=LINE('',#50796,#11816);
#8767=LINE('',#50798,#11817);
#8768=LINE('',#50799,#11818);
#8769=LINE('',#50805,#11819);
#8770=LINE('',#50807,#11820);
#8771=LINE('',#50808,#11821);
#8772=LINE('',#50812,#11822);
#8773=LINE('',#50814,#11823);
#8774=LINE('',#50815,#11824);
#8775=LINE('',#50819,#11825);
#8776=LINE('',#50821,#11826);
#8777=LINE('',#50822,#11827);
#8778=LINE('',#50824,#11828);
#8779=LINE('',#50825,#11829);
#8780=LINE('',#50829,#11830);
#8781=LINE('',#50831,#11831);
#8782=LINE('',#50832,#11832);
#8783=LINE('',#50834,#11833);
#8784=LINE('',#50835,#11834);
#8785=LINE('',#50837,#11835);
#8786=LINE('',#50838,#11836);
#8787=LINE('',#50840,#11837);
#8788=LINE('',#50841,#11838);
#8789=LINE('',#50843,#11839);
#8790=LINE('',#50844,#11840);
#8791=LINE('',#50846,#11841);
#8792=LINE('',#50847,#11842);
#8793=LINE('',#50849,#11843);
#8794=LINE('',#50850,#11844);
#8795=LINE('',#50852,#11845);
#8796=LINE('',#50853,#11846);
#8797=LINE('',#50860,#11847);
#8798=LINE('',#50862,#11848);
#8799=LINE('',#50863,#11849);
#8800=LINE('',#50867,#11850);
#8801=LINE('',#50869,#11851);
#8802=LINE('',#50870,#11852);
#8803=LINE('',#50874,#11853);
#8804=LINE('',#50876,#11854);
#8805=LINE('',#50877,#11855);
#8806=LINE('',#50879,#11856);
#8807=LINE('',#50880,#11857);
#8808=LINE('',#50884,#11858);
#8809=LINE('',#50886,#11859);
#8810=LINE('',#50887,#11860);
#8811=LINE('',#50889,#11861);
#8812=LINE('',#50890,#11862);
#8813=LINE('',#50892,#11863);
#8814=LINE('',#50893,#11864);
#8815=LINE('',#50895,#11865);
#8816=LINE('',#50896,#11866);
#8817=LINE('',#50898,#11867);
#8818=LINE('',#50899,#11868);
#8819=LINE('',#50901,#11869);
#8820=LINE('',#50902,#11870);
#8821=LINE('',#50904,#11871);
#8822=LINE('',#50905,#11872);
#8823=LINE('',#50907,#11873);
#8824=LINE('',#50908,#11874);
#8825=LINE('',#50915,#11875);
#8826=LINE('',#50916,#11876);
#8827=LINE('',#50918,#11877);
#8828=LINE('',#50919,#11878);
#8829=LINE('',#50922,#11879);
#8830=LINE('',#50923,#11880);
#8831=LINE('',#50926,#11881);
#8832=LINE('',#50928,#11882);
#8833=LINE('',#50929,#11883);
#8834=LINE('',#50932,#11884);
#8835=LINE('',#50934,#11885);
#8836=LINE('',#50935,#11886);
#8837=LINE('',#50938,#11887);
#8838=LINE('',#50939,#11888);
#8839=LINE('',#50942,#11889);
#8840=LINE('',#50943,#11890);
#8841=LINE('',#50945,#11891);
#8842=LINE('',#50946,#11892);
#8843=LINE('',#50950,#11893);
#8844=LINE('',#50952,#11894);
#8845=LINE('',#50953,#11895);
#8846=LINE('',#50955,#11896);
#8847=LINE('',#50956,#11897);
#8848=LINE('',#50958,#11898);
#8849=LINE('',#50959,#11899);
#8850=LINE('',#50961,#11900);
#8851=LINE('',#50962,#11901);
#8852=LINE('',#50964,#11902);
#8853=LINE('',#50970,#11903);
#8854=LINE('',#50972,#11904);
#8855=LINE('',#50973,#11905);
#8856=LINE('',#50977,#11906);
#8857=LINE('',#50979,#11907);
#8858=LINE('',#50980,#11908);
#8859=LINE('',#50984,#11909);
#8860=LINE('',#50986,#11910);
#8861=LINE('',#50987,#11911);
#8862=LINE('',#50989,#11912);
#8863=LINE('',#50990,#11913);
#8864=LINE('',#50994,#11914);
#8865=LINE('',#50996,#11915);
#8866=LINE('',#50997,#11916);
#8867=LINE('',#50999,#11917);
#8868=LINE('',#51000,#11918);
#8869=LINE('',#51002,#11919);
#8870=LINE('',#51003,#11920);
#8871=LINE('',#51005,#11921);
#8872=LINE('',#51006,#11922);
#8873=LINE('',#51008,#11923);
#8874=LINE('',#51009,#11924);
#8875=LINE('',#51011,#11925);
#8876=LINE('',#51012,#11926);
#8877=LINE('',#51014,#11927);
#8878=LINE('',#51015,#11928);
#8879=LINE('',#51017,#11929);
#8880=LINE('',#51018,#11930);
#8881=LINE('',#51025,#11931);
#8882=LINE('',#51027,#11932);
#8883=LINE('',#51028,#11933);
#8884=LINE('',#51032,#11934);
#8885=LINE('',#51033,#11935);
#8886=LINE('',#51035,#11936);
#8887=LINE('',#51036,#11937);
#8888=LINE('',#51038,#11938);
#8889=LINE('',#51039,#11939);
#8890=LINE('',#51043,#11940);
#8891=LINE('',#51045,#11941);
#8892=LINE('',#51046,#11942);
#8893=LINE('',#51050,#11943);
#8894=LINE('',#51051,#11944);
#8895=LINE('',#51053,#11945);
#8896=LINE('',#51054,#11946);
#8897=LINE('',#51056,#11947);
#8898=LINE('',#51057,#11948);
#8899=LINE('',#51059,#11949);
#8900=LINE('',#51060,#11950);
#8901=LINE('',#51063,#11951);
#8902=LINE('',#51064,#11952);
#8903=LINE('',#51065,#11953);
#8904=LINE('',#51067,#11954);
#8905=LINE('',#51070,#11955);
#8906=LINE('',#51071,#11956);
#8907=LINE('',#51073,#11957);
#8908=LINE('',#51074,#11958);
#8909=LINE('',#51080,#11959);
#8910=LINE('',#51082,#11960);
#8911=LINE('',#51083,#11961);
#8912=LINE('',#51087,#11962);
#8913=LINE('',#51089,#11963);
#8914=LINE('',#51090,#11964);
#8915=LINE('',#51094,#11965);
#8916=LINE('',#51096,#11966);
#8917=LINE('',#51097,#11967);
#8918=LINE('',#51099,#11968);
#8919=LINE('',#51100,#11969);
#8920=LINE('',#51104,#11970);
#8921=LINE('',#51106,#11971);
#8922=LINE('',#51107,#11972);
#8923=LINE('',#51109,#11973);
#8924=LINE('',#51110,#11974);
#8925=LINE('',#51112,#11975);
#8926=LINE('',#51113,#11976);
#8927=LINE('',#51115,#11977);
#8928=LINE('',#51116,#11978);
#8929=LINE('',#51118,#11979);
#8930=LINE('',#51119,#11980);
#8931=LINE('',#51121,#11981);
#8932=LINE('',#51122,#11982);
#8933=LINE('',#51124,#11983);
#8934=LINE('',#51125,#11984);
#8935=LINE('',#51127,#11985);
#8936=LINE('',#51128,#11986);
#8937=LINE('',#51135,#11987);
#8938=LINE('',#51137,#11988);
#8939=LINE('',#51138,#11989);
#8940=LINE('',#51142,#11990);
#8941=LINE('',#51144,#11991);
#8942=LINE('',#51145,#11992);
#8943=LINE('',#51149,#11993);
#8944=LINE('',#51151,#11994);
#8945=LINE('',#51152,#11995);
#8946=LINE('',#51154,#11996);
#8947=LINE('',#51155,#11997);
#8948=LINE('',#51159,#11998);
#8949=LINE('',#51161,#11999);
#8950=LINE('',#51162,#12000);
#8951=LINE('',#51164,#12001);
#8952=LINE('',#51165,#12002);
#8953=LINE('',#51167,#12003);
#8954=LINE('',#51168,#12004);
#8955=LINE('',#51170,#12005);
#8956=LINE('',#51171,#12006);
#8957=LINE('',#51173,#12007);
#8958=LINE('',#51174,#12008);
#8959=LINE('',#51176,#12009);
#8960=LINE('',#51177,#12010);
#8961=LINE('',#51179,#12011);
#8962=LINE('',#51180,#12012);
#8963=LINE('',#51182,#12013);
#8964=LINE('',#51183,#12014);
#8965=LINE('',#51190,#12015);
#8966=LINE('',#51191,#12016);
#8967=LINE('',#51193,#12017);
#8968=LINE('',#51194,#12018);
#8969=LINE('',#51197,#12019);
#8970=LINE('',#51198,#12020);
#8971=LINE('',#51201,#12021);
#8972=LINE('',#51203,#12022);
#8973=LINE('',#51204,#12023);
#8974=LINE('',#51207,#12024);
#8975=LINE('',#51209,#12025);
#8976=LINE('',#51210,#12026);
#8977=LINE('',#51213,#12027);
#8978=LINE('',#51214,#12028);
#8979=LINE('',#51217,#12029);
#8980=LINE('',#51218,#12030);
#8981=LINE('',#51220,#12031);
#8982=LINE('',#51221,#12032);
#8983=LINE('',#51225,#12033);
#8984=LINE('',#51227,#12034);
#8985=LINE('',#51228,#12035);
#8986=LINE('',#51230,#12036);
#8987=LINE('',#51231,#12037);
#8988=LINE('',#51233,#12038);
#8989=LINE('',#51234,#12039);
#8990=LINE('',#51236,#12040);
#8991=LINE('',#51237,#12041);
#8992=LINE('',#51239,#12042);
#8993=LINE('',#51245,#12043);
#8994=LINE('',#51247,#12044);
#8995=LINE('',#51248,#12045);
#8996=LINE('',#51252,#12046);
#8997=LINE('',#51254,#12047);
#8998=LINE('',#51255,#12048);
#8999=LINE('',#51259,#12049);
#9000=LINE('',#51261,#12050);
#9001=LINE('',#51262,#12051);
#9002=LINE('',#51264,#12052);
#9003=LINE('',#51265,#12053);
#9004=LINE('',#51269,#12054);
#9005=LINE('',#51271,#12055);
#9006=LINE('',#51272,#12056);
#9007=LINE('',#51274,#12057);
#9008=LINE('',#51275,#12058);
#9009=LINE('',#51277,#12059);
#9010=LINE('',#51278,#12060);
#9011=LINE('',#51280,#12061);
#9012=LINE('',#51281,#12062);
#9013=LINE('',#51283,#12063);
#9014=LINE('',#51284,#12064);
#9015=LINE('',#51286,#12065);
#9016=LINE('',#51287,#12066);
#9017=LINE('',#51289,#12067);
#9018=LINE('',#51290,#12068);
#9019=LINE('',#51292,#12069);
#9020=LINE('',#51293,#12070);
#9021=LINE('',#51300,#12071);
#9022=LINE('',#51302,#12072);
#9023=LINE('',#51303,#12073);
#9024=LINE('',#51307,#12074);
#9025=LINE('',#51308,#12075);
#9026=LINE('',#51310,#12076);
#9027=LINE('',#51311,#12077);
#9028=LINE('',#51313,#12078);
#9029=LINE('',#51314,#12079);
#9030=LINE('',#51318,#12080);
#9031=LINE('',#51320,#12081);
#9032=LINE('',#51321,#12082);
#9033=LINE('',#51325,#12083);
#9034=LINE('',#51326,#12084);
#9035=LINE('',#51328,#12085);
#9036=LINE('',#51329,#12086);
#9037=LINE('',#51331,#12087);
#9038=LINE('',#51332,#12088);
#9039=LINE('',#51334,#12089);
#9040=LINE('',#51335,#12090);
#9041=LINE('',#51338,#12091);
#9042=LINE('',#51339,#12092);
#9043=LINE('',#51340,#12093);
#9044=LINE('',#51342,#12094);
#9045=LINE('',#51345,#12095);
#9046=LINE('',#51346,#12096);
#9047=LINE('',#51348,#12097);
#9048=LINE('',#51349,#12098);
#9049=LINE('',#51355,#12099);
#9050=LINE('',#51357,#12100);
#9051=LINE('',#51358,#12101);
#9052=LINE('',#51362,#12102);
#9053=LINE('',#51364,#12103);
#9054=LINE('',#51365,#12104);
#9055=LINE('',#51369,#12105);
#9056=LINE('',#51371,#12106);
#9057=LINE('',#51372,#12107);
#9058=LINE('',#51374,#12108);
#9059=LINE('',#51375,#12109);
#9060=LINE('',#51379,#12110);
#9061=LINE('',#51381,#12111);
#9062=LINE('',#51382,#12112);
#9063=LINE('',#51384,#12113);
#9064=LINE('',#51385,#12114);
#9065=LINE('',#51387,#12115);
#9066=LINE('',#51388,#12116);
#9067=LINE('',#51390,#12117);
#9068=LINE('',#51391,#12118);
#9069=LINE('',#51393,#12119);
#9070=LINE('',#51394,#12120);
#9071=LINE('',#51396,#12121);
#9072=LINE('',#51397,#12122);
#9073=LINE('',#51399,#12123);
#9074=LINE('',#51400,#12124);
#9075=LINE('',#51402,#12125);
#9076=LINE('',#51403,#12126);
#9077=LINE('',#51410,#12127);
#9078=LINE('',#51412,#12128);
#9079=LINE('',#51413,#12129);
#9080=LINE('',#51417,#12130);
#9081=LINE('',#51419,#12131);
#9082=LINE('',#51420,#12132);
#9083=LINE('',#51424,#12133);
#9084=LINE('',#51426,#12134);
#9085=LINE('',#51427,#12135);
#9086=LINE('',#51429,#12136);
#9087=LINE('',#51430,#12137);
#9088=LINE('',#51434,#12138);
#9089=LINE('',#51436,#12139);
#9090=LINE('',#51437,#12140);
#9091=LINE('',#51439,#12141);
#9092=LINE('',#51440,#12142);
#9093=LINE('',#51442,#12143);
#9094=LINE('',#51443,#12144);
#9095=LINE('',#51445,#12145);
#9096=LINE('',#51446,#12146);
#9097=LINE('',#51448,#12147);
#9098=LINE('',#51449,#12148);
#9099=LINE('',#51451,#12149);
#9100=LINE('',#51452,#12150);
#9101=LINE('',#51454,#12151);
#9102=LINE('',#51455,#12152);
#9103=LINE('',#51457,#12153);
#9104=LINE('',#51458,#12154);
#9105=LINE('',#51465,#12155);
#9106=LINE('',#51466,#12156);
#9107=LINE('',#51468,#12157);
#9108=LINE('',#51469,#12158);
#9109=LINE('',#51472,#12159);
#9110=LINE('',#51473,#12160);
#9111=LINE('',#51476,#12161);
#9112=LINE('',#51478,#12162);
#9113=LINE('',#51479,#12163);
#9114=LINE('',#51482,#12164);
#9115=LINE('',#51484,#12165);
#9116=LINE('',#51485,#12166);
#9117=LINE('',#51488,#12167);
#9118=LINE('',#51489,#12168);
#9119=LINE('',#51492,#12169);
#9120=LINE('',#51493,#12170);
#9121=LINE('',#51495,#12171);
#9122=LINE('',#51496,#12172);
#9123=LINE('',#51500,#12173);
#9124=LINE('',#51502,#12174);
#9125=LINE('',#51503,#12175);
#9126=LINE('',#51505,#12176);
#9127=LINE('',#51506,#12177);
#9128=LINE('',#51508,#12178);
#9129=LINE('',#51509,#12179);
#9130=LINE('',#51511,#12180);
#9131=LINE('',#51512,#12181);
#9132=LINE('',#51514,#12182);
#9133=LINE('',#51520,#12183);
#9134=LINE('',#51522,#12184);
#9135=LINE('',#51523,#12185);
#9136=LINE('',#51527,#12186);
#9137=LINE('',#51529,#12187);
#9138=LINE('',#51530,#12188);
#9139=LINE('',#51534,#12189);
#9140=LINE('',#51536,#12190);
#9141=LINE('',#51537,#12191);
#9142=LINE('',#51539,#12192);
#9143=LINE('',#51540,#12193);
#9144=LINE('',#51544,#12194);
#9145=LINE('',#51546,#12195);
#9146=LINE('',#51547,#12196);
#9147=LINE('',#51549,#12197);
#9148=LINE('',#51550,#12198);
#9149=LINE('',#51552,#12199);
#9150=LINE('',#51553,#12200);
#9151=LINE('',#51555,#12201);
#9152=LINE('',#51556,#12202);
#9153=LINE('',#51558,#12203);
#9154=LINE('',#51559,#12204);
#9155=LINE('',#51561,#12205);
#9156=LINE('',#51562,#12206);
#9157=LINE('',#51564,#12207);
#9158=LINE('',#51565,#12208);
#9159=LINE('',#51567,#12209);
#9160=LINE('',#51568,#12210);
#9161=LINE('',#51575,#12211);
#9162=LINE('',#51577,#12212);
#9163=LINE('',#51578,#12213);
#9164=LINE('',#51582,#12214);
#9165=LINE('',#51583,#12215);
#9166=LINE('',#51585,#12216);
#9167=LINE('',#51586,#12217);
#9168=LINE('',#51588,#12218);
#9169=LINE('',#51589,#12219);
#9170=LINE('',#51593,#12220);
#9171=LINE('',#51595,#12221);
#9172=LINE('',#51596,#12222);
#9173=LINE('',#51600,#12223);
#9174=LINE('',#51601,#12224);
#9175=LINE('',#51603,#12225);
#9176=LINE('',#51604,#12226);
#9177=LINE('',#51606,#12227);
#9178=LINE('',#51607,#12228);
#9179=LINE('',#51609,#12229);
#9180=LINE('',#51610,#12230);
#9181=LINE('',#51613,#12231);
#9182=LINE('',#51614,#12232);
#9183=LINE('',#51615,#12233);
#9184=LINE('',#51617,#12234);
#9185=LINE('',#51620,#12235);
#9186=LINE('',#51621,#12236);
#9187=LINE('',#51623,#12237);
#9188=LINE('',#51624,#12238);
#9189=LINE('',#51630,#12239);
#9190=LINE('',#51632,#12240);
#9191=LINE('',#51633,#12241);
#9192=LINE('',#51637,#12242);
#9193=LINE('',#51639,#12243);
#9194=LINE('',#51640,#12244);
#9195=LINE('',#51644,#12245);
#9196=LINE('',#51646,#12246);
#9197=LINE('',#51647,#12247);
#9198=LINE('',#51649,#12248);
#9199=LINE('',#51650,#12249);
#9200=LINE('',#51654,#12250);
#9201=LINE('',#51656,#12251);
#9202=LINE('',#51657,#12252);
#9203=LINE('',#51659,#12253);
#9204=LINE('',#51660,#12254);
#9205=LINE('',#51662,#12255);
#9206=LINE('',#51663,#12256);
#9207=LINE('',#51665,#12257);
#9208=LINE('',#51666,#12258);
#9209=LINE('',#51668,#12259);
#9210=LINE('',#51669,#12260);
#9211=LINE('',#51671,#12261);
#9212=LINE('',#51672,#12262);
#9213=LINE('',#51674,#12263);
#9214=LINE('',#51675,#12264);
#9215=LINE('',#51677,#12265);
#9216=LINE('',#51678,#12266);
#9217=LINE('',#51685,#12267);
#9218=LINE('',#51687,#12268);
#9219=LINE('',#51688,#12269);
#9220=LINE('',#51692,#12270);
#9221=LINE('',#51694,#12271);
#9222=LINE('',#51695,#12272);
#9223=LINE('',#51699,#12273);
#9224=LINE('',#51701,#12274);
#9225=LINE('',#51702,#12275);
#9226=LINE('',#51704,#12276);
#9227=LINE('',#51705,#12277);
#9228=LINE('',#51709,#12278);
#9229=LINE('',#51711,#12279);
#9230=LINE('',#51712,#12280);
#9231=LINE('',#51714,#12281);
#9232=LINE('',#51715,#12282);
#9233=LINE('',#51717,#12283);
#9234=LINE('',#51718,#12284);
#9235=LINE('',#51720,#12285);
#9236=LINE('',#51721,#12286);
#9237=LINE('',#51723,#12287);
#9238=LINE('',#51724,#12288);
#9239=LINE('',#51726,#12289);
#9240=LINE('',#51727,#12290);
#9241=LINE('',#51729,#12291);
#9242=LINE('',#51730,#12292);
#9243=LINE('',#51732,#12293);
#9244=LINE('',#51733,#12294);
#9245=LINE('',#51740,#12295);
#9246=LINE('',#51741,#12296);
#9247=LINE('',#51743,#12297);
#9248=LINE('',#51744,#12298);
#9249=LINE('',#51747,#12299);
#9250=LINE('',#51748,#12300);
#9251=LINE('',#51751,#12301);
#9252=LINE('',#51753,#12302);
#9253=LINE('',#51754,#12303);
#9254=LINE('',#51757,#12304);
#9255=LINE('',#51759,#12305);
#9256=LINE('',#51760,#12306);
#9257=LINE('',#51763,#12307);
#9258=LINE('',#51764,#12308);
#9259=LINE('',#51767,#12309);
#9260=LINE('',#51768,#12310);
#9261=LINE('',#51770,#12311);
#9262=LINE('',#51771,#12312);
#9263=LINE('',#51775,#12313);
#9264=LINE('',#51777,#12314);
#9265=LINE('',#51778,#12315);
#9266=LINE('',#51780,#12316);
#9267=LINE('',#51781,#12317);
#9268=LINE('',#51783,#12318);
#9269=LINE('',#51784,#12319);
#9270=LINE('',#51786,#12320);
#9271=LINE('',#51787,#12321);
#9272=LINE('',#51789,#12322);
#9273=LINE('',#51795,#12323);
#9274=LINE('',#51797,#12324);
#9275=LINE('',#51798,#12325);
#9276=LINE('',#51802,#12326);
#9277=LINE('',#51804,#12327);
#9278=LINE('',#51805,#12328);
#9279=LINE('',#51809,#12329);
#9280=LINE('',#51811,#12330);
#9281=LINE('',#51812,#12331);
#9282=LINE('',#51814,#12332);
#9283=LINE('',#51815,#12333);
#9284=LINE('',#51819,#12334);
#9285=LINE('',#51821,#12335);
#9286=LINE('',#51822,#12336);
#9287=LINE('',#51824,#12337);
#9288=LINE('',#51825,#12338);
#9289=LINE('',#51827,#12339);
#9290=LINE('',#51828,#12340);
#9291=LINE('',#51830,#12341);
#9292=LINE('',#51831,#12342);
#9293=LINE('',#51833,#12343);
#9294=LINE('',#51834,#12344);
#9295=LINE('',#51836,#12345);
#9296=LINE('',#51837,#12346);
#9297=LINE('',#51839,#12347);
#9298=LINE('',#51840,#12348);
#9299=LINE('',#51842,#12349);
#9300=LINE('',#51843,#12350);
#9301=LINE('',#51850,#12351);
#9302=LINE('',#51852,#12352);
#9303=LINE('',#51853,#12353);
#9304=LINE('',#51857,#12354);
#9305=LINE('',#51858,#12355);
#9306=LINE('',#51860,#12356);
#9307=LINE('',#51861,#12357);
#9308=LINE('',#51863,#12358);
#9309=LINE('',#51864,#12359);
#9310=LINE('',#51868,#12360);
#9311=LINE('',#51870,#12361);
#9312=LINE('',#51871,#12362);
#9313=LINE('',#51875,#12363);
#9314=LINE('',#51876,#12364);
#9315=LINE('',#51878,#12365);
#9316=LINE('',#51879,#12366);
#9317=LINE('',#51881,#12367);
#9318=LINE('',#51882,#12368);
#9319=LINE('',#51884,#12369);
#9320=LINE('',#51885,#12370);
#9321=LINE('',#51888,#12371);
#9322=LINE('',#51889,#12372);
#9323=LINE('',#51890,#12373);
#9324=LINE('',#51892,#12374);
#9325=LINE('',#51895,#12375);
#9326=LINE('',#51896,#12376);
#9327=LINE('',#51898,#12377);
#9328=LINE('',#51899,#12378);
#9329=LINE('',#51905,#12379);
#9330=LINE('',#51907,#12380);
#9331=LINE('',#51908,#12381);
#9332=LINE('',#51912,#12382);
#9333=LINE('',#51914,#12383);
#9334=LINE('',#51915,#12384);
#9335=LINE('',#51919,#12385);
#9336=LINE('',#51921,#12386);
#9337=LINE('',#51922,#12387);
#9338=LINE('',#51924,#12388);
#9339=LINE('',#51925,#12389);
#9340=LINE('',#51929,#12390);
#9341=LINE('',#51931,#12391);
#9342=LINE('',#51932,#12392);
#9343=LINE('',#51934,#12393);
#9344=LINE('',#51935,#12394);
#9345=LINE('',#51937,#12395);
#9346=LINE('',#51938,#12396);
#9347=LINE('',#51940,#12397);
#9348=LINE('',#51941,#12398);
#9349=LINE('',#51943,#12399);
#9350=LINE('',#51944,#12400);
#9351=LINE('',#51946,#12401);
#9352=LINE('',#51947,#12402);
#9353=LINE('',#51949,#12403);
#9354=LINE('',#51950,#12404);
#9355=LINE('',#51952,#12405);
#9356=LINE('',#51953,#12406);
#9357=LINE('',#51960,#12407);
#9358=LINE('',#51962,#12408);
#9359=LINE('',#51963,#12409);
#9360=LINE('',#51967,#12410);
#9361=LINE('',#51969,#12411);
#9362=LINE('',#51970,#12412);
#9363=LINE('',#51974,#12413);
#9364=LINE('',#51976,#12414);
#9365=LINE('',#51977,#12415);
#9366=LINE('',#51979,#12416);
#9367=LINE('',#51980,#12417);
#9368=LINE('',#51984,#12418);
#9369=LINE('',#51986,#12419);
#9370=LINE('',#51987,#12420);
#9371=LINE('',#51989,#12421);
#9372=LINE('',#51990,#12422);
#9373=LINE('',#51992,#12423);
#9374=LINE('',#51993,#12424);
#9375=LINE('',#51995,#12425);
#9376=LINE('',#51996,#12426);
#9377=LINE('',#51998,#12427);
#9378=LINE('',#51999,#12428);
#9379=LINE('',#52001,#12429);
#9380=LINE('',#52002,#12430);
#9381=LINE('',#52004,#12431);
#9382=LINE('',#52005,#12432);
#9383=LINE('',#52007,#12433);
#9384=LINE('',#52008,#12434);
#9385=LINE('',#52015,#12435);
#9386=LINE('',#52016,#12436);
#9387=LINE('',#52018,#12437);
#9388=LINE('',#52019,#12438);
#9389=LINE('',#52022,#12439);
#9390=LINE('',#52023,#12440);
#9391=LINE('',#52026,#12441);
#9392=LINE('',#52028,#12442);
#9393=LINE('',#52029,#12443);
#9394=LINE('',#52032,#12444);
#9395=LINE('',#52034,#12445);
#9396=LINE('',#52035,#12446);
#9397=LINE('',#52038,#12447);
#9398=LINE('',#52039,#12448);
#9399=LINE('',#52042,#12449);
#9400=LINE('',#52043,#12450);
#9401=LINE('',#52045,#12451);
#9402=LINE('',#52046,#12452);
#9403=LINE('',#52050,#12453);
#9404=LINE('',#52052,#12454);
#9405=LINE('',#52053,#12455);
#9406=LINE('',#52055,#12456);
#9407=LINE('',#52056,#12457);
#9408=LINE('',#52058,#12458);
#9409=LINE('',#52059,#12459);
#9410=LINE('',#52061,#12460);
#9411=LINE('',#52062,#12461);
#9412=LINE('',#52064,#12462);
#9413=LINE('',#52070,#12463);
#9414=LINE('',#52072,#12464);
#9415=LINE('',#52073,#12465);
#9416=LINE('',#52077,#12466);
#9417=LINE('',#52079,#12467);
#9418=LINE('',#52080,#12468);
#9419=LINE('',#52084,#12469);
#9420=LINE('',#52086,#12470);
#9421=LINE('',#52087,#12471);
#9422=LINE('',#52089,#12472);
#9423=LINE('',#52090,#12473);
#9424=LINE('',#52094,#12474);
#9425=LINE('',#52096,#12475);
#9426=LINE('',#52097,#12476);
#9427=LINE('',#52099,#12477);
#9428=LINE('',#52100,#12478);
#9429=LINE('',#52102,#12479);
#9430=LINE('',#52103,#12480);
#9431=LINE('',#52105,#12481);
#9432=LINE('',#52106,#12482);
#9433=LINE('',#52108,#12483);
#9434=LINE('',#52109,#12484);
#9435=LINE('',#52111,#12485);
#9436=LINE('',#52112,#12486);
#9437=LINE('',#52114,#12487);
#9438=LINE('',#52115,#12488);
#9439=LINE('',#52117,#12489);
#9440=LINE('',#52118,#12490);
#9441=LINE('',#52125,#12491);
#9442=LINE('',#52127,#12492);
#9443=LINE('',#52128,#12493);
#9444=LINE('',#52132,#12494);
#9445=LINE('',#52133,#12495);
#9446=LINE('',#52135,#12496);
#9447=LINE('',#52136,#12497);
#9448=LINE('',#52138,#12498);
#9449=LINE('',#52139,#12499);
#9450=LINE('',#52143,#12500);
#9451=LINE('',#52145,#12501);
#9452=LINE('',#52146,#12502);
#9453=LINE('',#52150,#12503);
#9454=LINE('',#52151,#12504);
#9455=LINE('',#52153,#12505);
#9456=LINE('',#52154,#12506);
#9457=LINE('',#52156,#12507);
#9458=LINE('',#52157,#12508);
#9459=LINE('',#52159,#12509);
#9460=LINE('',#52160,#12510);
#9461=LINE('',#52163,#12511);
#9462=LINE('',#52164,#12512);
#9463=LINE('',#52165,#12513);
#9464=LINE('',#52167,#12514);
#9465=LINE('',#52170,#12515);
#9466=LINE('',#52171,#12516);
#9467=LINE('',#52173,#12517);
#9468=LINE('',#52174,#12518);
#9469=LINE('',#52180,#12519);
#9470=LINE('',#52182,#12520);
#9471=LINE('',#52183,#12521);
#9472=LINE('',#52187,#12522);
#9473=LINE('',#52189,#12523);
#9474=LINE('',#52190,#12524);
#9475=LINE('',#52194,#12525);
#9476=LINE('',#52196,#12526);
#9477=LINE('',#52197,#12527);
#9478=LINE('',#52199,#12528);
#9479=LINE('',#52200,#12529);
#9480=LINE('',#52204,#12530);
#9481=LINE('',#52206,#12531);
#9482=LINE('',#52207,#12532);
#9483=LINE('',#52209,#12533);
#9484=LINE('',#52210,#12534);
#9485=LINE('',#52212,#12535);
#9486=LINE('',#52213,#12536);
#9487=LINE('',#52215,#12537);
#9488=LINE('',#52216,#12538);
#9489=LINE('',#52218,#12539);
#9490=LINE('',#52219,#12540);
#9491=LINE('',#52221,#12541);
#9492=LINE('',#52222,#12542);
#9493=LINE('',#52224,#12543);
#9494=LINE('',#52225,#12544);
#9495=LINE('',#52227,#12545);
#9496=LINE('',#52228,#12546);
#9497=LINE('',#52235,#12547);
#9498=LINE('',#52237,#12548);
#9499=LINE('',#52238,#12549);
#9500=LINE('',#52242,#12550);
#9501=LINE('',#52244,#12551);
#9502=LINE('',#52245,#12552);
#9503=LINE('',#52249,#12553);
#9504=LINE('',#52251,#12554);
#9505=LINE('',#52252,#12555);
#9506=LINE('',#52254,#12556);
#9507=LINE('',#52255,#12557);
#9508=LINE('',#52259,#12558);
#9509=LINE('',#52261,#12559);
#9510=LINE('',#52262,#12560);
#9511=LINE('',#52264,#12561);
#9512=LINE('',#52265,#12562);
#9513=LINE('',#52267,#12563);
#9514=LINE('',#52268,#12564);
#9515=LINE('',#52270,#12565);
#9516=LINE('',#52271,#12566);
#9517=LINE('',#52273,#12567);
#9518=LINE('',#52274,#12568);
#9519=LINE('',#52276,#12569);
#9520=LINE('',#52277,#12570);
#9521=LINE('',#52279,#12571);
#9522=LINE('',#52280,#12572);
#9523=LINE('',#52282,#12573);
#9524=LINE('',#52283,#12574);
#9525=LINE('',#52290,#12575);
#9526=LINE('',#52291,#12576);
#9527=LINE('',#52293,#12577);
#9528=LINE('',#52294,#12578);
#9529=LINE('',#52297,#12579);
#9530=LINE('',#52298,#12580);
#9531=LINE('',#52301,#12581);
#9532=LINE('',#52303,#12582);
#9533=LINE('',#52304,#12583);
#9534=LINE('',#52307,#12584);
#9535=LINE('',#52309,#12585);
#9536=LINE('',#52310,#12586);
#9537=LINE('',#52313,#12587);
#9538=LINE('',#52314,#12588);
#9539=LINE('',#52317,#12589);
#9540=LINE('',#52318,#12590);
#9541=LINE('',#52320,#12591);
#9542=LINE('',#52321,#12592);
#9543=LINE('',#52325,#12593);
#9544=LINE('',#52327,#12594);
#9545=LINE('',#52328,#12595);
#9546=LINE('',#52330,#12596);
#9547=LINE('',#52331,#12597);
#9548=LINE('',#52333,#12598);
#9549=LINE('',#52334,#12599);
#9550=LINE('',#52336,#12600);
#9551=LINE('',#52337,#12601);
#9552=LINE('',#52339,#12602);
#9553=LINE('',#52345,#12603);
#9554=LINE('',#52347,#12604);
#9555=LINE('',#52348,#12605);
#9556=LINE('',#52352,#12606);
#9557=LINE('',#52354,#12607);
#9558=LINE('',#52355,#12608);
#9559=LINE('',#52359,#12609);
#9560=LINE('',#52361,#12610);
#9561=LINE('',#52362,#12611);
#9562=LINE('',#52364,#12612);
#9563=LINE('',#52365,#12613);
#9564=LINE('',#52369,#12614);
#9565=LINE('',#52371,#12615);
#9566=LINE('',#52372,#12616);
#9567=LINE('',#52374,#12617);
#9568=LINE('',#52375,#12618);
#9569=LINE('',#52377,#12619);
#9570=LINE('',#52378,#12620);
#9571=LINE('',#52380,#12621);
#9572=LINE('',#52381,#12622);
#9573=LINE('',#52383,#12623);
#9574=LINE('',#52384,#12624);
#9575=LINE('',#52386,#12625);
#9576=LINE('',#52387,#12626);
#9577=LINE('',#52389,#12627);
#9578=LINE('',#52390,#12628);
#9579=LINE('',#52392,#12629);
#9580=LINE('',#52393,#12630);
#9581=LINE('',#52400,#12631);
#9582=LINE('',#52402,#12632);
#9583=LINE('',#52403,#12633);
#9584=LINE('',#52407,#12634);
#9585=LINE('',#52408,#12635);
#9586=LINE('',#52410,#12636);
#9587=LINE('',#52411,#12637);
#9588=LINE('',#52413,#12638);
#9589=LINE('',#52414,#12639);
#9590=LINE('',#52418,#12640);
#9591=LINE('',#52420,#12641);
#9592=LINE('',#52421,#12642);
#9593=LINE('',#52425,#12643);
#9594=LINE('',#52426,#12644);
#9595=LINE('',#52428,#12645);
#9596=LINE('',#52429,#12646);
#9597=LINE('',#52431,#12647);
#9598=LINE('',#52432,#12648);
#9599=LINE('',#52434,#12649);
#9600=LINE('',#52435,#12650);
#9601=LINE('',#52438,#12651);
#9602=LINE('',#52439,#12652);
#9603=LINE('',#52440,#12653);
#9604=LINE('',#52442,#12654);
#9605=LINE('',#52445,#12655);
#9606=LINE('',#52446,#12656);
#9607=LINE('',#52448,#12657);
#9608=LINE('',#52449,#12658);
#9609=LINE('',#52455,#12659);
#9610=LINE('',#52457,#12660);
#9611=LINE('',#52458,#12661);
#9612=LINE('',#52462,#12662);
#9613=LINE('',#52464,#12663);
#9614=LINE('',#52465,#12664);
#9615=LINE('',#52469,#12665);
#9616=LINE('',#52471,#12666);
#9617=LINE('',#52472,#12667);
#9618=LINE('',#52474,#12668);
#9619=LINE('',#52475,#12669);
#9620=LINE('',#52479,#12670);
#9621=LINE('',#52481,#12671);
#9622=LINE('',#52482,#12672);
#9623=LINE('',#52484,#12673);
#9624=LINE('',#52485,#12674);
#9625=LINE('',#52487,#12675);
#9626=LINE('',#52488,#12676);
#9627=LINE('',#52490,#12677);
#9628=LINE('',#52491,#12678);
#9629=LINE('',#52493,#12679);
#9630=LINE('',#52494,#12680);
#9631=LINE('',#52496,#12681);
#9632=LINE('',#52497,#12682);
#9633=LINE('',#52499,#12683);
#9634=LINE('',#52500,#12684);
#9635=LINE('',#52502,#12685);
#9636=LINE('',#52503,#12686);
#9637=LINE('',#52510,#12687);
#9638=LINE('',#52512,#12688);
#9639=LINE('',#52513,#12689);
#9640=LINE('',#52517,#12690);
#9641=LINE('',#52519,#12691);
#9642=LINE('',#52520,#12692);
#9643=LINE('',#52524,#12693);
#9644=LINE('',#52526,#12694);
#9645=LINE('',#52527,#12695);
#9646=LINE('',#52529,#12696);
#9647=LINE('',#52530,#12697);
#9648=LINE('',#52534,#12698);
#9649=LINE('',#52536,#12699);
#9650=LINE('',#52537,#12700);
#9651=LINE('',#52539,#12701);
#9652=LINE('',#52540,#12702);
#9653=LINE('',#52542,#12703);
#9654=LINE('',#52543,#12704);
#9655=LINE('',#52545,#12705);
#9656=LINE('',#52546,#12706);
#9657=LINE('',#52548,#12707);
#9658=LINE('',#52549,#12708);
#9659=LINE('',#52551,#12709);
#9660=LINE('',#52552,#12710);
#9661=LINE('',#52554,#12711);
#9662=LINE('',#52555,#12712);
#9663=LINE('',#52557,#12713);
#9664=LINE('',#52558,#12714);
#9665=LINE('',#52568,#12715);
#9666=LINE('',#52574,#12716);
#9667=LINE('',#52581,#12717);
#9668=LINE('',#52585,#12718);
#9669=LINE('',#52587,#12719);
#9670=LINE('',#52588,#12720);
#9671=LINE('',#52592,#12721);
#9672=LINE('',#52594,#12722);
#9673=LINE('',#52595,#12723);
#9674=LINE('',#52599,#12724);
#9675=LINE('',#52601,#12725);
#9676=LINE('',#52602,#12726);
#9677=LINE('',#52604,#12727);
#9678=LINE('',#52605,#12728);
#9679=LINE('',#52609,#12729);
#9680=LINE('',#52611,#12730);
#9681=LINE('',#52612,#12731);
#9682=LINE('',#52614,#12732);
#9683=LINE('',#52615,#12733);
#9684=LINE('',#52617,#12734);
#9685=LINE('',#52618,#12735);
#9686=LINE('',#52620,#12736);
#9687=LINE('',#52621,#12737);
#9688=LINE('',#52623,#12738);
#9689=LINE('',#52624,#12739);
#9690=LINE('',#52626,#12740);
#9691=LINE('',#52627,#12741);
#9692=LINE('',#52629,#12742);
#9693=LINE('',#52630,#12743);
#9694=LINE('',#52632,#12744);
#9695=LINE('',#52633,#12745);
#9696=LINE('',#52640,#12746);
#9697=LINE('',#52642,#12747);
#9698=LINE('',#52643,#12748);
#9699=LINE('',#52647,#12749);
#9700=LINE('',#52649,#12750);
#9701=LINE('',#52650,#12751);
#9702=LINE('',#52654,#12752);
#9703=LINE('',#52656,#12753);
#9704=LINE('',#52657,#12754);
#9705=LINE('',#52659,#12755);
#9706=LINE('',#52660,#12756);
#9707=LINE('',#52664,#12757);
#9708=LINE('',#52666,#12758);
#9709=LINE('',#52667,#12759);
#9710=LINE('',#52669,#12760);
#9711=LINE('',#52670,#12761);
#9712=LINE('',#52672,#12762);
#9713=LINE('',#52673,#12763);
#9714=LINE('',#52675,#12764);
#9715=LINE('',#52676,#12765);
#9716=LINE('',#52678,#12766);
#9717=LINE('',#52679,#12767);
#9718=LINE('',#52681,#12768);
#9719=LINE('',#52682,#12769);
#9720=LINE('',#52684,#12770);
#9721=LINE('',#52685,#12771);
#9722=LINE('',#52687,#12772);
#9723=LINE('',#52688,#12773);
#9724=LINE('',#52698,#12774);
#9725=LINE('',#52704,#12775);
#9726=LINE('',#52709,#12776);
#9727=LINE('',#52713,#12777);
#9728=LINE('',#52720,#12778);
#9729=LINE('',#52723,#12779);
#9730=LINE('',#52726,#12780);
#9731=LINE('',#52873,#12781);
#9732=LINE('',#52877,#12782);
#9733=LINE('',#52881,#12783);
#9734=LINE('',#52885,#12784);
#9735=LINE('',#52889,#12785);
#9736=LINE('',#52895,#12786);
#9737=LINE('',#52899,#12787);
#9738=LINE('',#52903,#12788);
#9739=LINE('',#52907,#12789);
#9740=LINE('',#52911,#12790);
#9741=LINE('',#52918,#12791);
#9742=LINE('',#52923,#12792);
#9743=LINE('',#52928,#12793);
#9744=LINE('',#52935,#12794);
#9745=LINE('',#52938,#12795);
#9746=LINE('',#52942,#12796);
#9747=LINE('',#52948,#12797);
#9748=LINE('',#52951,#12798);
#10584=VECTOR('',#37671,39.77639320225);
#10585=VECTOR('',#37678,38.5);
#10586=VECTOR('',#37687,40.);
#10587=VECTOR('',#37690,36.97360679775);
#10588=VECTOR('',#37701,26.25);
#10589=VECTOR('',#37710,26.);
#10590=VECTOR('',#37719,31.9267766952966);
#10591=VECTOR('',#37726,33.);
#10592=VECTOR('',#37737,33.8502380998955);
#10593=VECTOR('',#37744,35.25);
#10594=VECTOR('',#37753,126.961414092626);
#10595=VECTOR('',#37760,129.25);
#10596=VECTOR('',#37769,124.);
#10597=VECTOR('',#37772,131.441987426416);
#10598=VECTOR('',#37779,133.);
#10599=VECTOR('',#37786,134.437780860397);
#10600=VECTOR('',#37793,135.25);
#10601=VECTOR('',#37800,135.912219139603);
#10602=VECTOR('',#37807,136.);
#10603=VECTOR('',#37812,10.);
#10604=VECTOR('',#37817,136.);
#10605=VECTOR('',#37824,10.);
#10606=VECTOR('',#37829,10.);
#10607=VECTOR('',#37836,10.);
#10608=VECTOR('',#37843,10.);
#10609=VECTOR('',#37850,10.);
#10610=VECTOR('',#37857,10.);
#10611=VECTOR('',#37864,10.);
#10612=VECTOR('',#37871,10.);
#10613=VECTOR('',#37878,10.);
#10614=VECTOR('',#37885,10.);
#10615=VECTOR('',#37892,10.);
#10616=VECTOR('',#37899,10.);
#10617=VECTOR('',#37906,10.);
#10618=VECTOR('',#37913,10.);
#10619=VECTOR('',#37920,10.);
#10620=VECTOR('',#37927,10.);
#10621=VECTOR('',#37934,10.);
#10622=VECTOR('',#37941,10.);
#10623=VECTOR('',#37948,10.);
#10624=VECTOR('',#37955,10.);
#10625=VECTOR('',#37962,10.);
#10626=VECTOR('',#37969,10.);
#10627=VECTOR('',#37976,10.);
#10628=VECTOR('',#37983,10.);
#10629=VECTOR('',#37990,10.);
#10630=VECTOR('',#37997,10.);
#10631=VECTOR('',#38004,10.);
#10632=VECTOR('',#38011,10.);
#10633=VECTOR('',#38018,10.);
#10634=VECTOR('',#38025,10.);
#10635=VECTOR('',#38032,10.);
#10636=VECTOR('',#38039,10.);
#10637=VECTOR('',#38046,10.);
#10638=VECTOR('',#38053,10.);
#10639=VECTOR('',#38060,10.);
#10640=VECTOR('',#38067,10.);
#10641=VECTOR('',#38074,10.);
#10642=VECTOR('',#38081,10.);
#10643=VECTOR('',#38088,10.);
#10644=VECTOR('',#38095,10.);
#10645=VECTOR('',#38102,10.);
#10646=VECTOR('',#38109,10.);
#10647=VECTOR('',#38116,10.);
#10648=VECTOR('',#38123,10.);
#10649=VECTOR('',#38130,10.);
#10650=VECTOR('',#38137,10.);
#10651=VECTOR('',#38144,10.);
#10652=VECTOR('',#38151,10.);
#10653=VECTOR('',#38158,10.);
#10654=VECTOR('',#38165,10.);
#10655=VECTOR('',#38172,10.);
#10656=VECTOR('',#38179,10.);
#10657=VECTOR('',#38186,10.);
#10658=VECTOR('',#38193,10.);
#10659=VECTOR('',#38200,10.);
#10660=VECTOR('',#38207,10.);
#10661=VECTOR('',#38214,10.);
#10662=VECTOR('',#38221,10.);
#10663=VECTOR('',#38228,10.);
#10664=VECTOR('',#38235,10.);
#10665=VECTOR('',#38242,10.);
#10666=VECTOR('',#38249,10.);
#10667=VECTOR('',#38256,10.);
#10668=VECTOR('',#38263,10.);
#10669=VECTOR('',#38270,10.);
#10670=VECTOR('',#38277,10.);
#10671=VECTOR('',#38284,10.);
#10672=VECTOR('',#38291,10.);
#10673=VECTOR('',#38298,10.);
#10674=VECTOR('',#38305,10.);
#10675=VECTOR('',#38312,10.);
#10676=VECTOR('',#38319,10.);
#10677=VECTOR('',#38326,10.);
#10678=VECTOR('',#38333,10.);
#10679=VECTOR('',#38340,10.);
#10680=VECTOR('',#38347,10.);
#10681=VECTOR('',#38354,10.);
#10682=VECTOR('',#38361,10.);
#10683=VECTOR('',#38368,10.);
#10684=VECTOR('',#38375,10.);
#10685=VECTOR('',#38382,10.);
#10686=VECTOR('',#38389,10.);
#10687=VECTOR('',#38396,10.);
#10688=VECTOR('',#38403,10.);
#10689=VECTOR('',#38410,10.);
#10690=VECTOR('',#38417,10.);
#10691=VECTOR('',#38424,10.);
#10692=VECTOR('',#38431,10.);
#10693=VECTOR('',#38438,10.);
#10694=VECTOR('',#38445,10.);
#10695=VECTOR('',#38452,10.);
#10696=VECTOR('',#38459,10.);
#10697=VECTOR('',#38466,10.);
#10698=VECTOR('',#38473,10.);
#10699=VECTOR('',#38480,10.);
#10700=VECTOR('',#38487,10.);
#10701=VECTOR('',#38494,10.);
#10702=VECTOR('',#38501,10.);
#10703=VECTOR('',#38508,10.);
#10704=VECTOR('',#38515,10.);
#10705=VECTOR('',#38522,10.);
#10706=VECTOR('',#38529,10.);
#10707=VECTOR('',#38536,10.);
#10708=VECTOR('',#38543,10.);
#10709=VECTOR('',#38550,10.);
#10710=VECTOR('',#38557,10.);
#10711=VECTOR('',#38564,10.);
#10712=VECTOR('',#38571,10.);
#10713=VECTOR('',#38578,10.);
#10714=VECTOR('',#38585,10.);
#10715=VECTOR('',#38592,10.);
#10716=VECTOR('',#38599,10.);
#10717=VECTOR('',#38606,10.);
#10718=VECTOR('',#38613,10.);
#10719=VECTOR('',#38620,10.);
#10720=VECTOR('',#38627,10.);
#10721=VECTOR('',#38634,10.);
#10722=VECTOR('',#38641,10.);
#10723=VECTOR('',#38648,10.);
#10724=VECTOR('',#38655,10.);
#10725=VECTOR('',#38662,10.);
#10726=VECTOR('',#38669,10.);
#10727=VECTOR('',#38676,10.);
#10728=VECTOR('',#38683,10.);
#10729=VECTOR('',#38690,10.);
#10730=VECTOR('',#38697,10.);
#10731=VECTOR('',#38704,10.);
#10732=VECTOR('',#38711,10.);
#10733=VECTOR('',#38718,10.);
#10734=VECTOR('',#38725,10.);
#10735=VECTOR('',#38732,10.);
#10736=VECTOR('',#38739,10.);
#10737=VECTOR('',#38746,10.);
#10738=VECTOR('',#38753,10.);
#10739=VECTOR('',#38760,10.);
#10740=VECTOR('',#38767,10.);
#10741=VECTOR('',#38774,10.);
#10742=VECTOR('',#38781,10.);
#10743=VECTOR('',#38788,10.);
#10744=VECTOR('',#38795,10.);
#10745=VECTOR('',#38802,10.);
#10746=VECTOR('',#38809,10.);
#10747=VECTOR('',#38816,10.);
#10748=VECTOR('',#38885,10.);
#10749=VECTOR('',#38888,10.);
#10750=VECTOR('',#38891,10.);
#10751=VECTOR('',#38896,10.);
#10752=VECTOR('',#38901,10.);
#10753=VECTOR('',#38906,10.);
#10754=VECTOR('',#38911,10.);
#10755=VECTOR('',#38928,10.);
#10756=VECTOR('',#38929,10.);
#10757=VECTOR('',#38930,10.);
#10758=VECTOR('',#38931,10.);
#10759=VECTOR('',#38934,10.);
#10760=VECTOR('',#38935,10.);
#10761=VECTOR('',#38938,10.);
#10762=VECTOR('',#38939,10.);
#10763=VECTOR('',#38940,10.);
#10764=VECTOR('',#38943,10.);
#10765=VECTOR('',#38944,10.);
#10766=VECTOR('',#38945,10.);
#10767=VECTOR('',#38948,10.);
#10768=VECTOR('',#38949,10.);
#10769=VECTOR('',#38952,10.);
#10770=VECTOR('',#38953,10.);
#10771=VECTOR('',#38956,10.);
#10772=VECTOR('',#38957,10.);
#10773=VECTOR('',#38960,10.);
#10774=VECTOR('',#38961,10.);
#10775=VECTOR('',#38962,10.);
#10776=VECTOR('',#38965,10.);
#10777=VECTOR('',#38966,10.);
#10778=VECTOR('',#38969,10.);
#10779=VECTOR('',#38970,10.);
#10780=VECTOR('',#38973,10.);
#10781=VECTOR('',#38974,10.);
#10782=VECTOR('',#38977,10.);
#10783=VECTOR('',#38984,10.);
#10784=VECTOR('',#38985,10.);
#10785=VECTOR('',#38986,10.);
#10786=VECTOR('',#38989,10.);
#10787=VECTOR('',#38990,10.);
#10788=VECTOR('',#38991,10.);
#10789=VECTOR('',#38994,10.);
#10790=VECTOR('',#38995,10.);
#10791=VECTOR('',#38996,10.);
#10792=VECTOR('',#38999,10.);
#10793=VECTOR('',#39000,10.);
#10794=VECTOR('',#39003,10.);
#10795=VECTOR('',#39004,10.);
#10796=VECTOR('',#39005,10.);
#10797=VECTOR('',#39008,10.);
#10798=VECTOR('',#39009,10.);
#10799=VECTOR('',#39012,10.);
#10800=VECTOR('',#39013,10.);
#10801=VECTOR('',#39016,10.);
#10802=VECTOR('',#39017,10.);
#10803=VECTOR('',#39020,10.);
#10804=VECTOR('',#39021,10.);
#10805=VECTOR('',#39024,10.);
#10806=VECTOR('',#39025,10.);
#10807=VECTOR('',#39028,10.);
#10808=VECTOR('',#39029,10.);
#10809=VECTOR('',#39032,10.);
#10810=VECTOR('',#39033,10.);
#10811=VECTOR('',#39042,10.);
#10812=VECTOR('',#39043,10.);
#10813=VECTOR('',#39044,10.);
#10814=VECTOR('',#39047,10.);
#10815=VECTOR('',#39048,10.);
#10816=VECTOR('',#39049,10.);
#10817=VECTOR('',#39050,10.);
#10818=VECTOR('',#39053,10.);
#10819=VECTOR('',#39054,10.);
#10820=VECTOR('',#39057,10.);
#10821=VECTOR('',#39058,10.);
#10822=VECTOR('',#39059,10.);
#10823=VECTOR('',#39062,10.);
#10824=VECTOR('',#39063,10.);
#10825=VECTOR('',#39064,10.);
#10826=VECTOR('',#39065,10.);
#10827=VECTOR('',#39068,10.);
#10828=VECTOR('',#39069,10.);
#10829=VECTOR('',#39072,10.);
#10830=VECTOR('',#39073,10.);
#10831=VECTOR('',#39076,10.);
#10832=VECTOR('',#39077,10.);
#10833=VECTOR('',#39078,10.);
#10834=VECTOR('',#39081,10.);
#10835=VECTOR('',#39084,10.);
#10836=VECTOR('',#39085,10.);
#10837=VECTOR('',#39088,10.);
#10838=VECTOR('',#39089,10.);
#10839=VECTOR('',#39096,10.);
#10840=VECTOR('',#39097,10.);
#10841=VECTOR('',#39098,10.);
#10842=VECTOR('',#39101,10.);
#10843=VECTOR('',#39102,10.);
#10844=VECTOR('',#39103,10.);
#10845=VECTOR('',#39106,10.);
#10846=VECTOR('',#39107,10.);
#10847=VECTOR('',#39108,10.);
#10848=VECTOR('',#39111,10.);
#10849=VECTOR('',#39112,10.);
#10850=VECTOR('',#39115,10.);
#10851=VECTOR('',#39116,10.);
#10852=VECTOR('',#39117,10.);
#10853=VECTOR('',#39120,10.);
#10854=VECTOR('',#39121,10.);
#10855=VECTOR('',#39124,10.);
#10856=VECTOR('',#39125,10.);
#10857=VECTOR('',#39128,10.);
#10858=VECTOR('',#39129,10.);
#10859=VECTOR('',#39132,10.);
#10860=VECTOR('',#39133,10.);
#10861=VECTOR('',#39136,10.);
#10862=VECTOR('',#39137,10.);
#10863=VECTOR('',#39140,10.);
#10864=VECTOR('',#39141,10.);
#10865=VECTOR('',#39144,10.);
#10866=VECTOR('',#39145,10.);
#10867=VECTOR('',#39154,10.);
#10868=VECTOR('',#39155,10.);
#10869=VECTOR('',#39156,10.);
#10870=VECTOR('',#39159,10.);
#10871=VECTOR('',#39160,10.);
#10872=VECTOR('',#39161,10.);
#10873=VECTOR('',#39164,10.);
#10874=VECTOR('',#39165,10.);
#10875=VECTOR('',#39166,10.);
#10876=VECTOR('',#39169,10.);
#10877=VECTOR('',#39170,10.);
#10878=VECTOR('',#39173,10.);
#10879=VECTOR('',#39174,10.);
#10880=VECTOR('',#39175,10.);
#10881=VECTOR('',#39178,10.);
#10882=VECTOR('',#39179,10.);
#10883=VECTOR('',#39182,10.);
#10884=VECTOR('',#39183,10.);
#10885=VECTOR('',#39186,10.);
#10886=VECTOR('',#39187,10.);
#10887=VECTOR('',#39190,10.);
#10888=VECTOR('',#39191,10.);
#10889=VECTOR('',#39194,10.);
#10890=VECTOR('',#39195,10.);
#10891=VECTOR('',#39198,10.);
#10892=VECTOR('',#39199,10.);
#10893=VECTOR('',#39202,10.);
#10894=VECTOR('',#39203,10.);
#10895=VECTOR('',#39212,10.);
#10896=VECTOR('',#39213,10.);
#10897=VECTOR('',#39214,10.);
#10898=VECTOR('',#39215,10.);
#10899=VECTOR('',#39218,10.);
#10900=VECTOR('',#39219,10.);
#10901=VECTOR('',#39222,10.);
#10902=VECTOR('',#39223,10.);
#10903=VECTOR('',#39224,10.);
#10904=VECTOR('',#39227,10.);
#10905=VECTOR('',#39228,10.);
#10906=VECTOR('',#39229,10.);
#10907=VECTOR('',#39232,10.);
#10908=VECTOR('',#39233,10.);
#10909=VECTOR('',#39236,10.);
#10910=VECTOR('',#39237,10.);
#10911=VECTOR('',#39240,10.);
#10912=VECTOR('',#39241,10.);
#10913=VECTOR('',#39244,10.);
#10914=VECTOR('',#39245,10.);
#10915=VECTOR('',#39246,10.);
#10916=VECTOR('',#39249,10.);
#10917=VECTOR('',#39250,10.);
#10918=VECTOR('',#39253,10.);
#10919=VECTOR('',#39254,10.);
#10920=VECTOR('',#39257,10.);
#10921=VECTOR('',#39258,10.);
#10922=VECTOR('',#39261,10.);
#10923=VECTOR('',#39268,10.);
#10924=VECTOR('',#39269,10.);
#10925=VECTOR('',#39270,10.);
#10926=VECTOR('',#39273,10.);
#10927=VECTOR('',#39274,10.);
#10928=VECTOR('',#39275,10.);
#10929=VECTOR('',#39278,10.);
#10930=VECTOR('',#39279,10.);
#10931=VECTOR('',#39280,10.);
#10932=VECTOR('',#39283,10.);
#10933=VECTOR('',#39284,10.);
#10934=VECTOR('',#39287,10.);
#10935=VECTOR('',#39288,10.);
#10936=VECTOR('',#39289,10.);
#10937=VECTOR('',#39292,10.);
#10938=VECTOR('',#39293,10.);
#10939=VECTOR('',#39296,10.);
#10940=VECTOR('',#39297,10.);
#10941=VECTOR('',#39300,10.);
#10942=VECTOR('',#39301,10.);
#10943=VECTOR('',#39304,10.);
#10944=VECTOR('',#39305,10.);
#10945=VECTOR('',#39308,10.);
#10946=VECTOR('',#39309,10.);
#10947=VECTOR('',#39312,10.);
#10948=VECTOR('',#39313,10.);
#10949=VECTOR('',#39316,10.);
#10950=VECTOR('',#39317,10.);
#10951=VECTOR('',#39326,10.);
#10952=VECTOR('',#39327,10.);
#10953=VECTOR('',#39328,10.);
#10954=VECTOR('',#39331,10.);
#10955=VECTOR('',#39332,10.);
#10956=VECTOR('',#39333,10.);
#10957=VECTOR('',#39334,10.);
#10958=VECTOR('',#39337,10.);
#10959=VECTOR('',#39338,10.);
#10960=VECTOR('',#39341,10.);
#10961=VECTOR('',#39342,10.);
#10962=VECTOR('',#39343,10.);
#10963=VECTOR('',#39346,10.);
#10964=VECTOR('',#39347,10.);
#10965=VECTOR('',#39348,10.);
#10966=VECTOR('',#39349,10.);
#10967=VECTOR('',#39352,10.);
#10968=VECTOR('',#39353,10.);
#10969=VECTOR('',#39356,10.);
#10970=VECTOR('',#39357,10.);
#10971=VECTOR('',#39360,10.);
#10972=VECTOR('',#39361,10.);
#10973=VECTOR('',#39362,10.);
#10974=VECTOR('',#39365,10.);
#10975=VECTOR('',#39368,10.);
#10976=VECTOR('',#39369,10.);
#10977=VECTOR('',#39372,10.);
#10978=VECTOR('',#39373,10.);
#10979=VECTOR('',#39380,10.);
#10980=VECTOR('',#39381,10.);
#10981=VECTOR('',#39382,10.);
#10982=VECTOR('',#39385,10.);
#10983=VECTOR('',#39386,10.);
#10984=VECTOR('',#39387,10.);
#10985=VECTOR('',#39390,10.);
#10986=VECTOR('',#39391,10.);
#10987=VECTOR('',#39392,10.);
#10988=VECTOR('',#39395,10.);
#10989=VECTOR('',#39396,10.);
#10990=VECTOR('',#39399,10.);
#10991=VECTOR('',#39400,10.);
#10992=VECTOR('',#39401,10.);
#10993=VECTOR('',#39404,10.);
#10994=VECTOR('',#39405,10.);
#10995=VECTOR('',#39408,10.);
#10996=VECTOR('',#39409,10.);
#10997=VECTOR('',#39412,10.);
#10998=VECTOR('',#39413,10.);
#10999=VECTOR('',#39416,10.);
#11000=VECTOR('',#39417,10.);
#11001=VECTOR('',#39420,10.);
#11002=VECTOR('',#39421,10.);
#11003=VECTOR('',#39424,10.);
#11004=VECTOR('',#39425,10.);
#11005=VECTOR('',#39428,10.);
#11006=VECTOR('',#39429,10.);
#11007=VECTOR('',#39438,10.);
#11008=VECTOR('',#39439,10.);
#11009=VECTOR('',#39440,10.);
#11010=VECTOR('',#39443,10.);
#11011=VECTOR('',#39444,10.);
#11012=VECTOR('',#39445,10.);
#11013=VECTOR('',#39448,10.);
#11014=VECTOR('',#39449,10.);
#11015=VECTOR('',#39450,10.);
#11016=VECTOR('',#39453,10.);
#11017=VECTOR('',#39454,10.);
#11018=VECTOR('',#39457,10.);
#11019=VECTOR('',#39458,10.);
#11020=VECTOR('',#39459,10.);
#11021=VECTOR('',#39462,10.);
#11022=VECTOR('',#39463,10.);
#11023=VECTOR('',#39466,10.);
#11024=VECTOR('',#39467,10.);
#11025=VECTOR('',#39470,10.);
#11026=VECTOR('',#39471,10.);
#11027=VECTOR('',#39474,10.);
#11028=VECTOR('',#39475,10.);
#11029=VECTOR('',#39478,10.);
#11030=VECTOR('',#39479,10.);
#11031=VECTOR('',#39482,10.);
#11032=VECTOR('',#39483,10.);
#11033=VECTOR('',#39486,10.);
#11034=VECTOR('',#39487,10.);
#11035=VECTOR('',#39496,10.);
#11036=VECTOR('',#39497,10.);
#11037=VECTOR('',#39498,10.);
#11038=VECTOR('',#39499,10.);
#11039=VECTOR('',#39502,10.);
#11040=VECTOR('',#39503,10.);
#11041=VECTOR('',#39506,10.);
#11042=VECTOR('',#39507,10.);
#11043=VECTOR('',#39508,10.);
#11044=VECTOR('',#39511,10.);
#11045=VECTOR('',#39512,10.);
#11046=VECTOR('',#39513,10.);
#11047=VECTOR('',#39516,10.);
#11048=VECTOR('',#39517,10.);
#11049=VECTOR('',#39520,10.);
#11050=VECTOR('',#39521,10.);
#11051=VECTOR('',#39524,10.);
#11052=VECTOR('',#39525,10.);
#11053=VECTOR('',#39528,10.);
#11054=VECTOR('',#39529,10.);
#11055=VECTOR('',#39530,10.);
#11056=VECTOR('',#39533,10.);
#11057=VECTOR('',#39534,10.);
#11058=VECTOR('',#39537,10.);
#11059=VECTOR('',#39538,10.);
#11060=VECTOR('',#39541,10.);
#11061=VECTOR('',#39542,10.);
#11062=VECTOR('',#39545,10.);
#11063=VECTOR('',#39552,10.);
#11064=VECTOR('',#39553,10.);
#11065=VECTOR('',#39554,10.);
#11066=VECTOR('',#39557,10.);
#11067=VECTOR('',#39558,10.);
#11068=VECTOR('',#39559,10.);
#11069=VECTOR('',#39562,10.);
#11070=VECTOR('',#39563,10.);
#11071=VECTOR('',#39564,10.);
#11072=VECTOR('',#39567,10.);
#11073=VECTOR('',#39568,10.);
#11074=VECTOR('',#39571,10.);
#11075=VECTOR('',#39572,10.);
#11076=VECTOR('',#39573,10.);
#11077=VECTOR('',#39576,10.);
#11078=VECTOR('',#39577,10.);
#11079=VECTOR('',#39580,10.);
#11080=VECTOR('',#39581,10.);
#11081=VECTOR('',#39584,10.);
#11082=VECTOR('',#39585,10.);
#11083=VECTOR('',#39588,10.);
#11084=VECTOR('',#39589,10.);
#11085=VECTOR('',#39592,10.);
#11086=VECTOR('',#39593,10.);
#11087=VECTOR('',#39596,10.);
#11088=VECTOR('',#39597,10.);
#11089=VECTOR('',#39600,10.);
#11090=VECTOR('',#39601,10.);
#11091=VECTOR('',#39610,10.);
#11092=VECTOR('',#39611,10.);
#11093=VECTOR('',#39612,10.);
#11094=VECTOR('',#39615,10.);
#11095=VECTOR('',#39616,10.);
#11096=VECTOR('',#39617,10.);
#11097=VECTOR('',#39618,10.);
#11098=VECTOR('',#39621,10.);
#11099=VECTOR('',#39622,10.);
#11100=VECTOR('',#39625,10.);
#11101=VECTOR('',#39626,10.);
#11102=VECTOR('',#39627,10.);
#11103=VECTOR('',#39630,10.);
#11104=VECTOR('',#39631,10.);
#11105=VECTOR('',#39632,10.);
#11106=VECTOR('',#39633,10.);
#11107=VECTOR('',#39636,10.);
#11108=VECTOR('',#39637,10.);
#11109=VECTOR('',#39640,10.);
#11110=VECTOR('',#39641,10.);
#11111=VECTOR('',#39644,10.);
#11112=VECTOR('',#39645,10.);
#11113=VECTOR('',#39646,10.);
#11114=VECTOR('',#39649,10.);
#11115=VECTOR('',#39652,10.);
#11116=VECTOR('',#39653,10.);
#11117=VECTOR('',#39656,10.);
#11118=VECTOR('',#39657,10.);
#11119=VECTOR('',#39664,10.);
#11120=VECTOR('',#39665,10.);
#11121=VECTOR('',#39666,10.);
#11122=VECTOR('',#39669,10.);
#11123=VECTOR('',#39670,10.);
#11124=VECTOR('',#39671,10.);
#11125=VECTOR('',#39674,10.);
#11126=VECTOR('',#39675,10.);
#11127=VECTOR('',#39676,10.);
#11128=VECTOR('',#39679,10.);
#11129=VECTOR('',#39680,10.);
#11130=VECTOR('',#39683,10.);
#11131=VECTOR('',#39684,10.);
#11132=VECTOR('',#39685,10.);
#11133=VECTOR('',#39688,10.);
#11134=VECTOR('',#39689,10.);
#11135=VECTOR('',#39692,10.);
#11136=VECTOR('',#39693,10.);
#11137=VECTOR('',#39696,10.);
#11138=VECTOR('',#39697,10.);
#11139=VECTOR('',#39700,10.);
#11140=VECTOR('',#39701,10.);
#11141=VECTOR('',#39704,10.);
#11142=VECTOR('',#39705,10.);
#11143=VECTOR('',#39708,10.);
#11144=VECTOR('',#39709,10.);
#11145=VECTOR('',#39712,10.);
#11146=VECTOR('',#39713,10.);
#11147=VECTOR('',#39722,10.);
#11148=VECTOR('',#39723,10.);
#11149=VECTOR('',#39724,10.);
#11150=VECTOR('',#39727,10.);
#11151=VECTOR('',#39728,10.);
#11152=VECTOR('',#39729,10.);
#11153=VECTOR('',#39732,10.);
#11154=VECTOR('',#39733,10.);
#11155=VECTOR('',#39734,10.);
#11156=VECTOR('',#39737,10.);
#11157=VECTOR('',#39738,10.);
#11158=VECTOR('',#39741,10.);
#11159=VECTOR('',#39742,10.);
#11160=VECTOR('',#39743,10.);
#11161=VECTOR('',#39746,10.);
#11162=VECTOR('',#39747,10.);
#11163=VECTOR('',#39750,10.);
#11164=VECTOR('',#39751,10.);
#11165=VECTOR('',#39754,10.);
#11166=VECTOR('',#39755,10.);
#11167=VECTOR('',#39758,10.);
#11168=VECTOR('',#39759,10.);
#11169=VECTOR('',#39762,10.);
#11170=VECTOR('',#39763,10.);
#11171=VECTOR('',#39766,10.);
#11172=VECTOR('',#39767,10.);
#11173=VECTOR('',#39770,10.);
#11174=VECTOR('',#39771,10.);
#11175=VECTOR('',#39780,10.);
#11176=VECTOR('',#39781,10.);
#11177=VECTOR('',#39782,10.);
#11178=VECTOR('',#39783,10.);
#11179=VECTOR('',#39786,10.);
#11180=VECTOR('',#39787,10.);
#11181=VECTOR('',#39790,10.);
#11182=VECTOR('',#39791,10.);
#11183=VECTOR('',#39792,10.);
#11184=VECTOR('',#39795,10.);
#11185=VECTOR('',#39796,10.);
#11186=VECTOR('',#39797,10.);
#11187=VECTOR('',#39800,10.);
#11188=VECTOR('',#39801,10.);
#11189=VECTOR('',#39804,10.);
#11190=VECTOR('',#39805,10.);
#11191=VECTOR('',#39808,10.);
#11192=VECTOR('',#39809,10.);
#11193=VECTOR('',#39812,10.);
#11194=VECTOR('',#39813,10.);
#11195=VECTOR('',#39814,10.);
#11196=VECTOR('',#39817,10.);
#11197=VECTOR('',#39818,10.);
#11198=VECTOR('',#39821,10.);
#11199=VECTOR('',#39822,10.);
#11200=VECTOR('',#39825,10.);
#11201=VECTOR('',#39826,10.);
#11202=VECTOR('',#39829,10.);
#11203=VECTOR('',#39836,10.);
#11204=VECTOR('',#39837,10.);
#11205=VECTOR('',#39838,10.);
#11206=VECTOR('',#39841,10.);
#11207=VECTOR('',#39842,10.);
#11208=VECTOR('',#39843,10.);
#11209=VECTOR('',#39846,10.);
#11210=VECTOR('',#39847,10.);
#11211=VECTOR('',#39848,10.);
#11212=VECTOR('',#39851,10.);
#11213=VECTOR('',#39852,10.);
#11214=VECTOR('',#39855,10.);
#11215=VECTOR('',#39856,10.);
#11216=VECTOR('',#39857,10.);
#11217=VECTOR('',#39860,10.);
#11218=VECTOR('',#39861,10.);
#11219=VECTOR('',#39864,10.);
#11220=VECTOR('',#39865,10.);
#11221=VECTOR('',#39868,10.);
#11222=VECTOR('',#39869,10.);
#11223=VECTOR('',#39872,10.);
#11224=VECTOR('',#39873,10.);
#11225=VECTOR('',#39876,10.);
#11226=VECTOR('',#39877,10.);
#11227=VECTOR('',#39880,10.);
#11228=VECTOR('',#39881,10.);
#11229=VECTOR('',#39884,10.);
#11230=VECTOR('',#39885,10.);
#11231=VECTOR('',#39894,10.);
#11232=VECTOR('',#39895,10.);
#11233=VECTOR('',#39896,10.);
#11234=VECTOR('',#39899,10.);
#11235=VECTOR('',#39900,10.);
#11236=VECTOR('',#39901,10.);
#11237=VECTOR('',#39902,10.);
#11238=VECTOR('',#39905,10.);
#11239=VECTOR('',#39906,10.);
#11240=VECTOR('',#39909,10.);
#11241=VECTOR('',#39910,10.);
#11242=VECTOR('',#39911,10.);
#11243=VECTOR('',#39914,10.);
#11244=VECTOR('',#39915,10.);
#11245=VECTOR('',#39916,10.);
#11246=VECTOR('',#39917,10.);
#11247=VECTOR('',#39920,10.);
#11248=VECTOR('',#39921,10.);
#11249=VECTOR('',#39924,10.);
#11250=VECTOR('',#39925,10.);
#11251=VECTOR('',#39928,10.);
#11252=VECTOR('',#39929,10.);
#11253=VECTOR('',#39930,10.);
#11254=VECTOR('',#39933,10.);
#11255=VECTOR('',#39936,10.);
#11256=VECTOR('',#39937,10.);
#11257=VECTOR('',#39940,10.);
#11258=VECTOR('',#39941,10.);
#11259=VECTOR('',#39948,10.);
#11260=VECTOR('',#39949,10.);
#11261=VECTOR('',#39950,10.);
#11262=VECTOR('',#39953,10.);
#11263=VECTOR('',#39954,10.);
#11264=VECTOR('',#39955,10.);
#11265=VECTOR('',#39958,10.);
#11266=VECTOR('',#39959,10.);
#11267=VECTOR('',#39960,10.);
#11268=VECTOR('',#39963,10.);
#11269=VECTOR('',#39964,10.);
#11270=VECTOR('',#39967,10.);
#11271=VECTOR('',#39968,10.);
#11272=VECTOR('',#39969,10.);
#11273=VECTOR('',#39972,10.);
#11274=VECTOR('',#39973,10.);
#11275=VECTOR('',#39976,10.);
#11276=VECTOR('',#39977,10.);
#11277=VECTOR('',#39980,10.);
#11278=VECTOR('',#39981,10.);
#11279=VECTOR('',#39984,10.);
#11280=VECTOR('',#39985,10.);
#11281=VECTOR('',#39988,10.);
#11282=VECTOR('',#39989,10.);
#11283=VECTOR('',#39992,10.);
#11284=VECTOR('',#39993,10.);
#11285=VECTOR('',#39996,10.);
#11286=VECTOR('',#39997,10.);
#11287=VECTOR('',#40006,10.);
#11288=VECTOR('',#40007,10.);
#11289=VECTOR('',#40008,10.);
#11290=VECTOR('',#40011,10.);
#11291=VECTOR('',#40012,10.);
#11292=VECTOR('',#40013,10.);
#11293=VECTOR('',#40016,10.);
#11294=VECTOR('',#40017,10.);
#11295=VECTOR('',#40018,10.);
#11296=VECTOR('',#40021,10.);
#11297=VECTOR('',#40022,10.);
#11298=VECTOR('',#40025,10.);
#11299=VECTOR('',#40026,10.);
#11300=VECTOR('',#40027,10.);
#11301=VECTOR('',#40030,10.);
#11302=VECTOR('',#40031,10.);
#11303=VECTOR('',#40034,10.);
#11304=VECTOR('',#40035,10.);
#11305=VECTOR('',#40038,10.);
#11306=VECTOR('',#40039,10.);
#11307=VECTOR('',#40042,10.);
#11308=VECTOR('',#40043,10.);
#11309=VECTOR('',#40046,10.);
#11310=VECTOR('',#40047,10.);
#11311=VECTOR('',#40050,10.);
#11312=VECTOR('',#40051,10.);
#11313=VECTOR('',#40054,10.);
#11314=VECTOR('',#40055,10.);
#11315=VECTOR('',#40064,10.);
#11316=VECTOR('',#40065,10.);
#11317=VECTOR('',#40066,10.);
#11318=VECTOR('',#40067,10.);
#11319=VECTOR('',#40070,10.);
#11320=VECTOR('',#40071,10.);
#11321=VECTOR('',#40074,10.);
#11322=VECTOR('',#40075,10.);
#11323=VECTOR('',#40076,10.);
#11324=VECTOR('',#40079,10.);
#11325=VECTOR('',#40080,10.);
#11326=VECTOR('',#40081,10.);
#11327=VECTOR('',#40084,10.);
#11328=VECTOR('',#40085,10.);
#11329=VECTOR('',#40088,10.);
#11330=VECTOR('',#40089,10.);
#11331=VECTOR('',#40092,10.);
#11332=VECTOR('',#40093,10.);
#11333=VECTOR('',#40096,10.);
#11334=VECTOR('',#40097,10.);
#11335=VECTOR('',#40098,10.);
#11336=VECTOR('',#40101,10.);
#11337=VECTOR('',#40102,10.);
#11338=VECTOR('',#40105,10.);
#11339=VECTOR('',#40106,10.);
#11340=VECTOR('',#40109,10.);
#11341=VECTOR('',#40110,10.);
#11342=VECTOR('',#40113,10.);
#11343=VECTOR('',#40120,10.);
#11344=VECTOR('',#40121,10.);
#11345=VECTOR('',#40122,10.);
#11346=VECTOR('',#40125,10.);
#11347=VECTOR('',#40126,10.);
#11348=VECTOR('',#40127,10.);
#11349=VECTOR('',#40130,10.);
#11350=VECTOR('',#40131,10.);
#11351=VECTOR('',#40132,10.);
#11352=VECTOR('',#40135,10.);
#11353=VECTOR('',#40136,10.);
#11354=VECTOR('',#40139,10.);
#11355=VECTOR('',#40140,10.);
#11356=VECTOR('',#40141,10.);
#11357=VECTOR('',#40144,10.);
#11358=VECTOR('',#40145,10.);
#11359=VECTOR('',#40148,10.);
#11360=VECTOR('',#40149,10.);
#11361=VECTOR('',#40152,10.);
#11362=VECTOR('',#40153,10.);
#11363=VECTOR('',#40156,10.);
#11364=VECTOR('',#40157,10.);
#11365=VECTOR('',#40160,10.);
#11366=VECTOR('',#40161,10.);
#11367=VECTOR('',#40164,10.);
#11368=VECTOR('',#40165,10.);
#11369=VECTOR('',#40168,10.);
#11370=VECTOR('',#40169,10.);
#11371=VECTOR('',#40178,10.);
#11372=VECTOR('',#40179,10.);
#11373=VECTOR('',#40180,10.);
#11374=VECTOR('',#40183,10.);
#11375=VECTOR('',#40184,10.);
#11376=VECTOR('',#40185,10.);
#11377=VECTOR('',#40186,10.);
#11378=VECTOR('',#40189,10.);
#11379=VECTOR('',#40190,10.);
#11380=VECTOR('',#40193,10.);
#11381=VECTOR('',#40194,10.);
#11382=VECTOR('',#40195,10.);
#11383=VECTOR('',#40198,10.);
#11384=VECTOR('',#40199,10.);
#11385=VECTOR('',#40200,10.);
#11386=VECTOR('',#40201,10.);
#11387=VECTOR('',#40204,10.);
#11388=VECTOR('',#40205,10.);
#11389=VECTOR('',#40208,10.);
#11390=VECTOR('',#40209,10.);
#11391=VECTOR('',#40212,10.);
#11392=VECTOR('',#40213,10.);
#11393=VECTOR('',#40214,10.);
#11394=VECTOR('',#40217,10.);
#11395=VECTOR('',#40220,10.);
#11396=VECTOR('',#40221,10.);
#11397=VECTOR('',#40224,10.);
#11398=VECTOR('',#40225,10.);
#11399=VECTOR('',#40232,10.);
#11400=VECTOR('',#40233,10.);
#11401=VECTOR('',#40234,10.);
#11402=VECTOR('',#40237,10.);
#11403=VECTOR('',#40238,10.);
#11404=VECTOR('',#40239,10.);
#11405=VECTOR('',#40242,10.);
#11406=VECTOR('',#40243,10.);
#11407=VECTOR('',#40244,10.);
#11408=VECTOR('',#40247,10.);
#11409=VECTOR('',#40248,10.);
#11410=VECTOR('',#40251,10.);
#11411=VECTOR('',#40252,10.);
#11412=VECTOR('',#40253,10.);
#11413=VECTOR('',#40256,10.);
#11414=VECTOR('',#40257,10.);
#11415=VECTOR('',#40260,10.);
#11416=VECTOR('',#40261,10.);
#11417=VECTOR('',#40264,10.);
#11418=VECTOR('',#40265,10.);
#11419=VECTOR('',#40268,10.);
#11420=VECTOR('',#40269,10.);
#11421=VECTOR('',#40272,10.);
#11422=VECTOR('',#40273,10.);
#11423=VECTOR('',#40276,10.);
#11424=VECTOR('',#40277,10.);
#11425=VECTOR('',#40280,10.);
#11426=VECTOR('',#40281,10.);
#11427=VECTOR('',#40290,10.);
#11428=VECTOR('',#40291,10.);
#11429=VECTOR('',#40292,10.);
#11430=VECTOR('',#40295,10.);
#11431=VECTOR('',#40296,10.);
#11432=VECTOR('',#40297,10.);
#11433=VECTOR('',#40300,10.);
#11434=VECTOR('',#40301,10.);
#11435=VECTOR('',#40302,10.);
#11436=VECTOR('',#40305,10.);
#11437=VECTOR('',#40306,10.);
#11438=VECTOR('',#40309,10.);
#11439=VECTOR('',#40310,10.);
#11440=VECTOR('',#40311,10.);
#11441=VECTOR('',#40314,10.);
#11442=VECTOR('',#40315,10.);
#11443=VECTOR('',#40318,10.);
#11444=VECTOR('',#40319,10.);
#11445=VECTOR('',#40322,10.);
#11446=VECTOR('',#40323,10.);
#11447=VECTOR('',#40326,10.);
#11448=VECTOR('',#40327,10.);
#11449=VECTOR('',#40330,10.);
#11450=VECTOR('',#40331,10.);
#11451=VECTOR('',#40334,10.);
#11452=VECTOR('',#40335,10.);
#11453=VECTOR('',#40338,10.);
#11454=VECTOR('',#40339,10.);
#11455=VECTOR('',#40348,10.);
#11456=VECTOR('',#40349,10.);
#11457=VECTOR('',#40350,10.);
#11458=VECTOR('',#40351,10.);
#11459=VECTOR('',#40354,10.);
#11460=VECTOR('',#40355,10.);
#11461=VECTOR('',#40358,10.);
#11462=VECTOR('',#40359,10.);
#11463=VECTOR('',#40360,10.);
#11464=VECTOR('',#40363,10.);
#11465=VECTOR('',#40364,10.);
#11466=VECTOR('',#40365,10.);
#11467=VECTOR('',#40368,10.);
#11468=VECTOR('',#40369,10.);
#11469=VECTOR('',#40372,10.);
#11470=VECTOR('',#40373,10.);
#11471=VECTOR('',#40376,10.);
#11472=VECTOR('',#40377,10.);
#11473=VECTOR('',#40380,10.);
#11474=VECTOR('',#40381,10.);
#11475=VECTOR('',#40382,10.);
#11476=VECTOR('',#40385,10.);
#11477=VECTOR('',#40386,10.);
#11478=VECTOR('',#40389,10.);
#11479=VECTOR('',#40390,10.);
#11480=VECTOR('',#40393,10.);
#11481=VECTOR('',#40394,10.);
#11482=VECTOR('',#40397,10.);
#11483=VECTOR('',#40404,10.);
#11484=VECTOR('',#40405,10.);
#11485=VECTOR('',#40406,10.);
#11486=VECTOR('',#40409,10.);
#11487=VECTOR('',#40410,10.);
#11488=VECTOR('',#40411,10.);
#11489=VECTOR('',#40414,10.);
#11490=VECTOR('',#40415,10.);
#11491=VECTOR('',#40416,10.);
#11492=VECTOR('',#40419,10.);
#11493=VECTOR('',#40420,10.);
#11494=VECTOR('',#40423,10.);
#11495=VECTOR('',#40424,10.);
#11496=VECTOR('',#40425,10.);
#11497=VECTOR('',#40428,10.);
#11498=VECTOR('',#40429,10.);
#11499=VECTOR('',#40432,10.);
#11500=VECTOR('',#40433,10.);
#11501=VECTOR('',#40436,10.);
#11502=VECTOR('',#40437,10.);
#11503=VECTOR('',#40440,10.);
#11504=VECTOR('',#40441,10.);
#11505=VECTOR('',#40444,10.);
#11506=VECTOR('',#40445,10.);
#11507=VECTOR('',#40448,10.);
#11508=VECTOR('',#40449,10.);
#11509=VECTOR('',#40452,10.);
#11510=VECTOR('',#40453,10.);
#11511=VECTOR('',#40462,10.);
#11512=VECTOR('',#40463,10.);
#11513=VECTOR('',#40464,10.);
#11514=VECTOR('',#40467,10.);
#11515=VECTOR('',#40468,10.);
#11516=VECTOR('',#40469,10.);
#11517=VECTOR('',#40470,10.);
#11518=VECTOR('',#40473,10.);
#11519=VECTOR('',#40474,10.);
#11520=VECTOR('',#40477,10.);
#11521=VECTOR('',#40478,10.);
#11522=VECTOR('',#40479,10.);
#11523=VECTOR('',#40482,10.);
#11524=VECTOR('',#40483,10.);
#11525=VECTOR('',#40484,10.);
#11526=VECTOR('',#40485,10.);
#11527=VECTOR('',#40488,10.);
#11528=VECTOR('',#40489,10.);
#11529=VECTOR('',#40492,10.);
#11530=VECTOR('',#40493,10.);
#11531=VECTOR('',#40496,10.);
#11532=VECTOR('',#40497,10.);
#11533=VECTOR('',#40498,10.);
#11534=VECTOR('',#40501,10.);
#11535=VECTOR('',#40504,10.);
#11536=VECTOR('',#40505,10.);
#11537=VECTOR('',#40508,10.);
#11538=VECTOR('',#40509,10.);
#11539=VECTOR('',#40516,10.);
#11540=VECTOR('',#40517,10.);
#11541=VECTOR('',#40518,10.);
#11542=VECTOR('',#40521,10.);
#11543=VECTOR('',#40522,10.);
#11544=VECTOR('',#40523,10.);
#11545=VECTOR('',#40526,10.);
#11546=VECTOR('',#40527,10.);
#11547=VECTOR('',#40528,10.);
#11548=VECTOR('',#40531,10.);
#11549=VECTOR('',#40532,10.);
#11550=VECTOR('',#40535,10.);
#11551=VECTOR('',#40536,10.);
#11552=VECTOR('',#40537,10.);
#11553=VECTOR('',#40540,10.);
#11554=VECTOR('',#40541,10.);
#11555=VECTOR('',#40544,10.);
#11556=VECTOR('',#40545,10.);
#11557=VECTOR('',#40548,10.);
#11558=VECTOR('',#40549,10.);
#11559=VECTOR('',#40552,10.);
#11560=VECTOR('',#40553,10.);
#11561=VECTOR('',#40556,10.);
#11562=VECTOR('',#40557,10.);
#11563=VECTOR('',#40560,10.);
#11564=VECTOR('',#40561,10.);
#11565=VECTOR('',#40564,10.);
#11566=VECTOR('',#40565,10.);
#11567=VECTOR('',#40574,10.);
#11568=VECTOR('',#40575,10.);
#11569=VECTOR('',#40576,10.);
#11570=VECTOR('',#40579,10.);
#11571=VECTOR('',#40580,10.);
#11572=VECTOR('',#40581,10.);
#11573=VECTOR('',#40584,10.);
#11574=VECTOR('',#40585,10.);
#11575=VECTOR('',#40586,10.);
#11576=VECTOR('',#40589,10.);
#11577=VECTOR('',#40590,10.);
#11578=VECTOR('',#40593,10.);
#11579=VECTOR('',#40594,10.);
#11580=VECTOR('',#40595,10.);
#11581=VECTOR('',#40598,10.);
#11582=VECTOR('',#40599,10.);
#11583=VECTOR('',#40602,10.);
#11584=VECTOR('',#40603,10.);
#11585=VECTOR('',#40606,10.);
#11586=VECTOR('',#40607,10.);
#11587=VECTOR('',#40610,10.);
#11588=VECTOR('',#40611,10.);
#11589=VECTOR('',#40614,10.);
#11590=VECTOR('',#40615,10.);
#11591=VECTOR('',#40618,10.);
#11592=VECTOR('',#40619,10.);
#11593=VECTOR('',#40622,10.);
#11594=VECTOR('',#40623,10.);
#11595=VECTOR('',#40632,10.);
#11596=VECTOR('',#40633,10.);
#11597=VECTOR('',#40634,10.);
#11598=VECTOR('',#40635,10.);
#11599=VECTOR('',#40638,10.);
#11600=VECTOR('',#40639,10.);
#11601=VECTOR('',#40642,10.);
#11602=VECTOR('',#40643,10.);
#11603=VECTOR('',#40644,10.);
#11604=VECTOR('',#40647,10.);
#11605=VECTOR('',#40648,10.);
#11606=VECTOR('',#40649,10.);
#11607=VECTOR('',#40652,10.);
#11608=VECTOR('',#40653,10.);
#11609=VECTOR('',#40656,10.);
#11610=VECTOR('',#40657,10.);
#11611=VECTOR('',#40660,10.);
#11612=VECTOR('',#40661,10.);
#11613=VECTOR('',#40664,10.);
#11614=VECTOR('',#40665,10.);
#11615=VECTOR('',#40666,10.);
#11616=VECTOR('',#40669,10.);
#11617=VECTOR('',#40670,10.);
#11618=VECTOR('',#40673,10.);
#11619=VECTOR('',#40674,10.);
#11620=VECTOR('',#40677,10.);
#11621=VECTOR('',#40678,10.);
#11622=VECTOR('',#40681,10.);
#11623=VECTOR('',#40688,10.);
#11624=VECTOR('',#40689,10.);
#11625=VECTOR('',#40690,10.);
#11626=VECTOR('',#40693,10.);
#11627=VECTOR('',#40694,10.);
#11628=VECTOR('',#40695,10.);
#11629=VECTOR('',#40698,10.);
#11630=VECTOR('',#40699,10.);
#11631=VECTOR('',#40700,10.);
#11632=VECTOR('',#40703,10.);
#11633=VECTOR('',#40704,10.);
#11634=VECTOR('',#40707,10.);
#11635=VECTOR('',#40708,10.);
#11636=VECTOR('',#40709,10.);
#11637=VECTOR('',#40712,10.);
#11638=VECTOR('',#40713,10.);
#11639=VECTOR('',#40716,10.);
#11640=VECTOR('',#40717,10.);
#11641=VECTOR('',#40720,10.);
#11642=VECTOR('',#40721,10.);
#11643=VECTOR('',#40724,10.);
#11644=VECTOR('',#40725,10.);
#11645=VECTOR('',#40728,10.);
#11646=VECTOR('',#40729,10.);
#11647=VECTOR('',#40732,10.);
#11648=VECTOR('',#40733,10.);
#11649=VECTOR('',#40736,10.);
#11650=VECTOR('',#40737,10.);
#11651=VECTOR('',#40746,10.);
#11652=VECTOR('',#40747,10.);
#11653=VECTOR('',#40748,10.);
#11654=VECTOR('',#40751,10.);
#11655=VECTOR('',#40752,10.);
#11656=VECTOR('',#40753,10.);
#11657=VECTOR('',#40754,10.);
#11658=VECTOR('',#40757,10.);
#11659=VECTOR('',#40758,10.);
#11660=VECTOR('',#40761,10.);
#11661=VECTOR('',#40762,10.);
#11662=VECTOR('',#40763,10.);
#11663=VECTOR('',#40766,10.);
#11664=VECTOR('',#40767,10.);
#11665=VECTOR('',#40768,10.);
#11666=VECTOR('',#40769,10.);
#11667=VECTOR('',#40772,10.);
#11668=VECTOR('',#40773,10.);
#11669=VECTOR('',#40776,10.);
#11670=VECTOR('',#40777,10.);
#11671=VECTOR('',#40780,10.);
#11672=VECTOR('',#40781,10.);
#11673=VECTOR('',#40782,10.);
#11674=VECTOR('',#40785,10.);
#11675=VECTOR('',#40788,10.);
#11676=VECTOR('',#40789,10.);
#11677=VECTOR('',#40792,10.);
#11678=VECTOR('',#40793,10.);
#11679=VECTOR('',#40800,10.);
#11680=VECTOR('',#40801,10.);
#11681=VECTOR('',#40802,10.);
#11682=VECTOR('',#40805,10.);
#11683=VECTOR('',#40806,10.);
#11684=VECTOR('',#40807,10.);
#11685=VECTOR('',#40810,10.);
#11686=VECTOR('',#40811,10.);
#11687=VECTOR('',#40812,10.);
#11688=VECTOR('',#40815,10.);
#11689=VECTOR('',#40816,10.);
#11690=VECTOR('',#40819,10.);
#11691=VECTOR('',#40820,10.);
#11692=VECTOR('',#40821,10.);
#11693=VECTOR('',#40824,10.);
#11694=VECTOR('',#40825,10.);
#11695=VECTOR('',#40828,10.);
#11696=VECTOR('',#40829,10.);
#11697=VECTOR('',#40832,10.);
#11698=VECTOR('',#40833,10.);
#11699=VECTOR('',#40836,10.);
#11700=VECTOR('',#40837,10.);
#11701=VECTOR('',#40840,10.);
#11702=VECTOR('',#40841,10.);
#11703=VECTOR('',#40844,10.);
#11704=VECTOR('',#40845,10.);
#11705=VECTOR('',#40848,10.);
#11706=VECTOR('',#40849,10.);
#11707=VECTOR('',#40858,10.);
#11708=VECTOR('',#40859,10.);
#11709=VECTOR('',#40860,10.);
#11710=VECTOR('',#40863,10.);
#11711=VECTOR('',#40864,10.);
#11712=VECTOR('',#40865,10.);
#11713=VECTOR('',#40868,10.);
#11714=VECTOR('',#40869,10.);
#11715=VECTOR('',#40870,10.);
#11716=VECTOR('',#40873,10.);
#11717=VECTOR('',#40874,10.);
#11718=VECTOR('',#40877,10.);
#11719=VECTOR('',#40878,10.);
#11720=VECTOR('',#40879,10.);
#11721=VECTOR('',#40882,10.);
#11722=VECTOR('',#40883,10.);
#11723=VECTOR('',#40886,10.);
#11724=VECTOR('',#40887,10.);
#11725=VECTOR('',#40890,10.);
#11726=VECTOR('',#40891,10.);
#11727=VECTOR('',#40894,10.);
#11728=VECTOR('',#40895,10.);
#11729=VECTOR('',#40898,10.);
#11730=VECTOR('',#40899,10.);
#11731=VECTOR('',#40902,10.);
#11732=VECTOR('',#40903,10.);
#11733=VECTOR('',#40906,10.);
#11734=VECTOR('',#40907,10.);
#11735=VECTOR('',#40916,10.);
#11736=VECTOR('',#40917,10.);
#11737=VECTOR('',#40918,10.);
#11738=VECTOR('',#40919,10.);
#11739=VECTOR('',#40922,10.);
#11740=VECTOR('',#40923,10.);
#11741=VECTOR('',#40926,10.);
#11742=VECTOR('',#40927,10.);
#11743=VECTOR('',#40928,10.);
#11744=VECTOR('',#40931,10.);
#11745=VECTOR('',#40932,10.);
#11746=VECTOR('',#40933,10.);
#11747=VECTOR('',#40936,10.);
#11748=VECTOR('',#40937,10.);
#11749=VECTOR('',#40940,10.);
#11750=VECTOR('',#40941,10.);
#11751=VECTOR('',#40944,10.);
#11752=VECTOR('',#40945,10.);
#11753=VECTOR('',#40948,10.);
#11754=VECTOR('',#40949,10.);
#11755=VECTOR('',#40950,10.);
#11756=VECTOR('',#40953,10.);
#11757=VECTOR('',#40954,10.);
#11758=VECTOR('',#40957,10.);
#11759=VECTOR('',#40958,10.);
#11760=VECTOR('',#40961,10.);
#11761=VECTOR('',#40962,10.);
#11762=VECTOR('',#40965,10.);
#11763=VECTOR('',#40972,10.);
#11764=VECTOR('',#40973,10.);
#11765=VECTOR('',#40974,10.);
#11766=VECTOR('',#40977,10.);
#11767=VECTOR('',#40978,10.);
#11768=VECTOR('',#40979,10.);
#11769=VECTOR('',#40982,10.);
#11770=VECTOR('',#40983,10.);
#11771=VECTOR('',#40984,10.);
#11772=VECTOR('',#40987,10.);
#11773=VECTOR('',#40988,10.);
#11774=VECTOR('',#40991,10.);
#11775=VECTOR('',#40992,10.);
#11776=VECTOR('',#40993,10.);
#11777=VECTOR('',#40996,10.);
#11778=VECTOR('',#40997,10.);
#11779=VECTOR('',#41000,10.);
#11780=VECTOR('',#41001,10.);
#11781=VECTOR('',#41004,10.);
#11782=VECTOR('',#41005,10.);
#11783=VECTOR('',#41008,10.);
#11784=VECTOR('',#41009,10.);
#11785=VECTOR('',#41012,10.);
#11786=VECTOR('',#41013,10.);
#11787=VECTOR('',#41016,10.);
#11788=VECTOR('',#41017,10.);
#11789=VECTOR('',#41020,10.);
#11790=VECTOR('',#41021,10.);
#11791=VECTOR('',#41030,10.);
#11792=VECTOR('',#41031,10.);
#11793=VECTOR('',#41032,10.);
#11794=VECTOR('',#41035,10.);
#11795=VECTOR('',#41036,10.);
#11796=VECTOR('',#41037,10.);
#11797=VECTOR('',#41038,10.);
#11798=VECTOR('',#41041,10.);
#11799=VECTOR('',#41042,10.);
#11800=VECTOR('',#41045,10.);
#11801=VECTOR('',#41046,10.);
#11802=VECTOR('',#41047,10.);
#11803=VECTOR('',#41050,10.);
#11804=VECTOR('',#41051,10.);
#11805=VECTOR('',#41052,10.);
#11806=VECTOR('',#41053,10.);
#11807=VECTOR('',#41056,10.);
#11808=VECTOR('',#41057,10.);
#11809=VECTOR('',#41060,10.);
#11810=VECTOR('',#41061,10.);
#11811=VECTOR('',#41064,10.);
#11812=VECTOR('',#41065,10.);
#11813=VECTOR('',#41066,10.);
#11814=VECTOR('',#41069,10.);
#11815=VECTOR('',#41072,10.);
#11816=VECTOR('',#41073,10.);
#11817=VECTOR('',#41076,10.);
#11818=VECTOR('',#41077,10.);
#11819=VECTOR('',#41084,10.);
#11820=VECTOR('',#41085,10.);
#11821=VECTOR('',#41086,10.);
#11822=VECTOR('',#41089,10.);
#11823=VECTOR('',#41090,10.);
#11824=VECTOR('',#41091,10.);
#11825=VECTOR('',#41094,10.);
#11826=VECTOR('',#41095,10.);
#11827=VECTOR('',#41096,10.);
#11828=VECTOR('',#41099,10.);
#11829=VECTOR('',#41100,10.);
#11830=VECTOR('',#41103,10.);
#11831=VECTOR('',#41104,10.);
#11832=VECTOR('',#41105,10.);
#11833=VECTOR('',#41108,10.);
#11834=VECTOR('',#41109,10.);
#11835=VECTOR('',#41112,10.);
#11836=VECTOR('',#41113,10.);
#11837=VECTOR('',#41116,10.);
#11838=VECTOR('',#41117,10.);
#11839=VECTOR('',#41120,10.);
#11840=VECTOR('',#41121,10.);
#11841=VECTOR('',#41124,10.);
#11842=VECTOR('',#41125,10.);
#11843=VECTOR('',#41128,10.);
#11844=VECTOR('',#41129,10.);
#11845=VECTOR('',#41132,10.);
#11846=VECTOR('',#41133,10.);
#11847=VECTOR('',#41142,10.);
#11848=VECTOR('',#41143,10.);
#11849=VECTOR('',#41144,10.);
#11850=VECTOR('',#41147,10.);
#11851=VECTOR('',#41148,10.);
#11852=VECTOR('',#41149,10.);
#11853=VECTOR('',#41152,10.);
#11854=VECTOR('',#41153,10.);
#11855=VECTOR('',#41154,10.);
#11856=VECTOR('',#41157,10.);
#11857=VECTOR('',#41158,10.);
#11858=VECTOR('',#41161,10.);
#11859=VECTOR('',#41162,10.);
#11860=VECTOR('',#41163,10.);
#11861=VECTOR('',#41166,10.);
#11862=VECTOR('',#41167,10.);
#11863=VECTOR('',#41170,10.);
#11864=VECTOR('',#41171,10.);
#11865=VECTOR('',#41174,10.);
#11866=VECTOR('',#41175,10.);
#11867=VECTOR('',#41178,10.);
#11868=VECTOR('',#41179,10.);
#11869=VECTOR('',#41182,10.);
#11870=VECTOR('',#41183,10.);
#11871=VECTOR('',#41186,10.);
#11872=VECTOR('',#41187,10.);
#11873=VECTOR('',#41190,10.);
#11874=VECTOR('',#41191,10.);
#11875=VECTOR('',#41200,10.);
#11876=VECTOR('',#41201,10.);
#11877=VECTOR('',#41202,10.);
#11878=VECTOR('',#41203,10.);
#11879=VECTOR('',#41206,10.);
#11880=VECTOR('',#41207,10.);
#11881=VECTOR('',#41210,10.);
#11882=VECTOR('',#41211,10.);
#11883=VECTOR('',#41212,10.);
#11884=VECTOR('',#41215,10.);
#11885=VECTOR('',#41216,10.);
#11886=VECTOR('',#41217,10.);
#11887=VECTOR('',#41220,10.);
#11888=VECTOR('',#41221,10.);
#11889=VECTOR('',#41224,10.);
#11890=VECTOR('',#41225,10.);
#11891=VECTOR('',#41228,10.);
#11892=VECTOR('',#41229,10.);
#11893=VECTOR('',#41232,10.);
#11894=VECTOR('',#41233,10.);
#11895=VECTOR('',#41234,10.);
#11896=VECTOR('',#41237,10.);
#11897=VECTOR('',#41238,10.);
#11898=VECTOR('',#41241,10.);
#11899=VECTOR('',#41242,10.);
#11900=VECTOR('',#41245,10.);
#11901=VECTOR('',#41246,10.);
#11902=VECTOR('',#41249,10.);
#11903=VECTOR('',#41256,10.);
#11904=VECTOR('',#41257,10.);
#11905=VECTOR('',#41258,10.);
#11906=VECTOR('',#41261,10.);
#11907=VECTOR('',#41262,10.);
#11908=VECTOR('',#41263,10.);
#11909=VECTOR('',#41266,10.);
#11910=VECTOR('',#41267,10.);
#11911=VECTOR('',#41268,10.);
#11912=VECTOR('',#41271,10.);
#11913=VECTOR('',#41272,10.);
#11914=VECTOR('',#41275,10.);
#11915=VECTOR('',#41276,10.);
#11916=VECTOR('',#41277,10.);
#11917=VECTOR('',#41280,10.);
#11918=VECTOR('',#41281,10.);
#11919=VECTOR('',#41284,10.);
#11920=VECTOR('',#41285,10.);
#11921=VECTOR('',#41288,10.);
#11922=VECTOR('',#41289,10.);
#11923=VECTOR('',#41292,10.);
#11924=VECTOR('',#41293,10.);
#11925=VECTOR('',#41296,10.);
#11926=VECTOR('',#41297,10.);
#11927=VECTOR('',#41300,10.);
#11928=VECTOR('',#41301,10.);
#11929=VECTOR('',#41304,10.);
#11930=VECTOR('',#41305,10.);
#11931=VECTOR('',#41314,10.);
#11932=VECTOR('',#41315,10.);
#11933=VECTOR('',#41316,10.);
#11934=VECTOR('',#41319,10.);
#11935=VECTOR('',#41320,10.);
#11936=VECTOR('',#41321,10.);
#11937=VECTOR('',#41322,10.);
#11938=VECTOR('',#41325,10.);
#11939=VECTOR('',#41326,10.);
#11940=VECTOR('',#41329,10.);
#11941=VECTOR('',#41330,10.);
#11942=VECTOR('',#41331,10.);
#11943=VECTOR('',#41334,10.);
#11944=VECTOR('',#41335,10.);
#11945=VECTOR('',#41336,10.);
#11946=VECTOR('',#41337,10.);
#11947=VECTOR('',#41340,10.);
#11948=VECTOR('',#41341,10.);
#11949=VECTOR('',#41344,10.);
#11950=VECTOR('',#41345,10.);
#11951=VECTOR('',#41348,10.);
#11952=VECTOR('',#41349,10.);
#11953=VECTOR('',#41350,10.);
#11954=VECTOR('',#41353,10.);
#11955=VECTOR('',#41356,10.);
#11956=VECTOR('',#41357,10.);
#11957=VECTOR('',#41360,10.);
#11958=VECTOR('',#41361,10.);
#11959=VECTOR('',#41368,10.);
#11960=VECTOR('',#41369,10.);
#11961=VECTOR('',#41370,10.);
#11962=VECTOR('',#41373,10.);
#11963=VECTOR('',#41374,10.);
#11964=VECTOR('',#41375,10.);
#11965=VECTOR('',#41378,10.);
#11966=VECTOR('',#41379,10.);
#11967=VECTOR('',#41380,10.);
#11968=VECTOR('',#41383,10.);
#11969=VECTOR('',#41384,10.);
#11970=VECTOR('',#41387,10.);
#11971=VECTOR('',#41388,10.);
#11972=VECTOR('',#41389,10.);
#11973=VECTOR('',#41392,10.);
#11974=VECTOR('',#41393,10.);
#11975=VECTOR('',#41396,10.);
#11976=VECTOR('',#41397,10.);
#11977=VECTOR('',#41400,10.);
#11978=VECTOR('',#41401,10.);
#11979=VECTOR('',#41404,10.);
#11980=VECTOR('',#41405,10.);
#11981=VECTOR('',#41408,10.);
#11982=VECTOR('',#41409,10.);
#11983=VECTOR('',#41412,10.);
#11984=VECTOR('',#41413,10.);
#11985=VECTOR('',#41416,10.);
#11986=VECTOR('',#41417,10.);
#11987=VECTOR('',#41426,10.);
#11988=VECTOR('',#41427,10.);
#11989=VECTOR('',#41428,10.);
#11990=VECTOR('',#41431,10.);
#11991=VECTOR('',#41432,10.);
#11992=VECTOR('',#41433,10.);
#11993=VECTOR('',#41436,10.);
#11994=VECTOR('',#41437,10.);
#11995=VECTOR('',#41438,10.);
#11996=VECTOR('',#41441,10.);
#11997=VECTOR('',#41442,10.);
#11998=VECTOR('',#41445,10.);
#11999=VECTOR('',#41446,10.);
#12000=VECTOR('',#41447,10.);
#12001=VECTOR('',#41450,10.);
#12002=VECTOR('',#41451,10.);
#12003=VECTOR('',#41454,10.);
#12004=VECTOR('',#41455,10.);
#12005=VECTOR('',#41458,10.);
#12006=VECTOR('',#41459,10.);
#12007=VECTOR('',#41462,10.);
#12008=VECTOR('',#41463,10.);
#12009=VECTOR('',#41466,10.);
#12010=VECTOR('',#41467,10.);
#12011=VECTOR('',#41470,10.);
#12012=VECTOR('',#41471,10.);
#12013=VECTOR('',#41474,10.);
#12014=VECTOR('',#41475,10.);
#12015=VECTOR('',#41484,10.);
#12016=VECTOR('',#41485,10.);
#12017=VECTOR('',#41486,10.);
#12018=VECTOR('',#41487,10.);
#12019=VECTOR('',#41490,10.);
#12020=VECTOR('',#41491,10.);
#12021=VECTOR('',#41494,10.);
#12022=VECTOR('',#41495,10.);
#12023=VECTOR('',#41496,10.);
#12024=VECTOR('',#41499,10.);
#12025=VECTOR('',#41500,10.);
#12026=VECTOR('',#41501,10.);
#12027=VECTOR('',#41504,10.);
#12028=VECTOR('',#41505,10.);
#12029=VECTOR('',#41508,10.);
#12030=VECTOR('',#41509,10.);
#12031=VECTOR('',#41512,10.);
#12032=VECTOR('',#41513,10.);
#12033=VECTOR('',#41516,10.);
#12034=VECTOR('',#41517,10.);
#12035=VECTOR('',#41518,10.);
#12036=VECTOR('',#41521,10.);
#12037=VECTOR('',#41522,10.);
#12038=VECTOR('',#41525,10.);
#12039=VECTOR('',#41526,10.);
#12040=VECTOR('',#41529,10.);
#12041=VECTOR('',#41530,10.);
#12042=VECTOR('',#41533,10.);
#12043=VECTOR('',#41540,10.);
#12044=VECTOR('',#41541,10.);
#12045=VECTOR('',#41542,10.);
#12046=VECTOR('',#41545,10.);
#12047=VECTOR('',#41546,10.);
#12048=VECTOR('',#41547,10.);
#12049=VECTOR('',#41550,10.);
#12050=VECTOR('',#41551,10.);
#12051=VECTOR('',#41552,10.);
#12052=VECTOR('',#41555,10.);
#12053=VECTOR('',#41556,10.);
#12054=VECTOR('',#41559,10.);
#12055=VECTOR('',#41560,10.);
#12056=VECTOR('',#41561,10.);
#12057=VECTOR('',#41564,10.);
#12058=VECTOR('',#41565,10.);
#12059=VECTOR('',#41568,10.);
#12060=VECTOR('',#41569,10.);
#12061=VECTOR('',#41572,10.);
#12062=VECTOR('',#41573,10.);
#12063=VECTOR('',#41576,10.);
#12064=VECTOR('',#41577,10.);
#12065=VECTOR('',#41580,10.);
#12066=VECTOR('',#41581,10.);
#12067=VECTOR('',#41584,10.);
#12068=VECTOR('',#41585,10.);
#12069=VECTOR('',#41588,10.);
#12070=VECTOR('',#41589,10.);
#12071=VECTOR('',#41598,10.);
#12072=VECTOR('',#41599,10.);
#12073=VECTOR('',#41600,10.);
#12074=VECTOR('',#41603,10.);
#12075=VECTOR('',#41604,10.);
#12076=VECTOR('',#41605,10.);
#12077=VECTOR('',#41606,10.);
#12078=VECTOR('',#41609,10.);
#12079=VECTOR('',#41610,10.);
#12080=VECTOR('',#41613,10.);
#12081=VECTOR('',#41614,10.);
#12082=VECTOR('',#41615,10.);
#12083=VECTOR('',#41618,10.);
#12084=VECTOR('',#41619,10.);
#12085=VECTOR('',#41620,10.);
#12086=VECTOR('',#41621,10.);
#12087=VECTOR('',#41624,10.);
#12088=VECTOR('',#41625,10.);
#12089=VECTOR('',#41628,10.);
#12090=VECTOR('',#41629,10.);
#12091=VECTOR('',#41632,10.);
#12092=VECTOR('',#41633,10.);
#12093=VECTOR('',#41634,10.);
#12094=VECTOR('',#41637,10.);
#12095=VECTOR('',#41640,10.);
#12096=VECTOR('',#41641,10.);
#12097=VECTOR('',#41644,10.);
#12098=VECTOR('',#41645,10.);
#12099=VECTOR('',#41652,10.);
#12100=VECTOR('',#41653,10.);
#12101=VECTOR('',#41654,10.);
#12102=VECTOR('',#41657,10.);
#12103=VECTOR('',#41658,10.);
#12104=VECTOR('',#41659,10.);
#12105=VECTOR('',#41662,10.);
#12106=VECTOR('',#41663,10.);
#12107=VECTOR('',#41664,10.);
#12108=VECTOR('',#41667,10.);
#12109=VECTOR('',#41668,10.);
#12110=VECTOR('',#41671,10.);
#12111=VECTOR('',#41672,10.);
#12112=VECTOR('',#41673,10.);
#12113=VECTOR('',#41676,10.);
#12114=VECTOR('',#41677,10.);
#12115=VECTOR('',#41680,10.);
#12116=VECTOR('',#41681,10.);
#12117=VECTOR('',#41684,10.);
#12118=VECTOR('',#41685,10.);
#12119=VECTOR('',#41688,10.);
#12120=VECTOR('',#41689,10.);
#12121=VECTOR('',#41692,10.);
#12122=VECTOR('',#41693,10.);
#12123=VECTOR('',#41696,10.);
#12124=VECTOR('',#41697,10.);
#12125=VECTOR('',#41700,10.);
#12126=VECTOR('',#41701,10.);
#12127=VECTOR('',#41710,10.);
#12128=VECTOR('',#41711,10.);
#12129=VECTOR('',#41712,10.);
#12130=VECTOR('',#41715,10.);
#12131=VECTOR('',#41716,10.);
#12132=VECTOR('',#41717,10.);
#12133=VECTOR('',#41720,10.);
#12134=VECTOR('',#41721,10.);
#12135=VECTOR('',#41722,10.);
#12136=VECTOR('',#41725,10.);
#12137=VECTOR('',#41726,10.);
#12138=VECTOR('',#41729,10.);
#12139=VECTOR('',#41730,10.);
#12140=VECTOR('',#41731,10.);
#12141=VECTOR('',#41734,10.);
#12142=VECTOR('',#41735,10.);
#12143=VECTOR('',#41738,10.);
#12144=VECTOR('',#41739,10.);
#12145=VECTOR('',#41742,10.);
#12146=VECTOR('',#41743,10.);
#12147=VECTOR('',#41746,10.);
#12148=VECTOR('',#41747,10.);
#12149=VECTOR('',#41750,10.);
#12150=VECTOR('',#41751,10.);
#12151=VECTOR('',#41754,10.);
#12152=VECTOR('',#41755,10.);
#12153=VECTOR('',#41758,10.);
#12154=VECTOR('',#41759,10.);
#12155=VECTOR('',#41768,10.);
#12156=VECTOR('',#41769,10.);
#12157=VECTOR('',#41770,10.);
#12158=VECTOR('',#41771,10.);
#12159=VECTOR('',#41774,10.);
#12160=VECTOR('',#41775,10.);
#12161=VECTOR('',#41778,10.);
#12162=VECTOR('',#41779,10.);
#12163=VECTOR('',#41780,10.);
#12164=VECTOR('',#41783,10.);
#12165=VECTOR('',#41784,10.);
#12166=VECTOR('',#41785,10.);
#12167=VECTOR('',#41788,10.);
#12168=VECTOR('',#41789,10.);
#12169=VECTOR('',#41792,10.);
#12170=VECTOR('',#41793,10.);
#12171=VECTOR('',#41796,10.);
#12172=VECTOR('',#41797,10.);
#12173=VECTOR('',#41800,10.);
#12174=VECTOR('',#41801,10.);
#12175=VECTOR('',#41802,10.);
#12176=VECTOR('',#41805,10.);
#12177=VECTOR('',#41806,10.);
#12178=VECTOR('',#41809,10.);
#12179=VECTOR('',#41810,10.);
#12180=VECTOR('',#41813,10.);
#12181=VECTOR('',#41814,10.);
#12182=VECTOR('',#41817,10.);
#12183=VECTOR('',#41824,10.);
#12184=VECTOR('',#41825,10.);
#12185=VECTOR('',#41826,10.);
#12186=VECTOR('',#41829,10.);
#12187=VECTOR('',#41830,10.);
#12188=VECTOR('',#41831,10.);
#12189=VECTOR('',#41834,10.);
#12190=VECTOR('',#41835,10.);
#12191=VECTOR('',#41836,10.);
#12192=VECTOR('',#41839,10.);
#12193=VECTOR('',#41840,10.);
#12194=VECTOR('',#41843,10.);
#12195=VECTOR('',#41844,10.);
#12196=VECTOR('',#41845,10.);
#12197=VECTOR('',#41848,10.);
#12198=VECTOR('',#41849,10.);
#12199=VECTOR('',#41852,10.);
#12200=VECTOR('',#41853,10.);
#12201=VECTOR('',#41856,10.);
#12202=VECTOR('',#41857,10.);
#12203=VECTOR('',#41860,10.);
#12204=VECTOR('',#41861,10.);
#12205=VECTOR('',#41864,10.);
#12206=VECTOR('',#41865,10.);
#12207=VECTOR('',#41868,10.);
#12208=VECTOR('',#41869,10.);
#12209=VECTOR('',#41872,10.);
#12210=VECTOR('',#41873,10.);
#12211=VECTOR('',#41882,10.);
#12212=VECTOR('',#41883,10.);
#12213=VECTOR('',#41884,10.);
#12214=VECTOR('',#41887,10.);
#12215=VECTOR('',#41888,10.);
#12216=VECTOR('',#41889,10.);
#12217=VECTOR('',#41890,10.);
#12218=VECTOR('',#41893,10.);
#12219=VECTOR('',#41894,10.);
#12220=VECTOR('',#41897,10.);
#12221=VECTOR('',#41898,10.);
#12222=VECTOR('',#41899,10.);
#12223=VECTOR('',#41902,10.);
#12224=VECTOR('',#41903,10.);
#12225=VECTOR('',#41904,10.);
#12226=VECTOR('',#41905,10.);
#12227=VECTOR('',#41908,10.);
#12228=VECTOR('',#41909,10.);
#12229=VECTOR('',#41912,10.);
#12230=VECTOR('',#41913,10.);
#12231=VECTOR('',#41916,10.);
#12232=VECTOR('',#41917,10.);
#12233=VECTOR('',#41918,10.);
#12234=VECTOR('',#41921,10.);
#12235=VECTOR('',#41924,10.);
#12236=VECTOR('',#41925,10.);
#12237=VECTOR('',#41928,10.);
#12238=VECTOR('',#41929,10.);
#12239=VECTOR('',#41936,10.);
#12240=VECTOR('',#41937,10.);
#12241=VECTOR('',#41938,10.);
#12242=VECTOR('',#41941,10.);
#12243=VECTOR('',#41942,10.);
#12244=VECTOR('',#41943,10.);
#12245=VECTOR('',#41946,10.);
#12246=VECTOR('',#41947,10.);
#12247=VECTOR('',#41948,10.);
#12248=VECTOR('',#41951,10.);
#12249=VECTOR('',#41952,10.);
#12250=VECTOR('',#41955,10.);
#12251=VECTOR('',#41956,10.);
#12252=VECTOR('',#41957,10.);
#12253=VECTOR('',#41960,10.);
#12254=VECTOR('',#41961,10.);
#12255=VECTOR('',#41964,10.);
#12256=VECTOR('',#41965,10.);
#12257=VECTOR('',#41968,10.);
#12258=VECTOR('',#41969,10.);
#12259=VECTOR('',#41972,10.);
#12260=VECTOR('',#41973,10.);
#12261=VECTOR('',#41976,10.);
#12262=VECTOR('',#41977,10.);
#12263=VECTOR('',#41980,10.);
#12264=VECTOR('',#41981,10.);
#12265=VECTOR('',#41984,10.);
#12266=VECTOR('',#41985,10.);
#12267=VECTOR('',#41994,10.);
#12268=VECTOR('',#41995,10.);
#12269=VECTOR('',#41996,10.);
#12270=VECTOR('',#41999,10.);
#12271=VECTOR('',#42000,10.);
#12272=VECTOR('',#42001,10.);
#12273=VECTOR('',#42004,10.);
#12274=VECTOR('',#42005,10.);
#12275=VECTOR('',#42006,10.);
#12276=VECTOR('',#42009,10.);
#12277=VECTOR('',#42010,10.);
#12278=VECTOR('',#42013,10.);
#12279=VECTOR('',#42014,10.);
#12280=VECTOR('',#42015,10.);
#12281=VECTOR('',#42018,10.);
#12282=VECTOR('',#42019,10.);
#12283=VECTOR('',#42022,10.);
#12284=VECTOR('',#42023,10.);
#12285=VECTOR('',#42026,10.);
#12286=VECTOR('',#42027,10.);
#12287=VECTOR('',#42030,10.);
#12288=VECTOR('',#42031,10.);
#12289=VECTOR('',#42034,10.);
#12290=VECTOR('',#42035,10.);
#12291=VECTOR('',#42038,10.);
#12292=VECTOR('',#42039,10.);
#12293=VECTOR('',#42042,10.);
#12294=VECTOR('',#42043,10.);
#12295=VECTOR('',#42052,10.);
#12296=VECTOR('',#42053,10.);
#12297=VECTOR('',#42054,10.);
#12298=VECTOR('',#42055,10.);
#12299=VECTOR('',#42058,10.);
#12300=VECTOR('',#42059,10.);
#12301=VECTOR('',#42062,10.);
#12302=VECTOR('',#42063,10.);
#12303=VECTOR('',#42064,10.);
#12304=VECTOR('',#42067,10.);
#12305=VECTOR('',#42068,10.);
#12306=VECTOR('',#42069,10.);
#12307=VECTOR('',#42072,10.);
#12308=VECTOR('',#42073,10.);
#12309=VECTOR('',#42076,10.);
#12310=VECTOR('',#42077,10.);
#12311=VECTOR('',#42080,10.);
#12312=VECTOR('',#42081,10.);
#12313=VECTOR('',#42084,10.);
#12314=VECTOR('',#42085,10.);
#12315=VECTOR('',#42086,10.);
#12316=VECTOR('',#42089,10.);
#12317=VECTOR('',#42090,10.);
#12318=VECTOR('',#42093,10.);
#12319=VECTOR('',#42094,10.);
#12320=VECTOR('',#42097,10.);
#12321=VECTOR('',#42098,10.);
#12322=VECTOR('',#42101,10.);
#12323=VECTOR('',#42108,10.);
#12324=VECTOR('',#42109,10.);
#12325=VECTOR('',#42110,10.);
#12326=VECTOR('',#42113,10.);
#12327=VECTOR('',#42114,10.);
#12328=VECTOR('',#42115,10.);
#12329=VECTOR('',#42118,10.);
#12330=VECTOR('',#42119,10.);
#12331=VECTOR('',#42120,10.);
#12332=VECTOR('',#42123,10.);
#12333=VECTOR('',#42124,10.);
#12334=VECTOR('',#42127,10.);
#12335=VECTOR('',#42128,10.);
#12336=VECTOR('',#42129,10.);
#12337=VECTOR('',#42132,10.);
#12338=VECTOR('',#42133,10.);
#12339=VECTOR('',#42136,10.);
#12340=VECTOR('',#42137,10.);
#12341=VECTOR('',#42140,10.);
#12342=VECTOR('',#42141,10.);
#12343=VECTOR('',#42144,10.);
#12344=VECTOR('',#42145,10.);
#12345=VECTOR('',#42148,10.);
#12346=VECTOR('',#42149,10.);
#12347=VECTOR('',#42152,10.);
#12348=VECTOR('',#42153,10.);
#12349=VECTOR('',#42156,10.);
#12350=VECTOR('',#42157,10.);
#12351=VECTOR('',#42166,10.);
#12352=VECTOR('',#42167,10.);
#12353=VECTOR('',#42168,10.);
#12354=VECTOR('',#42171,10.);
#12355=VECTOR('',#42172,10.);
#12356=VECTOR('',#42173,10.);
#12357=VECTOR('',#42174,10.);
#12358=VECTOR('',#42177,10.);
#12359=VECTOR('',#42178,10.);
#12360=VECTOR('',#42181,10.);
#12361=VECTOR('',#42182,10.);
#12362=VECTOR('',#42183,10.);
#12363=VECTOR('',#42186,10.);
#12364=VECTOR('',#42187,10.);
#12365=VECTOR('',#42188,10.);
#12366=VECTOR('',#42189,10.);
#12367=VECTOR('',#42192,10.);
#12368=VECTOR('',#42193,10.);
#12369=VECTOR('',#42196,10.);
#12370=VECTOR('',#42197,10.);
#12371=VECTOR('',#42200,10.);
#12372=VECTOR('',#42201,10.);
#12373=VECTOR('',#42202,10.);
#12374=VECTOR('',#42205,10.);
#12375=VECTOR('',#42208,10.);
#12376=VECTOR('',#42209,10.);
#12377=VECTOR('',#42212,10.);
#12378=VECTOR('',#42213,10.);
#12379=VECTOR('',#42220,10.);
#12380=VECTOR('',#42221,10.);
#12381=VECTOR('',#42222,10.);
#12382=VECTOR('',#42225,10.);
#12383=VECTOR('',#42226,10.);
#12384=VECTOR('',#42227,10.);
#12385=VECTOR('',#42230,10.);
#12386=VECTOR('',#42231,10.);
#12387=VECTOR('',#42232,10.);
#12388=VECTOR('',#42235,10.);
#12389=VECTOR('',#42236,10.);
#12390=VECTOR('',#42239,10.);
#12391=VECTOR('',#42240,10.);
#12392=VECTOR('',#42241,10.);
#12393=VECTOR('',#42244,10.);
#12394=VECTOR('',#42245,10.);
#12395=VECTOR('',#42248,10.);
#12396=VECTOR('',#42249,10.);
#12397=VECTOR('',#42252,10.);
#12398=VECTOR('',#42253,10.);
#12399=VECTOR('',#42256,10.);
#12400=VECTOR('',#42257,10.);
#12401=VECTOR('',#42260,10.);
#12402=VECTOR('',#42261,10.);
#12403=VECTOR('',#42264,10.);
#12404=VECTOR('',#42265,10.);
#12405=VECTOR('',#42268,10.);
#12406=VECTOR('',#42269,10.);
#12407=VECTOR('',#42278,10.);
#12408=VECTOR('',#42279,10.);
#12409=VECTOR('',#42280,10.);
#12410=VECTOR('',#42283,10.);
#12411=VECTOR('',#42284,10.);
#12412=VECTOR('',#42285,10.);
#12413=VECTOR('',#42288,10.);
#12414=VECTOR('',#42289,10.);
#12415=VECTOR('',#42290,10.);
#12416=VECTOR('',#42293,10.);
#12417=VECTOR('',#42294,10.);
#12418=VECTOR('',#42297,10.);
#12419=VECTOR('',#42298,10.);
#12420=VECTOR('',#42299,10.);
#12421=VECTOR('',#42302,10.);
#12422=VECTOR('',#42303,10.);
#12423=VECTOR('',#42306,10.);
#12424=VECTOR('',#42307,10.);
#12425=VECTOR('',#42310,10.);
#12426=VECTOR('',#42311,10.);
#12427=VECTOR('',#42314,10.);
#12428=VECTOR('',#42315,10.);
#12429=VECTOR('',#42318,10.);
#12430=VECTOR('',#42319,10.);
#12431=VECTOR('',#42322,10.);
#12432=VECTOR('',#42323,10.);
#12433=VECTOR('',#42326,10.);
#12434=VECTOR('',#42327,10.);
#12435=VECTOR('',#42336,10.);
#12436=VECTOR('',#42337,10.);
#12437=VECTOR('',#42338,10.);
#12438=VECTOR('',#42339,10.);
#12439=VECTOR('',#42342,10.);
#12440=VECTOR('',#42343,10.);
#12441=VECTOR('',#42346,10.);
#12442=VECTOR('',#42347,10.);
#12443=VECTOR('',#42348,10.);
#12444=VECTOR('',#42351,10.);
#12445=VECTOR('',#42352,10.);
#12446=VECTOR('',#42353,10.);
#12447=VECTOR('',#42356,10.);
#12448=VECTOR('',#42357,10.);
#12449=VECTOR('',#42360,10.);
#12450=VECTOR('',#42361,10.);
#12451=VECTOR('',#42364,10.);
#12452=VECTOR('',#42365,10.);
#12453=VECTOR('',#42368,10.);
#12454=VECTOR('',#42369,10.);
#12455=VECTOR('',#42370,10.);
#12456=VECTOR('',#42373,10.);
#12457=VECTOR('',#42374,10.);
#12458=VECTOR('',#42377,10.);
#12459=VECTOR('',#42378,10.);
#12460=VECTOR('',#42381,10.);
#12461=VECTOR('',#42382,10.);
#12462=VECTOR('',#42385,10.);
#12463=VECTOR('',#42392,10.);
#12464=VECTOR('',#42393,10.);
#12465=VECTOR('',#42394,10.);
#12466=VECTOR('',#42397,10.);
#12467=VECTOR('',#42398,10.);
#12468=VECTOR('',#42399,10.);
#12469=VECTOR('',#42402,10.);
#12470=VECTOR('',#42403,10.);
#12471=VECTOR('',#42404,10.);
#12472=VECTOR('',#42407,10.);
#12473=VECTOR('',#42408,10.);
#12474=VECTOR('',#42411,10.);
#12475=VECTOR('',#42412,10.);
#12476=VECTOR('',#42413,10.);
#12477=VECTOR('',#42416,10.);
#12478=VECTOR('',#42417,10.);
#12479=VECTOR('',#42420,10.);
#12480=VECTOR('',#42421,10.);
#12481=VECTOR('',#42424,10.);
#12482=VECTOR('',#42425,10.);
#12483=VECTOR('',#42428,10.);
#12484=VECTOR('',#42429,10.);
#12485=VECTOR('',#42432,10.);
#12486=VECTOR('',#42433,10.);
#12487=VECTOR('',#42436,10.);
#12488=VECTOR('',#42437,10.);
#12489=VECTOR('',#42440,10.);
#12490=VECTOR('',#42441,10.);
#12491=VECTOR('',#42450,10.);
#12492=VECTOR('',#42451,10.);
#12493=VECTOR('',#42452,10.);
#12494=VECTOR('',#42455,10.);
#12495=VECTOR('',#42456,10.);
#12496=VECTOR('',#42457,10.);
#12497=VECTOR('',#42458,10.);
#12498=VECTOR('',#42461,10.);
#12499=VECTOR('',#42462,10.);
#12500=VECTOR('',#42465,10.);
#12501=VECTOR('',#42466,10.);
#12502=VECTOR('',#42467,10.);
#12503=VECTOR('',#42470,10.);
#12504=VECTOR('',#42471,10.);
#12505=VECTOR('',#42472,10.);
#12506=VECTOR('',#42473,10.);
#12507=VECTOR('',#42476,10.);
#12508=VECTOR('',#42477,10.);
#12509=VECTOR('',#42480,10.);
#12510=VECTOR('',#42481,10.);
#12511=VECTOR('',#42484,10.);
#12512=VECTOR('',#42485,10.);
#12513=VECTOR('',#42486,10.);
#12514=VECTOR('',#42489,10.);
#12515=VECTOR('',#42492,10.);
#12516=VECTOR('',#42493,10.);
#12517=VECTOR('',#42496,10.);
#12518=VECTOR('',#42497,10.);
#12519=VECTOR('',#42504,10.);
#12520=VECTOR('',#42505,10.);
#12521=VECTOR('',#42506,10.);
#12522=VECTOR('',#42509,10.);
#12523=VECTOR('',#42510,10.);
#12524=VECTOR('',#42511,10.);
#12525=VECTOR('',#42514,10.);
#12526=VECTOR('',#42515,10.);
#12527=VECTOR('',#42516,10.);
#12528=VECTOR('',#42519,10.);
#12529=VECTOR('',#42520,10.);
#12530=VECTOR('',#42523,10.);
#12531=VECTOR('',#42524,10.);
#12532=VECTOR('',#42525,10.);
#12533=VECTOR('',#42528,10.);
#12534=VECTOR('',#42529,10.);
#12535=VECTOR('',#42532,10.);
#12536=VECTOR('',#42533,10.);
#12537=VECTOR('',#42536,10.);
#12538=VECTOR('',#42537,10.);
#12539=VECTOR('',#42540,10.);
#12540=VECTOR('',#42541,10.);
#12541=VECTOR('',#42544,10.);
#12542=VECTOR('',#42545,10.);
#12543=VECTOR('',#42548,10.);
#12544=VECTOR('',#42549,10.);
#12545=VECTOR('',#42552,10.);
#12546=VECTOR('',#42553,10.);
#12547=VECTOR('',#42562,10.);
#12548=VECTOR('',#42563,10.);
#12549=VECTOR('',#42564,10.);
#12550=VECTOR('',#42567,10.);
#12551=VECTOR('',#42568,10.);
#12552=VECTOR('',#42569,10.);
#12553=VECTOR('',#42572,10.);
#12554=VECTOR('',#42573,10.);
#12555=VECTOR('',#42574,10.);
#12556=VECTOR('',#42577,10.);
#12557=VECTOR('',#42578,10.);
#12558=VECTOR('',#42581,10.);
#12559=VECTOR('',#42582,10.);
#12560=VECTOR('',#42583,10.);
#12561=VECTOR('',#42586,10.);
#12562=VECTOR('',#42587,10.);
#12563=VECTOR('',#42590,10.);
#12564=VECTOR('',#42591,10.);
#12565=VECTOR('',#42594,10.);
#12566=VECTOR('',#42595,10.);
#12567=VECTOR('',#42598,10.);
#12568=VECTOR('',#42599,10.);
#12569=VECTOR('',#42602,10.);
#12570=VECTOR('',#42603,10.);
#12571=VECTOR('',#42606,10.);
#12572=VECTOR('',#42607,10.);
#12573=VECTOR('',#42610,10.);
#12574=VECTOR('',#42611,10.);
#12575=VECTOR('',#42620,10.);
#12576=VECTOR('',#42621,10.);
#12577=VECTOR('',#42622,10.);
#12578=VECTOR('',#42623,10.);
#12579=VECTOR('',#42626,10.);
#12580=VECTOR('',#42627,10.);
#12581=VECTOR('',#42630,10.);
#12582=VECTOR('',#42631,10.);
#12583=VECTOR('',#42632,10.);
#12584=VECTOR('',#42635,10.);
#12585=VECTOR('',#42636,10.);
#12586=VECTOR('',#42637,10.);
#12587=VECTOR('',#42640,10.);
#12588=VECTOR('',#42641,10.);
#12589=VECTOR('',#42644,10.);
#12590=VECTOR('',#42645,10.);
#12591=VECTOR('',#42648,10.);
#12592=VECTOR('',#42649,10.);
#12593=VECTOR('',#42652,10.);
#12594=VECTOR('',#42653,10.);
#12595=VECTOR('',#42654,10.);
#12596=VECTOR('',#42657,10.);
#12597=VECTOR('',#42658,10.);
#12598=VECTOR('',#42661,10.);
#12599=VECTOR('',#42662,10.);
#12600=VECTOR('',#42665,10.);
#12601=VECTOR('',#42666,10.);
#12602=VECTOR('',#42669,10.);
#12603=VECTOR('',#42676,10.);
#12604=VECTOR('',#42677,10.);
#12605=VECTOR('',#42678,10.);
#12606=VECTOR('',#42681,10.);
#12607=VECTOR('',#42682,10.);
#12608=VECTOR('',#42683,10.);
#12609=VECTOR('',#42686,10.);
#12610=VECTOR('',#42687,10.);
#12611=VECTOR('',#42688,10.);
#12612=VECTOR('',#42691,10.);
#12613=VECTOR('',#42692,10.);
#12614=VECTOR('',#42695,10.);
#12615=VECTOR('',#42696,10.);
#12616=VECTOR('',#42697,10.);
#12617=VECTOR('',#42700,10.);
#12618=VECTOR('',#42701,10.);
#12619=VECTOR('',#42704,10.);
#12620=VECTOR('',#42705,10.);
#12621=VECTOR('',#42708,10.);
#12622=VECTOR('',#42709,10.);
#12623=VECTOR('',#42712,10.);
#12624=VECTOR('',#42713,10.);
#12625=VECTOR('',#42716,10.);
#12626=VECTOR('',#42717,10.);
#12627=VECTOR('',#42720,10.);
#12628=VECTOR('',#42721,10.);
#12629=VECTOR('',#42724,10.);
#12630=VECTOR('',#42725,10.);
#12631=VECTOR('',#42734,10.);
#12632=VECTOR('',#42735,10.);
#12633=VECTOR('',#42736,10.);
#12634=VECTOR('',#42739,10.);
#12635=VECTOR('',#42740,10.);
#12636=VECTOR('',#42741,10.);
#12637=VECTOR('',#42742,10.);
#12638=VECTOR('',#42745,10.);
#12639=VECTOR('',#42746,10.);
#12640=VECTOR('',#42749,10.);
#12641=VECTOR('',#42750,10.);
#12642=VECTOR('',#42751,10.);
#12643=VECTOR('',#42754,10.);
#12644=VECTOR('',#42755,10.);
#12645=VECTOR('',#42756,10.);
#12646=VECTOR('',#42757,10.);
#12647=VECTOR('',#42760,10.);
#12648=VECTOR('',#42761,10.);
#12649=VECTOR('',#42764,10.);
#12650=VECTOR('',#42765,10.);
#12651=VECTOR('',#42768,10.);
#12652=VECTOR('',#42769,10.);
#12653=VECTOR('',#42770,10.);
#12654=VECTOR('',#42773,10.);
#12655=VECTOR('',#42776,10.);
#12656=VECTOR('',#42777,10.);
#12657=VECTOR('',#42780,10.);
#12658=VECTOR('',#42781,10.);
#12659=VECTOR('',#42788,10.);
#12660=VECTOR('',#42789,10.);
#12661=VECTOR('',#42790,10.);
#12662=VECTOR('',#42793,10.);
#12663=VECTOR('',#42794,10.);
#12664=VECTOR('',#42795,10.);
#12665=VECTOR('',#42798,10.);
#12666=VECTOR('',#42799,10.);
#12667=VECTOR('',#42800,10.);
#12668=VECTOR('',#42803,10.);
#12669=VECTOR('',#42804,10.);
#12670=VECTOR('',#42807,10.);
#12671=VECTOR('',#42808,10.);
#12672=VECTOR('',#42809,10.);
#12673=VECTOR('',#42812,10.);
#12674=VECTOR('',#42813,10.);
#12675=VECTOR('',#42816,10.);
#12676=VECTOR('',#42817,10.);
#12677=VECTOR('',#42820,10.);
#12678=VECTOR('',#42821,10.);
#12679=VECTOR('',#42824,10.);
#12680=VECTOR('',#42825,10.);
#12681=VECTOR('',#42828,10.);
#12682=VECTOR('',#42829,10.);
#12683=VECTOR('',#42832,10.);
#12684=VECTOR('',#42833,10.);
#12685=VECTOR('',#42836,10.);
#12686=VECTOR('',#42837,10.);
#12687=VECTOR('',#42846,10.);
#12688=VECTOR('',#42847,10.);
#12689=VECTOR('',#42848,10.);
#12690=VECTOR('',#42851,10.);
#12691=VECTOR('',#42852,10.);
#12692=VECTOR('',#42853,10.);
#12693=VECTOR('',#42856,10.);
#12694=VECTOR('',#42857,10.);
#12695=VECTOR('',#42858,10.);
#12696=VECTOR('',#42861,10.);
#12697=VECTOR('',#42862,10.);
#12698=VECTOR('',#42865,10.);
#12699=VECTOR('',#42866,10.);
#12700=VECTOR('',#42867,10.);
#12701=VECTOR('',#42870,10.);
#12702=VECTOR('',#42871,10.);
#12703=VECTOR('',#42874,10.);
#12704=VECTOR('',#42875,10.);
#12705=VECTOR('',#42878,10.);
#12706=VECTOR('',#42879,10.);
#12707=VECTOR('',#42882,10.);
#12708=VECTOR('',#42883,10.);
#12709=VECTOR('',#42886,10.);
#12710=VECTOR('',#42887,10.);
#12711=VECTOR('',#42890,10.);
#12712=VECTOR('',#42891,10.);
#12713=VECTOR('',#42894,10.);
#12714=VECTOR('',#42895,10.);
#12715=VECTOR('',#42908,127.185823536562);
#12716=VECTOR('',#42915,128.);
#12717=VECTOR('',#42924,127.);
#12718=VECTOR('',#42927,10.);
#12719=VECTOR('',#42928,10.);
#12720=VECTOR('',#42929,10.);
#12721=VECTOR('',#42932,10.);
#12722=VECTOR('',#42933,10.);
#12723=VECTOR('',#42934,10.);
#12724=VECTOR('',#42937,10.);
#12725=VECTOR('',#42938,10.);
#12726=VECTOR('',#42939,10.);
#12727=VECTOR('',#42942,10.);
#12728=VECTOR('',#42943,10.);
#12729=VECTOR('',#42946,10.);
#12730=VECTOR('',#42947,10.);
#12731=VECTOR('',#42948,10.);
#12732=VECTOR('',#42951,10.);
#12733=VECTOR('',#42952,10.);
#12734=VECTOR('',#42955,10.);
#12735=VECTOR('',#42956,10.);
#12736=VECTOR('',#42959,10.);
#12737=VECTOR('',#42960,10.);
#12738=VECTOR('',#42963,10.);
#12739=VECTOR('',#42964,10.);
#12740=VECTOR('',#42967,10.);
#12741=VECTOR('',#42968,10.);
#12742=VECTOR('',#42971,10.);
#12743=VECTOR('',#42972,10.);
#12744=VECTOR('',#42975,10.);
#12745=VECTOR('',#42976,10.);
#12746=VECTOR('',#42985,10.);
#12747=VECTOR('',#42986,10.);
#12748=VECTOR('',#42987,10.);
#12749=VECTOR('',#42990,10.);
#12750=VECTOR('',#42991,10.);
#12751=VECTOR('',#42992,10.);
#12752=VECTOR('',#42995,10.);
#12753=VECTOR('',#42996,10.);
#12754=VECTOR('',#42997,10.);
#12755=VECTOR('',#43000,10.);
#12756=VECTOR('',#43001,10.);
#12757=VECTOR('',#43004,10.);
#12758=VECTOR('',#43005,10.);
#12759=VECTOR('',#43006,10.);
#12760=VECTOR('',#43009,10.);
#12761=VECTOR('',#43010,10.);
#12762=VECTOR('',#43013,10.);
#12763=VECTOR('',#43014,10.);
#12764=VECTOR('',#43017,10.);
#12765=VECTOR('',#43018,10.);
#12766=VECTOR('',#43021,10.);
#12767=VECTOR('',#43022,10.);
#12768=VECTOR('',#43025,10.);
#12769=VECTOR('',#43026,10.);
#12770=VECTOR('',#43029,10.);
#12771=VECTOR('',#43030,10.);
#12772=VECTOR('',#43033,10.);
#12773=VECTOR('',#43034,10.);
#12774=VECTOR('',#43047,138.753401519042);
#12775=VECTOR('',#43054,139.);
#12776=VECTOR('',#43061,137.5);
#12777=VECTOR('',#43066,129.064176463438);
#12778=VECTOR('',#43075,138.823223304703);
#12779=VECTOR('',#43078,138.5);
#12780=VECTOR('',#43083,137.926776695297);
#12781=VECTOR('',#43374,7.18);
#12782=VECTOR('',#43379,7.18);
#12783=VECTOR('',#43384,7.18);
#12784=VECTOR('',#43389,7.18);
#12785=VECTOR('',#43394,7.18);
#12786=VECTOR('',#43401,25.);
#12787=VECTOR('',#43406,23.);
#12788=VECTOR('',#43411,10.);
#12789=VECTOR('',#43416,10.);
#12790=VECTOR('',#43421,10.);
#12791=VECTOR('',#43432,25.16);
#12792=VECTOR('',#43439,27.);
#12793=VECTOR('',#43446,29.58);
#12794=VECTOR('',#43455,32.6);
#12795=VECTOR('',#43460,32.9);
#12796=VECTOR('',#43465,43.);
#12797=VECTOR('',#43472,124.75);
#12798=VECTOR('',#43477,126.75);
#13634=CIRCLE('',#34368,40.);
#13635=CIRCLE('',#34369,40.);
#13636=CIRCLE('',#34370,39.5527864045);
#13637=CIRCLE('',#34371,39.5527864045);
#13638=CIRCLE('',#34373,37.4472135955);
#13639=CIRCLE('',#34374,37.4472135955);
#13640=CIRCLE('',#34376,40.);
#13641=CIRCLE('',#34378,36.5);
#13642=CIRCLE('',#34380,33.2);
#13643=CIRCLE('',#34382,26.5);
#13644=CIRCLE('',#34383,26.);
#13645=CIRCLE('',#34384,26.);
#13646=CIRCLE('',#34386,26.);
#13647=CIRCLE('',#34388,29.58);
#13648=CIRCLE('',#34390,31.5);
#13649=CIRCLE('',#34391,32.3535533905933);
#13650=CIRCLE('',#34392,32.3535533905933);
#13651=CIRCLE('',#34394,33.6464466094067);
#13652=CIRCLE('',#34395,33.6464466094067);
#13653=CIRCLE('',#34397,25.16);
#13654=CIRCLE('',#34399,34.0540295903842);
#13655=CIRCLE('',#34400,34.0540295903842);
#13656=CIRCLE('',#34402,36.5);
#13657=CIRCLE('',#34404,126.506803038084);
#13658=CIRCLE('',#34405,126.506803038084);
#13659=CIRCLE('',#34406,127.416025147169);
#13660=CIRCLE('',#34407,127.416025147169);
#13661=CIRCLE('',#34409,131.083974852831);
#13662=CIRCLE('',#34410,131.083974852831);
#13663=CIRCLE('',#34412,121.);
#13664=CIRCLE('',#34414,131.8);
#13665=CIRCLE('',#34415,131.8);
#13666=CIRCLE('',#34417,134.2);
#13667=CIRCLE('',#34418,134.2);
#13668=CIRCLE('',#34420,134.675561720794);
#13669=CIRCLE('',#34421,134.675561720794);
#13670=CIRCLE('',#34423,135.824438279206);
#13671=CIRCLE('',#34424,135.824438279206);
#13672=CIRCLE('',#34426,136.);
#13673=CIRCLE('',#34427,136.);
#13674=CIRCLE('',#34429,136.);
#13675=CIRCLE('',#34432,136.);
#13676=CIRCLE('',#34433,136.);
#13677=CIRCLE('',#34434,136.);
#13678=CIRCLE('',#34437,136.);
#13679=CIRCLE('',#34439,136.);
#13680=CIRCLE('',#34442,136.);
#13681=CIRCLE('',#34445,136.);
#13682=CIRCLE('',#34448,136.);
#13683=CIRCLE('',#34451,136.);
#13684=CIRCLE('',#34454,136.);
#13685=CIRCLE('',#34457,136.);
#13686=CIRCLE('',#34460,136.);
#13687=CIRCLE('',#34463,136.);
#13688=CIRCLE('',#34466,136.);
#13689=CIRCLE('',#34469,136.);
#13690=CIRCLE('',#34472,136.);
#13691=CIRCLE('',#34475,136.);
#13692=CIRCLE('',#34478,136.);
#13693=CIRCLE('',#34481,136.);
#13694=CIRCLE('',#34484,136.);
#13695=CIRCLE('',#34487,136.);
#13696=CIRCLE('',#34490,136.);
#13697=CIRCLE('',#34493,136.);
#13698=CIRCLE('',#34496,136.);
#13699=CIRCLE('',#34499,136.);
#13700=CIRCLE('',#34502,136.);
#13701=CIRCLE('',#34505,136.);
#13702=CIRCLE('',#34508,136.);
#13703=CIRCLE('',#34511,136.);
#13704=CIRCLE('',#34514,136.);
#13705=CIRCLE('',#34517,136.);
#13706=CIRCLE('',#34520,136.);
#13707=CIRCLE('',#34523,136.);
#13708=CIRCLE('',#34526,136.);
#13709=CIRCLE('',#34529,136.);
#13710=CIRCLE('',#34532,136.);
#13711=CIRCLE('',#34535,136.);
#13712=CIRCLE('',#34538,136.);
#13713=CIRCLE('',#34541,136.);
#13714=CIRCLE('',#34544,136.);
#13715=CIRCLE('',#34547,136.);
#13716=CIRCLE('',#34550,136.);
#13717=CIRCLE('',#34553,136.);
#13718=CIRCLE('',#34556,136.);
#13719=CIRCLE('',#34559,136.);
#13720=CIRCLE('',#34562,136.);
#13721=CIRCLE('',#34565,136.);
#13722=CIRCLE('',#34568,136.);
#13723=CIRCLE('',#34571,136.);
#13724=CIRCLE('',#34574,136.);
#13725=CIRCLE('',#34577,136.);
#13726=CIRCLE('',#34580,136.);
#13727=CIRCLE('',#34583,136.);
#13728=CIRCLE('',#34586,136.);
#13729=CIRCLE('',#34589,136.);
#13730=CIRCLE('',#34592,136.);
#13731=CIRCLE('',#34595,136.);
#13732=CIRCLE('',#34598,136.);
#13733=CIRCLE('',#34601,136.);
#13734=CIRCLE('',#34604,136.);
#13735=CIRCLE('',#34607,136.);
#13736=CIRCLE('',#34610,136.);
#13737=CIRCLE('',#34613,136.);
#13738=CIRCLE('',#34616,136.);
#13739=CIRCLE('',#34619,136.);
#13740=CIRCLE('',#34622,136.);
#13741=CIRCLE('',#34625,136.);
#13742=CIRCLE('',#34628,136.);
#13743=CIRCLE('',#34631,136.);
#13744=CIRCLE('',#34634,136.);
#13745=CIRCLE('',#34637,136.);
#13746=CIRCLE('',#34640,136.);
#13747=CIRCLE('',#34643,136.);
#13748=CIRCLE('',#34646,136.);
#13749=CIRCLE('',#34649,136.);
#13750=CIRCLE('',#34652,136.);
#13751=CIRCLE('',#34655,136.);
#13752=CIRCLE('',#34658,136.);
#13753=CIRCLE('',#34661,136.);
#13754=CIRCLE('',#34664,136.);
#13755=CIRCLE('',#34667,136.);
#13756=CIRCLE('',#34670,136.);
#13757=CIRCLE('',#34673,136.);
#13758=CIRCLE('',#34676,136.);
#13759=CIRCLE('',#34679,136.);
#13760=CIRCLE('',#34682,136.);
#13761=CIRCLE('',#34685,136.);
#13762=CIRCLE('',#34688,136.);
#13763=CIRCLE('',#34691,136.);
#13764=CIRCLE('',#34694,136.);
#13765=CIRCLE('',#34697,136.);
#13766=CIRCLE('',#34700,136.);
#13767=CIRCLE('',#34703,136.);
#13768=CIRCLE('',#34706,136.);
#13769=CIRCLE('',#34709,136.);
#13770=CIRCLE('',#34712,136.);
#13771=CIRCLE('',#34715,136.);
#13772=CIRCLE('',#34718,136.);
#13773=CIRCLE('',#34721,136.);
#13774=CIRCLE('',#34724,136.);
#13775=CIRCLE('',#34727,136.);
#13776=CIRCLE('',#34730,136.);
#13777=CIRCLE('',#34733,136.);
#13778=CIRCLE('',#34736,136.);
#13779=CIRCLE('',#34739,136.);
#13780=CIRCLE('',#34742,136.);
#13781=CIRCLE('',#34745,136.);
#13782=CIRCLE('',#34748,136.);
#13783=CIRCLE('',#34751,136.);
#13784=CIRCLE('',#34754,136.);
#13785=CIRCLE('',#34757,136.);
#13786=CIRCLE('',#34760,136.);
#13787=CIRCLE('',#34763,136.);
#13788=CIRCLE('',#34766,136.);
#13789=CIRCLE('',#34769,136.);
#13790=CIRCLE('',#34772,136.);
#13791=CIRCLE('',#34775,136.);
#13792=CIRCLE('',#34778,136.);
#13793=CIRCLE('',#34781,136.);
#13794=CIRCLE('',#34784,136.);
#13795=CIRCLE('',#34787,136.);
#13796=CIRCLE('',#34790,136.);
#13797=CIRCLE('',#34793,136.);
#13798=CIRCLE('',#34796,136.);
#13799=CIRCLE('',#34799,136.);
#13800=CIRCLE('',#34802,136.);
#13801=CIRCLE('',#34805,136.);
#13802=CIRCLE('',#34808,136.);
#13803=CIRCLE('',#34811,136.);
#13804=CIRCLE('',#34814,136.);
#13805=CIRCLE('',#34817,136.);
#13806=CIRCLE('',#34820,136.);
#13807=CIRCLE('',#34823,136.);
#13808=CIRCLE('',#34826,136.);
#13809=CIRCLE('',#34829,136.);
#13810=CIRCLE('',#34832,136.);
#13811=CIRCLE('',#34835,136.);
#13812=CIRCLE('',#34838,136.);
#13813=CIRCLE('',#34841,136.);
#13814=CIRCLE('',#34844,136.);
#13815=CIRCLE('',#34847,136.);
#13816=CIRCLE('',#34850,136.);
#13817=CIRCLE('',#34853,136.);
#13818=CIRCLE('',#34856,136.);
#13819=CIRCLE('',#34859,136.);
#13820=CIRCLE('',#34862,136.);
#13821=CIRCLE('',#34865,51.5);
#13822=CIRCLE('',#34866,52.);
#13823=CIRCLE('',#34868,14.5);
#13824=CIRCLE('',#34869,15.);
#13825=CIRCLE('',#34871,51.5);
#13826=CIRCLE('',#34872,52.);
#13827=CIRCLE('',#34874,14.5);
#13828=CIRCLE('',#34875,15.);
#13829=CIRCLE('',#34877,51.5);
#13830=CIRCLE('',#34878,52.);
#13831=CIRCLE('',#34880,14.5);
#13832=CIRCLE('',#34881,15.);
#13833=CIRCLE('',#34883,52.);
#13834=CIRCLE('',#34884,51.5);
#13835=CIRCLE('',#34886,15.);
#13836=CIRCLE('',#34887,14.5);
#13837=CIRCLE('',#34889,52.);
#13838=CIRCLE('',#34890,51.5);
#13839=CIRCLE('',#34892,15.);
#13840=CIRCLE('',#34893,14.5);
#13841=CIRCLE('',#34895,15.);
#13842=CIRCLE('',#34897,52.);
#13843=CIRCLE('',#34899,15.);
#13844=CIRCLE('',#34901,52.);
#13845=CIRCLE('',#34903,15.);
#13846=CIRCLE('',#34905,52.);
#13847=CIRCLE('',#34907,7.18);
#13848=CIRCLE('',#34908,7.18);
#13849=CIRCLE('',#34909,7.18);
#13850=CIRCLE('',#34910,7.18);
#13851=CIRCLE('',#34911,7.18);
#13852=CIRCLE('',#35921,127.371647073124);
#13853=CIRCLE('',#35922,127.371647073124);
#13854=CIRCLE('',#35923,127.);
#13855=CIRCLE('',#35924,127.);
#13856=CIRCLE('',#35926,128.628352926876);
#13857=CIRCLE('',#35927,128.628352926876);
#13858=CIRCLE('',#35929,127.);
#13859=CIRCLE('',#35961,138.506803038084);
#13860=CIRCLE('',#35962,138.506803038084);
#13861=CIRCLE('',#35963,139.);
#13862=CIRCLE('',#35964,139.);
#13863=CIRCLE('',#35966,139.);
#13864=CIRCLE('',#35967,139.);
#13865=CIRCLE('',#35970,129.5);
#13866=CIRCLE('',#35972,137.5);
#13867=CIRCLE('',#35974,138.646446609407);
#13868=CIRCLE('',#35976,138.353553390593);
#13869=CIRCLE('',#36123,7.18);
#13870=CIRCLE('',#36125,7.18);
#13871=CIRCLE('',#36127,7.18);
#13872=CIRCLE('',#36129,7.18);
#13873=CIRCLE('',#36131,7.18);
#13874=CIRCLE('',#36133,27.);
#13875=CIRCLE('',#36134,23.);
#13876=CIRCLE('',#36136,23.);
#13877=CIRCLE('',#36138,15.);
#13878=CIRCLE('',#36140,52.);
#13879=CIRCLE('',#36142,15.);
#13880=CIRCLE('',#36144,52.);
#13881=CIRCLE('',#36147,25.16);
#13882=CIRCLE('',#36150,27.);
#13883=CIRCLE('',#36153,29.58);
#13884=CIRCLE('',#36155,32.6);
#13885=CIRCLE('',#36157,32.6);
#13886=CIRCLE('',#36160,46.);
#13887=CIRCLE('',#36162,123.);
#13888=CIRCLE('',#36164,126.5);
#14532=VERTEX_POINT('',#47306);
#14533=VERTEX_POINT('',#47307);
#14534=VERTEX_POINT('',#47310);
#14535=VERTEX_POINT('',#47312);
#14536=VERTEX_POINT('',#47316);
#14537=VERTEX_POINT('',#47318);
#14538=VERTEX_POINT('',#47322);
#14539=VERTEX_POINT('',#47326);
#14540=VERTEX_POINT('',#47330);
#14541=VERTEX_POINT('',#47333);
#14542=VERTEX_POINT('',#47335);
#14543=VERTEX_POINT('',#47337);
#14544=VERTEX_POINT('',#47341);
#14545=VERTEX_POINT('',#47345);
#14546=VERTEX_POINT('',#47348);
#14547=VERTEX_POINT('',#47350);
#14548=VERTEX_POINT('',#47352);
#14549=VERTEX_POINT('',#47356);
#14550=VERTEX_POINT('',#47358);
#14551=VERTEX_POINT('',#47362);
#14552=VERTEX_POINT('',#47365);
#14553=VERTEX_POINT('',#47367);
#14554=VERTEX_POINT('',#47371);
#14555=VERTEX_POINT('',#47375);
#14556=VERTEX_POINT('',#47376);
#14557=VERTEX_POINT('',#47379);
#14558=VERTEX_POINT('',#47381);
#14559=VERTEX_POINT('',#47385);
#14560=VERTEX_POINT('',#47387);
#14561=VERTEX_POINT('',#47391);
#14562=VERTEX_POINT('',#47395);
#14563=VERTEX_POINT('',#47397);
#14564=VERTEX_POINT('',#47401);
#14565=VERTEX_POINT('',#47403);
#14566=VERTEX_POINT('',#47407);
#14567=VERTEX_POINT('',#47409);
#14568=VERTEX_POINT('',#47413);
#14569=VERTEX_POINT('',#47415);
#14570=VERTEX_POINT('',#47419);
#14571=VERTEX_POINT('',#47421);
#14572=VERTEX_POINT('',#47425);
#14573=VERTEX_POINT('',#47427);
#14574=VERTEX_POINT('',#47429);
#14575=VERTEX_POINT('',#47431);
#14576=VERTEX_POINT('',#47433);
#14577=VERTEX_POINT('',#47435);
#14578=VERTEX_POINT('',#47437);
#14579=VERTEX_POINT('',#47440);
#14580=VERTEX_POINT('',#47442);
#14581=VERTEX_POINT('',#47444);
#14582=VERTEX_POINT('',#47446);
#14583=VERTEX_POINT('',#47449);
#14584=VERTEX_POINT('',#47450);
#14585=VERTEX_POINT('',#47452);
#14586=VERTEX_POINT('',#47454);
#14587=VERTEX_POINT('',#47456);
#14588=VERTEX_POINT('',#47458);
#14589=VERTEX_POINT('',#47460);
#14590=VERTEX_POINT('',#47462);
#14591=VERTEX_POINT('',#47465);
#14592=VERTEX_POINT('',#47466);
#14593=VERTEX_POINT('',#47468);
#14594=VERTEX_POINT('',#47470);
#14595=VERTEX_POINT('',#47472);
#14596=VERTEX_POINT('',#47474);
#14597=VERTEX_POINT('',#47476);
#14598=VERTEX_POINT('',#47478);
#14599=VERTEX_POINT('',#47481);
#14600=VERTEX_POINT('',#47482);
#14601=VERTEX_POINT('',#47484);
#14602=VERTEX_POINT('',#47486);
#14603=VERTEX_POINT('',#47488);
#14604=VERTEX_POINT('',#47490);
#14605=VERTEX_POINT('',#47492);
#14606=VERTEX_POINT('',#47494);
#14607=VERTEX_POINT('',#47497);
#14608=VERTEX_POINT('',#47498);
#14609=VERTEX_POINT('',#47500);
#14610=VERTEX_POINT('',#47502);
#14611=VERTEX_POINT('',#47504);
#14612=VERTEX_POINT('',#47506);
#14613=VERTEX_POINT('',#47508);
#14614=VERTEX_POINT('',#47510);
#14615=VERTEX_POINT('',#47513);
#14616=VERTEX_POINT('',#47514);
#14617=VERTEX_POINT('',#47516);
#14618=VERTEX_POINT('',#47518);
#14619=VERTEX_POINT('',#47520);
#14620=VERTEX_POINT('',#47522);
#14621=VERTEX_POINT('',#47524);
#14622=VERTEX_POINT('',#47526);
#14623=VERTEX_POINT('',#47529);
#14624=VERTEX_POINT('',#47530);
#14625=VERTEX_POINT('',#47532);
#14626=VERTEX_POINT('',#47534);
#14627=VERTEX_POINT('',#47536);
#14628=VERTEX_POINT('',#47538);
#14629=VERTEX_POINT('',#47540);
#14630=VERTEX_POINT('',#47542);
#14631=VERTEX_POINT('',#47545);
#14632=VERTEX_POINT('',#47546);
#14633=VERTEX_POINT('',#47548);
#14634=VERTEX_POINT('',#47550);
#14635=VERTEX_POINT('',#47552);
#14636=VERTEX_POINT('',#47554);
#14637=VERTEX_POINT('',#47556);
#14638=VERTEX_POINT('',#47558);
#14639=VERTEX_POINT('',#47561);
#14640=VERTEX_POINT('',#47562);
#14641=VERTEX_POINT('',#47564);
#14642=VERTEX_POINT('',#47566);
#14643=VERTEX_POINT('',#47568);
#14644=VERTEX_POINT('',#47570);
#14645=VERTEX_POINT('',#47572);
#14646=VERTEX_POINT('',#47574);
#14647=VERTEX_POINT('',#47577);
#14648=VERTEX_POINT('',#47578);
#14649=VERTEX_POINT('',#47580);
#14650=VERTEX_POINT('',#47582);
#14651=VERTEX_POINT('',#47584);
#14652=VERTEX_POINT('',#47586);
#14653=VERTEX_POINT('',#47588);
#14654=VERTEX_POINT('',#47590);
#14655=VERTEX_POINT('',#47593);
#14656=VERTEX_POINT('',#47594);
#14657=VERTEX_POINT('',#47596);
#14658=VERTEX_POINT('',#47598);
#14659=VERTEX_POINT('',#47600);
#14660=VERTEX_POINT('',#47602);
#14661=VERTEX_POINT('',#47604);
#14662=VERTEX_POINT('',#47606);
#14663=VERTEX_POINT('',#47609);
#14664=VERTEX_POINT('',#47610);
#14665=VERTEX_POINT('',#47612);
#14666=VERTEX_POINT('',#47614);
#14667=VERTEX_POINT('',#47616);
#14668=VERTEX_POINT('',#47618);
#14669=VERTEX_POINT('',#47620);
#14670=VERTEX_POINT('',#47622);
#14671=VERTEX_POINT('',#47625);
#14672=VERTEX_POINT('',#47626);
#14673=VERTEX_POINT('',#47628);
#14674=VERTEX_POINT('',#47630);
#14675=VERTEX_POINT('',#47632);
#14676=VERTEX_POINT('',#47634);
#14677=VERTEX_POINT('',#47636);
#14678=VERTEX_POINT('',#47638);
#14679=VERTEX_POINT('',#47641);
#14680=VERTEX_POINT('',#47642);
#14681=VERTEX_POINT('',#47644);
#14682=VERTEX_POINT('',#47646);
#14683=VERTEX_POINT('',#47648);
#14684=VERTEX_POINT('',#47650);
#14685=VERTEX_POINT('',#47652);
#14686=VERTEX_POINT('',#47654);
#14687=VERTEX_POINT('',#47657);
#14688=VERTEX_POINT('',#47658);
#14689=VERTEX_POINT('',#47660);
#14690=VERTEX_POINT('',#47662);
#14691=VERTEX_POINT('',#47664);
#14692=VERTEX_POINT('',#47666);
#14693=VERTEX_POINT('',#47668);
#14694=VERTEX_POINT('',#47670);
#14695=VERTEX_POINT('',#47673);
#14696=VERTEX_POINT('',#47674);
#14697=VERTEX_POINT('',#47676);
#14698=VERTEX_POINT('',#47678);
#14699=VERTEX_POINT('',#47680);
#14700=VERTEX_POINT('',#47682);
#14701=VERTEX_POINT('',#47684);
#14702=VERTEX_POINT('',#47686);
#14703=VERTEX_POINT('',#47689);
#14704=VERTEX_POINT('',#47690);
#14705=VERTEX_POINT('',#47692);
#14706=VERTEX_POINT('',#47694);
#14707=VERTEX_POINT('',#47696);
#14708=VERTEX_POINT('',#47698);
#14709=VERTEX_POINT('',#47700);
#14710=VERTEX_POINT('',#47702);
#14711=VERTEX_POINT('',#47705);
#14712=VERTEX_POINT('',#47706);
#14713=VERTEX_POINT('',#47708);
#14714=VERTEX_POINT('',#47710);
#14715=VERTEX_POINT('',#47712);
#14716=VERTEX_POINT('',#47714);
#14717=VERTEX_POINT('',#47716);
#14718=VERTEX_POINT('',#47718);
#14719=VERTEX_POINT('',#47721);
#14720=VERTEX_POINT('',#47722);
#14721=VERTEX_POINT('',#47724);
#14722=VERTEX_POINT('',#47726);
#14723=VERTEX_POINT('',#47728);
#14724=VERTEX_POINT('',#47730);
#14725=VERTEX_POINT('',#47732);
#14726=VERTEX_POINT('',#47734);
#14727=VERTEX_POINT('',#47737);
#14728=VERTEX_POINT('',#47738);
#14729=VERTEX_POINT('',#47740);
#14730=VERTEX_POINT('',#47742);
#14731=VERTEX_POINT('',#47744);
#14732=VERTEX_POINT('',#47746);
#14733=VERTEX_POINT('',#47748);
#14734=VERTEX_POINT('',#47750);
#14735=VERTEX_POINT('',#47753);
#14736=VERTEX_POINT('',#47754);
#14737=VERTEX_POINT('',#47756);
#14738=VERTEX_POINT('',#47758);
#14739=VERTEX_POINT('',#47760);
#14740=VERTEX_POINT('',#47762);
#14741=VERTEX_POINT('',#47764);
#14742=VERTEX_POINT('',#47766);
#14743=VERTEX_POINT('',#47769);
#14744=VERTEX_POINT('',#47770);
#14745=VERTEX_POINT('',#47772);
#14746=VERTEX_POINT('',#47774);
#14747=VERTEX_POINT('',#47776);
#14748=VERTEX_POINT('',#47778);
#14749=VERTEX_POINT('',#47780);
#14750=VERTEX_POINT('',#47782);
#14751=VERTEX_POINT('',#47785);
#14752=VERTEX_POINT('',#47786);
#14753=VERTEX_POINT('',#47788);
#14754=VERTEX_POINT('',#47790);
#14755=VERTEX_POINT('',#47792);
#14756=VERTEX_POINT('',#47794);
#14757=VERTEX_POINT('',#47796);
#14758=VERTEX_POINT('',#47798);
#14759=VERTEX_POINT('',#47801);
#14760=VERTEX_POINT('',#47802);
#14761=VERTEX_POINT('',#47804);
#14762=VERTEX_POINT('',#47806);
#14763=VERTEX_POINT('',#47808);
#14764=VERTEX_POINT('',#47810);
#14765=VERTEX_POINT('',#47812);
#14766=VERTEX_POINT('',#47814);
#14767=VERTEX_POINT('',#47817);
#14768=VERTEX_POINT('',#47818);
#14769=VERTEX_POINT('',#47820);
#14770=VERTEX_POINT('',#47822);
#14771=VERTEX_POINT('',#47824);
#14772=VERTEX_POINT('',#47826);
#14773=VERTEX_POINT('',#47828);
#14774=VERTEX_POINT('',#47830);
#14775=VERTEX_POINT('',#47833);
#14776=VERTEX_POINT('',#47834);
#14777=VERTEX_POINT('',#47836);
#14778=VERTEX_POINT('',#47838);
#14779=VERTEX_POINT('',#47840);
#14780=VERTEX_POINT('',#47842);
#14781=VERTEX_POINT('',#47844);
#14782=VERTEX_POINT('',#47846);
#14783=VERTEX_POINT('',#47849);
#14784=VERTEX_POINT('',#47850);
#14785=VERTEX_POINT('',#47852);
#14786=VERTEX_POINT('',#47854);
#14787=VERTEX_POINT('',#47856);
#14788=VERTEX_POINT('',#47858);
#14789=VERTEX_POINT('',#47860);
#14790=VERTEX_POINT('',#47862);
#14791=VERTEX_POINT('',#47865);
#14792=VERTEX_POINT('',#47866);
#14793=VERTEX_POINT('',#47868);
#14794=VERTEX_POINT('',#47870);
#14795=VERTEX_POINT('',#47872);
#14796=VERTEX_POINT('',#47874);
#14797=VERTEX_POINT('',#47876);
#14798=VERTEX_POINT('',#47878);
#14799=VERTEX_POINT('',#47881);
#14800=VERTEX_POINT('',#47882);
#14801=VERTEX_POINT('',#47884);
#14802=VERTEX_POINT('',#47886);
#14803=VERTEX_POINT('',#47888);
#14804=VERTEX_POINT('',#47890);
#14805=VERTEX_POINT('',#47892);
#14806=VERTEX_POINT('',#47894);
#14807=VERTEX_POINT('',#47897);
#14808=VERTEX_POINT('',#47898);
#14809=VERTEX_POINT('',#47900);
#14810=VERTEX_POINT('',#47902);
#14811=VERTEX_POINT('',#47904);
#14812=VERTEX_POINT('',#47906);
#14813=VERTEX_POINT('',#47908);
#14814=VERTEX_POINT('',#47910);
#14815=VERTEX_POINT('',#47913);
#14816=VERTEX_POINT('',#47914);
#14817=VERTEX_POINT('',#47916);
#14818=VERTEX_POINT('',#47918);
#14819=VERTEX_POINT('',#47920);
#14820=VERTEX_POINT('',#47922);
#14821=VERTEX_POINT('',#47924);
#14822=VERTEX_POINT('',#47926);
#14823=VERTEX_POINT('',#47929);
#14824=VERTEX_POINT('',#47930);
#14825=VERTEX_POINT('',#47932);
#14826=VERTEX_POINT('',#47934);
#14827=VERTEX_POINT('',#47936);
#14828=VERTEX_POINT('',#47938);
#14829=VERTEX_POINT('',#47940);
#14830=VERTEX_POINT('',#47942);
#14831=VERTEX_POINT('',#47945);
#14832=VERTEX_POINT('',#47946);
#14833=VERTEX_POINT('',#47948);
#14834=VERTEX_POINT('',#47950);
#14835=VERTEX_POINT('',#47952);
#14836=VERTEX_POINT('',#47954);
#14837=VERTEX_POINT('',#47956);
#14838=VERTEX_POINT('',#47958);
#14839=VERTEX_POINT('',#47961);
#14840=VERTEX_POINT('',#47962);
#14841=VERTEX_POINT('',#47964);
#14842=VERTEX_POINT('',#47966);
#14843=VERTEX_POINT('',#47968);
#14844=VERTEX_POINT('',#47970);
#14845=VERTEX_POINT('',#47972);
#14846=VERTEX_POINT('',#47974);
#14847=VERTEX_POINT('',#47977);
#14848=VERTEX_POINT('',#47978);
#14849=VERTEX_POINT('',#47980);
#14850=VERTEX_POINT('',#47982);
#14851=VERTEX_POINT('',#47984);
#14852=VERTEX_POINT('',#47986);
#14853=VERTEX_POINT('',#47988);
#14854=VERTEX_POINT('',#47990);
#14855=VERTEX_POINT('',#47993);
#14856=VERTEX_POINT('',#47994);
#14857=VERTEX_POINT('',#47996);
#14858=VERTEX_POINT('',#47998);
#14859=VERTEX_POINT('',#48000);
#14860=VERTEX_POINT('',#48002);
#14861=VERTEX_POINT('',#48004);
#14862=VERTEX_POINT('',#48006);
#14863=VERTEX_POINT('',#48009);
#14864=VERTEX_POINT('',#48010);
#14865=VERTEX_POINT('',#48012);
#14866=VERTEX_POINT('',#48014);
#14867=VERTEX_POINT('',#48016);
#14868=VERTEX_POINT('',#48018);
#14869=VERTEX_POINT('',#48020);
#14870=VERTEX_POINT('',#48022);
#14871=VERTEX_POINT('',#48025);
#14872=VERTEX_POINT('',#48026);
#14873=VERTEX_POINT('',#48028);
#14874=VERTEX_POINT('',#48030);
#14875=VERTEX_POINT('',#48032);
#14876=VERTEX_POINT('',#48034);
#14877=VERTEX_POINT('',#48036);
#14878=VERTEX_POINT('',#48038);
#14879=VERTEX_POINT('',#48041);
#14880=VERTEX_POINT('',#48042);
#14881=VERTEX_POINT('',#48044);
#14882=VERTEX_POINT('',#48046);
#14883=VERTEX_POINT('',#48048);
#14884=VERTEX_POINT('',#48050);
#14885=VERTEX_POINT('',#48052);
#14886=VERTEX_POINT('',#48054);
#14887=VERTEX_POINT('',#48057);
#14888=VERTEX_POINT('',#48058);
#14889=VERTEX_POINT('',#48060);
#14890=VERTEX_POINT('',#48062);
#14891=VERTEX_POINT('',#48064);
#14892=VERTEX_POINT('',#48066);
#14893=VERTEX_POINT('',#48068);
#14894=VERTEX_POINT('',#48070);
#14895=VERTEX_POINT('',#48073);
#14896=VERTEX_POINT('',#48074);
#14897=VERTEX_POINT('',#48076);
#14898=VERTEX_POINT('',#48078);
#14899=VERTEX_POINT('',#48080);
#14900=VERTEX_POINT('',#48082);
#14901=VERTEX_POINT('',#48084);
#14902=VERTEX_POINT('',#48086);
#14903=VERTEX_POINT('',#48089);
#14904=VERTEX_POINT('',#48090);
#14905=VERTEX_POINT('',#48092);
#14906=VERTEX_POINT('',#48094);
#14907=VERTEX_POINT('',#48096);
#14908=VERTEX_POINT('',#48098);
#14909=VERTEX_POINT('',#48100);
#14910=VERTEX_POINT('',#48102);
#14911=VERTEX_POINT('',#48105);
#14912=VERTEX_POINT('',#48106);
#14913=VERTEX_POINT('',#48108);
#14914=VERTEX_POINT('',#48110);
#14915=VERTEX_POINT('',#48112);
#14916=VERTEX_POINT('',#48114);
#14917=VERTEX_POINT('',#48116);
#14918=VERTEX_POINT('',#48118);
#14919=VERTEX_POINT('',#48121);
#14920=VERTEX_POINT('',#48122);
#14921=VERTEX_POINT('',#48124);
#14922=VERTEX_POINT('',#48126);
#14923=VERTEX_POINT('',#48128);
#14924=VERTEX_POINT('',#48130);
#14925=VERTEX_POINT('',#48132);
#14926=VERTEX_POINT('',#48134);
#14927=VERTEX_POINT('',#48137);
#14928=VERTEX_POINT('',#48138);
#14929=VERTEX_POINT('',#48140);
#14930=VERTEX_POINT('',#48142);
#14931=VERTEX_POINT('',#48144);
#14932=VERTEX_POINT('',#48146);
#14933=VERTEX_POINT('',#48148);
#14934=VERTEX_POINT('',#48150);
#14935=VERTEX_POINT('',#48153);
#14936=VERTEX_POINT('',#48154);
#14937=VERTEX_POINT('',#48156);
#14938=VERTEX_POINT('',#48158);
#14939=VERTEX_POINT('',#48160);
#14940=VERTEX_POINT('',#48162);
#14941=VERTEX_POINT('',#48164);
#14942=VERTEX_POINT('',#48166);
#14943=VERTEX_POINT('',#48169);
#14944=VERTEX_POINT('',#48170);
#14945=VERTEX_POINT('',#48172);
#14946=VERTEX_POINT('',#48174);
#14947=VERTEX_POINT('',#48176);
#14948=VERTEX_POINT('',#48178);
#14949=VERTEX_POINT('',#48180);
#14950=VERTEX_POINT('',#48182);
#14951=VERTEX_POINT('',#48185);
#14952=VERTEX_POINT('',#48186);
#14953=VERTEX_POINT('',#48188);
#14954=VERTEX_POINT('',#48190);
#14955=VERTEX_POINT('',#48192);
#14956=VERTEX_POINT('',#48194);
#14957=VERTEX_POINT('',#48196);
#14958=VERTEX_POINT('',#48198);
#14959=VERTEX_POINT('',#48201);
#14960=VERTEX_POINT('',#48202);
#14961=VERTEX_POINT('',#48204);
#14962=VERTEX_POINT('',#48206);
#14963=VERTEX_POINT('',#48208);
#14964=VERTEX_POINT('',#48210);
#14965=VERTEX_POINT('',#48212);
#14966=VERTEX_POINT('',#48214);
#14967=VERTEX_POINT('',#48217);
#14968=VERTEX_POINT('',#48218);
#14969=VERTEX_POINT('',#48220);
#14970=VERTEX_POINT('',#48222);
#14971=VERTEX_POINT('',#48224);
#14972=VERTEX_POINT('',#48226);
#14973=VERTEX_POINT('',#48228);
#14974=VERTEX_POINT('',#48230);
#14975=VERTEX_POINT('',#48233);
#14976=VERTEX_POINT('',#48234);
#14977=VERTEX_POINT('',#48236);
#14978=VERTEX_POINT('',#48238);
#14979=VERTEX_POINT('',#48240);
#14980=VERTEX_POINT('',#48242);
#14981=VERTEX_POINT('',#48244);
#14982=VERTEX_POINT('',#48246);
#14983=VERTEX_POINT('',#48249);
#14984=VERTEX_POINT('',#48250);
#14985=VERTEX_POINT('',#48252);
#14986=VERTEX_POINT('',#48254);
#14987=VERTEX_POINT('',#48256);
#14988=VERTEX_POINT('',#48258);
#14989=VERTEX_POINT('',#48260);
#14990=VERTEX_POINT('',#48262);
#14991=VERTEX_POINT('',#48265);
#14992=VERTEX_POINT('',#48266);
#14993=VERTEX_POINT('',#48268);
#14994=VERTEX_POINT('',#48270);
#14995=VERTEX_POINT('',#48272);
#14996=VERTEX_POINT('',#48274);
#14997=VERTEX_POINT('',#48276);
#14998=VERTEX_POINT('',#48278);
#14999=VERTEX_POINT('',#48281);
#15000=VERTEX_POINT('',#48282);
#15001=VERTEX_POINT('',#48284);
#15002=VERTEX_POINT('',#48286);
#15003=VERTEX_POINT('',#48288);
#15004=VERTEX_POINT('',#48290);
#15005=VERTEX_POINT('',#48292);
#15006=VERTEX_POINT('',#48294);
#15007=VERTEX_POINT('',#48297);
#15008=VERTEX_POINT('',#48298);
#15009=VERTEX_POINT('',#48300);
#15010=VERTEX_POINT('',#48302);
#15011=VERTEX_POINT('',#48304);
#15012=VERTEX_POINT('',#48306);
#15013=VERTEX_POINT('',#48308);
#15014=VERTEX_POINT('',#48310);
#15015=VERTEX_POINT('',#48313);
#15016=VERTEX_POINT('',#48314);
#15017=VERTEX_POINT('',#48316);
#15018=VERTEX_POINT('',#48318);
#15019=VERTEX_POINT('',#48320);
#15020=VERTEX_POINT('',#48322);
#15021=VERTEX_POINT('',#48324);
#15022=VERTEX_POINT('',#48326);
#15023=VERTEX_POINT('',#48329);
#15024=VERTEX_POINT('',#48330);
#15025=VERTEX_POINT('',#48332);
#15026=VERTEX_POINT('',#48334);
#15027=VERTEX_POINT('',#48336);
#15028=VERTEX_POINT('',#48338);
#15029=VERTEX_POINT('',#48340);
#15030=VERTEX_POINT('',#48342);
#15031=VERTEX_POINT('',#48345);
#15032=VERTEX_POINT('',#48346);
#15033=VERTEX_POINT('',#48348);
#15034=VERTEX_POINT('',#48350);
#15035=VERTEX_POINT('',#48352);
#15036=VERTEX_POINT('',#48354);
#15037=VERTEX_POINT('',#48356);
#15038=VERTEX_POINT('',#48358);
#15039=VERTEX_POINT('',#48361);
#15040=VERTEX_POINT('',#48362);
#15041=VERTEX_POINT('',#48364);
#15042=VERTEX_POINT('',#48366);
#15043=VERTEX_POINT('',#48368);
#15044=VERTEX_POINT('',#48370);
#15045=VERTEX_POINT('',#48372);
#15046=VERTEX_POINT('',#48374);
#15047=VERTEX_POINT('',#48377);
#15048=VERTEX_POINT('',#48378);
#15049=VERTEX_POINT('',#48380);
#15050=VERTEX_POINT('',#48382);
#15051=VERTEX_POINT('',#48384);
#15052=VERTEX_POINT('',#48386);
#15053=VERTEX_POINT('',#48388);
#15054=VERTEX_POINT('',#48390);
#15055=VERTEX_POINT('',#48393);
#15056=VERTEX_POINT('',#48394);
#15057=VERTEX_POINT('',#48396);
#15058=VERTEX_POINT('',#48398);
#15059=VERTEX_POINT('',#48400);
#15060=VERTEX_POINT('',#48402);
#15061=VERTEX_POINT('',#48404);
#15062=VERTEX_POINT('',#48406);
#15063=VERTEX_POINT('',#48409);
#15064=VERTEX_POINT('',#48410);
#15065=VERTEX_POINT('',#48412);
#15066=VERTEX_POINT('',#48414);
#15067=VERTEX_POINT('',#48416);
#15068=VERTEX_POINT('',#48418);
#15069=VERTEX_POINT('',#48420);
#15070=VERTEX_POINT('',#48422);
#15071=VERTEX_POINT('',#48425);
#15072=VERTEX_POINT('',#48426);
#15073=VERTEX_POINT('',#48428);
#15074=VERTEX_POINT('',#48430);
#15075=VERTEX_POINT('',#48432);
#15076=VERTEX_POINT('',#48434);
#15077=VERTEX_POINT('',#48436);
#15078=VERTEX_POINT('',#48438);
#15079=VERTEX_POINT('',#48441);
#15080=VERTEX_POINT('',#48442);
#15081=VERTEX_POINT('',#48444);
#15082=VERTEX_POINT('',#48446);
#15083=VERTEX_POINT('',#48448);
#15084=VERTEX_POINT('',#48450);
#15085=VERTEX_POINT('',#48452);
#15086=VERTEX_POINT('',#48454);
#15087=VERTEX_POINT('',#48457);
#15088=VERTEX_POINT('',#48458);
#15089=VERTEX_POINT('',#48460);
#15090=VERTEX_POINT('',#48462);
#15091=VERTEX_POINT('',#48464);
#15092=VERTEX_POINT('',#48466);
#15093=VERTEX_POINT('',#48468);
#15094=VERTEX_POINT('',#48470);
#15095=VERTEX_POINT('',#48473);
#15096=VERTEX_POINT('',#48474);
#15097=VERTEX_POINT('',#48476);
#15098=VERTEX_POINT('',#48478);
#15099=VERTEX_POINT('',#48480);
#15100=VERTEX_POINT('',#48482);
#15101=VERTEX_POINT('',#48484);
#15102=VERTEX_POINT('',#48486);
#15103=VERTEX_POINT('',#48489);
#15104=VERTEX_POINT('',#48490);
#15105=VERTEX_POINT('',#48492);
#15106=VERTEX_POINT('',#48494);
#15107=VERTEX_POINT('',#48496);
#15108=VERTEX_POINT('',#48498);
#15109=VERTEX_POINT('',#48500);
#15110=VERTEX_POINT('',#48502);
#15111=VERTEX_POINT('',#48505);
#15112=VERTEX_POINT('',#48506);
#15113=VERTEX_POINT('',#48508);
#15114=VERTEX_POINT('',#48510);
#15115=VERTEX_POINT('',#48512);
#15116=VERTEX_POINT('',#48514);
#15117=VERTEX_POINT('',#48516);
#15118=VERTEX_POINT('',#48518);
#15119=VERTEX_POINT('',#48521);
#15120=VERTEX_POINT('',#48522);
#15121=VERTEX_POINT('',#48524);
#15122=VERTEX_POINT('',#48526);
#15123=VERTEX_POINT('',#48528);
#15124=VERTEX_POINT('',#48530);
#15125=VERTEX_POINT('',#48532);
#15126=VERTEX_POINT('',#48534);
#15127=VERTEX_POINT('',#48537);
#15128=VERTEX_POINT('',#48538);
#15129=VERTEX_POINT('',#48540);
#15130=VERTEX_POINT('',#48542);
#15131=VERTEX_POINT('',#48544);
#15132=VERTEX_POINT('',#48546);
#15133=VERTEX_POINT('',#48548);
#15134=VERTEX_POINT('',#48550);
#15135=VERTEX_POINT('',#48553);
#15136=VERTEX_POINT('',#48554);
#15137=VERTEX_POINT('',#48556);
#15138=VERTEX_POINT('',#48558);
#15139=VERTEX_POINT('',#48560);
#15140=VERTEX_POINT('',#48562);
#15141=VERTEX_POINT('',#48564);
#15142=VERTEX_POINT('',#48566);
#15143=VERTEX_POINT('',#48569);
#15144=VERTEX_POINT('',#48570);
#15145=VERTEX_POINT('',#48572);
#15146=VERTEX_POINT('',#48574);
#15147=VERTEX_POINT('',#48576);
#15148=VERTEX_POINT('',#48578);
#15149=VERTEX_POINT('',#48580);
#15150=VERTEX_POINT('',#48582);
#15151=VERTEX_POINT('',#48586);
#15152=VERTEX_POINT('',#48587);
#15153=VERTEX_POINT('',#48589);
#15154=VERTEX_POINT('',#48594);
#15155=VERTEX_POINT('',#48601);
#15156=VERTEX_POINT('',#48603);
#15157=VERTEX_POINT('',#48610);
#15158=VERTEX_POINT('',#48612);
#15159=VERTEX_POINT('',#48619);
#15160=VERTEX_POINT('',#48621);
#15161=VERTEX_POINT('',#48628);
#15162=VERTEX_POINT('',#48630);
#15163=VERTEX_POINT('',#48637);
#15164=VERTEX_POINT('',#48639);
#15165=VERTEX_POINT('',#48646);
#15166=VERTEX_POINT('',#48648);
#15167=VERTEX_POINT('',#48655);
#15168=VERTEX_POINT('',#48657);
#15169=VERTEX_POINT('',#48664);
#15170=VERTEX_POINT('',#48666);
#15171=VERTEX_POINT('',#48676);
#15172=VERTEX_POINT('',#48678);
#15173=VERTEX_POINT('',#48682);
#15174=VERTEX_POINT('',#48686);
#15175=VERTEX_POINT('',#48690);
#15176=VERTEX_POINT('',#48694);
#15177=VERTEX_POINT('',#48698);
#15178=VERTEX_POINT('',#48702);
#15179=VERTEX_POINT('',#48704);
#15180=VERTEX_POINT('',#48706);
#15181=VERTEX_POINT('',#48708);
#15182=VERTEX_POINT('',#48710);
#15183=VERTEX_POINT('',#48713);
#15184=VERTEX_POINT('',#48714);
#15185=VERTEX_POINT('',#48717);
#15186=VERTEX_POINT('',#48721);
#15187=VERTEX_POINT('',#48725);
#15188=VERTEX_POINT('',#48727);
#15189=VERTEX_POINT('',#48731);
#15190=VERTEX_POINT('',#48733);
#15191=VERTEX_POINT('',#48737);
#15192=VERTEX_POINT('',#48741);
#15193=VERTEX_POINT('',#48748);
#15194=VERTEX_POINT('',#48749);
#15195=VERTEX_POINT('',#48751);
#15196=VERTEX_POINT('',#48768);
#15197=VERTEX_POINT('',#48769);
#15198=VERTEX_POINT('',#48771);
#15199=VERTEX_POINT('',#48775);
#15200=VERTEX_POINT('',#48776);
#15201=VERTEX_POINT('',#48778);
#15202=VERTEX_POINT('',#48782);
#15203=VERTEX_POINT('',#48783);
#15204=VERTEX_POINT('',#48785);
#15205=VERTEX_POINT('',#48792);
#15206=VERTEX_POINT('',#48793);
#15207=VERTEX_POINT('',#48795);
#15208=VERTEX_POINT('',#48823);
#15209=VERTEX_POINT('',#48824);
#15210=VERTEX_POINT('',#48826);
#15211=VERTEX_POINT('',#48830);
#15212=VERTEX_POINT('',#48831);
#15213=VERTEX_POINT('',#48834);
#15214=VERTEX_POINT('',#48841);
#15215=VERTEX_POINT('',#48842);
#15216=VERTEX_POINT('',#48844);
#15217=VERTEX_POINT('',#48848);
#15218=VERTEX_POINT('',#48849);
#15219=VERTEX_POINT('',#48852);
#15220=VERTEX_POINT('',#48862);
#15221=VERTEX_POINT('',#48869);
#15222=VERTEX_POINT('',#48878);
#15223=VERTEX_POINT('',#48879);
#15224=VERTEX_POINT('',#48881);
#15225=VERTEX_POINT('',#48885);
#15226=VERTEX_POINT('',#48886);
#15227=VERTEX_POINT('',#48888);
#15228=VERTEX_POINT('',#48892);
#15229=VERTEX_POINT('',#48893);
#15230=VERTEX_POINT('',#48895);
#15231=VERTEX_POINT('',#48902);
#15232=VERTEX_POINT('',#48903);
#15233=VERTEX_POINT('',#48905);
#15234=VERTEX_POINT('',#48933);
#15235=VERTEX_POINT('',#48934);
#15236=VERTEX_POINT('',#48936);
#15237=VERTEX_POINT('',#48940);
#15238=VERTEX_POINT('',#48941);
#15239=VERTEX_POINT('',#48943);
#15240=VERTEX_POINT('',#48947);
#15241=VERTEX_POINT('',#48948);
#15242=VERTEX_POINT('',#48950);
#15243=VERTEX_POINT('',#48957);
#15244=VERTEX_POINT('',#48958);
#15245=VERTEX_POINT('',#48960);
#15246=VERTEX_POINT('',#48988);
#15247=VERTEX_POINT('',#48989);
#15248=VERTEX_POINT('',#48992);
#15249=VERTEX_POINT('',#48996);
#15250=VERTEX_POINT('',#49000);
#15251=VERTEX_POINT('',#49002);
#15252=VERTEX_POINT('',#49006);
#15253=VERTEX_POINT('',#49008);
#15254=VERTEX_POINT('',#49012);
#15255=VERTEX_POINT('',#49016);
#15256=VERTEX_POINT('',#49023);
#15257=VERTEX_POINT('',#49024);
#15258=VERTEX_POINT('',#49026);
#15259=VERTEX_POINT('',#49043);
#15260=VERTEX_POINT('',#49044);
#15261=VERTEX_POINT('',#49046);
#15262=VERTEX_POINT('',#49050);
#15263=VERTEX_POINT('',#49051);
#15264=VERTEX_POINT('',#49053);
#15265=VERTEX_POINT('',#49057);
#15266=VERTEX_POINT('',#49058);
#15267=VERTEX_POINT('',#49060);
#15268=VERTEX_POINT('',#49067);
#15269=VERTEX_POINT('',#49068);
#15270=VERTEX_POINT('',#49070);
#15271=VERTEX_POINT('',#49098);
#15272=VERTEX_POINT('',#49099);
#15273=VERTEX_POINT('',#49101);
#15274=VERTEX_POINT('',#49105);
#15275=VERTEX_POINT('',#49106);
#15276=VERTEX_POINT('',#49109);
#15277=VERTEX_POINT('',#49116);
#15278=VERTEX_POINT('',#49117);
#15279=VERTEX_POINT('',#49119);
#15280=VERTEX_POINT('',#49123);
#15281=VERTEX_POINT('',#49124);
#15282=VERTEX_POINT('',#49127);
#15283=VERTEX_POINT('',#49137);
#15284=VERTEX_POINT('',#49144);
#15285=VERTEX_POINT('',#49153);
#15286=VERTEX_POINT('',#49154);
#15287=VERTEX_POINT('',#49156);
#15288=VERTEX_POINT('',#49160);
#15289=VERTEX_POINT('',#49161);
#15290=VERTEX_POINT('',#49163);
#15291=VERTEX_POINT('',#49167);
#15292=VERTEX_POINT('',#49168);
#15293=VERTEX_POINT('',#49170);
#15294=VERTEX_POINT('',#49177);
#15295=VERTEX_POINT('',#49178);
#15296=VERTEX_POINT('',#49180);
#15297=VERTEX_POINT('',#49208);
#15298=VERTEX_POINT('',#49209);
#15299=VERTEX_POINT('',#49211);
#15300=VERTEX_POINT('',#49215);
#15301=VERTEX_POINT('',#49216);
#15302=VERTEX_POINT('',#49218);
#15303=VERTEX_POINT('',#49222);
#15304=VERTEX_POINT('',#49223);
#15305=VERTEX_POINT('',#49225);
#15306=VERTEX_POINT('',#49232);
#15307=VERTEX_POINT('',#49233);
#15308=VERTEX_POINT('',#49235);
#15309=VERTEX_POINT('',#49263);
#15310=VERTEX_POINT('',#49264);
#15311=VERTEX_POINT('',#49267);
#15312=VERTEX_POINT('',#49271);
#15313=VERTEX_POINT('',#49275);
#15314=VERTEX_POINT('',#49277);
#15315=VERTEX_POINT('',#49281);
#15316=VERTEX_POINT('',#49283);
#15317=VERTEX_POINT('',#49287);
#15318=VERTEX_POINT('',#49291);
#15319=VERTEX_POINT('',#49298);
#15320=VERTEX_POINT('',#49299);
#15321=VERTEX_POINT('',#49301);
#15322=VERTEX_POINT('',#49318);
#15323=VERTEX_POINT('',#49319);
#15324=VERTEX_POINT('',#49321);
#15325=VERTEX_POINT('',#49325);
#15326=VERTEX_POINT('',#49326);
#15327=VERTEX_POINT('',#49328);
#15328=VERTEX_POINT('',#49332);
#15329=VERTEX_POINT('',#49333);
#15330=VERTEX_POINT('',#49335);
#15331=VERTEX_POINT('',#49342);
#15332=VERTEX_POINT('',#49343);
#15333=VERTEX_POINT('',#49345);
#15334=VERTEX_POINT('',#49373);
#15335=VERTEX_POINT('',#49374);
#15336=VERTEX_POINT('',#49376);
#15337=VERTEX_POINT('',#49380);
#15338=VERTEX_POINT('',#49381);
#15339=VERTEX_POINT('',#49384);
#15340=VERTEX_POINT('',#49391);
#15341=VERTEX_POINT('',#49392);
#15342=VERTEX_POINT('',#49394);
#15343=VERTEX_POINT('',#49398);
#15344=VERTEX_POINT('',#49399);
#15345=VERTEX_POINT('',#49402);
#15346=VERTEX_POINT('',#49412);
#15347=VERTEX_POINT('',#49419);
#15348=VERTEX_POINT('',#49428);
#15349=VERTEX_POINT('',#49429);
#15350=VERTEX_POINT('',#49431);
#15351=VERTEX_POINT('',#49435);
#15352=VERTEX_POINT('',#49436);
#15353=VERTEX_POINT('',#49438);
#15354=VERTEX_POINT('',#49442);
#15355=VERTEX_POINT('',#49443);
#15356=VERTEX_POINT('',#49445);
#15357=VERTEX_POINT('',#49452);
#15358=VERTEX_POINT('',#49453);
#15359=VERTEX_POINT('',#49455);
#15360=VERTEX_POINT('',#49483);
#15361=VERTEX_POINT('',#49484);
#15362=VERTEX_POINT('',#49486);
#15363=VERTEX_POINT('',#49490);
#15364=VERTEX_POINT('',#49491);
#15365=VERTEX_POINT('',#49493);
#15366=VERTEX_POINT('',#49497);
#15367=VERTEX_POINT('',#49498);
#15368=VERTEX_POINT('',#49500);
#15369=VERTEX_POINT('',#49507);
#15370=VERTEX_POINT('',#49508);
#15371=VERTEX_POINT('',#49510);
#15372=VERTEX_POINT('',#49538);
#15373=VERTEX_POINT('',#49539);
#15374=VERTEX_POINT('',#49542);
#15375=VERTEX_POINT('',#49546);
#15376=VERTEX_POINT('',#49550);
#15377=VERTEX_POINT('',#49552);
#15378=VERTEX_POINT('',#49556);
#15379=VERTEX_POINT('',#49558);
#15380=VERTEX_POINT('',#49562);
#15381=VERTEX_POINT('',#49566);
#15382=VERTEX_POINT('',#49573);
#15383=VERTEX_POINT('',#49574);
#15384=VERTEX_POINT('',#49576);
#15385=VERTEX_POINT('',#49593);
#15386=VERTEX_POINT('',#49594);
#15387=VERTEX_POINT('',#49596);
#15388=VERTEX_POINT('',#49600);
#15389=VERTEX_POINT('',#49601);
#15390=VERTEX_POINT('',#49603);
#15391=VERTEX_POINT('',#49607);
#15392=VERTEX_POINT('',#49608);
#15393=VERTEX_POINT('',#49610);
#15394=VERTEX_POINT('',#49617);
#15395=VERTEX_POINT('',#49618);
#15396=VERTEX_POINT('',#49620);
#15397=VERTEX_POINT('',#49648);
#15398=VERTEX_POINT('',#49649);
#15399=VERTEX_POINT('',#49651);
#15400=VERTEX_POINT('',#49655);
#15401=VERTEX_POINT('',#49656);
#15402=VERTEX_POINT('',#49659);
#15403=VERTEX_POINT('',#49666);
#15404=VERTEX_POINT('',#49667);
#15405=VERTEX_POINT('',#49669);
#15406=VERTEX_POINT('',#49673);
#15407=VERTEX_POINT('',#49674);
#15408=VERTEX_POINT('',#49677);
#15409=VERTEX_POINT('',#49687);
#15410=VERTEX_POINT('',#49694);
#15411=VERTEX_POINT('',#49703);
#15412=VERTEX_POINT('',#49704);
#15413=VERTEX_POINT('',#49706);
#15414=VERTEX_POINT('',#49710);
#15415=VERTEX_POINT('',#49711);
#15416=VERTEX_POINT('',#49713);
#15417=VERTEX_POINT('',#49717);
#15418=VERTEX_POINT('',#49718);
#15419=VERTEX_POINT('',#49720);
#15420=VERTEX_POINT('',#49727);
#15421=VERTEX_POINT('',#49728);
#15422=VERTEX_POINT('',#49730);
#15423=VERTEX_POINT('',#49758);
#15424=VERTEX_POINT('',#49759);
#15425=VERTEX_POINT('',#49761);
#15426=VERTEX_POINT('',#49765);
#15427=VERTEX_POINT('',#49766);
#15428=VERTEX_POINT('',#49768);
#15429=VERTEX_POINT('',#49772);
#15430=VERTEX_POINT('',#49773);
#15431=VERTEX_POINT('',#49775);
#15432=VERTEX_POINT('',#49782);
#15433=VERTEX_POINT('',#49783);
#15434=VERTEX_POINT('',#49785);
#15435=VERTEX_POINT('',#49813);
#15436=VERTEX_POINT('',#49814);
#15437=VERTEX_POINT('',#49817);
#15438=VERTEX_POINT('',#49821);
#15439=VERTEX_POINT('',#49825);
#15440=VERTEX_POINT('',#49827);
#15441=VERTEX_POINT('',#49831);
#15442=VERTEX_POINT('',#49833);
#15443=VERTEX_POINT('',#49837);
#15444=VERTEX_POINT('',#49841);
#15445=VERTEX_POINT('',#49848);
#15446=VERTEX_POINT('',#49849);
#15447=VERTEX_POINT('',#49851);
#15448=VERTEX_POINT('',#49868);
#15449=VERTEX_POINT('',#49869);
#15450=VERTEX_POINT('',#49871);
#15451=VERTEX_POINT('',#49875);
#15452=VERTEX_POINT('',#49876);
#15453=VERTEX_POINT('',#49878);
#15454=VERTEX_POINT('',#49882);
#15455=VERTEX_POINT('',#49883);
#15456=VERTEX_POINT('',#49885);
#15457=VERTEX_POINT('',#49892);
#15458=VERTEX_POINT('',#49893);
#15459=VERTEX_POINT('',#49895);
#15460=VERTEX_POINT('',#49923);
#15461=VERTEX_POINT('',#49924);
#15462=VERTEX_POINT('',#49926);
#15463=VERTEX_POINT('',#49930);
#15464=VERTEX_POINT('',#49931);
#15465=VERTEX_POINT('',#49934);
#15466=VERTEX_POINT('',#49941);
#15467=VERTEX_POINT('',#49942);
#15468=VERTEX_POINT('',#49944);
#15469=VERTEX_POINT('',#49948);
#15470=VERTEX_POINT('',#49949);
#15471=VERTEX_POINT('',#49952);
#15472=VERTEX_POINT('',#49962);
#15473=VERTEX_POINT('',#49969);
#15474=VERTEX_POINT('',#49978);
#15475=VERTEX_POINT('',#49979);
#15476=VERTEX_POINT('',#49981);
#15477=VERTEX_POINT('',#49985);
#15478=VERTEX_POINT('',#49986);
#15479=VERTEX_POINT('',#49988);
#15480=VERTEX_POINT('',#49992);
#15481=VERTEX_POINT('',#49993);
#15482=VERTEX_POINT('',#49995);
#15483=VERTEX_POINT('',#50002);
#15484=VERTEX_POINT('',#50003);
#15485=VERTEX_POINT('',#50005);
#15486=VERTEX_POINT('',#50033);
#15487=VERTEX_POINT('',#50034);
#15488=VERTEX_POINT('',#50036);
#15489=VERTEX_POINT('',#50040);
#15490=VERTEX_POINT('',#50041);
#15491=VERTEX_POINT('',#50043);
#15492=VERTEX_POINT('',#50047);
#15493=VERTEX_POINT('',#50048);
#15494=VERTEX_POINT('',#50050);
#15495=VERTEX_POINT('',#50057);
#15496=VERTEX_POINT('',#50058);
#15497=VERTEX_POINT('',#50060);
#15498=VERTEX_POINT('',#50088);
#15499=VERTEX_POINT('',#50089);
#15500=VERTEX_POINT('',#50092);
#15501=VERTEX_POINT('',#50096);
#15502=VERTEX_POINT('',#50100);
#15503=VERTEX_POINT('',#50102);
#15504=VERTEX_POINT('',#50106);
#15505=VERTEX_POINT('',#50108);
#15506=VERTEX_POINT('',#50112);
#15507=VERTEX_POINT('',#50116);
#15508=VERTEX_POINT('',#50123);
#15509=VERTEX_POINT('',#50124);
#15510=VERTEX_POINT('',#50126);
#15511=VERTEX_POINT('',#50143);
#15512=VERTEX_POINT('',#50144);
#15513=VERTEX_POINT('',#50146);
#15514=VERTEX_POINT('',#50150);
#15515=VERTEX_POINT('',#50151);
#15516=VERTEX_POINT('',#50153);
#15517=VERTEX_POINT('',#50157);
#15518=VERTEX_POINT('',#50158);
#15519=VERTEX_POINT('',#50160);
#15520=VERTEX_POINT('',#50167);
#15521=VERTEX_POINT('',#50168);
#15522=VERTEX_POINT('',#50170);
#15523=VERTEX_POINT('',#50198);
#15524=VERTEX_POINT('',#50199);
#15525=VERTEX_POINT('',#50201);
#15526=VERTEX_POINT('',#50205);
#15527=VERTEX_POINT('',#50206);
#15528=VERTEX_POINT('',#50209);
#15529=VERTEX_POINT('',#50216);
#15530=VERTEX_POINT('',#50217);
#15531=VERTEX_POINT('',#50219);
#15532=VERTEX_POINT('',#50223);
#15533=VERTEX_POINT('',#50224);
#15534=VERTEX_POINT('',#50227);
#15535=VERTEX_POINT('',#50237);
#15536=VERTEX_POINT('',#50244);
#15537=VERTEX_POINT('',#50253);
#15538=VERTEX_POINT('',#50254);
#15539=VERTEX_POINT('',#50256);
#15540=VERTEX_POINT('',#50260);
#15541=VERTEX_POINT('',#50261);
#15542=VERTEX_POINT('',#50263);
#15543=VERTEX_POINT('',#50267);
#15544=VERTEX_POINT('',#50268);
#15545=VERTEX_POINT('',#50270);
#15546=VERTEX_POINT('',#50277);
#15547=VERTEX_POINT('',#50278);
#15548=VERTEX_POINT('',#50280);
#15549=VERTEX_POINT('',#50308);
#15550=VERTEX_POINT('',#50309);
#15551=VERTEX_POINT('',#50311);
#15552=VERTEX_POINT('',#50315);
#15553=VERTEX_POINT('',#50316);
#15554=VERTEX_POINT('',#50318);
#15555=VERTEX_POINT('',#50322);
#15556=VERTEX_POINT('',#50323);
#15557=VERTEX_POINT('',#50325);
#15558=VERTEX_POINT('',#50332);
#15559=VERTEX_POINT('',#50333);
#15560=VERTEX_POINT('',#50335);
#15561=VERTEX_POINT('',#50363);
#15562=VERTEX_POINT('',#50364);
#15563=VERTEX_POINT('',#50367);
#15564=VERTEX_POINT('',#50371);
#15565=VERTEX_POINT('',#50375);
#15566=VERTEX_POINT('',#50377);
#15567=VERTEX_POINT('',#50381);
#15568=VERTEX_POINT('',#50383);
#15569=VERTEX_POINT('',#50387);
#15570=VERTEX_POINT('',#50391);
#15571=VERTEX_POINT('',#50398);
#15572=VERTEX_POINT('',#50399);
#15573=VERTEX_POINT('',#50401);
#15574=VERTEX_POINT('',#50418);
#15575=VERTEX_POINT('',#50419);
#15576=VERTEX_POINT('',#50421);
#15577=VERTEX_POINT('',#50425);
#15578=VERTEX_POINT('',#50426);
#15579=VERTEX_POINT('',#50428);
#15580=VERTEX_POINT('',#50432);
#15581=VERTEX_POINT('',#50433);
#15582=VERTEX_POINT('',#50435);
#15583=VERTEX_POINT('',#50442);
#15584=VERTEX_POINT('',#50443);
#15585=VERTEX_POINT('',#50445);
#15586=VERTEX_POINT('',#50473);
#15587=VERTEX_POINT('',#50474);
#15588=VERTEX_POINT('',#50476);
#15589=VERTEX_POINT('',#50480);
#15590=VERTEX_POINT('',#50481);
#15591=VERTEX_POINT('',#50484);
#15592=VERTEX_POINT('',#50491);
#15593=VERTEX_POINT('',#50492);
#15594=VERTEX_POINT('',#50494);
#15595=VERTEX_POINT('',#50498);
#15596=VERTEX_POINT('',#50499);
#15597=VERTEX_POINT('',#50502);
#15598=VERTEX_POINT('',#50512);
#15599=VERTEX_POINT('',#50519);
#15600=VERTEX_POINT('',#50528);
#15601=VERTEX_POINT('',#50529);
#15602=VERTEX_POINT('',#50531);
#15603=VERTEX_POINT('',#50535);
#15604=VERTEX_POINT('',#50536);
#15605=VERTEX_POINT('',#50538);
#15606=VERTEX_POINT('',#50542);
#15607=VERTEX_POINT('',#50543);
#15608=VERTEX_POINT('',#50545);
#15609=VERTEX_POINT('',#50552);
#15610=VERTEX_POINT('',#50553);
#15611=VERTEX_POINT('',#50555);
#15612=VERTEX_POINT('',#50583);
#15613=VERTEX_POINT('',#50584);
#15614=VERTEX_POINT('',#50586);
#15615=VERTEX_POINT('',#50590);
#15616=VERTEX_POINT('',#50591);
#15617=VERTEX_POINT('',#50593);
#15618=VERTEX_POINT('',#50597);
#15619=VERTEX_POINT('',#50598);
#15620=VERTEX_POINT('',#50600);
#15621=VERTEX_POINT('',#50607);
#15622=VERTEX_POINT('',#50608);
#15623=VERTEX_POINT('',#50610);
#15624=VERTEX_POINT('',#50638);
#15625=VERTEX_POINT('',#50639);
#15626=VERTEX_POINT('',#50642);
#15627=VERTEX_POINT('',#50646);
#15628=VERTEX_POINT('',#50650);
#15629=VERTEX_POINT('',#50652);
#15630=VERTEX_POINT('',#50656);
#15631=VERTEX_POINT('',#50658);
#15632=VERTEX_POINT('',#50662);
#15633=VERTEX_POINT('',#50666);
#15634=VERTEX_POINT('',#50673);
#15635=VERTEX_POINT('',#50674);
#15636=VERTEX_POINT('',#50676);
#15637=VERTEX_POINT('',#50693);
#15638=VERTEX_POINT('',#50694);
#15639=VERTEX_POINT('',#50696);
#15640=VERTEX_POINT('',#50700);
#15641=VERTEX_POINT('',#50701);
#15642=VERTEX_POINT('',#50703);
#15643=VERTEX_POINT('',#50707);
#15644=VERTEX_POINT('',#50708);
#15645=VERTEX_POINT('',#50710);
#15646=VERTEX_POINT('',#50717);
#15647=VERTEX_POINT('',#50718);
#15648=VERTEX_POINT('',#50720);
#15649=VERTEX_POINT('',#50748);
#15650=VERTEX_POINT('',#50749);
#15651=VERTEX_POINT('',#50751);
#15652=VERTEX_POINT('',#50755);
#15653=VERTEX_POINT('',#50756);
#15654=VERTEX_POINT('',#50759);
#15655=VERTEX_POINT('',#50766);
#15656=VERTEX_POINT('',#50767);
#15657=VERTEX_POINT('',#50769);
#15658=VERTEX_POINT('',#50773);
#15659=VERTEX_POINT('',#50774);
#15660=VERTEX_POINT('',#50777);
#15661=VERTEX_POINT('',#50787);
#15662=VERTEX_POINT('',#50794);
#15663=VERTEX_POINT('',#50803);
#15664=VERTEX_POINT('',#50804);
#15665=VERTEX_POINT('',#50806);
#15666=VERTEX_POINT('',#50810);
#15667=VERTEX_POINT('',#50811);
#15668=VERTEX_POINT('',#50813);
#15669=VERTEX_POINT('',#50817);
#15670=VERTEX_POINT('',#50818);
#15671=VERTEX_POINT('',#50820);
#15672=VERTEX_POINT('',#50827);
#15673=VERTEX_POINT('',#50828);
#15674=VERTEX_POINT('',#50830);
#15675=VERTEX_POINT('',#50858);
#15676=VERTEX_POINT('',#50859);
#15677=VERTEX_POINT('',#50861);
#15678=VERTEX_POINT('',#50865);
#15679=VERTEX_POINT('',#50866);
#15680=VERTEX_POINT('',#50868);
#15681=VERTEX_POINT('',#50872);
#15682=VERTEX_POINT('',#50873);
#15683=VERTEX_POINT('',#50875);
#15684=VERTEX_POINT('',#50882);
#15685=VERTEX_POINT('',#50883);
#15686=VERTEX_POINT('',#50885);
#15687=VERTEX_POINT('',#50913);
#15688=VERTEX_POINT('',#50914);
#15689=VERTEX_POINT('',#50917);
#15690=VERTEX_POINT('',#50921);
#15691=VERTEX_POINT('',#50925);
#15692=VERTEX_POINT('',#50927);
#15693=VERTEX_POINT('',#50931);
#15694=VERTEX_POINT('',#50933);
#15695=VERTEX_POINT('',#50937);
#15696=VERTEX_POINT('',#50941);
#15697=VERTEX_POINT('',#50948);
#15698=VERTEX_POINT('',#50949);
#15699=VERTEX_POINT('',#50951);
#15700=VERTEX_POINT('',#50968);
#15701=VERTEX_POINT('',#50969);
#15702=VERTEX_POINT('',#50971);
#15703=VERTEX_POINT('',#50975);
#15704=VERTEX_POINT('',#50976);
#15705=VERTEX_POINT('',#50978);
#15706=VERTEX_POINT('',#50982);
#15707=VERTEX_POINT('',#50983);
#15708=VERTEX_POINT('',#50985);
#15709=VERTEX_POINT('',#50992);
#15710=VERTEX_POINT('',#50993);
#15711=VERTEX_POINT('',#50995);
#15712=VERTEX_POINT('',#51023);
#15713=VERTEX_POINT('',#51024);
#15714=VERTEX_POINT('',#51026);
#15715=VERTEX_POINT('',#51030);
#15716=VERTEX_POINT('',#51031);
#15717=VERTEX_POINT('',#51034);
#15718=VERTEX_POINT('',#51041);
#15719=VERTEX_POINT('',#51042);
#15720=VERTEX_POINT('',#51044);
#15721=VERTEX_POINT('',#51048);
#15722=VERTEX_POINT('',#51049);
#15723=VERTEX_POINT('',#51052);
#15724=VERTEX_POINT('',#51062);
#15725=VERTEX_POINT('',#51069);
#15726=VERTEX_POINT('',#51078);
#15727=VERTEX_POINT('',#51079);
#15728=VERTEX_POINT('',#51081);
#15729=VERTEX_POINT('',#51085);
#15730=VERTEX_POINT('',#51086);
#15731=VERTEX_POINT('',#51088);
#15732=VERTEX_POINT('',#51092);
#15733=VERTEX_POINT('',#51093);
#15734=VERTEX_POINT('',#51095);
#15735=VERTEX_POINT('',#51102);
#15736=VERTEX_POINT('',#51103);
#15737=VERTEX_POINT('',#51105);
#15738=VERTEX_POINT('',#51133);
#15739=VERTEX_POINT('',#51134);
#15740=VERTEX_POINT('',#51136);
#15741=VERTEX_POINT('',#51140);
#15742=VERTEX_POINT('',#51141);
#15743=VERTEX_POINT('',#51143);
#15744=VERTEX_POINT('',#51147);
#15745=VERTEX_POINT('',#51148);
#15746=VERTEX_POINT('',#51150);
#15747=VERTEX_POINT('',#51157);
#15748=VERTEX_POINT('',#51158);
#15749=VERTEX_POINT('',#51160);
#15750=VERTEX_POINT('',#51188);
#15751=VERTEX_POINT('',#51189);
#15752=VERTEX_POINT('',#51192);
#15753=VERTEX_POINT('',#51196);
#15754=VERTEX_POINT('',#51200);
#15755=VERTEX_POINT('',#51202);
#15756=VERTEX_POINT('',#51206);
#15757=VERTEX_POINT('',#51208);
#15758=VERTEX_POINT('',#51212);
#15759=VERTEX_POINT('',#51216);
#15760=VERTEX_POINT('',#51223);
#15761=VERTEX_POINT('',#51224);
#15762=VERTEX_POINT('',#51226);
#15763=VERTEX_POINT('',#51243);
#15764=VERTEX_POINT('',#51244);
#15765=VERTEX_POINT('',#51246);
#15766=VERTEX_POINT('',#51250);
#15767=VERTEX_POINT('',#51251);
#15768=VERTEX_POINT('',#51253);
#15769=VERTEX_POINT('',#51257);
#15770=VERTEX_POINT('',#51258);
#15771=VERTEX_POINT('',#51260);
#15772=VERTEX_POINT('',#51267);
#15773=VERTEX_POINT('',#51268);
#15774=VERTEX_POINT('',#51270);
#15775=VERTEX_POINT('',#51298);
#15776=VERTEX_POINT('',#51299);
#15777=VERTEX_POINT('',#51301);
#15778=VERTEX_POINT('',#51305);
#15779=VERTEX_POINT('',#51306);
#15780=VERTEX_POINT('',#51309);
#15781=VERTEX_POINT('',#51316);
#15782=VERTEX_POINT('',#51317);
#15783=VERTEX_POINT('',#51319);
#15784=VERTEX_POINT('',#51323);
#15785=VERTEX_POINT('',#51324);
#15786=VERTEX_POINT('',#51327);
#15787=VERTEX_POINT('',#51337);
#15788=VERTEX_POINT('',#51344);
#15789=VERTEX_POINT('',#51353);
#15790=VERTEX_POINT('',#51354);
#15791=VERTEX_POINT('',#51356);
#15792=VERTEX_POINT('',#51360);
#15793=VERTEX_POINT('',#51361);
#15794=VERTEX_POINT('',#51363);
#15795=VERTEX_POINT('',#51367);
#15796=VERTEX_POINT('',#51368);
#15797=VERTEX_POINT('',#51370);
#15798=VERTEX_POINT('',#51377);
#15799=VERTEX_POINT('',#51378);
#15800=VERTEX_POINT('',#51380);
#15801=VERTEX_POINT('',#51408);
#15802=VERTEX_POINT('',#51409);
#15803=VERTEX_POINT('',#51411);
#15804=VERTEX_POINT('',#51415);
#15805=VERTEX_POINT('',#51416);
#15806=VERTEX_POINT('',#51418);
#15807=VERTEX_POINT('',#51422);
#15808=VERTEX_POINT('',#51423);
#15809=VERTEX_POINT('',#51425);
#15810=VERTEX_POINT('',#51432);
#15811=VERTEX_POINT('',#51433);
#15812=VERTEX_POINT('',#51435);
#15813=VERTEX_POINT('',#51463);
#15814=VERTEX_POINT('',#51464);
#15815=VERTEX_POINT('',#51467);
#15816=VERTEX_POINT('',#51471);
#15817=VERTEX_POINT('',#51475);
#15818=VERTEX_POINT('',#51477);
#15819=VERTEX_POINT('',#51481);
#15820=VERTEX_POINT('',#51483);
#15821=VERTEX_POINT('',#51487);
#15822=VERTEX_POINT('',#51491);
#15823=VERTEX_POINT('',#51498);
#15824=VERTEX_POINT('',#51499);
#15825=VERTEX_POINT('',#51501);
#15826=VERTEX_POINT('',#51518);
#15827=VERTEX_POINT('',#51519);
#15828=VERTEX_POINT('',#51521);
#15829=VERTEX_POINT('',#51525);
#15830=VERTEX_POINT('',#51526);
#15831=VERTEX_POINT('',#51528);
#15832=VERTEX_POINT('',#51532);
#15833=VERTEX_POINT('',#51533);
#15834=VERTEX_POINT('',#51535);
#15835=VERTEX_POINT('',#51542);
#15836=VERTEX_POINT('',#51543);
#15837=VERTEX_POINT('',#51545);
#15838=VERTEX_POINT('',#51573);
#15839=VERTEX_POINT('',#51574);
#15840=VERTEX_POINT('',#51576);
#15841=VERTEX_POINT('',#51580);
#15842=VERTEX_POINT('',#51581);
#15843=VERTEX_POINT('',#51584);
#15844=VERTEX_POINT('',#51591);
#15845=VERTEX_POINT('',#51592);
#15846=VERTEX_POINT('',#51594);
#15847=VERTEX_POINT('',#51598);
#15848=VERTEX_POINT('',#51599);
#15849=VERTEX_POINT('',#51602);
#15850=VERTEX_POINT('',#51612);
#15851=VERTEX_POINT('',#51619);
#15852=VERTEX_POINT('',#51628);
#15853=VERTEX_POINT('',#51629);
#15854=VERTEX_POINT('',#51631);
#15855=VERTEX_POINT('',#51635);
#15856=VERTEX_POINT('',#51636);
#15857=VERTEX_POINT('',#51638);
#15858=VERTEX_POINT('',#51642);
#15859=VERTEX_POINT('',#51643);
#15860=VERTEX_POINT('',#51645);
#15861=VERTEX_POINT('',#51652);
#15862=VERTEX_POINT('',#51653);
#15863=VERTEX_POINT('',#51655);
#15864=VERTEX_POINT('',#51683);
#15865=VERTEX_POINT('',#51684);
#15866=VERTEX_POINT('',#51686);
#15867=VERTEX_POINT('',#51690);
#15868=VERTEX_POINT('',#51691);
#15869=VERTEX_POINT('',#51693);
#15870=VERTEX_POINT('',#51697);
#15871=VERTEX_POINT('',#51698);
#15872=VERTEX_POINT('',#51700);
#15873=VERTEX_POINT('',#51707);
#15874=VERTEX_POINT('',#51708);
#15875=VERTEX_POINT('',#51710);
#15876=VERTEX_POINT('',#51738);
#15877=VERTEX_POINT('',#51739);
#15878=VERTEX_POINT('',#51742);
#15879=VERTEX_POINT('',#51746);
#15880=VERTEX_POINT('',#51750);
#15881=VERTEX_POINT('',#51752);
#15882=VERTEX_POINT('',#51756);
#15883=VERTEX_POINT('',#51758);
#15884=VERTEX_POINT('',#51762);
#15885=VERTEX_POINT('',#51766);
#15886=VERTEX_POINT('',#51773);
#15887=VERTEX_POINT('',#51774);
#15888=VERTEX_POINT('',#51776);
#15889=VERTEX_POINT('',#51793);
#15890=VERTEX_POINT('',#51794);
#15891=VERTEX_POINT('',#51796);
#15892=VERTEX_POINT('',#51800);
#15893=VERTEX_POINT('',#51801);
#15894=VERTEX_POINT('',#51803);
#15895=VERTEX_POINT('',#51807);
#15896=VERTEX_POINT('',#51808);
#15897=VERTEX_POINT('',#51810);
#15898=VERTEX_POINT('',#51817);
#15899=VERTEX_POINT('',#51818);
#15900=VERTEX_POINT('',#51820);
#15901=VERTEX_POINT('',#51848);
#15902=VERTEX_POINT('',#51849);
#15903=VERTEX_POINT('',#51851);
#15904=VERTEX_POINT('',#51855);
#15905=VERTEX_POINT('',#51856);
#15906=VERTEX_POINT('',#51859);
#15907=VERTEX_POINT('',#51866);
#15908=VERTEX_POINT('',#51867);
#15909=VERTEX_POINT('',#51869);
#15910=VERTEX_POINT('',#51873);
#15911=VERTEX_POINT('',#51874);
#15912=VERTEX_POINT('',#51877);
#15913=VERTEX_POINT('',#51887);
#15914=VERTEX_POINT('',#51894);
#15915=VERTEX_POINT('',#51903);
#15916=VERTEX_POINT('',#51904);
#15917=VERTEX_POINT('',#51906);
#15918=VERTEX_POINT('',#51910);
#15919=VERTEX_POINT('',#51911);
#15920=VERTEX_POINT('',#51913);
#15921=VERTEX_POINT('',#51917);
#15922=VERTEX_POINT('',#51918);
#15923=VERTEX_POINT('',#51920);
#15924=VERTEX_POINT('',#51927);
#15925=VERTEX_POINT('',#51928);
#15926=VERTEX_POINT('',#51930);
#15927=VERTEX_POINT('',#51958);
#15928=VERTEX_POINT('',#51959);
#15929=VERTEX_POINT('',#51961);
#15930=VERTEX_POINT('',#51965);
#15931=VERTEX_POINT('',#51966);
#15932=VERTEX_POINT('',#51968);
#15933=VERTEX_POINT('',#51972);
#15934=VERTEX_POINT('',#51973);
#15935=VERTEX_POINT('',#51975);
#15936=VERTEX_POINT('',#51982);
#15937=VERTEX_POINT('',#51983);
#15938=VERTEX_POINT('',#51985);
#15939=VERTEX_POINT('',#52013);
#15940=VERTEX_POINT('',#52014);
#15941=VERTEX_POINT('',#52017);
#15942=VERTEX_POINT('',#52021);
#15943=VERTEX_POINT('',#52025);
#15944=VERTEX_POINT('',#52027);
#15945=VERTEX_POINT('',#52031);
#15946=VERTEX_POINT('',#52033);
#15947=VERTEX_POINT('',#52037);
#15948=VERTEX_POINT('',#52041);
#15949=VERTEX_POINT('',#52048);
#15950=VERTEX_POINT('',#52049);
#15951=VERTEX_POINT('',#52051);
#15952=VERTEX_POINT('',#52068);
#15953=VERTEX_POINT('',#52069);
#15954=VERTEX_POINT('',#52071);
#15955=VERTEX_POINT('',#52075);
#15956=VERTEX_POINT('',#52076);
#15957=VERTEX_POINT('',#52078);
#15958=VERTEX_POINT('',#52082);
#15959=VERTEX_POINT('',#52083);
#15960=VERTEX_POINT('',#52085);
#15961=VERTEX_POINT('',#52092);
#15962=VERTEX_POINT('',#52093);
#15963=VERTEX_POINT('',#52095);
#15964=VERTEX_POINT('',#52123);
#15965=VERTEX_POINT('',#52124);
#15966=VERTEX_POINT('',#52126);
#15967=VERTEX_POINT('',#52130);
#15968=VERTEX_POINT('',#52131);
#15969=VERTEX_POINT('',#52134);
#15970=VERTEX_POINT('',#52141);
#15971=VERTEX_POINT('',#52142);
#15972=VERTEX_POINT('',#52144);
#15973=VERTEX_POINT('',#52148);
#15974=VERTEX_POINT('',#52149);
#15975=VERTEX_POINT('',#52152);
#15976=VERTEX_POINT('',#52162);
#15977=VERTEX_POINT('',#52169);
#15978=VERTEX_POINT('',#52178);
#15979=VERTEX_POINT('',#52179);
#15980=VERTEX_POINT('',#52181);
#15981=VERTEX_POINT('',#52185);
#15982=VERTEX_POINT('',#52186);
#15983=VERTEX_POINT('',#52188);
#15984=VERTEX_POINT('',#52192);
#15985=VERTEX_POINT('',#52193);
#15986=VERTEX_POINT('',#52195);
#15987=VERTEX_POINT('',#52202);
#15988=VERTEX_POINT('',#52203);
#15989=VERTEX_POINT('',#52205);
#15990=VERTEX_POINT('',#52233);
#15991=VERTEX_POINT('',#52234);
#15992=VERTEX_POINT('',#52236);
#15993=VERTEX_POINT('',#52240);
#15994=VERTEX_POINT('',#52241);
#15995=VERTEX_POINT('',#52243);
#15996=VERTEX_POINT('',#52247);
#15997=VERTEX_POINT('',#52248);
#15998=VERTEX_POINT('',#52250);
#15999=VERTEX_POINT('',#52257);
#16000=VERTEX_POINT('',#52258);
#16001=VERTEX_POINT('',#52260);
#16002=VERTEX_POINT('',#52288);
#16003=VERTEX_POINT('',#52289);
#16004=VERTEX_POINT('',#52292);
#16005=VERTEX_POINT('',#52296);
#16006=VERTEX_POINT('',#52300);
#16007=VERTEX_POINT('',#52302);
#16008=VERTEX_POINT('',#52306);
#16009=VERTEX_POINT('',#52308);
#16010=VERTEX_POINT('',#52312);
#16011=VERTEX_POINT('',#52316);
#16012=VERTEX_POINT('',#52323);
#16013=VERTEX_POINT('',#52324);
#16014=VERTEX_POINT('',#52326);
#16015=VERTEX_POINT('',#52343);
#16016=VERTEX_POINT('',#52344);
#16017=VERTEX_POINT('',#52346);
#16018=VERTEX_POINT('',#52350);
#16019=VERTEX_POINT('',#52351);
#16020=VERTEX_POINT('',#52353);
#16021=VERTEX_POINT('',#52357);
#16022=VERTEX_POINT('',#52358);
#16023=VERTEX_POINT('',#52360);
#16024=VERTEX_POINT('',#52367);
#16025=VERTEX_POINT('',#52368);
#16026=VERTEX_POINT('',#52370);
#16027=VERTEX_POINT('',#52398);
#16028=VERTEX_POINT('',#52399);
#16029=VERTEX_POINT('',#52401);
#16030=VERTEX_POINT('',#52405);
#16031=VERTEX_POINT('',#52406);
#16032=VERTEX_POINT('',#52409);
#16033=VERTEX_POINT('',#52416);
#16034=VERTEX_POINT('',#52417);
#16035=VERTEX_POINT('',#52419);
#16036=VERTEX_POINT('',#52423);
#16037=VERTEX_POINT('',#52424);
#16038=VERTEX_POINT('',#52427);
#16039=VERTEX_POINT('',#52437);
#16040=VERTEX_POINT('',#52444);
#16041=VERTEX_POINT('',#52453);
#16042=VERTEX_POINT('',#52454);
#16043=VERTEX_POINT('',#52456);
#16044=VERTEX_POINT('',#52460);
#16045=VERTEX_POINT('',#52461);
#16046=VERTEX_POINT('',#52463);
#16047=VERTEX_POINT('',#52467);
#16048=VERTEX_POINT('',#52468);
#16049=VERTEX_POINT('',#52470);
#16050=VERTEX_POINT('',#52477);
#16051=VERTEX_POINT('',#52478);
#16052=VERTEX_POINT('',#52480);
#16053=VERTEX_POINT('',#52508);
#16054=VERTEX_POINT('',#52509);
#16055=VERTEX_POINT('',#52511);
#16056=VERTEX_POINT('',#52515);
#16057=VERTEX_POINT('',#52516);
#16058=VERTEX_POINT('',#52518);
#16059=VERTEX_POINT('',#52522);
#16060=VERTEX_POINT('',#52523);
#16061=VERTEX_POINT('',#52525);
#16062=VERTEX_POINT('',#52532);
#16063=VERTEX_POINT('',#52533);
#16064=VERTEX_POINT('',#52535);
#16065=VERTEX_POINT('',#52563);
#16066=VERTEX_POINT('',#52564);
#16067=VERTEX_POINT('',#52567);
#16068=VERTEX_POINT('',#52569);
#16069=VERTEX_POINT('',#52573);
#16070=VERTEX_POINT('',#52575);
#16071=VERTEX_POINT('',#52579);
#16072=VERTEX_POINT('',#52583);
#16073=VERTEX_POINT('',#52584);
#16074=VERTEX_POINT('',#52586);
#16075=VERTEX_POINT('',#52590);
#16076=VERTEX_POINT('',#52591);
#16077=VERTEX_POINT('',#52593);
#16078=VERTEX_POINT('',#52597);
#16079=VERTEX_POINT('',#52598);
#16080=VERTEX_POINT('',#52600);
#16081=VERTEX_POINT('',#52607);
#16082=VERTEX_POINT('',#52608);
#16083=VERTEX_POINT('',#52610);
#16084=VERTEX_POINT('',#52638);
#16085=VERTEX_POINT('',#52639);
#16086=VERTEX_POINT('',#52641);
#16087=VERTEX_POINT('',#52645);
#16088=VERTEX_POINT('',#52646);
#16089=VERTEX_POINT('',#52648);
#16090=VERTEX_POINT('',#52652);
#16091=VERTEX_POINT('',#52653);
#16092=VERTEX_POINT('',#52655);
#16093=VERTEX_POINT('',#52662);
#16094=VERTEX_POINT('',#52663);
#16095=VERTEX_POINT('',#52665);
#16096=VERTEX_POINT('',#52693);
#16097=VERTEX_POINT('',#52694);
#16098=VERTEX_POINT('',#52697);
#16099=VERTEX_POINT('',#52699);
#16100=VERTEX_POINT('',#52703);
#16101=VERTEX_POINT('',#52705);
#16102=VERTEX_POINT('',#52711);
#16103=VERTEX_POINT('',#52715);
#16104=VERTEX_POINT('',#52718);
#16105=VERTEX_POINT('',#52722);
#16106=VERTEX_POINT('',#52872);
#16107=VERTEX_POINT('',#52876);
#16108=VERTEX_POINT('',#52880);
#16109=VERTEX_POINT('',#52884);
#16110=VERTEX_POINT('',#52888);
#16111=VERTEX_POINT('',#52892);
#16112=VERTEX_POINT('',#52894);
#16113=VERTEX_POINT('',#52898);
#16114=VERTEX_POINT('',#52902);
#16115=VERTEX_POINT('',#52906);
#16116=VERTEX_POINT('',#52910);
#16117=VERTEX_POINT('',#52917);
#16118=VERTEX_POINT('',#52922);
#16119=VERTEX_POINT('',#52927);
#16120=VERTEX_POINT('',#52931);
#16121=VERTEX_POINT('',#52934);
#16122=VERTEX_POINT('',#52940);
#16123=VERTEX_POINT('',#52944);
#16124=VERTEX_POINT('',#52947);
#17453=EDGE_CURVE('',#14532,#14533,#13634,.T.);
#17454=EDGE_CURVE('',#14533,#14532,#13635,.T.);
#17455=EDGE_CURVE('',#14532,#14534,#7534,.T.);
#17456=EDGE_CURVE('',#14534,#14535,#13636,.T.);
#17457=EDGE_CURVE('',#14535,#14534,#13637,.T.);
#17458=EDGE_CURVE('',#14535,#14536,#7535,.T.);
#17459=EDGE_CURVE('',#14537,#14536,#13638,.T.);
#17460=EDGE_CURVE('',#14536,#14537,#13639,.T.);
#17461=EDGE_CURVE('',#14538,#14538,#13640,.T.);
#17462=EDGE_CURVE('',#14538,#14533,#7536,.T.);
#17463=EDGE_CURVE('',#14537,#14539,#7537,.T.);
#17464=EDGE_CURVE('',#14539,#14539,#13641,.T.);
#17465=EDGE_CURVE('',#14540,#14540,#13642,.T.);
#17466=EDGE_CURVE('',#14541,#14541,#13643,.T.);
#17467=EDGE_CURVE('',#14541,#14542,#7538,.T.);
#17468=EDGE_CURVE('',#14542,#14543,#13644,.T.);
#17469=EDGE_CURVE('',#14543,#14542,#13645,.T.);
#17470=EDGE_CURVE('',#14544,#14544,#13646,.T.);
#17471=EDGE_CURVE('',#14544,#14543,#7539,.T.);
#17472=EDGE_CURVE('',#14545,#14545,#13647,.T.);
#17473=EDGE_CURVE('',#14546,#14546,#13648,.T.);
#17474=EDGE_CURVE('',#14546,#14547,#7540,.T.);
#17475=EDGE_CURVE('',#14547,#14548,#13649,.T.);
#17476=EDGE_CURVE('',#14548,#14547,#13650,.T.);
#17477=EDGE_CURVE('',#14548,#14549,#7541,.T.);
#17478=EDGE_CURVE('',#14550,#14549,#13651,.T.);
#17479=EDGE_CURVE('',#14549,#14550,#13652,.T.);
#17480=EDGE_CURVE('',#14551,#14551,#13653,.T.);
#17481=EDGE_CURVE('',#14550,#14552,#7542,.T.);
#17482=EDGE_CURVE('',#14552,#14553,#13654,.T.);
#17483=EDGE_CURVE('',#14553,#14552,#13655,.T.);
#17484=EDGE_CURVE('',#14553,#14554,#7543,.T.);
#17485=EDGE_CURVE('',#14554,#14554,#13656,.T.);
#17486=EDGE_CURVE('',#14555,#14556,#13657,.T.);
#17487=EDGE_CURVE('',#14556,#14555,#13658,.T.);
#17488=EDGE_CURVE('',#14555,#14557,#7544,.T.);
#17489=EDGE_CURVE('',#14557,#14558,#13659,.T.);
#17490=EDGE_CURVE('',#14558,#14557,#13660,.T.);
#17491=EDGE_CURVE('',#14558,#14559,#7545,.T.);
#17492=EDGE_CURVE('',#14560,#14559,#13661,.T.);
#17493=EDGE_CURVE('',#14559,#14560,#13662,.T.);
#17494=EDGE_CURVE('',#14561,#14561,#13663,.T.);
#17495=EDGE_CURVE('',#14561,#14556,#7546,.T.);
#17496=EDGE_CURVE('',#14560,#14562,#7547,.T.);
#17497=EDGE_CURVE('',#14562,#14563,#13664,.T.);
#17498=EDGE_CURVE('',#14563,#14562,#13665,.T.);
#17499=EDGE_CURVE('',#14563,#14564,#7548,.T.);
#17500=EDGE_CURVE('',#14565,#14564,#13666,.T.);
#17501=EDGE_CURVE('',#14564,#14565,#13667,.T.);
#17502=EDGE_CURVE('',#14565,#14566,#7549,.T.);
#17503=EDGE_CURVE('',#14566,#14567,#13668,.T.);
#17504=EDGE_CURVE('',#14567,#14566,#13669,.T.);
#17505=EDGE_CURVE('',#14567,#14568,#7550,.T.);
#17506=EDGE_CURVE('',#14569,#14568,#13670,.T.);
#17507=EDGE_CURVE('',#14568,#14569,#13671,.T.);
#17508=EDGE_CURVE('',#14569,#14570,#7551,.T.);
#17509=EDGE_CURVE('',#14570,#14571,#13672,.T.);
#17510=EDGE_CURVE('',#14571,#14570,#13673,.T.);
#17511=EDGE_CURVE('',#14571,#14572,#7552,.T.);
#17512=EDGE_CURVE('',#14572,#14573,#13674,.T.);
#17513=EDGE_CURVE('',#14574,#14573,#842,.F.);
#17514=EDGE_CURVE('',#14574,#14575,#7553,.T.);
#17515=EDGE_CURVE('',#14576,#14575,#843,.F.);
#17516=EDGE_CURVE('',#14576,#14577,#13675,.T.);
#17517=EDGE_CURVE('',#14577,#14578,#7554,.T.);
#17518=EDGE_CURVE('',#14578,#14578,#13676,.T.);
#17519=EDGE_CURVE('',#14577,#14579,#13677,.T.);
#17520=EDGE_CURVE('',#14580,#14579,#844,.F.);
#17521=EDGE_CURVE('',#14580,#14581,#7555,.T.);
#17522=EDGE_CURVE('',#14582,#14581,#845,.F.);
#17523=EDGE_CURVE('',#14582,#14572,#13678,.T.);
#17524=EDGE_CURVE('',#14583,#14584,#7556,.T.);
#17525=EDGE_CURVE('',#14585,#14584,#846,.F.);
#17526=EDGE_CURVE('',#14585,#14586,#13679,.T.);
#17527=EDGE_CURVE('',#14587,#14586,#847,.F.);
#17528=EDGE_CURVE('',#14587,#14588,#7557,.T.);
#17529=EDGE_CURVE('',#14589,#14588,#848,.F.);
#17530=EDGE_CURVE('',#14589,#14590,#13680,.T.);
#17531=EDGE_CURVE('',#14583,#14590,#849,.F.);
#17532=EDGE_CURVE('',#14591,#14592,#7558,.T.);
#17533=EDGE_CURVE('',#14593,#14592,#850,.F.);
#17534=EDGE_CURVE('',#14593,#14594,#13681,.T.);
#17535=EDGE_CURVE('',#14595,#14594,#851,.F.);
#17536=EDGE_CURVE('',#14595,#14596,#7559,.T.);
#17537=EDGE_CURVE('',#14597,#14596,#852,.F.);
#17538=EDGE_CURVE('',#14597,#14598,#13682,.T.);
#17539=EDGE_CURVE('',#14591,#14598,#853,.F.);
#17540=EDGE_CURVE('',#14599,#14600,#7560,.T.);
#17541=EDGE_CURVE('',#14601,#14600,#854,.F.);
#17542=EDGE_CURVE('',#14601,#14602,#13683,.T.);
#17543=EDGE_CURVE('',#14603,#14602,#855,.F.);
#17544=EDGE_CURVE('',#14603,#14604,#7561,.T.);
#17545=EDGE_CURVE('',#14605,#14604,#856,.F.);
#17546=EDGE_CURVE('',#14605,#14606,#13684,.T.);
#17547=EDGE_CURVE('',#14599,#14606,#857,.F.);
#17548=EDGE_CURVE('',#14607,#14608,#7562,.T.);
#17549=EDGE_CURVE('',#14609,#14608,#858,.F.);
#17550=EDGE_CURVE('',#14609,#14610,#13685,.T.);
#17551=EDGE_CURVE('',#14611,#14610,#859,.F.);
#17552=EDGE_CURVE('',#14611,#14612,#7563,.T.);
#17553=EDGE_CURVE('',#14613,#14612,#860,.F.);
#17554=EDGE_CURVE('',#14613,#14614,#13686,.T.);
#17555=EDGE_CURVE('',#14607,#14614,#861,.F.);
#17556=EDGE_CURVE('',#14615,#14616,#7564,.T.);
#17557=EDGE_CURVE('',#14617,#14616,#862,.F.);
#17558=EDGE_CURVE('',#14617,#14618,#13687,.T.);
#17559=EDGE_CURVE('',#14619,#14618,#863,.F.);
#17560=EDGE_CURVE('',#14619,#14620,#7565,.T.);
#17561=EDGE_CURVE('',#14621,#14620,#864,.F.);
#17562=EDGE_CURVE('',#14621,#14622,#13688,.T.);
#17563=EDGE_CURVE('',#14615,#14622,#865,.F.);
#17564=EDGE_CURVE('',#14623,#14624,#7566,.T.);
#17565=EDGE_CURVE('',#14625,#14624,#866,.F.);
#17566=EDGE_CURVE('',#14625,#14626,#13689,.T.);
#17567=EDGE_CURVE('',#14627,#14626,#867,.F.);
#17568=EDGE_CURVE('',#14627,#14628,#7567,.T.);
#17569=EDGE_CURVE('',#14629,#14628,#868,.F.);
#17570=EDGE_CURVE('',#14629,#14630,#13690,.T.);
#17571=EDGE_CURVE('',#14623,#14630,#869,.F.);
#17572=EDGE_CURVE('',#14631,#14632,#7568,.T.);
#17573=EDGE_CURVE('',#14633,#14632,#870,.F.);
#17574=EDGE_CURVE('',#14633,#14634,#13691,.T.);
#17575=EDGE_CURVE('',#14635,#14634,#871,.F.);
#17576=EDGE_CURVE('',#14635,#14636,#7569,.T.);
#17577=EDGE_CURVE('',#14637,#14636,#872,.F.);
#17578=EDGE_CURVE('',#14637,#14638,#13692,.T.);
#17579=EDGE_CURVE('',#14631,#14638,#873,.F.);
#17580=EDGE_CURVE('',#14639,#14640,#7570,.T.);
#17581=EDGE_CURVE('',#14641,#14640,#874,.F.);
#17582=EDGE_CURVE('',#14641,#14642,#13693,.T.);
#17583=EDGE_CURVE('',#14643,#14642,#875,.F.);
#17584=EDGE_CURVE('',#14643,#14644,#7571,.T.);
#17585=EDGE_CURVE('',#14645,#14644,#876,.F.);
#17586=EDGE_CURVE('',#14645,#14646,#13694,.T.);
#17587=EDGE_CURVE('',#14639,#14646,#877,.F.);
#17588=EDGE_CURVE('',#14647,#14648,#7572,.T.);
#17589=EDGE_CURVE('',#14649,#14648,#878,.F.);
#17590=EDGE_CURVE('',#14649,#14650,#13695,.T.);
#17591=EDGE_CURVE('',#14651,#14650,#879,.F.);
#17592=EDGE_CURVE('',#14651,#14652,#7573,.T.);
#17593=EDGE_CURVE('',#14653,#14652,#880,.F.);
#17594=EDGE_CURVE('',#14653,#14654,#13696,.T.);
#17595=EDGE_CURVE('',#14647,#14654,#881,.F.);
#17596=EDGE_CURVE('',#14655,#14656,#7574,.T.);
#17597=EDGE_CURVE('',#14657,#14656,#882,.F.);
#17598=EDGE_CURVE('',#14657,#14658,#13697,.T.);
#17599=EDGE_CURVE('',#14659,#14658,#883,.F.);
#17600=EDGE_CURVE('',#14659,#14660,#7575,.T.);
#17601=EDGE_CURVE('',#14661,#14660,#884,.F.);
#17602=EDGE_CURVE('',#14661,#14662,#13698,.T.);
#17603=EDGE_CURVE('',#14655,#14662,#885,.F.);
#17604=EDGE_CURVE('',#14663,#14664,#7576,.T.);
#17605=EDGE_CURVE('',#14665,#14664,#886,.F.);
#17606=EDGE_CURVE('',#14665,#14666,#13699,.T.);
#17607=EDGE_CURVE('',#14667,#14666,#887,.F.);
#17608=EDGE_CURVE('',#14667,#14668,#7577,.T.);
#17609=EDGE_CURVE('',#14669,#14668,#888,.F.);
#17610=EDGE_CURVE('',#14669,#14670,#13700,.T.);
#17611=EDGE_CURVE('',#14663,#14670,#889,.F.);
#17612=EDGE_CURVE('',#14671,#14672,#7578,.T.);
#17613=EDGE_CURVE('',#14673,#14672,#890,.F.);
#17614=EDGE_CURVE('',#14673,#14674,#13701,.T.);
#17615=EDGE_CURVE('',#14675,#14674,#891,.F.);
#17616=EDGE_CURVE('',#14675,#14676,#7579,.T.);
#17617=EDGE_CURVE('',#14677,#14676,#892,.F.);
#17618=EDGE_CURVE('',#14677,#14678,#13702,.T.);
#17619=EDGE_CURVE('',#14671,#14678,#893,.F.);
#17620=EDGE_CURVE('',#14679,#14680,#7580,.T.);
#17621=EDGE_CURVE('',#14681,#14680,#894,.F.);
#17622=EDGE_CURVE('',#14681,#14682,#13703,.T.);
#17623=EDGE_CURVE('',#14683,#14682,#895,.F.);
#17624=EDGE_CURVE('',#14683,#14684,#7581,.T.);
#17625=EDGE_CURVE('',#14685,#14684,#896,.F.);
#17626=EDGE_CURVE('',#14685,#14686,#13704,.T.);
#17627=EDGE_CURVE('',#14679,#14686,#897,.F.);
#17628=EDGE_CURVE('',#14687,#14688,#7582,.T.);
#17629=EDGE_CURVE('',#14689,#14688,#898,.F.);
#17630=EDGE_CURVE('',#14689,#14690,#13705,.T.);
#17631=EDGE_CURVE('',#14691,#14690,#899,.F.);
#17632=EDGE_CURVE('',#14691,#14692,#7583,.T.);
#17633=EDGE_CURVE('',#14693,#14692,#900,.F.);
#17634=EDGE_CURVE('',#14693,#14694,#13706,.T.);
#17635=EDGE_CURVE('',#14687,#14694,#901,.F.);
#17636=EDGE_CURVE('',#14695,#14696,#7584,.T.);
#17637=EDGE_CURVE('',#14697,#14696,#902,.F.);
#17638=EDGE_CURVE('',#14697,#14698,#13707,.T.);
#17639=EDGE_CURVE('',#14699,#14698,#903,.F.);
#17640=EDGE_CURVE('',#14699,#14700,#7585,.T.);
#17641=EDGE_CURVE('',#14701,#14700,#904,.F.);
#17642=EDGE_CURVE('',#14701,#14702,#13708,.T.);
#17643=EDGE_CURVE('',#14695,#14702,#905,.F.);
#17644=EDGE_CURVE('',#14703,#14704,#7586,.T.);
#17645=EDGE_CURVE('',#14705,#14704,#906,.F.);
#17646=EDGE_CURVE('',#14705,#14706,#13709,.T.);
#17647=EDGE_CURVE('',#14707,#14706,#907,.F.);
#17648=EDGE_CURVE('',#14707,#14708,#7587,.T.);
#17649=EDGE_CURVE('',#14709,#14708,#908,.F.);
#17650=EDGE_CURVE('',#14709,#14710,#13710,.T.);
#17651=EDGE_CURVE('',#14703,#14710,#909,.F.);
#17652=EDGE_CURVE('',#14711,#14712,#7588,.T.);
#17653=EDGE_CURVE('',#14713,#14712,#910,.F.);
#17654=EDGE_CURVE('',#14713,#14714,#13711,.T.);
#17655=EDGE_CURVE('',#14715,#14714,#911,.F.);
#17656=EDGE_CURVE('',#14715,#14716,#7589,.T.);
#17657=EDGE_CURVE('',#14717,#14716,#912,.F.);
#17658=EDGE_CURVE('',#14717,#14718,#13712,.T.);
#17659=EDGE_CURVE('',#14711,#14718,#913,.F.);
#17660=EDGE_CURVE('',#14719,#14720,#7590,.T.);
#17661=EDGE_CURVE('',#14721,#14720,#914,.F.);
#17662=EDGE_CURVE('',#14721,#14722,#13713,.T.);
#17663=EDGE_CURVE('',#14723,#14722,#915,.F.);
#17664=EDGE_CURVE('',#14723,#14724,#7591,.T.);
#17665=EDGE_CURVE('',#14725,#14724,#916,.F.);
#17666=EDGE_CURVE('',#14725,#14726,#13714,.T.);
#17667=EDGE_CURVE('',#14719,#14726,#917,.F.);
#17668=EDGE_CURVE('',#14727,#14728,#7592,.T.);
#17669=EDGE_CURVE('',#14729,#14728,#918,.F.);
#17670=EDGE_CURVE('',#14729,#14730,#13715,.T.);
#17671=EDGE_CURVE('',#14731,#14730,#919,.F.);
#17672=EDGE_CURVE('',#14731,#14732,#7593,.T.);
#17673=EDGE_CURVE('',#14733,#14732,#920,.F.);
#17674=EDGE_CURVE('',#14733,#14734,#13716,.T.);
#17675=EDGE_CURVE('',#14727,#14734,#921,.F.);
#17676=EDGE_CURVE('',#14735,#14736,#7594,.T.);
#17677=EDGE_CURVE('',#14737,#14736,#922,.F.);
#17678=EDGE_CURVE('',#14737,#14738,#13717,.T.);
#17679=EDGE_CURVE('',#14739,#14738,#923,.F.);
#17680=EDGE_CURVE('',#14739,#14740,#7595,.T.);
#17681=EDGE_CURVE('',#14741,#14740,#924,.F.);
#17682=EDGE_CURVE('',#14741,#14742,#13718,.T.);
#17683=EDGE_CURVE('',#14735,#14742,#925,.F.);
#17684=EDGE_CURVE('',#14743,#14744,#7596,.T.);
#17685=EDGE_CURVE('',#14745,#14744,#926,.F.);
#17686=EDGE_CURVE('',#14745,#14746,#13719,.T.);
#17687=EDGE_CURVE('',#14747,#14746,#927,.F.);
#17688=EDGE_CURVE('',#14747,#14748,#7597,.T.);
#17689=EDGE_CURVE('',#14749,#14748,#928,.F.);
#17690=EDGE_CURVE('',#14749,#14750,#13720,.T.);
#17691=EDGE_CURVE('',#14743,#14750,#929,.F.);
#17692=EDGE_CURVE('',#14751,#14752,#7598,.T.);
#17693=EDGE_CURVE('',#14753,#14752,#930,.F.);
#17694=EDGE_CURVE('',#14753,#14754,#13721,.T.);
#17695=EDGE_CURVE('',#14755,#14754,#931,.F.);
#17696=EDGE_CURVE('',#14755,#14756,#7599,.T.);
#17697=EDGE_CURVE('',#14757,#14756,#932,.F.);
#17698=EDGE_CURVE('',#14757,#14758,#13722,.T.);
#17699=EDGE_CURVE('',#14751,#14758,#933,.F.);
#17700=EDGE_CURVE('',#14759,#14760,#7600,.T.);
#17701=EDGE_CURVE('',#14761,#14760,#934,.F.);
#17702=EDGE_CURVE('',#14761,#14762,#13723,.T.);
#17703=EDGE_CURVE('',#14763,#14762,#935,.F.);
#17704=EDGE_CURVE('',#14763,#14764,#7601,.T.);
#17705=EDGE_CURVE('',#14765,#14764,#936,.F.);
#17706=EDGE_CURVE('',#14765,#14766,#13724,.T.);
#17707=EDGE_CURVE('',#14759,#14766,#937,.F.);
#17708=EDGE_CURVE('',#14767,#14768,#7602,.T.);
#17709=EDGE_CURVE('',#14769,#14768,#938,.F.);
#17710=EDGE_CURVE('',#14769,#14770,#13725,.T.);
#17711=EDGE_CURVE('',#14771,#14770,#939,.F.);
#17712=EDGE_CURVE('',#14771,#14772,#7603,.T.);
#17713=EDGE_CURVE('',#14773,#14772,#940,.F.);
#17714=EDGE_CURVE('',#14773,#14774,#13726,.T.);
#17715=EDGE_CURVE('',#14767,#14774,#941,.F.);
#17716=EDGE_CURVE('',#14775,#14776,#7604,.T.);
#17717=EDGE_CURVE('',#14777,#14776,#942,.F.);
#17718=EDGE_CURVE('',#14777,#14778,#13727,.T.);
#17719=EDGE_CURVE('',#14779,#14778,#943,.F.);
#17720=EDGE_CURVE('',#14779,#14780,#7605,.T.);
#17721=EDGE_CURVE('',#14781,#14780,#944,.F.);
#17722=EDGE_CURVE('',#14781,#14782,#13728,.T.);
#17723=EDGE_CURVE('',#14775,#14782,#945,.F.);
#17724=EDGE_CURVE('',#14783,#14784,#7606,.T.);
#17725=EDGE_CURVE('',#14785,#14784,#946,.F.);
#17726=EDGE_CURVE('',#14785,#14786,#13729,.T.);
#17727=EDGE_CURVE('',#14787,#14786,#947,.F.);
#17728=EDGE_CURVE('',#14787,#14788,#7607,.T.);
#17729=EDGE_CURVE('',#14789,#14788,#948,.F.);
#17730=EDGE_CURVE('',#14789,#14790,#13730,.T.);
#17731=EDGE_CURVE('',#14783,#14790,#949,.F.);
#17732=EDGE_CURVE('',#14791,#14792,#7608,.T.);
#17733=EDGE_CURVE('',#14793,#14792,#950,.F.);
#17734=EDGE_CURVE('',#14793,#14794,#13731,.T.);
#17735=EDGE_CURVE('',#14795,#14794,#951,.F.);
#17736=EDGE_CURVE('',#14795,#14796,#7609,.T.);
#17737=EDGE_CURVE('',#14797,#14796,#952,.F.);
#17738=EDGE_CURVE('',#14797,#14798,#13732,.T.);
#17739=EDGE_CURVE('',#14791,#14798,#953,.F.);
#17740=EDGE_CURVE('',#14799,#14800,#7610,.T.);
#17741=EDGE_CURVE('',#14801,#14800,#954,.F.);
#17742=EDGE_CURVE('',#14801,#14802,#13733,.T.);
#17743=EDGE_CURVE('',#14803,#14802,#955,.F.);
#17744=EDGE_CURVE('',#14803,#14804,#7611,.T.);
#17745=EDGE_CURVE('',#14805,#14804,#956,.F.);
#17746=EDGE_CURVE('',#14805,#14806,#13734,.T.);
#17747=EDGE_CURVE('',#14799,#14806,#957,.F.);
#17748=EDGE_CURVE('',#14807,#14808,#7612,.T.);
#17749=EDGE_CURVE('',#14809,#14808,#958,.F.);
#17750=EDGE_CURVE('',#14809,#14810,#13735,.T.);
#17751=EDGE_CURVE('',#14811,#14810,#959,.F.);
#17752=EDGE_CURVE('',#14811,#14812,#7613,.T.);
#17753=EDGE_CURVE('',#14813,#14812,#960,.F.);
#17754=EDGE_CURVE('',#14813,#14814,#13736,.T.);
#17755=EDGE_CURVE('',#14807,#14814,#961,.F.);
#17756=EDGE_CURVE('',#14815,#14816,#7614,.T.);
#17757=EDGE_CURVE('',#14817,#14816,#962,.F.);
#17758=EDGE_CURVE('',#14817,#14818,#13737,.T.);
#17759=EDGE_CURVE('',#14819,#14818,#963,.F.);
#17760=EDGE_CURVE('',#14819,#14820,#7615,.T.);
#17761=EDGE_CURVE('',#14821,#14820,#964,.F.);
#17762=EDGE_CURVE('',#14821,#14822,#13738,.T.);
#17763=EDGE_CURVE('',#14815,#14822,#965,.F.);
#17764=EDGE_CURVE('',#14823,#14824,#7616,.T.);
#17765=EDGE_CURVE('',#14825,#14824,#966,.F.);
#17766=EDGE_CURVE('',#14825,#14826,#13739,.T.);
#17767=EDGE_CURVE('',#14827,#14826,#967,.F.);
#17768=EDGE_CURVE('',#14827,#14828,#7617,.T.);
#17769=EDGE_CURVE('',#14829,#14828,#968,.F.);
#17770=EDGE_CURVE('',#14829,#14830,#13740,.T.);
#17771=EDGE_CURVE('',#14823,#14830,#969,.F.);
#17772=EDGE_CURVE('',#14831,#14832,#7618,.T.);
#17773=EDGE_CURVE('',#14833,#14832,#970,.F.);
#17774=EDGE_CURVE('',#14833,#14834,#13741,.T.);
#17775=EDGE_CURVE('',#14835,#14834,#971,.F.);
#17776=EDGE_CURVE('',#14835,#14836,#7619,.T.);
#17777=EDGE_CURVE('',#14837,#14836,#972,.F.);
#17778=EDGE_CURVE('',#14837,#14838,#13742,.T.);
#17779=EDGE_CURVE('',#14831,#14838,#973,.F.);
#17780=EDGE_CURVE('',#14839,#14840,#7620,.T.);
#17781=EDGE_CURVE('',#14841,#14840,#974,.F.);
#17782=EDGE_CURVE('',#14841,#14842,#13743,.T.);
#17783=EDGE_CURVE('',#14843,#14842,#975,.F.);
#17784=EDGE_CURVE('',#14843,#14844,#7621,.T.);
#17785=EDGE_CURVE('',#14845,#14844,#976,.F.);
#17786=EDGE_CURVE('',#14845,#14846,#13744,.T.);
#17787=EDGE_CURVE('',#14839,#14846,#977,.F.);
#17788=EDGE_CURVE('',#14847,#14848,#7622,.T.);
#17789=EDGE_CURVE('',#14849,#14848,#978,.F.);
#17790=EDGE_CURVE('',#14849,#14850,#13745,.T.);
#17791=EDGE_CURVE('',#14851,#14850,#979,.F.);
#17792=EDGE_CURVE('',#14851,#14852,#7623,.T.);
#17793=EDGE_CURVE('',#14853,#14852,#980,.F.);
#17794=EDGE_CURVE('',#14853,#14854,#13746,.T.);
#17795=EDGE_CURVE('',#14847,#14854,#981,.F.);
#17796=EDGE_CURVE('',#14855,#14856,#7624,.T.);
#17797=EDGE_CURVE('',#14857,#14856,#982,.F.);
#17798=EDGE_CURVE('',#14857,#14858,#13747,.T.);
#17799=EDGE_CURVE('',#14859,#14858,#983,.F.);
#17800=EDGE_CURVE('',#14859,#14860,#7625,.T.);
#17801=EDGE_CURVE('',#14861,#14860,#984,.F.);
#17802=EDGE_CURVE('',#14861,#14862,#13748,.T.);
#17803=EDGE_CURVE('',#14855,#14862,#985,.F.);
#17804=EDGE_CURVE('',#14863,#14864,#7626,.T.);
#17805=EDGE_CURVE('',#14865,#14864,#986,.F.);
#17806=EDGE_CURVE('',#14865,#14866,#13749,.T.);
#17807=EDGE_CURVE('',#14867,#14866,#987,.F.);
#17808=EDGE_CURVE('',#14867,#14868,#7627,.T.);
#17809=EDGE_CURVE('',#14869,#14868,#988,.F.);
#17810=EDGE_CURVE('',#14869,#14870,#13750,.T.);
#17811=EDGE_CURVE('',#14863,#14870,#989,.F.);
#17812=EDGE_CURVE('',#14871,#14872,#7628,.T.);
#17813=EDGE_CURVE('',#14873,#14872,#990,.F.);
#17814=EDGE_CURVE('',#14873,#14874,#13751,.T.);
#17815=EDGE_CURVE('',#14875,#14874,#991,.F.);
#17816=EDGE_CURVE('',#14875,#14876,#7629,.T.);
#17817=EDGE_CURVE('',#14877,#14876,#992,.F.);
#17818=EDGE_CURVE('',#14877,#14878,#13752,.T.);
#17819=EDGE_CURVE('',#14871,#14878,#993,.F.);
#17820=EDGE_CURVE('',#14879,#14880,#7630,.T.);
#17821=EDGE_CURVE('',#14881,#14880,#994,.F.);
#17822=EDGE_CURVE('',#14881,#14882,#13753,.T.);
#17823=EDGE_CURVE('',#14883,#14882,#995,.F.);
#17824=EDGE_CURVE('',#14883,#14884,#7631,.T.);
#17825=EDGE_CURVE('',#14885,#14884,#996,.F.);
#17826=EDGE_CURVE('',#14885,#14886,#13754,.T.);
#17827=EDGE_CURVE('',#14879,#14886,#997,.F.);
#17828=EDGE_CURVE('',#14887,#14888,#7632,.T.);
#17829=EDGE_CURVE('',#14889,#14888,#998,.F.);
#17830=EDGE_CURVE('',#14889,#14890,#13755,.T.);
#17831=EDGE_CURVE('',#14891,#14890,#999,.F.);
#17832=EDGE_CURVE('',#14891,#14892,#7633,.T.);
#17833=EDGE_CURVE('',#14893,#14892,#1000,.F.);
#17834=EDGE_CURVE('',#14893,#14894,#13756,.T.);
#17835=EDGE_CURVE('',#14887,#14894,#1001,.F.);
#17836=EDGE_CURVE('',#14895,#14896,#7634,.T.);
#17837=EDGE_CURVE('',#14897,#14896,#1002,.F.);
#17838=EDGE_CURVE('',#14897,#14898,#13757,.T.);
#17839=EDGE_CURVE('',#14899,#14898,#1003,.F.);
#17840=EDGE_CURVE('',#14899,#14900,#7635,.T.);
#17841=EDGE_CURVE('',#14901,#14900,#1004,.F.);
#17842=EDGE_CURVE('',#14901,#14902,#13758,.T.);
#17843=EDGE_CURVE('',#14895,#14902,#1005,.F.);
#17844=EDGE_CURVE('',#14903,#14904,#7636,.T.);
#17845=EDGE_CURVE('',#14905,#14904,#1006,.F.);
#17846=EDGE_CURVE('',#14905,#14906,#13759,.T.);
#17847=EDGE_CURVE('',#14907,#14906,#1007,.F.);
#17848=EDGE_CURVE('',#14907,#14908,#7637,.T.);
#17849=EDGE_CURVE('',#14909,#14908,#1008,.F.);
#17850=EDGE_CURVE('',#14909,#14910,#13760,.T.);
#17851=EDGE_CURVE('',#14903,#14910,#1009,.F.);
#17852=EDGE_CURVE('',#14911,#14912,#7638,.T.);
#17853=EDGE_CURVE('',#14913,#14912,#1010,.F.);
#17854=EDGE_CURVE('',#14913,#14914,#13761,.T.);
#17855=EDGE_CURVE('',#14915,#14914,#1011,.F.);
#17856=EDGE_CURVE('',#14915,#14916,#7639,.T.);
#17857=EDGE_CURVE('',#14917,#14916,#1012,.F.);
#17858=EDGE_CURVE('',#14917,#14918,#13762,.T.);
#17859=EDGE_CURVE('',#14911,#14918,#1013,.F.);
#17860=EDGE_CURVE('',#14919,#14920,#7640,.T.);
#17861=EDGE_CURVE('',#14921,#14920,#1014,.F.);
#17862=EDGE_CURVE('',#14921,#14922,#13763,.T.);
#17863=EDGE_CURVE('',#14923,#14922,#1015,.F.);
#17864=EDGE_CURVE('',#14923,#14924,#7641,.T.);
#17865=EDGE_CURVE('',#14925,#14924,#1016,.F.);
#17866=EDGE_CURVE('',#14925,#14926,#13764,.T.);
#17867=EDGE_CURVE('',#14919,#14926,#1017,.F.);
#17868=EDGE_CURVE('',#14927,#14928,#7642,.T.);
#17869=EDGE_CURVE('',#14929,#14928,#1018,.F.);
#17870=EDGE_CURVE('',#14929,#14930,#13765,.T.);
#17871=EDGE_CURVE('',#14931,#14930,#1019,.F.);
#17872=EDGE_CURVE('',#14931,#14932,#7643,.T.);
#17873=EDGE_CURVE('',#14933,#14932,#1020,.F.);
#17874=EDGE_CURVE('',#14933,#14934,#13766,.T.);
#17875=EDGE_CURVE('',#14927,#14934,#1021,.F.);
#17876=EDGE_CURVE('',#14935,#14936,#7644,.T.);
#17877=EDGE_CURVE('',#14937,#14936,#1022,.F.);
#17878=EDGE_CURVE('',#14937,#14938,#13767,.T.);
#17879=EDGE_CURVE('',#14939,#14938,#1023,.F.);
#17880=EDGE_CURVE('',#14939,#14940,#7645,.T.);
#17881=EDGE_CURVE('',#14941,#14940,#1024,.F.);
#17882=EDGE_CURVE('',#14941,#14942,#13768,.T.);
#17883=EDGE_CURVE('',#14935,#14942,#1025,.F.);
#17884=EDGE_CURVE('',#14943,#14944,#7646,.T.);
#17885=EDGE_CURVE('',#14945,#14944,#1026,.F.);
#17886=EDGE_CURVE('',#14945,#14946,#13769,.T.);
#17887=EDGE_CURVE('',#14947,#14946,#1027,.F.);
#17888=EDGE_CURVE('',#14947,#14948,#7647,.T.);
#17889=EDGE_CURVE('',#14949,#14948,#1028,.F.);
#17890=EDGE_CURVE('',#14949,#14950,#13770,.T.);
#17891=EDGE_CURVE('',#14943,#14950,#1029,.F.);
#17892=EDGE_CURVE('',#14951,#14952,#7648,.T.);
#17893=EDGE_CURVE('',#14953,#14952,#1030,.F.);
#17894=EDGE_CURVE('',#14953,#14954,#13771,.T.);
#17895=EDGE_CURVE('',#14955,#14954,#1031,.F.);
#17896=EDGE_CURVE('',#14955,#14956,#7649,.T.);
#17897=EDGE_CURVE('',#14957,#14956,#1032,.F.);
#17898=EDGE_CURVE('',#14957,#14958,#13772,.T.);
#17899=EDGE_CURVE('',#14951,#14958,#1033,.F.);
#17900=EDGE_CURVE('',#14959,#14960,#7650,.T.);
#17901=EDGE_CURVE('',#14961,#14960,#1034,.F.);
#17902=EDGE_CURVE('',#14961,#14962,#13773,.T.);
#17903=EDGE_CURVE('',#14963,#14962,#1035,.F.);
#17904=EDGE_CURVE('',#14963,#14964,#7651,.T.);
#17905=EDGE_CURVE('',#14965,#14964,#1036,.F.);
#17906=EDGE_CURVE('',#14965,#14966,#13774,.T.);
#17907=EDGE_CURVE('',#14959,#14966,#1037,.F.);
#17908=EDGE_CURVE('',#14967,#14968,#7652,.T.);
#17909=EDGE_CURVE('',#14969,#14968,#1038,.F.);
#17910=EDGE_CURVE('',#14969,#14970,#13775,.T.);
#17911=EDGE_CURVE('',#14971,#14970,#1039,.F.);
#17912=EDGE_CURVE('',#14971,#14972,#7653,.T.);
#17913=EDGE_CURVE('',#14973,#14972,#1040,.F.);
#17914=EDGE_CURVE('',#14973,#14974,#13776,.T.);
#17915=EDGE_CURVE('',#14967,#14974,#1041,.F.);
#17916=EDGE_CURVE('',#14975,#14976,#7654,.T.);
#17917=EDGE_CURVE('',#14977,#14976,#1042,.F.);
#17918=EDGE_CURVE('',#14977,#14978,#13777,.T.);
#17919=EDGE_CURVE('',#14979,#14978,#1043,.F.);
#17920=EDGE_CURVE('',#14979,#14980,#7655,.T.);
#17921=EDGE_CURVE('',#14981,#14980,#1044,.F.);
#17922=EDGE_CURVE('',#14981,#14982,#13778,.T.);
#17923=EDGE_CURVE('',#14975,#14982,#1045,.F.);
#17924=EDGE_CURVE('',#14983,#14984,#7656,.T.);
#17925=EDGE_CURVE('',#14985,#14984,#1046,.F.);
#17926=EDGE_CURVE('',#14985,#14986,#13779,.T.);
#17927=EDGE_CURVE('',#14987,#14986,#1047,.F.);
#17928=EDGE_CURVE('',#14987,#14988,#7657,.T.);
#17929=EDGE_CURVE('',#14989,#14988,#1048,.F.);
#17930=EDGE_CURVE('',#14989,#14990,#13780,.T.);
#17931=EDGE_CURVE('',#14983,#14990,#1049,.F.);
#17932=EDGE_CURVE('',#14991,#14992,#7658,.T.);
#17933=EDGE_CURVE('',#14993,#14992,#1050,.F.);
#17934=EDGE_CURVE('',#14993,#14994,#13781,.T.);
#17935=EDGE_CURVE('',#14995,#14994,#1051,.F.);
#17936=EDGE_CURVE('',#14995,#14996,#7659,.T.);
#17937=EDGE_CURVE('',#14997,#14996,#1052,.F.);
#17938=EDGE_CURVE('',#14997,#14998,#13782,.T.);
#17939=EDGE_CURVE('',#14991,#14998,#1053,.F.);
#17940=EDGE_CURVE('',#14999,#15000,#7660,.T.);
#17941=EDGE_CURVE('',#15001,#15000,#1054,.F.);
#17942=EDGE_CURVE('',#15001,#15002,#13783,.T.);
#17943=EDGE_CURVE('',#15003,#15002,#1055,.F.);
#17944=EDGE_CURVE('',#15003,#15004,#7661,.T.);
#17945=EDGE_CURVE('',#15005,#15004,#1056,.F.);
#17946=EDGE_CURVE('',#15005,#15006,#13784,.T.);
#17947=EDGE_CURVE('',#14999,#15006,#1057,.F.);
#17948=EDGE_CURVE('',#15007,#15008,#7662,.T.);
#17949=EDGE_CURVE('',#15009,#15008,#1058,.F.);
#17950=EDGE_CURVE('',#15009,#15010,#13785,.T.);
#17951=EDGE_CURVE('',#15011,#15010,#1059,.F.);
#17952=EDGE_CURVE('',#15011,#15012,#7663,.T.);
#17953=EDGE_CURVE('',#15013,#15012,#1060,.F.);
#17954=EDGE_CURVE('',#15013,#15014,#13786,.T.);
#17955=EDGE_CURVE('',#15007,#15014,#1061,.F.);
#17956=EDGE_CURVE('',#15015,#15016,#7664,.T.);
#17957=EDGE_CURVE('',#15017,#15016,#1062,.F.);
#17958=EDGE_CURVE('',#15017,#15018,#13787,.T.);
#17959=EDGE_CURVE('',#15019,#15018,#1063,.F.);
#17960=EDGE_CURVE('',#15019,#15020,#7665,.T.);
#17961=EDGE_CURVE('',#15021,#15020,#1064,.F.);
#17962=EDGE_CURVE('',#15021,#15022,#13788,.T.);
#17963=EDGE_CURVE('',#15015,#15022,#1065,.F.);
#17964=EDGE_CURVE('',#15023,#15024,#7666,.T.);
#17965=EDGE_CURVE('',#15025,#15024,#1066,.F.);
#17966=EDGE_CURVE('',#15025,#15026,#13789,.T.);
#17967=EDGE_CURVE('',#15027,#15026,#1067,.F.);
#17968=EDGE_CURVE('',#15027,#15028,#7667,.T.);
#17969=EDGE_CURVE('',#15029,#15028,#1068,.F.);
#17970=EDGE_CURVE('',#15029,#15030,#13790,.T.);
#17971=EDGE_CURVE('',#15023,#15030,#1069,.F.);
#17972=EDGE_CURVE('',#15031,#15032,#7668,.T.);
#17973=EDGE_CURVE('',#15033,#15032,#1070,.F.);
#17974=EDGE_CURVE('',#15033,#15034,#13791,.T.);
#17975=EDGE_CURVE('',#15035,#15034,#1071,.F.);
#17976=EDGE_CURVE('',#15035,#15036,#7669,.T.);
#17977=EDGE_CURVE('',#15037,#15036,#1072,.F.);
#17978=EDGE_CURVE('',#15037,#15038,#13792,.T.);
#17979=EDGE_CURVE('',#15031,#15038,#1073,.F.);
#17980=EDGE_CURVE('',#15039,#15040,#7670,.T.);
#17981=EDGE_CURVE('',#15041,#15040,#1074,.F.);
#17982=EDGE_CURVE('',#15041,#15042,#13793,.T.);
#17983=EDGE_CURVE('',#15043,#15042,#1075,.F.);
#17984=EDGE_CURVE('',#15043,#15044,#7671,.T.);
#17985=EDGE_CURVE('',#15045,#15044,#1076,.F.);
#17986=EDGE_CURVE('',#15045,#15046,#13794,.T.);
#17987=EDGE_CURVE('',#15039,#15046,#1077,.F.);
#17988=EDGE_CURVE('',#15047,#15048,#7672,.T.);
#17989=EDGE_CURVE('',#15049,#15048,#1078,.F.);
#17990=EDGE_CURVE('',#15049,#15050,#13795,.T.);
#17991=EDGE_CURVE('',#15051,#15050,#1079,.F.);
#17992=EDGE_CURVE('',#15051,#15052,#7673,.T.);
#17993=EDGE_CURVE('',#15053,#15052,#1080,.F.);
#17994=EDGE_CURVE('',#15053,#15054,#13796,.T.);
#17995=EDGE_CURVE('',#15047,#15054,#1081,.F.);
#17996=EDGE_CURVE('',#15055,#15056,#7674,.T.);
#17997=EDGE_CURVE('',#15057,#15056,#1082,.F.);
#17998=EDGE_CURVE('',#15057,#15058,#13797,.T.);
#17999=EDGE_CURVE('',#15059,#15058,#1083,.F.);
#18000=EDGE_CURVE('',#15059,#15060,#7675,.T.);
#18001=EDGE_CURVE('',#15061,#15060,#1084,.F.);
#18002=EDGE_CURVE('',#15061,#15062,#13798,.T.);
#18003=EDGE_CURVE('',#15055,#15062,#1085,.F.);
#18004=EDGE_CURVE('',#15063,#15064,#7676,.T.);
#18005=EDGE_CURVE('',#15065,#15064,#1086,.F.);
#18006=EDGE_CURVE('',#15065,#15066,#13799,.T.);
#18007=EDGE_CURVE('',#15067,#15066,#1087,.F.);
#18008=EDGE_CURVE('',#15067,#15068,#7677,.T.);
#18009=EDGE_CURVE('',#15069,#15068,#1088,.F.);
#18010=EDGE_CURVE('',#15069,#15070,#13800,.T.);
#18011=EDGE_CURVE('',#15063,#15070,#1089,.F.);
#18012=EDGE_CURVE('',#15071,#15072,#7678,.T.);
#18013=EDGE_CURVE('',#15073,#15072,#1090,.F.);
#18014=EDGE_CURVE('',#15073,#15074,#13801,.T.);
#18015=EDGE_CURVE('',#15075,#15074,#1091,.F.);
#18016=EDGE_CURVE('',#15075,#15076,#7679,.T.);
#18017=EDGE_CURVE('',#15077,#15076,#1092,.F.);
#18018=EDGE_CURVE('',#15077,#15078,#13802,.T.);
#18019=EDGE_CURVE('',#15071,#15078,#1093,.F.);
#18020=EDGE_CURVE('',#15079,#15080,#7680,.T.);
#18021=EDGE_CURVE('',#15081,#15080,#1094,.F.);
#18022=EDGE_CURVE('',#15081,#15082,#13803,.T.);
#18023=EDGE_CURVE('',#15083,#15082,#1095,.F.);
#18024=EDGE_CURVE('',#15083,#15084,#7681,.T.);
#18025=EDGE_CURVE('',#15085,#15084,#1096,.F.);
#18026=EDGE_CURVE('',#15085,#15086,#13804,.T.);
#18027=EDGE_CURVE('',#15079,#15086,#1097,.F.);
#18028=EDGE_CURVE('',#15087,#15088,#7682,.T.);
#18029=EDGE_CURVE('',#15089,#15088,#1098,.F.);
#18030=EDGE_CURVE('',#15089,#15090,#13805,.T.);
#18031=EDGE_CURVE('',#15091,#15090,#1099,.F.);
#18032=EDGE_CURVE('',#15091,#15092,#7683,.T.);
#18033=EDGE_CURVE('',#15093,#15092,#1100,.F.);
#18034=EDGE_CURVE('',#15093,#15094,#13806,.T.);
#18035=EDGE_CURVE('',#15087,#15094,#1101,.F.);
#18036=EDGE_CURVE('',#15095,#15096,#7684,.T.);
#18037=EDGE_CURVE('',#15097,#15096,#1102,.F.);
#18038=EDGE_CURVE('',#15097,#15098,#13807,.T.);
#18039=EDGE_CURVE('',#15099,#15098,#1103,.F.);
#18040=EDGE_CURVE('',#15099,#15100,#7685,.T.);
#18041=EDGE_CURVE('',#15101,#15100,#1104,.F.);
#18042=EDGE_CURVE('',#15101,#15102,#13808,.T.);
#18043=EDGE_CURVE('',#15095,#15102,#1105,.F.);
#18044=EDGE_CURVE('',#15103,#15104,#7686,.T.);
#18045=EDGE_CURVE('',#15105,#15104,#1106,.F.);
#18046=EDGE_CURVE('',#15105,#15106,#13809,.T.);
#18047=EDGE_CURVE('',#15107,#15106,#1107,.F.);
#18048=EDGE_CURVE('',#15107,#15108,#7687,.T.);
#18049=EDGE_CURVE('',#15109,#15108,#1108,.F.);
#18050=EDGE_CURVE('',#15109,#15110,#13810,.T.);
#18051=EDGE_CURVE('',#15103,#15110,#1109,.F.);
#18052=EDGE_CURVE('',#15111,#15112,#7688,.T.);
#18053=EDGE_CURVE('',#15113,#15112,#1110,.F.);
#18054=EDGE_CURVE('',#15113,#15114,#13811,.T.);
#18055=EDGE_CURVE('',#15115,#15114,#1111,.F.);
#18056=EDGE_CURVE('',#15115,#15116,#7689,.T.);
#18057=EDGE_CURVE('',#15117,#15116,#1112,.F.);
#18058=EDGE_CURVE('',#15117,#15118,#13812,.T.);
#18059=EDGE_CURVE('',#15111,#15118,#1113,.F.);
#18060=EDGE_CURVE('',#15119,#15120,#7690,.T.);
#18061=EDGE_CURVE('',#15121,#15120,#1114,.F.);
#18062=EDGE_CURVE('',#15121,#15122,#13813,.T.);
#18063=EDGE_CURVE('',#15123,#15122,#1115,.F.);
#18064=EDGE_CURVE('',#15123,#15124,#7691,.T.);
#18065=EDGE_CURVE('',#15125,#15124,#1116,.F.);
#18066=EDGE_CURVE('',#15125,#15126,#13814,.T.);
#18067=EDGE_CURVE('',#15119,#15126,#1117,.F.);
#18068=EDGE_CURVE('',#15127,#15128,#7692,.T.);
#18069=EDGE_CURVE('',#15129,#15128,#1118,.F.);
#18070=EDGE_CURVE('',#15129,#15130,#13815,.T.);
#18071=EDGE_CURVE('',#15131,#15130,#1119,.F.);
#18072=EDGE_CURVE('',#15131,#15132,#7693,.T.);
#18073=EDGE_CURVE('',#15133,#15132,#1120,.F.);
#18074=EDGE_CURVE('',#15133,#15134,#13816,.T.);
#18075=EDGE_CURVE('',#15127,#15134,#1121,.F.);
#18076=EDGE_CURVE('',#15135,#15136,#7694,.T.);
#18077=EDGE_CURVE('',#15137,#15136,#1122,.F.);
#18078=EDGE_CURVE('',#15137,#15138,#13817,.T.);
#18079=EDGE_CURVE('',#15139,#15138,#1123,.F.);
#18080=EDGE_CURVE('',#15139,#15140,#7695,.T.);
#18081=EDGE_CURVE('',#15141,#15140,#1124,.F.);
#18082=EDGE_CURVE('',#15141,#15142,#13818,.T.);
#18083=EDGE_CURVE('',#15135,#15142,#1125,.F.);
#18084=EDGE_CURVE('',#15143,#15144,#7696,.T.);
#18085=EDGE_CURVE('',#15145,#15144,#1126,.F.);
#18086=EDGE_CURVE('',#15145,#15146,#13819,.T.);
#18087=EDGE_CURVE('',#15147,#15146,#1127,.F.);
#18088=EDGE_CURVE('',#15147,#15148,#7697,.T.);
#18089=EDGE_CURVE('',#15149,#15148,#1128,.F.);
#18090=EDGE_CURVE('',#15149,#15150,#13820,.T.);
#18091=EDGE_CURVE('',#15143,#15150,#1129,.F.);
#18092=EDGE_CURVE('',#15151,#15152,#13821,.T.);
#18093=EDGE_CURVE('',#15152,#15153,#347,.T.);
#18094=EDGE_CURVE('',#15153,#15154,#13822,.T.);
#18095=EDGE_CURVE('',#15151,#15154,#348,.T.);
#18096=EDGE_CURVE('',#15152,#15155,#13823,.T.);
#18097=EDGE_CURVE('',#15155,#15156,#349,.T.);
#18098=EDGE_CURVE('',#15156,#15153,#13824,.T.);
#18099=EDGE_CURVE('',#15155,#15157,#13825,.T.);
#18100=EDGE_CURVE('',#15157,#15158,#350,.T.);
#18101=EDGE_CURVE('',#15158,#15156,#13826,.T.);
#18102=EDGE_CURVE('',#15157,#15159,#13827,.T.);
#18103=EDGE_CURVE('',#15159,#15160,#351,.T.);
#18104=EDGE_CURVE('',#15160,#15158,#13828,.T.);
#18105=EDGE_CURVE('',#15159,#15161,#13829,.T.);
#18106=EDGE_CURVE('',#15161,#15162,#352,.T.);
#18107=EDGE_CURVE('',#15162,#15160,#13830,.T.);
#18108=EDGE_CURVE('',#15161,#15163,#13831,.T.);
#18109=EDGE_CURVE('',#15163,#15164,#353,.T.);
#18110=EDGE_CURVE('',#15164,#15162,#13832,.T.);
#18111=EDGE_CURVE('',#15165,#15164,#13833,.T.);
#18112=EDGE_CURVE('',#15163,#15166,#13834,.T.);
#18113=EDGE_CURVE('',#15166,#15165,#354,.T.);
#18114=EDGE_CURVE('',#15167,#15165,#13835,.T.);
#18115=EDGE_CURVE('',#15166,#15168,#13836,.T.);
#18116=EDGE_CURVE('',#15168,#15167,#355,.T.);
#18117=EDGE_CURVE('',#15169,#15167,#13837,.T.);
#18118=EDGE_CURVE('',#15168,#15170,#13838,.T.);
#18119=EDGE_CURVE('',#15170,#15169,#356,.T.);
#18120=EDGE_CURVE('',#15154,#15169,#13839,.T.);
#18121=EDGE_CURVE('',#15170,#15151,#13840,.T.);
#18122=EDGE_CURVE('',#15171,#15164,#7698,.T.);
#18123=EDGE_CURVE('',#15172,#15171,#13841,.T.);
#18124=EDGE_CURVE('',#15172,#15162,#7699,.T.);
#18125=EDGE_CURVE('',#15173,#15165,#7700,.T.);
#18126=EDGE_CURVE('',#15171,#15173,#13842,.T.);
#18127=EDGE_CURVE('',#15174,#15167,#7701,.T.);
#18128=EDGE_CURVE('',#15173,#15174,#13843,.T.);
#18129=EDGE_CURVE('',#15175,#15169,#7702,.T.);
#18130=EDGE_CURVE('',#15174,#15175,#13844,.T.);
#18131=EDGE_CURVE('',#15176,#15154,#7703,.T.);
#18132=EDGE_CURVE('',#15175,#15176,#13845,.T.);
#18133=EDGE_CURVE('',#15177,#15153,#7704,.T.);
#18134=EDGE_CURVE('',#15176,#15177,#13846,.T.);
#18135=EDGE_CURVE('',#15178,#15178,#13847,.T.);
#18136=EDGE_CURVE('',#15179,#15179,#13848,.T.);
#18137=EDGE_CURVE('',#15180,#15180,#13849,.T.);
#18138=EDGE_CURVE('',#15181,#15181,#13850,.T.);
#18139=EDGE_CURVE('',#15182,#15182,#13851,.T.);
#18140=EDGE_CURVE('',#15183,#15184,#7705,.T.);
#18141=EDGE_CURVE('',#15184,#14589,#7706,.T.);
#18142=EDGE_CURVE('',#14588,#15185,#7707,.T.);
#18143=EDGE_CURVE('',#15185,#15183,#7708,.T.);
#18144=EDGE_CURVE('',#15186,#15184,#7709,.T.);
#18145=EDGE_CURVE('',#14590,#15186,#7710,.T.);
#18146=EDGE_CURVE('',#15187,#15183,#7711,.T.);
#18147=EDGE_CURVE('',#15187,#15188,#7712,.T.);
#18148=EDGE_CURVE('',#15188,#15186,#7713,.T.);
#18149=EDGE_CURVE('',#15185,#15189,#7714,.T.);
#18150=EDGE_CURVE('',#15189,#15190,#7715,.T.);
#18151=EDGE_CURVE('',#15190,#15187,#7716,.T.);
#18152=EDGE_CURVE('',#15191,#15188,#7717,.T.);
#18153=EDGE_CURVE('',#15186,#15191,#7718,.T.);
#18154=EDGE_CURVE('',#15192,#15189,#7719,.T.);
#18155=EDGE_CURVE('',#15190,#15192,#7720,.T.);
#18156=EDGE_CURVE('',#14586,#15192,#7721,.T.);
#18157=EDGE_CURVE('',#15189,#14587,#7722,.T.);
#18158=EDGE_CURVE('',#15193,#15194,#7723,.T.);
#18159=EDGE_CURVE('',#15195,#15193,#7724,.T.);
#18160=EDGE_CURVE('',#15194,#15195,#7725,.T.);
#18161=EDGE_CURVE('',#14584,#15195,#7726,.T.);
#18162=EDGE_CURVE('',#15193,#14585,#7727,.T.);
#18163=EDGE_CURVE('',#15188,#15194,#7728,.T.);
#18164=EDGE_CURVE('',#15195,#15191,#7729,.T.);
#18165=EDGE_CURVE('',#15194,#15190,#7730,.T.);
#18166=EDGE_CURVE('',#15192,#15193,#7731,.T.);
#18167=EDGE_CURVE('',#15191,#14583,#7732,.T.);
#18168=EDGE_CURVE('',#15196,#15197,#7733,.T.);
#18169=EDGE_CURVE('',#15198,#15196,#7734,.T.);
#18170=EDGE_CURVE('',#15197,#15198,#7735,.T.);
#18171=EDGE_CURVE('',#15199,#15200,#7736,.T.);
#18172=EDGE_CURVE('',#15201,#15199,#7737,.T.);
#18173=EDGE_CURVE('',#15200,#15201,#7738,.T.);
#18174=EDGE_CURVE('',#15202,#15203,#7739,.T.);
#18175=EDGE_CURVE('',#15204,#15202,#7740,.T.);
#18176=EDGE_CURVE('',#15203,#15204,#7741,.T.);
#18177=EDGE_CURVE('',#14594,#15204,#7742,.T.);
#18178=EDGE_CURVE('',#15202,#14595,#7743,.T.);
#18179=EDGE_CURVE('',#15205,#15206,#7744,.T.);
#18180=EDGE_CURVE('',#15207,#15205,#7745,.T.);
#18181=EDGE_CURVE('',#15206,#15207,#7746,.T.);
#18182=EDGE_CURVE('',#14592,#15207,#7747,.T.);
#18183=EDGE_CURVE('',#15205,#14593,#7748,.T.);
#18184=EDGE_CURVE('',#15199,#15206,#7749,.T.);
#18185=EDGE_CURVE('',#15207,#15201,#7750,.T.);
#18186=EDGE_CURVE('',#15206,#15203,#7751,.T.);
#18187=EDGE_CURVE('',#15204,#15205,#7752,.T.);
#18188=EDGE_CURVE('',#15196,#15202,#7753,.T.);
#18189=EDGE_CURVE('',#15203,#15198,#7754,.T.);
#18190=EDGE_CURVE('',#14598,#15200,#7755,.T.);
#18191=EDGE_CURVE('',#15201,#14591,#7756,.T.);
#18192=EDGE_CURVE('',#15200,#15197,#7757,.T.);
#18193=EDGE_CURVE('',#15198,#15199,#7758,.T.);
#18194=EDGE_CURVE('',#14596,#15196,#7759,.T.);
#18195=EDGE_CURVE('',#15197,#14597,#7760,.T.);
#18196=EDGE_CURVE('',#15208,#15209,#7761,.T.);
#18197=EDGE_CURVE('',#15210,#15208,#7762,.T.);
#18198=EDGE_CURVE('',#15209,#15210,#7763,.T.);
#18199=EDGE_CURVE('',#15211,#15212,#7764,.T.);
#18200=EDGE_CURVE('',#15212,#15210,#7765,.T.);
#18201=EDGE_CURVE('',#15208,#15213,#7766,.T.);
#18202=EDGE_CURVE('',#15213,#15211,#7767,.T.);
#18203=EDGE_CURVE('',#14606,#15209,#7768,.T.);
#18204=EDGE_CURVE('',#15210,#14599,#7769,.T.);
#18205=EDGE_CURVE('',#15214,#15215,#7770,.T.);
#18206=EDGE_CURVE('',#15216,#15214,#7771,.T.);
#18207=EDGE_CURVE('',#15215,#15216,#7772,.T.);
#18208=EDGE_CURVE('',#15217,#15218,#7773,.T.);
#18209=EDGE_CURVE('',#15218,#15216,#7774,.T.);
#18210=EDGE_CURVE('',#15214,#15219,#7775,.T.);
#18211=EDGE_CURVE('',#15219,#15217,#7776,.T.);
#18212=EDGE_CURVE('',#15209,#15215,#7777,.T.);
#18213=EDGE_CURVE('',#15216,#15208,#7778,.T.);
#18214=EDGE_CURVE('',#14604,#15214,#7779,.T.);
#18215=EDGE_CURVE('',#15215,#14605,#7780,.T.);
#18216=EDGE_CURVE('',#15211,#15220,#7781,.T.);
#18217=EDGE_CURVE('',#15220,#14601,#7782,.T.);
#18218=EDGE_CURVE('',#14600,#15212,#7783,.T.);
#18219=EDGE_CURVE('',#15213,#15218,#7784,.T.);
#18220=EDGE_CURVE('',#15221,#15217,#7785,.T.);
#18221=EDGE_CURVE('',#15221,#15220,#7786,.T.);
#18222=EDGE_CURVE('',#15219,#14603,#7787,.T.);
#18223=EDGE_CURVE('',#14602,#15221,#7788,.T.);
#18224=EDGE_CURVE('',#15222,#15223,#7789,.T.);
#18225=EDGE_CURVE('',#15224,#15222,#7790,.T.);
#18226=EDGE_CURVE('',#15223,#15224,#7791,.T.);
#18227=EDGE_CURVE('',#15225,#15226,#7792,.T.);
#18228=EDGE_CURVE('',#15227,#15225,#7793,.T.);
#18229=EDGE_CURVE('',#15226,#15227,#7794,.T.);
#18230=EDGE_CURVE('',#15228,#15229,#7795,.T.);
#18231=EDGE_CURVE('',#15230,#15228,#7796,.T.);
#18232=EDGE_CURVE('',#15229,#15230,#7797,.T.);
#18233=EDGE_CURVE('',#14610,#15230,#7798,.T.);
#18234=EDGE_CURVE('',#15228,#14611,#7799,.T.);
#18235=EDGE_CURVE('',#15231,#15232,#7800,.T.);
#18236=EDGE_CURVE('',#15233,#15231,#7801,.T.);
#18237=EDGE_CURVE('',#15232,#15233,#7802,.T.);
#18238=EDGE_CURVE('',#14608,#15233,#7803,.T.);
#18239=EDGE_CURVE('',#15231,#14609,#7804,.T.);
#18240=EDGE_CURVE('',#15225,#15232,#7805,.T.);
#18241=EDGE_CURVE('',#15233,#15227,#7806,.T.);
#18242=EDGE_CURVE('',#15232,#15229,#7807,.T.);
#18243=EDGE_CURVE('',#15230,#15231,#7808,.T.);
#18244=EDGE_CURVE('',#15222,#15228,#7809,.T.);
#18245=EDGE_CURVE('',#15229,#15224,#7810,.T.);
#18246=EDGE_CURVE('',#14614,#15226,#7811,.T.);
#18247=EDGE_CURVE('',#15227,#14607,#7812,.T.);
#18248=EDGE_CURVE('',#15226,#15223,#7813,.T.);
#18249=EDGE_CURVE('',#15224,#15225,#7814,.T.);
#18250=EDGE_CURVE('',#14612,#15222,#7815,.T.);
#18251=EDGE_CURVE('',#15223,#14613,#7816,.T.);
#18252=EDGE_CURVE('',#15234,#15235,#7817,.T.);
#18253=EDGE_CURVE('',#15236,#15234,#7818,.T.);
#18254=EDGE_CURVE('',#15235,#15236,#7819,.T.);
#18255=EDGE_CURVE('',#15237,#15238,#7820,.T.);
#18256=EDGE_CURVE('',#15239,#15237,#7821,.T.);
#18257=EDGE_CURVE('',#15238,#15239,#7822,.T.);
#18258=EDGE_CURVE('',#15240,#15241,#7823,.T.);
#18259=EDGE_CURVE('',#15242,#15240,#7824,.T.);
#18260=EDGE_CURVE('',#15241,#15242,#7825,.T.);
#18261=EDGE_CURVE('',#14618,#15242,#7826,.T.);
#18262=EDGE_CURVE('',#15240,#14619,#7827,.T.);
#18263=EDGE_CURVE('',#15243,#15244,#7828,.T.);
#18264=EDGE_CURVE('',#15245,#15243,#7829,.T.);
#18265=EDGE_CURVE('',#15244,#15245,#7830,.T.);
#18266=EDGE_CURVE('',#14616,#15245,#7831,.T.);
#18267=EDGE_CURVE('',#15243,#14617,#7832,.T.);
#18268=EDGE_CURVE('',#15237,#15244,#7833,.T.);
#18269=EDGE_CURVE('',#15245,#15239,#7834,.T.);
#18270=EDGE_CURVE('',#15244,#15241,#7835,.T.);
#18271=EDGE_CURVE('',#15242,#15243,#7836,.T.);
#18272=EDGE_CURVE('',#15234,#15240,#7837,.T.);
#18273=EDGE_CURVE('',#15241,#15236,#7838,.T.);
#18274=EDGE_CURVE('',#14622,#15238,#7839,.T.);
#18275=EDGE_CURVE('',#15239,#14615,#7840,.T.);
#18276=EDGE_CURVE('',#15238,#15235,#7841,.T.);
#18277=EDGE_CURVE('',#15236,#15237,#7842,.T.);
#18278=EDGE_CURVE('',#14620,#15234,#7843,.T.);
#18279=EDGE_CURVE('',#15235,#14621,#7844,.T.);
#18280=EDGE_CURVE('',#15246,#15247,#7845,.T.);
#18281=EDGE_CURVE('',#15247,#14629,#7846,.T.);
#18282=EDGE_CURVE('',#14628,#15248,#7847,.T.);
#18283=EDGE_CURVE('',#15248,#15246,#7848,.T.);
#18284=EDGE_CURVE('',#15249,#15247,#7849,.T.);
#18285=EDGE_CURVE('',#14630,#15249,#7850,.T.);
#18286=EDGE_CURVE('',#15250,#15246,#7851,.T.);
#18287=EDGE_CURVE('',#15250,#15251,#7852,.T.);
#18288=EDGE_CURVE('',#15251,#15249,#7853,.T.);
#18289=EDGE_CURVE('',#15248,#15252,#7854,.T.);
#18290=EDGE_CURVE('',#15252,#15253,#7855,.T.);
#18291=EDGE_CURVE('',#15253,#15250,#7856,.T.);
#18292=EDGE_CURVE('',#15254,#15251,#7857,.T.);
#18293=EDGE_CURVE('',#15249,#15254,#7858,.T.);
#18294=EDGE_CURVE('',#15255,#15252,#7859,.T.);
#18295=EDGE_CURVE('',#15253,#15255,#7860,.T.);
#18296=EDGE_CURVE('',#14626,#15255,#7861,.T.);
#18297=EDGE_CURVE('',#15252,#14627,#7862,.T.);
#18298=EDGE_CURVE('',#15256,#15257,#7863,.T.);
#18299=EDGE_CURVE('',#15258,#15256,#7864,.T.);
#18300=EDGE_CURVE('',#15257,#15258,#7865,.T.);
#18301=EDGE_CURVE('',#14624,#15258,#7866,.T.);
#18302=EDGE_CURVE('',#15256,#14625,#7867,.T.);
#18303=EDGE_CURVE('',#15251,#15257,#7868,.T.);
#18304=EDGE_CURVE('',#15258,#15254,#7869,.T.);
#18305=EDGE_CURVE('',#15257,#15253,#7870,.T.);
#18306=EDGE_CURVE('',#15255,#15256,#7871,.T.);
#18307=EDGE_CURVE('',#15254,#14623,#7872,.T.);
#18308=EDGE_CURVE('',#15259,#15260,#7873,.T.);
#18309=EDGE_CURVE('',#15261,#15259,#7874,.T.);
#18310=EDGE_CURVE('',#15260,#15261,#7875,.T.);
#18311=EDGE_CURVE('',#15262,#15263,#7876,.T.);
#18312=EDGE_CURVE('',#15264,#15262,#7877,.T.);
#18313=EDGE_CURVE('',#15263,#15264,#7878,.T.);
#18314=EDGE_CURVE('',#15265,#15266,#7879,.T.);
#18315=EDGE_CURVE('',#15267,#15265,#7880,.T.);
#18316=EDGE_CURVE('',#15266,#15267,#7881,.T.);
#18317=EDGE_CURVE('',#14634,#15267,#7882,.T.);
#18318=EDGE_CURVE('',#15265,#14635,#7883,.T.);
#18319=EDGE_CURVE('',#15268,#15269,#7884,.T.);
#18320=EDGE_CURVE('',#15270,#15268,#7885,.T.);
#18321=EDGE_CURVE('',#15269,#15270,#7886,.T.);
#18322=EDGE_CURVE('',#14632,#15270,#7887,.T.);
#18323=EDGE_CURVE('',#15268,#14633,#7888,.T.);
#18324=EDGE_CURVE('',#15262,#15269,#7889,.T.);
#18325=EDGE_CURVE('',#15270,#15264,#7890,.T.);
#18326=EDGE_CURVE('',#15269,#15266,#7891,.T.);
#18327=EDGE_CURVE('',#15267,#15268,#7892,.T.);
#18328=EDGE_CURVE('',#15259,#15265,#7893,.T.);
#18329=EDGE_CURVE('',#15266,#15261,#7894,.T.);
#18330=EDGE_CURVE('',#14638,#15263,#7895,.T.);
#18331=EDGE_CURVE('',#15264,#14631,#7896,.T.);
#18332=EDGE_CURVE('',#15263,#15260,#7897,.T.);
#18333=EDGE_CURVE('',#15261,#15262,#7898,.T.);
#18334=EDGE_CURVE('',#14636,#15259,#7899,.T.);
#18335=EDGE_CURVE('',#15260,#14637,#7900,.T.);
#18336=EDGE_CURVE('',#15271,#15272,#7901,.T.);
#18337=EDGE_CURVE('',#15273,#15271,#7902,.T.);
#18338=EDGE_CURVE('',#15272,#15273,#7903,.T.);
#18339=EDGE_CURVE('',#15274,#15275,#7904,.T.);
#18340=EDGE_CURVE('',#15275,#15273,#7905,.T.);
#18341=EDGE_CURVE('',#15271,#15276,#7906,.T.);
#18342=EDGE_CURVE('',#15276,#15274,#7907,.T.);
#18343=EDGE_CURVE('',#14646,#15272,#7908,.T.);
#18344=EDGE_CURVE('',#15273,#14639,#7909,.T.);
#18345=EDGE_CURVE('',#15277,#15278,#7910,.T.);
#18346=EDGE_CURVE('',#15279,#15277,#7911,.T.);
#18347=EDGE_CURVE('',#15278,#15279,#7912,.T.);
#18348=EDGE_CURVE('',#15280,#15281,#7913,.T.);
#18349=EDGE_CURVE('',#15281,#15279,#7914,.T.);
#18350=EDGE_CURVE('',#15277,#15282,#7915,.T.);
#18351=EDGE_CURVE('',#15282,#15280,#7916,.T.);
#18352=EDGE_CURVE('',#15272,#15278,#7917,.T.);
#18353=EDGE_CURVE('',#15279,#15271,#7918,.T.);
#18354=EDGE_CURVE('',#14644,#15277,#7919,.T.);
#18355=EDGE_CURVE('',#15278,#14645,#7920,.T.);
#18356=EDGE_CURVE('',#15274,#15283,#7921,.T.);
#18357=EDGE_CURVE('',#15283,#14641,#7922,.T.);
#18358=EDGE_CURVE('',#14640,#15275,#7923,.T.);
#18359=EDGE_CURVE('',#15276,#15281,#7924,.T.);
#18360=EDGE_CURVE('',#15284,#15280,#7925,.T.);
#18361=EDGE_CURVE('',#15284,#15283,#7926,.T.);
#18362=EDGE_CURVE('',#15282,#14643,#7927,.T.);
#18363=EDGE_CURVE('',#14642,#15284,#7928,.T.);
#18364=EDGE_CURVE('',#15285,#15286,#7929,.T.);
#18365=EDGE_CURVE('',#15287,#15285,#7930,.T.);
#18366=EDGE_CURVE('',#15286,#15287,#7931,.T.);
#18367=EDGE_CURVE('',#15288,#15289,#7932,.T.);
#18368=EDGE_CURVE('',#15290,#15288,#7933,.T.);
#18369=EDGE_CURVE('',#15289,#15290,#7934,.T.);
#18370=EDGE_CURVE('',#15291,#15292,#7935,.T.);
#18371=EDGE_CURVE('',#15293,#15291,#7936,.T.);
#18372=EDGE_CURVE('',#15292,#15293,#7937,.T.);
#18373=EDGE_CURVE('',#14650,#15293,#7938,.T.);
#18374=EDGE_CURVE('',#15291,#14651,#7939,.T.);
#18375=EDGE_CURVE('',#15294,#15295,#7940,.T.);
#18376=EDGE_CURVE('',#15296,#15294,#7941,.T.);
#18377=EDGE_CURVE('',#15295,#15296,#7942,.T.);
#18378=EDGE_CURVE('',#14648,#15296,#7943,.T.);
#18379=EDGE_CURVE('',#15294,#14649,#7944,.T.);
#18380=EDGE_CURVE('',#15288,#15295,#7945,.T.);
#18381=EDGE_CURVE('',#15296,#15290,#7946,.T.);
#18382=EDGE_CURVE('',#15295,#15292,#7947,.T.);
#18383=EDGE_CURVE('',#15293,#15294,#7948,.T.);
#18384=EDGE_CURVE('',#15285,#15291,#7949,.T.);
#18385=EDGE_CURVE('',#15292,#15287,#7950,.T.);
#18386=EDGE_CURVE('',#14654,#15289,#7951,.T.);
#18387=EDGE_CURVE('',#15290,#14647,#7952,.T.);
#18388=EDGE_CURVE('',#15289,#15286,#7953,.T.);
#18389=EDGE_CURVE('',#15287,#15288,#7954,.T.);
#18390=EDGE_CURVE('',#14652,#15285,#7955,.T.);
#18391=EDGE_CURVE('',#15286,#14653,#7956,.T.);
#18392=EDGE_CURVE('',#15297,#15298,#7957,.T.);
#18393=EDGE_CURVE('',#15299,#15297,#7958,.T.);
#18394=EDGE_CURVE('',#15298,#15299,#7959,.T.);
#18395=EDGE_CURVE('',#15300,#15301,#7960,.T.);
#18396=EDGE_CURVE('',#15302,#15300,#7961,.T.);
#18397=EDGE_CURVE('',#15301,#15302,#7962,.T.);
#18398=EDGE_CURVE('',#15303,#15304,#7963,.T.);
#18399=EDGE_CURVE('',#15305,#15303,#7964,.T.);
#18400=EDGE_CURVE('',#15304,#15305,#7965,.T.);
#18401=EDGE_CURVE('',#14658,#15305,#7966,.T.);
#18402=EDGE_CURVE('',#15303,#14659,#7967,.T.);
#18403=EDGE_CURVE('',#15306,#15307,#7968,.T.);
#18404=EDGE_CURVE('',#15308,#15306,#7969,.T.);
#18405=EDGE_CURVE('',#15307,#15308,#7970,.T.);
#18406=EDGE_CURVE('',#14656,#15308,#7971,.T.);
#18407=EDGE_CURVE('',#15306,#14657,#7972,.T.);
#18408=EDGE_CURVE('',#15300,#15307,#7973,.T.);
#18409=EDGE_CURVE('',#15308,#15302,#7974,.T.);
#18410=EDGE_CURVE('',#15307,#15304,#7975,.T.);
#18411=EDGE_CURVE('',#15305,#15306,#7976,.T.);
#18412=EDGE_CURVE('',#15297,#15303,#7977,.T.);
#18413=EDGE_CURVE('',#15304,#15299,#7978,.T.);
#18414=EDGE_CURVE('',#14662,#15301,#7979,.T.);
#18415=EDGE_CURVE('',#15302,#14655,#7980,.T.);
#18416=EDGE_CURVE('',#15301,#15298,#7981,.T.);
#18417=EDGE_CURVE('',#15299,#15300,#7982,.T.);
#18418=EDGE_CURVE('',#14660,#15297,#7983,.T.);
#18419=EDGE_CURVE('',#15298,#14661,#7984,.T.);
#18420=EDGE_CURVE('',#15309,#15310,#7985,.T.);
#18421=EDGE_CURVE('',#15310,#14669,#7986,.T.);
#18422=EDGE_CURVE('',#14668,#15311,#7987,.T.);
#18423=EDGE_CURVE('',#15311,#15309,#7988,.T.);
#18424=EDGE_CURVE('',#15312,#15310,#7989,.T.);
#18425=EDGE_CURVE('',#14670,#15312,#7990,.T.);
#18426=EDGE_CURVE('',#15313,#15309,#7991,.T.);
#18427=EDGE_CURVE('',#15313,#15314,#7992,.T.);
#18428=EDGE_CURVE('',#15314,#15312,#7993,.T.);
#18429=EDGE_CURVE('',#15311,#15315,#7994,.T.);
#18430=EDGE_CURVE('',#15315,#15316,#7995,.T.);
#18431=EDGE_CURVE('',#15316,#15313,#7996,.T.);
#18432=EDGE_CURVE('',#15317,#15314,#7997,.T.);
#18433=EDGE_CURVE('',#15312,#15317,#7998,.T.);
#18434=EDGE_CURVE('',#15318,#15315,#7999,.T.);
#18435=EDGE_CURVE('',#15316,#15318,#8000,.T.);
#18436=EDGE_CURVE('',#14666,#15318,#8001,.T.);
#18437=EDGE_CURVE('',#15315,#14667,#8002,.T.);
#18438=EDGE_CURVE('',#15319,#15320,#8003,.T.);
#18439=EDGE_CURVE('',#15321,#15319,#8004,.T.);
#18440=EDGE_CURVE('',#15320,#15321,#8005,.T.);
#18441=EDGE_CURVE('',#14664,#15321,#8006,.T.);
#18442=EDGE_CURVE('',#15319,#14665,#8007,.T.);
#18443=EDGE_CURVE('',#15314,#15320,#8008,.T.);
#18444=EDGE_CURVE('',#15321,#15317,#8009,.T.);
#18445=EDGE_CURVE('',#15320,#15316,#8010,.T.);
#18446=EDGE_CURVE('',#15318,#15319,#8011,.T.);
#18447=EDGE_CURVE('',#15317,#14663,#8012,.T.);
#18448=EDGE_CURVE('',#15322,#15323,#8013,.T.);
#18449=EDGE_CURVE('',#15324,#15322,#8014,.T.);
#18450=EDGE_CURVE('',#15323,#15324,#8015,.T.);
#18451=EDGE_CURVE('',#15325,#15326,#8016,.T.);
#18452=EDGE_CURVE('',#15327,#15325,#8017,.T.);
#18453=EDGE_CURVE('',#15326,#15327,#8018,.T.);
#18454=EDGE_CURVE('',#15328,#15329,#8019,.T.);
#18455=EDGE_CURVE('',#15330,#15328,#8020,.T.);
#18456=EDGE_CURVE('',#15329,#15330,#8021,.T.);
#18457=EDGE_CURVE('',#14674,#15330,#8022,.T.);
#18458=EDGE_CURVE('',#15328,#14675,#8023,.T.);
#18459=EDGE_CURVE('',#15331,#15332,#8024,.T.);
#18460=EDGE_CURVE('',#15333,#15331,#8025,.T.);
#18461=EDGE_CURVE('',#15332,#15333,#8026,.T.);
#18462=EDGE_CURVE('',#14672,#15333,#8027,.T.);
#18463=EDGE_CURVE('',#15331,#14673,#8028,.T.);
#18464=EDGE_CURVE('',#15325,#15332,#8029,.T.);
#18465=EDGE_CURVE('',#15333,#15327,#8030,.T.);
#18466=EDGE_CURVE('',#15332,#15329,#8031,.T.);
#18467=EDGE_CURVE('',#15330,#15331,#8032,.T.);
#18468=EDGE_CURVE('',#15322,#15328,#8033,.T.);
#18469=EDGE_CURVE('',#15329,#15324,#8034,.T.);
#18470=EDGE_CURVE('',#14678,#15326,#8035,.T.);
#18471=EDGE_CURVE('',#15327,#14671,#8036,.T.);
#18472=EDGE_CURVE('',#15326,#15323,#8037,.T.);
#18473=EDGE_CURVE('',#15324,#15325,#8038,.T.);
#18474=EDGE_CURVE('',#14676,#15322,#8039,.T.);
#18475=EDGE_CURVE('',#15323,#14677,#8040,.T.);
#18476=EDGE_CURVE('',#15334,#15335,#8041,.T.);
#18477=EDGE_CURVE('',#15336,#15334,#8042,.T.);
#18478=EDGE_CURVE('',#15335,#15336,#8043,.T.);
#18479=EDGE_CURVE('',#15337,#15338,#8044,.T.);
#18480=EDGE_CURVE('',#15338,#15336,#8045,.T.);
#18481=EDGE_CURVE('',#15334,#15339,#8046,.T.);
#18482=EDGE_CURVE('',#15339,#15337,#8047,.T.);
#18483=EDGE_CURVE('',#14686,#15335,#8048,.T.);
#18484=EDGE_CURVE('',#15336,#14679,#8049,.T.);
#18485=EDGE_CURVE('',#15340,#15341,#8050,.T.);
#18486=EDGE_CURVE('',#15342,#15340,#8051,.T.);
#18487=EDGE_CURVE('',#15341,#15342,#8052,.T.);
#18488=EDGE_CURVE('',#15343,#15344,#8053,.T.);
#18489=EDGE_CURVE('',#15344,#15342,#8054,.T.);
#18490=EDGE_CURVE('',#15340,#15345,#8055,.T.);
#18491=EDGE_CURVE('',#15345,#15343,#8056,.T.);
#18492=EDGE_CURVE('',#15335,#15341,#8057,.T.);
#18493=EDGE_CURVE('',#15342,#15334,#8058,.T.);
#18494=EDGE_CURVE('',#14684,#15340,#8059,.T.);
#18495=EDGE_CURVE('',#15341,#14685,#8060,.T.);
#18496=EDGE_CURVE('',#15337,#15346,#8061,.T.);
#18497=EDGE_CURVE('',#15346,#14681,#8062,.T.);
#18498=EDGE_CURVE('',#14680,#15338,#8063,.T.);
#18499=EDGE_CURVE('',#15339,#15344,#8064,.T.);
#18500=EDGE_CURVE('',#15347,#15343,#8065,.T.);
#18501=EDGE_CURVE('',#15347,#15346,#8066,.T.);
#18502=EDGE_CURVE('',#15345,#14683,#8067,.T.);
#18503=EDGE_CURVE('',#14682,#15347,#8068,.T.);
#18504=EDGE_CURVE('',#15348,#15349,#8069,.T.);
#18505=EDGE_CURVE('',#15350,#15348,#8070,.T.);
#18506=EDGE_CURVE('',#15349,#15350,#8071,.T.);
#18507=EDGE_CURVE('',#15351,#15352,#8072,.T.);
#18508=EDGE_CURVE('',#15353,#15351,#8073,.T.);
#18509=EDGE_CURVE('',#15352,#15353,#8074,.T.);
#18510=EDGE_CURVE('',#15354,#15355,#8075,.T.);
#18511=EDGE_CURVE('',#15356,#15354,#8076,.T.);
#18512=EDGE_CURVE('',#15355,#15356,#8077,.T.);
#18513=EDGE_CURVE('',#14690,#15356,#8078,.T.);
#18514=EDGE_CURVE('',#15354,#14691,#8079,.T.);
#18515=EDGE_CURVE('',#15357,#15358,#8080,.T.);
#18516=EDGE_CURVE('',#15359,#15357,#8081,.T.);
#18517=EDGE_CURVE('',#15358,#15359,#8082,.T.);
#18518=EDGE_CURVE('',#14688,#15359,#8083,.T.);
#18519=EDGE_CURVE('',#15357,#14689,#8084,.T.);
#18520=EDGE_CURVE('',#15351,#15358,#8085,.T.);
#18521=EDGE_CURVE('',#15359,#15353,#8086,.T.);
#18522=EDGE_CURVE('',#15358,#15355,#8087,.T.);
#18523=EDGE_CURVE('',#15356,#15357,#8088,.T.);
#18524=EDGE_CURVE('',#15348,#15354,#8089,.T.);
#18525=EDGE_CURVE('',#15355,#15350,#8090,.T.);
#18526=EDGE_CURVE('',#14694,#15352,#8091,.T.);
#18527=EDGE_CURVE('',#15353,#14687,#8092,.T.);
#18528=EDGE_CURVE('',#15352,#15349,#8093,.T.);
#18529=EDGE_CURVE('',#15350,#15351,#8094,.T.);
#18530=EDGE_CURVE('',#14692,#15348,#8095,.T.);
#18531=EDGE_CURVE('',#15349,#14693,#8096,.T.);
#18532=EDGE_CURVE('',#15360,#15361,#8097,.T.);
#18533=EDGE_CURVE('',#15362,#15360,#8098,.T.);
#18534=EDGE_CURVE('',#15361,#15362,#8099,.T.);
#18535=EDGE_CURVE('',#15363,#15364,#8100,.T.);
#18536=EDGE_CURVE('',#15365,#15363,#8101,.T.);
#18537=EDGE_CURVE('',#15364,#15365,#8102,.T.);
#18538=EDGE_CURVE('',#15366,#15367,#8103,.T.);
#18539=EDGE_CURVE('',#15368,#15366,#8104,.T.);
#18540=EDGE_CURVE('',#15367,#15368,#8105,.T.);
#18541=EDGE_CURVE('',#14698,#15368,#8106,.T.);
#18542=EDGE_CURVE('',#15366,#14699,#8107,.T.);
#18543=EDGE_CURVE('',#15369,#15370,#8108,.T.);
#18544=EDGE_CURVE('',#15371,#15369,#8109,.T.);
#18545=EDGE_CURVE('',#15370,#15371,#8110,.T.);
#18546=EDGE_CURVE('',#14696,#15371,#8111,.T.);
#18547=EDGE_CURVE('',#15369,#14697,#8112,.T.);
#18548=EDGE_CURVE('',#15363,#15370,#8113,.T.);
#18549=EDGE_CURVE('',#15371,#15365,#8114,.T.);
#18550=EDGE_CURVE('',#15370,#15367,#8115,.T.);
#18551=EDGE_CURVE('',#15368,#15369,#8116,.T.);
#18552=EDGE_CURVE('',#15360,#15366,#8117,.T.);
#18553=EDGE_CURVE('',#15367,#15362,#8118,.T.);
#18554=EDGE_CURVE('',#14702,#15364,#8119,.T.);
#18555=EDGE_CURVE('',#15365,#14695,#8120,.T.);
#18556=EDGE_CURVE('',#15364,#15361,#8121,.T.);
#18557=EDGE_CURVE('',#15362,#15363,#8122,.T.);
#18558=EDGE_CURVE('',#14700,#15360,#8123,.T.);
#18559=EDGE_CURVE('',#15361,#14701,#8124,.T.);
#18560=EDGE_CURVE('',#15372,#15373,#8125,.T.);
#18561=EDGE_CURVE('',#15373,#14709,#8126,.T.);
#18562=EDGE_CURVE('',#14708,#15374,#8127,.T.);
#18563=EDGE_CURVE('',#15374,#15372,#8128,.T.);
#18564=EDGE_CURVE('',#15375,#15373,#8129,.T.);
#18565=EDGE_CURVE('',#14710,#15375,#8130,.T.);
#18566=EDGE_CURVE('',#15376,#15372,#8131,.T.);
#18567=EDGE_CURVE('',#15376,#15377,#8132,.T.);
#18568=EDGE_CURVE('',#15377,#15375,#8133,.T.);
#18569=EDGE_CURVE('',#15374,#15378,#8134,.T.);
#18570=EDGE_CURVE('',#15378,#15379,#8135,.T.);
#18571=EDGE_CURVE('',#15379,#15376,#8136,.T.);
#18572=EDGE_CURVE('',#15380,#15377,#8137,.T.);
#18573=EDGE_CURVE('',#15375,#15380,#8138,.T.);
#18574=EDGE_CURVE('',#15381,#15378,#8139,.T.);
#18575=EDGE_CURVE('',#15379,#15381,#8140,.T.);
#18576=EDGE_CURVE('',#14706,#15381,#8141,.T.);
#18577=EDGE_CURVE('',#15378,#14707,#8142,.T.);
#18578=EDGE_CURVE('',#15382,#15383,#8143,.T.);
#18579=EDGE_CURVE('',#15384,#15382,#8144,.T.);
#18580=EDGE_CURVE('',#15383,#15384,#8145,.T.);
#18581=EDGE_CURVE('',#14704,#15384,#8146,.T.);
#18582=EDGE_CURVE('',#15382,#14705,#8147,.T.);
#18583=EDGE_CURVE('',#15377,#15383,#8148,.T.);
#18584=EDGE_CURVE('',#15384,#15380,#8149,.T.);
#18585=EDGE_CURVE('',#15383,#15379,#8150,.T.);
#18586=EDGE_CURVE('',#15381,#15382,#8151,.T.);
#18587=EDGE_CURVE('',#15380,#14703,#8152,.T.);
#18588=EDGE_CURVE('',#15385,#15386,#8153,.T.);
#18589=EDGE_CURVE('',#15387,#15385,#8154,.T.);
#18590=EDGE_CURVE('',#15386,#15387,#8155,.T.);
#18591=EDGE_CURVE('',#15388,#15389,#8156,.T.);
#18592=EDGE_CURVE('',#15390,#15388,#8157,.T.);
#18593=EDGE_CURVE('',#15389,#15390,#8158,.T.);
#18594=EDGE_CURVE('',#15391,#15392,#8159,.T.);
#18595=EDGE_CURVE('',#15393,#15391,#8160,.T.);
#18596=EDGE_CURVE('',#15392,#15393,#8161,.T.);
#18597=EDGE_CURVE('',#14714,#15393,#8162,.T.);
#18598=EDGE_CURVE('',#15391,#14715,#8163,.T.);
#18599=EDGE_CURVE('',#15394,#15395,#8164,.T.);
#18600=EDGE_CURVE('',#15396,#15394,#8165,.T.);
#18601=EDGE_CURVE('',#15395,#15396,#8166,.T.);
#18602=EDGE_CURVE('',#14712,#15396,#8167,.T.);
#18603=EDGE_CURVE('',#15394,#14713,#8168,.T.);
#18604=EDGE_CURVE('',#15388,#15395,#8169,.T.);
#18605=EDGE_CURVE('',#15396,#15390,#8170,.T.);
#18606=EDGE_CURVE('',#15395,#15392,#8171,.T.);
#18607=EDGE_CURVE('',#15393,#15394,#8172,.T.);
#18608=EDGE_CURVE('',#15385,#15391,#8173,.T.);
#18609=EDGE_CURVE('',#15392,#15387,#8174,.T.);
#18610=EDGE_CURVE('',#14718,#15389,#8175,.T.);
#18611=EDGE_CURVE('',#15390,#14711,#8176,.T.);
#18612=EDGE_CURVE('',#15389,#15386,#8177,.T.);
#18613=EDGE_CURVE('',#15387,#15388,#8178,.T.);
#18614=EDGE_CURVE('',#14716,#15385,#8179,.T.);
#18615=EDGE_CURVE('',#15386,#14717,#8180,.T.);
#18616=EDGE_CURVE('',#15397,#15398,#8181,.T.);
#18617=EDGE_CURVE('',#15399,#15397,#8182,.T.);
#18618=EDGE_CURVE('',#15398,#15399,#8183,.T.);
#18619=EDGE_CURVE('',#15400,#15401,#8184,.T.);
#18620=EDGE_CURVE('',#15401,#15399,#8185,.T.);
#18621=EDGE_CURVE('',#15397,#15402,#8186,.T.);
#18622=EDGE_CURVE('',#15402,#15400,#8187,.T.);
#18623=EDGE_CURVE('',#14726,#15398,#8188,.T.);
#18624=EDGE_CURVE('',#15399,#14719,#8189,.T.);
#18625=EDGE_CURVE('',#15403,#15404,#8190,.T.);
#18626=EDGE_CURVE('',#15405,#15403,#8191,.T.);
#18627=EDGE_CURVE('',#15404,#15405,#8192,.T.);
#18628=EDGE_CURVE('',#15406,#15407,#8193,.T.);
#18629=EDGE_CURVE('',#15407,#15405,#8194,.T.);
#18630=EDGE_CURVE('',#15403,#15408,#8195,.T.);
#18631=EDGE_CURVE('',#15408,#15406,#8196,.T.);
#18632=EDGE_CURVE('',#15398,#15404,#8197,.T.);
#18633=EDGE_CURVE('',#15405,#15397,#8198,.T.);
#18634=EDGE_CURVE('',#14724,#15403,#8199,.T.);
#18635=EDGE_CURVE('',#15404,#14725,#8200,.T.);
#18636=EDGE_CURVE('',#15400,#15409,#8201,.T.);
#18637=EDGE_CURVE('',#15409,#14721,#8202,.T.);
#18638=EDGE_CURVE('',#14720,#15401,#8203,.T.);
#18639=EDGE_CURVE('',#15402,#15407,#8204,.T.);
#18640=EDGE_CURVE('',#15410,#15406,#8205,.T.);
#18641=EDGE_CURVE('',#15410,#15409,#8206,.T.);
#18642=EDGE_CURVE('',#15408,#14723,#8207,.T.);
#18643=EDGE_CURVE('',#14722,#15410,#8208,.T.);
#18644=EDGE_CURVE('',#15411,#15412,#8209,.T.);
#18645=EDGE_CURVE('',#15413,#15411,#8210,.T.);
#18646=EDGE_CURVE('',#15412,#15413,#8211,.T.);
#18647=EDGE_CURVE('',#15414,#15415,#8212,.T.);
#18648=EDGE_CURVE('',#15416,#15414,#8213,.T.);
#18649=EDGE_CURVE('',#15415,#15416,#8214,.T.);
#18650=EDGE_CURVE('',#15417,#15418,#8215,.T.);
#18651=EDGE_CURVE('',#15419,#15417,#8216,.T.);
#18652=EDGE_CURVE('',#15418,#15419,#8217,.T.);
#18653=EDGE_CURVE('',#14579,#15419,#8218,.T.);
#18654=EDGE_CURVE('',#15417,#14580,#8219,.T.);
#18655=EDGE_CURVE('',#15420,#15421,#8220,.T.);
#18656=EDGE_CURVE('',#15422,#15420,#8221,.T.);
#18657=EDGE_CURVE('',#15421,#15422,#8222,.T.);
#18658=EDGE_CURVE('',#14575,#15422,#8223,.T.);
#18659=EDGE_CURVE('',#15420,#14576,#8224,.T.);
#18660=EDGE_CURVE('',#15414,#15421,#8225,.T.);
#18661=EDGE_CURVE('',#15422,#15416,#8226,.T.);
#18662=EDGE_CURVE('',#15421,#15418,#8227,.T.);
#18663=EDGE_CURVE('',#15419,#15420,#8228,.T.);
#18664=EDGE_CURVE('',#15411,#15417,#8229,.T.);
#18665=EDGE_CURVE('',#15418,#15413,#8230,.T.);
#18666=EDGE_CURVE('',#14573,#15415,#8231,.T.);
#18667=EDGE_CURVE('',#15416,#14574,#8232,.T.);
#18668=EDGE_CURVE('',#15415,#15412,#8233,.T.);
#18669=EDGE_CURVE('',#15413,#15414,#8234,.T.);
#18670=EDGE_CURVE('',#14581,#15411,#8235,.T.);
#18671=EDGE_CURVE('',#15412,#14582,#8236,.T.);
#18672=EDGE_CURVE('',#15423,#15424,#8237,.T.);
#18673=EDGE_CURVE('',#15425,#15423,#8238,.T.);
#18674=EDGE_CURVE('',#15424,#15425,#8239,.T.);
#18675=EDGE_CURVE('',#15426,#15427,#8240,.T.);
#18676=EDGE_CURVE('',#15428,#15426,#8241,.T.);
#18677=EDGE_CURVE('',#15427,#15428,#8242,.T.);
#18678=EDGE_CURVE('',#15429,#15430,#8243,.T.);
#18679=EDGE_CURVE('',#15431,#15429,#8244,.T.);
#18680=EDGE_CURVE('',#15430,#15431,#8245,.T.);
#18681=EDGE_CURVE('',#14730,#15431,#8246,.T.);
#18682=EDGE_CURVE('',#15429,#14731,#8247,.T.);
#18683=EDGE_CURVE('',#15432,#15433,#8248,.T.);
#18684=EDGE_CURVE('',#15434,#15432,#8249,.T.);
#18685=EDGE_CURVE('',#15433,#15434,#8250,.T.);
#18686=EDGE_CURVE('',#14728,#15434,#8251,.T.);
#18687=EDGE_CURVE('',#15432,#14729,#8252,.T.);
#18688=EDGE_CURVE('',#15426,#15433,#8253,.T.);
#18689=EDGE_CURVE('',#15434,#15428,#8254,.T.);
#18690=EDGE_CURVE('',#15433,#15430,#8255,.T.);
#18691=EDGE_CURVE('',#15431,#15432,#8256,.T.);
#18692=EDGE_CURVE('',#15423,#15429,#8257,.T.);
#18693=EDGE_CURVE('',#15430,#15425,#8258,.T.);
#18694=EDGE_CURVE('',#14734,#15427,#8259,.T.);
#18695=EDGE_CURVE('',#15428,#14727,#8260,.T.);
#18696=EDGE_CURVE('',#15427,#15424,#8261,.T.);
#18697=EDGE_CURVE('',#15425,#15426,#8262,.T.);
#18698=EDGE_CURVE('',#14732,#15423,#8263,.T.);
#18699=EDGE_CURVE('',#15424,#14733,#8264,.T.);
#18700=EDGE_CURVE('',#15435,#15436,#8265,.T.);
#18701=EDGE_CURVE('',#15436,#14741,#8266,.T.);
#18702=EDGE_CURVE('',#14740,#15437,#8267,.T.);
#18703=EDGE_CURVE('',#15437,#15435,#8268,.T.);
#18704=EDGE_CURVE('',#15438,#15436,#8269,.T.);
#18705=EDGE_CURVE('',#14742,#15438,#8270,.T.);
#18706=EDGE_CURVE('',#15439,#15435,#8271,.T.);
#18707=EDGE_CURVE('',#15439,#15440,#8272,.T.);
#18708=EDGE_CURVE('',#15440,#15438,#8273,.T.);
#18709=EDGE_CURVE('',#15437,#15441,#8274,.T.);
#18710=EDGE_CURVE('',#15441,#15442,#8275,.T.);
#18711=EDGE_CURVE('',#15442,#15439,#8276,.T.);
#18712=EDGE_CURVE('',#15443,#15440,#8277,.T.);
#18713=EDGE_CURVE('',#15438,#15443,#8278,.T.);
#18714=EDGE_CURVE('',#15444,#15441,#8279,.T.);
#18715=EDGE_CURVE('',#15442,#15444,#8280,.T.);
#18716=EDGE_CURVE('',#14738,#15444,#8281,.T.);
#18717=EDGE_CURVE('',#15441,#14739,#8282,.T.);
#18718=EDGE_CURVE('',#15445,#15446,#8283,.T.);
#18719=EDGE_CURVE('',#15447,#15445,#8284,.T.);
#18720=EDGE_CURVE('',#15446,#15447,#8285,.T.);
#18721=EDGE_CURVE('',#14736,#15447,#8286,.T.);
#18722=EDGE_CURVE('',#15445,#14737,#8287,.T.);
#18723=EDGE_CURVE('',#15440,#15446,#8288,.T.);
#18724=EDGE_CURVE('',#15447,#15443,#8289,.T.);
#18725=EDGE_CURVE('',#15446,#15442,#8290,.T.);
#18726=EDGE_CURVE('',#15444,#15445,#8291,.T.);
#18727=EDGE_CURVE('',#15443,#14735,#8292,.T.);
#18728=EDGE_CURVE('',#15448,#15449,#8293,.T.);
#18729=EDGE_CURVE('',#15450,#15448,#8294,.T.);
#18730=EDGE_CURVE('',#15449,#15450,#8295,.T.);
#18731=EDGE_CURVE('',#15451,#15452,#8296,.T.);
#18732=EDGE_CURVE('',#15453,#15451,#8297,.T.);
#18733=EDGE_CURVE('',#15452,#15453,#8298,.T.);
#18734=EDGE_CURVE('',#15454,#15455,#8299,.T.);
#18735=EDGE_CURVE('',#15456,#15454,#8300,.T.);
#18736=EDGE_CURVE('',#15455,#15456,#8301,.T.);
#18737=EDGE_CURVE('',#14746,#15456,#8302,.T.);
#18738=EDGE_CURVE('',#15454,#14747,#8303,.T.);
#18739=EDGE_CURVE('',#15457,#15458,#8304,.T.);
#18740=EDGE_CURVE('',#15459,#15457,#8305,.T.);
#18741=EDGE_CURVE('',#15458,#15459,#8306,.T.);
#18742=EDGE_CURVE('',#14744,#15459,#8307,.T.);
#18743=EDGE_CURVE('',#15457,#14745,#8308,.T.);
#18744=EDGE_CURVE('',#15451,#15458,#8309,.T.);
#18745=EDGE_CURVE('',#15459,#15453,#8310,.T.);
#18746=EDGE_CURVE('',#15458,#15455,#8311,.T.);
#18747=EDGE_CURVE('',#15456,#15457,#8312,.T.);
#18748=EDGE_CURVE('',#15448,#15454,#8313,.T.);
#18749=EDGE_CURVE('',#15455,#15450,#8314,.T.);
#18750=EDGE_CURVE('',#14750,#15452,#8315,.T.);
#18751=EDGE_CURVE('',#15453,#14743,#8316,.T.);
#18752=EDGE_CURVE('',#15452,#15449,#8317,.T.);
#18753=EDGE_CURVE('',#15450,#15451,#8318,.T.);
#18754=EDGE_CURVE('',#14748,#15448,#8319,.T.);
#18755=EDGE_CURVE('',#15449,#14749,#8320,.T.);
#18756=EDGE_CURVE('',#15460,#15461,#8321,.T.);
#18757=EDGE_CURVE('',#15462,#15460,#8322,.T.);
#18758=EDGE_CURVE('',#15461,#15462,#8323,.T.);
#18759=EDGE_CURVE('',#15463,#15464,#8324,.T.);
#18760=EDGE_CURVE('',#15464,#15462,#8325,.T.);
#18761=EDGE_CURVE('',#15460,#15465,#8326,.T.);
#18762=EDGE_CURVE('',#15465,#15463,#8327,.T.);
#18763=EDGE_CURVE('',#14758,#15461,#8328,.T.);
#18764=EDGE_CURVE('',#15462,#14751,#8329,.T.);
#18765=EDGE_CURVE('',#15466,#15467,#8330,.T.);
#18766=EDGE_CURVE('',#15468,#15466,#8331,.T.);
#18767=EDGE_CURVE('',#15467,#15468,#8332,.T.);
#18768=EDGE_CURVE('',#15469,#15470,#8333,.T.);
#18769=EDGE_CURVE('',#15470,#15468,#8334,.T.);
#18770=EDGE_CURVE('',#15466,#15471,#8335,.T.);
#18771=EDGE_CURVE('',#15471,#15469,#8336,.T.);
#18772=EDGE_CURVE('',#15461,#15467,#8337,.T.);
#18773=EDGE_CURVE('',#15468,#15460,#8338,.T.);
#18774=EDGE_CURVE('',#14756,#15466,#8339,.T.);
#18775=EDGE_CURVE('',#15467,#14757,#8340,.T.);
#18776=EDGE_CURVE('',#15463,#15472,#8341,.T.);
#18777=EDGE_CURVE('',#15472,#14753,#8342,.T.);
#18778=EDGE_CURVE('',#14752,#15464,#8343,.T.);
#18779=EDGE_CURVE('',#15465,#15470,#8344,.T.);
#18780=EDGE_CURVE('',#15473,#15469,#8345,.T.);
#18781=EDGE_CURVE('',#15473,#15472,#8346,.T.);
#18782=EDGE_CURVE('',#15471,#14755,#8347,.T.);
#18783=EDGE_CURVE('',#14754,#15473,#8348,.T.);
#18784=EDGE_CURVE('',#15474,#15475,#8349,.T.);
#18785=EDGE_CURVE('',#15476,#15474,#8350,.T.);
#18786=EDGE_CURVE('',#15475,#15476,#8351,.T.);
#18787=EDGE_CURVE('',#15477,#15478,#8352,.T.);
#18788=EDGE_CURVE('',#15479,#15477,#8353,.T.);
#18789=EDGE_CURVE('',#15478,#15479,#8354,.T.);
#18790=EDGE_CURVE('',#15480,#15481,#8355,.T.);
#18791=EDGE_CURVE('',#15482,#15480,#8356,.T.);
#18792=EDGE_CURVE('',#15481,#15482,#8357,.T.);
#18793=EDGE_CURVE('',#14762,#15482,#8358,.T.);
#18794=EDGE_CURVE('',#15480,#14763,#8359,.T.);
#18795=EDGE_CURVE('',#15483,#15484,#8360,.T.);
#18796=EDGE_CURVE('',#15485,#15483,#8361,.T.);
#18797=EDGE_CURVE('',#15484,#15485,#8362,.T.);
#18798=EDGE_CURVE('',#14760,#15485,#8363,.T.);
#18799=EDGE_CURVE('',#15483,#14761,#8364,.T.);
#18800=EDGE_CURVE('',#15477,#15484,#8365,.T.);
#18801=EDGE_CURVE('',#15485,#15479,#8366,.T.);
#18802=EDGE_CURVE('',#15484,#15481,#8367,.T.);
#18803=EDGE_CURVE('',#15482,#15483,#8368,.T.);
#18804=EDGE_CURVE('',#15474,#15480,#8369,.T.);
#18805=EDGE_CURVE('',#15481,#15476,#8370,.T.);
#18806=EDGE_CURVE('',#14766,#15478,#8371,.T.);
#18807=EDGE_CURVE('',#15479,#14759,#8372,.T.);
#18808=EDGE_CURVE('',#15478,#15475,#8373,.T.);
#18809=EDGE_CURVE('',#15476,#15477,#8374,.T.);
#18810=EDGE_CURVE('',#14764,#15474,#8375,.T.);
#18811=EDGE_CURVE('',#15475,#14765,#8376,.T.);
#18812=EDGE_CURVE('',#15486,#15487,#8377,.T.);
#18813=EDGE_CURVE('',#15488,#15486,#8378,.T.);
#18814=EDGE_CURVE('',#15487,#15488,#8379,.T.);
#18815=EDGE_CURVE('',#15489,#15490,#8380,.T.);
#18816=EDGE_CURVE('',#15491,#15489,#8381,.T.);
#18817=EDGE_CURVE('',#15490,#15491,#8382,.T.);
#18818=EDGE_CURVE('',#15492,#15493,#8383,.T.);
#18819=EDGE_CURVE('',#15494,#15492,#8384,.T.);
#18820=EDGE_CURVE('',#15493,#15494,#8385,.T.);
#18821=EDGE_CURVE('',#14770,#15494,#8386,.T.);
#18822=EDGE_CURVE('',#15492,#14771,#8387,.T.);
#18823=EDGE_CURVE('',#15495,#15496,#8388,.T.);
#18824=EDGE_CURVE('',#15497,#15495,#8389,.T.);
#18825=EDGE_CURVE('',#15496,#15497,#8390,.T.);
#18826=EDGE_CURVE('',#14768,#15497,#8391,.T.);
#18827=EDGE_CURVE('',#15495,#14769,#8392,.T.);
#18828=EDGE_CURVE('',#15489,#15496,#8393,.T.);
#18829=EDGE_CURVE('',#15497,#15491,#8394,.T.);
#18830=EDGE_CURVE('',#15496,#15493,#8395,.T.);
#18831=EDGE_CURVE('',#15494,#15495,#8396,.T.);
#18832=EDGE_CURVE('',#15486,#15492,#8397,.T.);
#18833=EDGE_CURVE('',#15493,#15488,#8398,.T.);
#18834=EDGE_CURVE('',#14774,#15490,#8399,.T.);
#18835=EDGE_CURVE('',#15491,#14767,#8400,.T.);
#18836=EDGE_CURVE('',#15490,#15487,#8401,.T.);
#18837=EDGE_CURVE('',#15488,#15489,#8402,.T.);
#18838=EDGE_CURVE('',#14772,#15486,#8403,.T.);
#18839=EDGE_CURVE('',#15487,#14773,#8404,.T.);
#18840=EDGE_CURVE('',#15498,#15499,#8405,.T.);
#18841=EDGE_CURVE('',#15499,#14781,#8406,.T.);
#18842=EDGE_CURVE('',#14780,#15500,#8407,.T.);
#18843=EDGE_CURVE('',#15500,#15498,#8408,.T.);
#18844=EDGE_CURVE('',#15501,#15499,#8409,.T.);
#18845=EDGE_CURVE('',#14782,#15501,#8410,.T.);
#18846=EDGE_CURVE('',#15502,#15498,#8411,.T.);
#18847=EDGE_CURVE('',#15502,#15503,#8412,.T.);
#18848=EDGE_CURVE('',#15503,#15501,#8413,.T.);
#18849=EDGE_CURVE('',#15500,#15504,#8414,.T.);
#18850=EDGE_CURVE('',#15504,#15505,#8415,.T.);
#18851=EDGE_CURVE('',#15505,#15502,#8416,.T.);
#18852=EDGE_CURVE('',#15506,#15503,#8417,.T.);
#18853=EDGE_CURVE('',#15501,#15506,#8418,.T.);
#18854=EDGE_CURVE('',#15507,#15504,#8419,.T.);
#18855=EDGE_CURVE('',#15505,#15507,#8420,.T.);
#18856=EDGE_CURVE('',#14778,#15507,#8421,.T.);
#18857=EDGE_CURVE('',#15504,#14779,#8422,.T.);
#18858=EDGE_CURVE('',#15508,#15509,#8423,.T.);
#18859=EDGE_CURVE('',#15510,#15508,#8424,.T.);
#18860=EDGE_CURVE('',#15509,#15510,#8425,.T.);
#18861=EDGE_CURVE('',#14776,#15510,#8426,.T.);
#18862=EDGE_CURVE('',#15508,#14777,#8427,.T.);
#18863=EDGE_CURVE('',#15503,#15509,#8428,.T.);
#18864=EDGE_CURVE('',#15510,#15506,#8429,.T.);
#18865=EDGE_CURVE('',#15509,#15505,#8430,.T.);
#18866=EDGE_CURVE('',#15507,#15508,#8431,.T.);
#18867=EDGE_CURVE('',#15506,#14775,#8432,.T.);
#18868=EDGE_CURVE('',#15511,#15512,#8433,.T.);
#18869=EDGE_CURVE('',#15513,#15511,#8434,.T.);
#18870=EDGE_CURVE('',#15512,#15513,#8435,.T.);
#18871=EDGE_CURVE('',#15514,#15515,#8436,.T.);
#18872=EDGE_CURVE('',#15516,#15514,#8437,.T.);
#18873=EDGE_CURVE('',#15515,#15516,#8438,.T.);
#18874=EDGE_CURVE('',#15517,#15518,#8439,.T.);
#18875=EDGE_CURVE('',#15519,#15517,#8440,.T.);
#18876=EDGE_CURVE('',#15518,#15519,#8441,.T.);
#18877=EDGE_CURVE('',#14786,#15519,#8442,.T.);
#18878=EDGE_CURVE('',#15517,#14787,#8443,.T.);
#18879=EDGE_CURVE('',#15520,#15521,#8444,.T.);
#18880=EDGE_CURVE('',#15522,#15520,#8445,.T.);
#18881=EDGE_CURVE('',#15521,#15522,#8446,.T.);
#18882=EDGE_CURVE('',#14784,#15522,#8447,.T.);
#18883=EDGE_CURVE('',#15520,#14785,#8448,.T.);
#18884=EDGE_CURVE('',#15514,#15521,#8449,.T.);
#18885=EDGE_CURVE('',#15522,#15516,#8450,.T.);
#18886=EDGE_CURVE('',#15521,#15518,#8451,.T.);
#18887=EDGE_CURVE('',#15519,#15520,#8452,.T.);
#18888=EDGE_CURVE('',#15511,#15517,#8453,.T.);
#18889=EDGE_CURVE('',#15518,#15513,#8454,.T.);
#18890=EDGE_CURVE('',#14790,#15515,#8455,.T.);
#18891=EDGE_CURVE('',#15516,#14783,#8456,.T.);
#18892=EDGE_CURVE('',#15515,#15512,#8457,.T.);
#18893=EDGE_CURVE('',#15513,#15514,#8458,.T.);
#18894=EDGE_CURVE('',#14788,#15511,#8459,.T.);
#18895=EDGE_CURVE('',#15512,#14789,#8460,.T.);
#18896=EDGE_CURVE('',#15523,#15524,#8461,.T.);
#18897=EDGE_CURVE('',#15525,#15523,#8462,.T.);
#18898=EDGE_CURVE('',#15524,#15525,#8463,.T.);
#18899=EDGE_CURVE('',#15526,#15527,#8464,.T.);
#18900=EDGE_CURVE('',#15527,#15525,#8465,.T.);
#18901=EDGE_CURVE('',#15523,#15528,#8466,.T.);
#18902=EDGE_CURVE('',#15528,#15526,#8467,.T.);
#18903=EDGE_CURVE('',#14798,#15524,#8468,.T.);
#18904=EDGE_CURVE('',#15525,#14791,#8469,.T.);
#18905=EDGE_CURVE('',#15529,#15530,#8470,.T.);
#18906=EDGE_CURVE('',#15531,#15529,#8471,.T.);
#18907=EDGE_CURVE('',#15530,#15531,#8472,.T.);
#18908=EDGE_CURVE('',#15532,#15533,#8473,.T.);
#18909=EDGE_CURVE('',#15533,#15531,#8474,.T.);
#18910=EDGE_CURVE('',#15529,#15534,#8475,.T.);
#18911=EDGE_CURVE('',#15534,#15532,#8476,.T.);
#18912=EDGE_CURVE('',#15524,#15530,#8477,.T.);
#18913=EDGE_CURVE('',#15531,#15523,#8478,.T.);
#18914=EDGE_CURVE('',#14796,#15529,#8479,.T.);
#18915=EDGE_CURVE('',#15530,#14797,#8480,.T.);
#18916=EDGE_CURVE('',#15526,#15535,#8481,.T.);
#18917=EDGE_CURVE('',#15535,#14793,#8482,.T.);
#18918=EDGE_CURVE('',#14792,#15527,#8483,.T.);
#18919=EDGE_CURVE('',#15528,#15533,#8484,.T.);
#18920=EDGE_CURVE('',#15536,#15532,#8485,.T.);
#18921=EDGE_CURVE('',#15536,#15535,#8486,.T.);
#18922=EDGE_CURVE('',#15534,#14795,#8487,.T.);
#18923=EDGE_CURVE('',#14794,#15536,#8488,.T.);
#18924=EDGE_CURVE('',#15537,#15538,#8489,.T.);
#18925=EDGE_CURVE('',#15539,#15537,#8490,.T.);
#18926=EDGE_CURVE('',#15538,#15539,#8491,.T.);
#18927=EDGE_CURVE('',#15540,#15541,#8492,.T.);
#18928=EDGE_CURVE('',#15542,#15540,#8493,.T.);
#18929=EDGE_CURVE('',#15541,#15542,#8494,.T.);
#18930=EDGE_CURVE('',#15543,#15544,#8495,.T.);
#18931=EDGE_CURVE('',#15545,#15543,#8496,.T.);
#18932=EDGE_CURVE('',#15544,#15545,#8497,.T.);
#18933=EDGE_CURVE('',#14802,#15545,#8498,.T.);
#18934=EDGE_CURVE('',#15543,#14803,#8499,.T.);
#18935=EDGE_CURVE('',#15546,#15547,#8500,.T.);
#18936=EDGE_CURVE('',#15548,#15546,#8501,.T.);
#18937=EDGE_CURVE('',#15547,#15548,#8502,.T.);
#18938=EDGE_CURVE('',#14800,#15548,#8503,.T.);
#18939=EDGE_CURVE('',#15546,#14801,#8504,.T.);
#18940=EDGE_CURVE('',#15540,#15547,#8505,.T.);
#18941=EDGE_CURVE('',#15548,#15542,#8506,.T.);
#18942=EDGE_CURVE('',#15547,#15544,#8507,.T.);
#18943=EDGE_CURVE('',#15545,#15546,#8508,.T.);
#18944=EDGE_CURVE('',#15537,#15543,#8509,.T.);
#18945=EDGE_CURVE('',#15544,#15539,#8510,.T.);
#18946=EDGE_CURVE('',#14806,#15541,#8511,.T.);
#18947=EDGE_CURVE('',#15542,#14799,#8512,.T.);
#18948=EDGE_CURVE('',#15541,#15538,#8513,.T.);
#18949=EDGE_CURVE('',#15539,#15540,#8514,.T.);
#18950=EDGE_CURVE('',#14804,#15537,#8515,.T.);
#18951=EDGE_CURVE('',#15538,#14805,#8516,.T.);
#18952=EDGE_CURVE('',#15549,#15550,#8517,.T.);
#18953=EDGE_CURVE('',#15551,#15549,#8518,.T.);
#18954=EDGE_CURVE('',#15550,#15551,#8519,.T.);
#18955=EDGE_CURVE('',#15552,#15553,#8520,.T.);
#18956=EDGE_CURVE('',#15554,#15552,#8521,.T.);
#18957=EDGE_CURVE('',#15553,#15554,#8522,.T.);
#18958=EDGE_CURVE('',#15555,#15556,#8523,.T.);
#18959=EDGE_CURVE('',#15557,#15555,#8524,.T.);
#18960=EDGE_CURVE('',#15556,#15557,#8525,.T.);
#18961=EDGE_CURVE('',#14810,#15557,#8526,.T.);
#18962=EDGE_CURVE('',#15555,#14811,#8527,.T.);
#18963=EDGE_CURVE('',#15558,#15559,#8528,.T.);
#18964=EDGE_CURVE('',#15560,#15558,#8529,.T.);
#18965=EDGE_CURVE('',#15559,#15560,#8530,.T.);
#18966=EDGE_CURVE('',#14808,#15560,#8531,.T.);
#18967=EDGE_CURVE('',#15558,#14809,#8532,.T.);
#18968=EDGE_CURVE('',#15552,#15559,#8533,.T.);
#18969=EDGE_CURVE('',#15560,#15554,#8534,.T.);
#18970=EDGE_CURVE('',#15559,#15556,#8535,.T.);
#18971=EDGE_CURVE('',#15557,#15558,#8536,.T.);
#18972=EDGE_CURVE('',#15549,#15555,#8537,.T.);
#18973=EDGE_CURVE('',#15556,#15551,#8538,.T.);
#18974=EDGE_CURVE('',#14814,#15553,#8539,.T.);
#18975=EDGE_CURVE('',#15554,#14807,#8540,.T.);
#18976=EDGE_CURVE('',#15553,#15550,#8541,.T.);
#18977=EDGE_CURVE('',#15551,#15552,#8542,.T.);
#18978=EDGE_CURVE('',#14812,#15549,#8543,.T.);
#18979=EDGE_CURVE('',#15550,#14813,#8544,.T.);
#18980=EDGE_CURVE('',#15561,#15562,#8545,.T.);
#18981=EDGE_CURVE('',#15562,#14821,#8546,.T.);
#18982=EDGE_CURVE('',#14820,#15563,#8547,.T.);
#18983=EDGE_CURVE('',#15563,#15561,#8548,.T.);
#18984=EDGE_CURVE('',#15564,#15562,#8549,.T.);
#18985=EDGE_CURVE('',#14822,#15564,#8550,.T.);
#18986=EDGE_CURVE('',#15565,#15561,#8551,.T.);
#18987=EDGE_CURVE('',#15565,#15566,#8552,.T.);
#18988=EDGE_CURVE('',#15566,#15564,#8553,.T.);
#18989=EDGE_CURVE('',#15563,#15567,#8554,.T.);
#18990=EDGE_CURVE('',#15567,#15568,#8555,.T.);
#18991=EDGE_CURVE('',#15568,#15565,#8556,.T.);
#18992=EDGE_CURVE('',#15569,#15566,#8557,.T.);
#18993=EDGE_CURVE('',#15564,#15569,#8558,.T.);
#18994=EDGE_CURVE('',#15570,#15567,#8559,.T.);
#18995=EDGE_CURVE('',#15568,#15570,#8560,.T.);
#18996=EDGE_CURVE('',#14818,#15570,#8561,.T.);
#18997=EDGE_CURVE('',#15567,#14819,#8562,.T.);
#18998=EDGE_CURVE('',#15571,#15572,#8563,.T.);
#18999=EDGE_CURVE('',#15573,#15571,#8564,.T.);
#19000=EDGE_CURVE('',#15572,#15573,#8565,.T.);
#19001=EDGE_CURVE('',#14816,#15573,#8566,.T.);
#19002=EDGE_CURVE('',#15571,#14817,#8567,.T.);
#19003=EDGE_CURVE('',#15566,#15572,#8568,.T.);
#19004=EDGE_CURVE('',#15573,#15569,#8569,.T.);
#19005=EDGE_CURVE('',#15572,#15568,#8570,.T.);
#19006=EDGE_CURVE('',#15570,#15571,#8571,.T.);
#19007=EDGE_CURVE('',#15569,#14815,#8572,.T.);
#19008=EDGE_CURVE('',#15574,#15575,#8573,.T.);
#19009=EDGE_CURVE('',#15576,#15574,#8574,.T.);
#19010=EDGE_CURVE('',#15575,#15576,#8575,.T.);
#19011=EDGE_CURVE('',#15577,#15578,#8576,.T.);
#19012=EDGE_CURVE('',#15579,#15577,#8577,.T.);
#19013=EDGE_CURVE('',#15578,#15579,#8578,.T.);
#19014=EDGE_CURVE('',#15580,#15581,#8579,.T.);
#19015=EDGE_CURVE('',#15582,#15580,#8580,.T.);
#19016=EDGE_CURVE('',#15581,#15582,#8581,.T.);
#19017=EDGE_CURVE('',#14826,#15582,#8582,.T.);
#19018=EDGE_CURVE('',#15580,#14827,#8583,.T.);
#19019=EDGE_CURVE('',#15583,#15584,#8584,.T.);
#19020=EDGE_CURVE('',#15585,#15583,#8585,.T.);
#19021=EDGE_CURVE('',#15584,#15585,#8586,.T.);
#19022=EDGE_CURVE('',#14824,#15585,#8587,.T.);
#19023=EDGE_CURVE('',#15583,#14825,#8588,.T.);
#19024=EDGE_CURVE('',#15577,#15584,#8589,.T.);
#19025=EDGE_CURVE('',#15585,#15579,#8590,.T.);
#19026=EDGE_CURVE('',#15584,#15581,#8591,.T.);
#19027=EDGE_CURVE('',#15582,#15583,#8592,.T.);
#19028=EDGE_CURVE('',#15574,#15580,#8593,.T.);
#19029=EDGE_CURVE('',#15581,#15576,#8594,.T.);
#19030=EDGE_CURVE('',#14830,#15578,#8595,.T.);
#19031=EDGE_CURVE('',#15579,#14823,#8596,.T.);
#19032=EDGE_CURVE('',#15578,#15575,#8597,.T.);
#19033=EDGE_CURVE('',#15576,#15577,#8598,.T.);
#19034=EDGE_CURVE('',#14828,#15574,#8599,.T.);
#19035=EDGE_CURVE('',#15575,#14829,#8600,.T.);
#19036=EDGE_CURVE('',#15586,#15587,#8601,.T.);
#19037=EDGE_CURVE('',#15588,#15586,#8602,.T.);
#19038=EDGE_CURVE('',#15587,#15588,#8603,.T.);
#19039=EDGE_CURVE('',#15589,#15590,#8604,.T.);
#19040=EDGE_CURVE('',#15590,#15588,#8605,.T.);
#19041=EDGE_CURVE('',#15586,#15591,#8606,.T.);
#19042=EDGE_CURVE('',#15591,#15589,#8607,.T.);
#19043=EDGE_CURVE('',#14838,#15587,#8608,.T.);
#19044=EDGE_CURVE('',#15588,#14831,#8609,.T.);
#19045=EDGE_CURVE('',#15592,#15593,#8610,.T.);
#19046=EDGE_CURVE('',#15594,#15592,#8611,.T.);
#19047=EDGE_CURVE('',#15593,#15594,#8612,.T.);
#19048=EDGE_CURVE('',#15595,#15596,#8613,.T.);
#19049=EDGE_CURVE('',#15596,#15594,#8614,.T.);
#19050=EDGE_CURVE('',#15592,#15597,#8615,.T.);
#19051=EDGE_CURVE('',#15597,#15595,#8616,.T.);
#19052=EDGE_CURVE('',#15587,#15593,#8617,.T.);
#19053=EDGE_CURVE('',#15594,#15586,#8618,.T.);
#19054=EDGE_CURVE('',#14836,#15592,#8619,.T.);
#19055=EDGE_CURVE('',#15593,#14837,#8620,.T.);
#19056=EDGE_CURVE('',#15589,#15598,#8621,.T.);
#19057=EDGE_CURVE('',#15598,#14833,#8622,.T.);
#19058=EDGE_CURVE('',#14832,#15590,#8623,.T.);
#19059=EDGE_CURVE('',#15591,#15596,#8624,.T.);
#19060=EDGE_CURVE('',#15599,#15595,#8625,.T.);
#19061=EDGE_CURVE('',#15599,#15598,#8626,.T.);
#19062=EDGE_CURVE('',#15597,#14835,#8627,.T.);
#19063=EDGE_CURVE('',#14834,#15599,#8628,.T.);
#19064=EDGE_CURVE('',#15600,#15601,#8629,.T.);
#19065=EDGE_CURVE('',#15602,#15600,#8630,.T.);
#19066=EDGE_CURVE('',#15601,#15602,#8631,.T.);
#19067=EDGE_CURVE('',#15603,#15604,#8632,.T.);
#19068=EDGE_CURVE('',#15605,#15603,#8633,.T.);
#19069=EDGE_CURVE('',#15604,#15605,#8634,.T.);
#19070=EDGE_CURVE('',#15606,#15607,#8635,.T.);
#19071=EDGE_CURVE('',#15608,#15606,#8636,.T.);
#19072=EDGE_CURVE('',#15607,#15608,#8637,.T.);
#19073=EDGE_CURVE('',#14842,#15608,#8638,.T.);
#19074=EDGE_CURVE('',#15606,#14843,#8639,.T.);
#19075=EDGE_CURVE('',#15609,#15610,#8640,.T.);
#19076=EDGE_CURVE('',#15611,#15609,#8641,.T.);
#19077=EDGE_CURVE('',#15610,#15611,#8642,.T.);
#19078=EDGE_CURVE('',#14840,#15611,#8643,.T.);
#19079=EDGE_CURVE('',#15609,#14841,#8644,.T.);
#19080=EDGE_CURVE('',#15603,#15610,#8645,.T.);
#19081=EDGE_CURVE('',#15611,#15605,#8646,.T.);
#19082=EDGE_CURVE('',#15610,#15607,#8647,.T.);
#19083=EDGE_CURVE('',#15608,#15609,#8648,.T.);
#19084=EDGE_CURVE('',#15600,#15606,#8649,.T.);
#19085=EDGE_CURVE('',#15607,#15602,#8650,.T.);
#19086=EDGE_CURVE('',#14846,#15604,#8651,.T.);
#19087=EDGE_CURVE('',#15605,#14839,#8652,.T.);
#19088=EDGE_CURVE('',#15604,#15601,#8653,.T.);
#19089=EDGE_CURVE('',#15602,#15603,#8654,.T.);
#19090=EDGE_CURVE('',#14844,#15600,#8655,.T.);
#19091=EDGE_CURVE('',#15601,#14845,#8656,.T.);
#19092=EDGE_CURVE('',#15612,#15613,#8657,.T.);
#19093=EDGE_CURVE('',#15614,#15612,#8658,.T.);
#19094=EDGE_CURVE('',#15613,#15614,#8659,.T.);
#19095=EDGE_CURVE('',#15615,#15616,#8660,.T.);
#19096=EDGE_CURVE('',#15617,#15615,#8661,.T.);
#19097=EDGE_CURVE('',#15616,#15617,#8662,.T.);
#19098=EDGE_CURVE('',#15618,#15619,#8663,.T.);
#19099=EDGE_CURVE('',#15620,#15618,#8664,.T.);
#19100=EDGE_CURVE('',#15619,#15620,#8665,.T.);
#19101=EDGE_CURVE('',#14850,#15620,#8666,.T.);
#19102=EDGE_CURVE('',#15618,#14851,#8667,.T.);
#19103=EDGE_CURVE('',#15621,#15622,#8668,.T.);
#19104=EDGE_CURVE('',#15623,#15621,#8669,.T.);
#19105=EDGE_CURVE('',#15622,#15623,#8670,.T.);
#19106=EDGE_CURVE('',#14848,#15623,#8671,.T.);
#19107=EDGE_CURVE('',#15621,#14849,#8672,.T.);
#19108=EDGE_CURVE('',#15615,#15622,#8673,.T.);
#19109=EDGE_CURVE('',#15623,#15617,#8674,.T.);
#19110=EDGE_CURVE('',#15622,#15619,#8675,.T.);
#19111=EDGE_CURVE('',#15620,#15621,#8676,.T.);
#19112=EDGE_CURVE('',#15612,#15618,#8677,.T.);
#19113=EDGE_CURVE('',#15619,#15614,#8678,.T.);
#19114=EDGE_CURVE('',#14854,#15616,#8679,.T.);
#19115=EDGE_CURVE('',#15617,#14847,#8680,.T.);
#19116=EDGE_CURVE('',#15616,#15613,#8681,.T.);
#19117=EDGE_CURVE('',#15614,#15615,#8682,.T.);
#19118=EDGE_CURVE('',#14852,#15612,#8683,.T.);
#19119=EDGE_CURVE('',#15613,#14853,#8684,.T.);
#19120=EDGE_CURVE('',#15624,#15625,#8685,.T.);
#19121=EDGE_CURVE('',#15625,#14861,#8686,.T.);
#19122=EDGE_CURVE('',#14860,#15626,#8687,.T.);
#19123=EDGE_CURVE('',#15626,#15624,#8688,.T.);
#19124=EDGE_CURVE('',#15627,#15625,#8689,.T.);
#19125=EDGE_CURVE('',#14862,#15627,#8690,.T.);
#19126=EDGE_CURVE('',#15628,#15624,#8691,.T.);
#19127=EDGE_CURVE('',#15628,#15629,#8692,.T.);
#19128=EDGE_CURVE('',#15629,#15627,#8693,.T.);
#19129=EDGE_CURVE('',#15626,#15630,#8694,.T.);
#19130=EDGE_CURVE('',#15630,#15631,#8695,.T.);
#19131=EDGE_CURVE('',#15631,#15628,#8696,.T.);
#19132=EDGE_CURVE('',#15632,#15629,#8697,.T.);
#19133=EDGE_CURVE('',#15627,#15632,#8698,.T.);
#19134=EDGE_CURVE('',#15633,#15630,#8699,.T.);
#19135=EDGE_CURVE('',#15631,#15633,#8700,.T.);
#19136=EDGE_CURVE('',#14858,#15633,#8701,.T.);
#19137=EDGE_CURVE('',#15630,#14859,#8702,.T.);
#19138=EDGE_CURVE('',#15634,#15635,#8703,.T.);
#19139=EDGE_CURVE('',#15636,#15634,#8704,.T.);
#19140=EDGE_CURVE('',#15635,#15636,#8705,.T.);
#19141=EDGE_CURVE('',#14856,#15636,#8706,.T.);
#19142=EDGE_CURVE('',#15634,#14857,#8707,.T.);
#19143=EDGE_CURVE('',#15629,#15635,#8708,.T.);
#19144=EDGE_CURVE('',#15636,#15632,#8709,.T.);
#19145=EDGE_CURVE('',#15635,#15631,#8710,.T.);
#19146=EDGE_CURVE('',#15633,#15634,#8711,.T.);
#19147=EDGE_CURVE('',#15632,#14855,#8712,.T.);
#19148=EDGE_CURVE('',#15637,#15638,#8713,.T.);
#19149=EDGE_CURVE('',#15639,#15637,#8714,.T.);
#19150=EDGE_CURVE('',#15638,#15639,#8715,.T.);
#19151=EDGE_CURVE('',#15640,#15641,#8716,.T.);
#19152=EDGE_CURVE('',#15642,#15640,#8717,.T.);
#19153=EDGE_CURVE('',#15641,#15642,#8718,.T.);
#19154=EDGE_CURVE('',#15643,#15644,#8719,.T.);
#19155=EDGE_CURVE('',#15645,#15643,#8720,.T.);
#19156=EDGE_CURVE('',#15644,#15645,#8721,.T.);
#19157=EDGE_CURVE('',#14866,#15645,#8722,.T.);
#19158=EDGE_CURVE('',#15643,#14867,#8723,.T.);
#19159=EDGE_CURVE('',#15646,#15647,#8724,.T.);
#19160=EDGE_CURVE('',#15648,#15646,#8725,.T.);
#19161=EDGE_CURVE('',#15647,#15648,#8726,.T.);
#19162=EDGE_CURVE('',#14864,#15648,#8727,.T.);
#19163=EDGE_CURVE('',#15646,#14865,#8728,.T.);
#19164=EDGE_CURVE('',#15640,#15647,#8729,.T.);
#19165=EDGE_CURVE('',#15648,#15642,#8730,.T.);
#19166=EDGE_CURVE('',#15647,#15644,#8731,.T.);
#19167=EDGE_CURVE('',#15645,#15646,#8732,.T.);
#19168=EDGE_CURVE('',#15637,#15643,#8733,.T.);
#19169=EDGE_CURVE('',#15644,#15639,#8734,.T.);
#19170=EDGE_CURVE('',#14870,#15641,#8735,.T.);
#19171=EDGE_CURVE('',#15642,#14863,#8736,.T.);
#19172=EDGE_CURVE('',#15641,#15638,#8737,.T.);
#19173=EDGE_CURVE('',#15639,#15640,#8738,.T.);
#19174=EDGE_CURVE('',#14868,#15637,#8739,.T.);
#19175=EDGE_CURVE('',#15638,#14869,#8740,.T.);
#19176=EDGE_CURVE('',#15649,#15650,#8741,.T.);
#19177=EDGE_CURVE('',#15651,#15649,#8742,.T.);
#19178=EDGE_CURVE('',#15650,#15651,#8743,.T.);
#19179=EDGE_CURVE('',#15652,#15653,#8744,.T.);
#19180=EDGE_CURVE('',#15653,#15651,#8745,.T.);
#19181=EDGE_CURVE('',#15649,#15654,#8746,.T.);
#19182=EDGE_CURVE('',#15654,#15652,#8747,.T.);
#19183=EDGE_CURVE('',#14878,#15650,#8748,.T.);
#19184=EDGE_CURVE('',#15651,#14871,#8749,.T.);
#19185=EDGE_CURVE('',#15655,#15656,#8750,.T.);
#19186=EDGE_CURVE('',#15657,#15655,#8751,.T.);
#19187=EDGE_CURVE('',#15656,#15657,#8752,.T.);
#19188=EDGE_CURVE('',#15658,#15659,#8753,.T.);
#19189=EDGE_CURVE('',#15659,#15657,#8754,.T.);
#19190=EDGE_CURVE('',#15655,#15660,#8755,.T.);
#19191=EDGE_CURVE('',#15660,#15658,#8756,.T.);
#19192=EDGE_CURVE('',#15650,#15656,#8757,.T.);
#19193=EDGE_CURVE('',#15657,#15649,#8758,.T.);
#19194=EDGE_CURVE('',#14876,#15655,#8759,.T.);
#19195=EDGE_CURVE('',#15656,#14877,#8760,.T.);
#19196=EDGE_CURVE('',#15652,#15661,#8761,.T.);
#19197=EDGE_CURVE('',#15661,#14873,#8762,.T.);
#19198=EDGE_CURVE('',#14872,#15653,#8763,.T.);
#19199=EDGE_CURVE('',#15654,#15659,#8764,.T.);
#19200=EDGE_CURVE('',#15662,#15658,#8765,.T.);
#19201=EDGE_CURVE('',#15662,#15661,#8766,.T.);
#19202=EDGE_CURVE('',#15660,#14875,#8767,.T.);
#19203=EDGE_CURVE('',#14874,#15662,#8768,.T.);
#19204=EDGE_CURVE('',#15663,#15664,#8769,.T.);
#19205=EDGE_CURVE('',#15665,#15663,#8770,.T.);
#19206=EDGE_CURVE('',#15664,#15665,#8771,.T.);
#19207=EDGE_CURVE('',#15666,#15667,#8772,.T.);
#19208=EDGE_CURVE('',#15668,#15666,#8773,.T.);
#19209=EDGE_CURVE('',#15667,#15668,#8774,.T.);
#19210=EDGE_CURVE('',#15669,#15670,#8775,.T.);
#19211=EDGE_CURVE('',#15671,#15669,#8776,.T.);
#19212=EDGE_CURVE('',#15670,#15671,#8777,.T.);
#19213=EDGE_CURVE('',#14882,#15671,#8778,.T.);
#19214=EDGE_CURVE('',#15669,#14883,#8779,.T.);
#19215=EDGE_CURVE('',#15672,#15673,#8780,.T.);
#19216=EDGE_CURVE('',#15674,#15672,#8781,.T.);
#19217=EDGE_CURVE('',#15673,#15674,#8782,.T.);
#19218=EDGE_CURVE('',#14880,#15674,#8783,.T.);
#19219=EDGE_CURVE('',#15672,#14881,#8784,.T.);
#19220=EDGE_CURVE('',#15666,#15673,#8785,.T.);
#19221=EDGE_CURVE('',#15674,#15668,#8786,.T.);
#19222=EDGE_CURVE('',#15673,#15670,#8787,.T.);
#19223=EDGE_CURVE('',#15671,#15672,#8788,.T.);
#19224=EDGE_CURVE('',#15663,#15669,#8789,.T.);
#19225=EDGE_CURVE('',#15670,#15665,#8790,.T.);
#19226=EDGE_CURVE('',#14886,#15667,#8791,.T.);
#19227=EDGE_CURVE('',#15668,#14879,#8792,.T.);
#19228=EDGE_CURVE('',#15667,#15664,#8793,.T.);
#19229=EDGE_CURVE('',#15665,#15666,#8794,.T.);
#19230=EDGE_CURVE('',#14884,#15663,#8795,.T.);
#19231=EDGE_CURVE('',#15664,#14885,#8796,.T.);
#19232=EDGE_CURVE('',#15675,#15676,#8797,.T.);
#19233=EDGE_CURVE('',#15677,#15675,#8798,.T.);
#19234=EDGE_CURVE('',#15676,#15677,#8799,.T.);
#19235=EDGE_CURVE('',#15678,#15679,#8800,.T.);
#19236=EDGE_CURVE('',#15680,#15678,#8801,.T.);
#19237=EDGE_CURVE('',#15679,#15680,#8802,.T.);
#19238=EDGE_CURVE('',#15681,#15682,#8803,.T.);
#19239=EDGE_CURVE('',#15683,#15681,#8804,.T.);
#19240=EDGE_CURVE('',#15682,#15683,#8805,.T.);
#19241=EDGE_CURVE('',#14890,#15683,#8806,.T.);
#19242=EDGE_CURVE('',#15681,#14891,#8807,.T.);
#19243=EDGE_CURVE('',#15684,#15685,#8808,.T.);
#19244=EDGE_CURVE('',#15686,#15684,#8809,.T.);
#19245=EDGE_CURVE('',#15685,#15686,#8810,.T.);
#19246=EDGE_CURVE('',#14888,#15686,#8811,.T.);
#19247=EDGE_CURVE('',#15684,#14889,#8812,.T.);
#19248=EDGE_CURVE('',#15678,#15685,#8813,.T.);
#19249=EDGE_CURVE('',#15686,#15680,#8814,.T.);
#19250=EDGE_CURVE('',#15685,#15682,#8815,.T.);
#19251=EDGE_CURVE('',#15683,#15684,#8816,.T.);
#19252=EDGE_CURVE('',#15675,#15681,#8817,.T.);
#19253=EDGE_CURVE('',#15682,#15677,#8818,.T.);
#19254=EDGE_CURVE('',#14894,#15679,#8819,.T.);
#19255=EDGE_CURVE('',#15680,#14887,#8820,.T.);
#19256=EDGE_CURVE('',#15679,#15676,#8821,.T.);
#19257=EDGE_CURVE('',#15677,#15678,#8822,.T.);
#19258=EDGE_CURVE('',#14892,#15675,#8823,.T.);
#19259=EDGE_CURVE('',#15676,#14893,#8824,.T.);
#19260=EDGE_CURVE('',#15687,#15688,#8825,.T.);
#19261=EDGE_CURVE('',#15688,#14901,#8826,.T.);
#19262=EDGE_CURVE('',#14900,#15689,#8827,.T.);
#19263=EDGE_CURVE('',#15689,#15687,#8828,.T.);
#19264=EDGE_CURVE('',#15690,#15688,#8829,.T.);
#19265=EDGE_CURVE('',#14902,#15690,#8830,.T.);
#19266=EDGE_CURVE('',#15691,#15687,#8831,.T.);
#19267=EDGE_CURVE('',#15691,#15692,#8832,.T.);
#19268=EDGE_CURVE('',#15692,#15690,#8833,.T.);
#19269=EDGE_CURVE('',#15689,#15693,#8834,.T.);
#19270=EDGE_CURVE('',#15693,#15694,#8835,.T.);
#19271=EDGE_CURVE('',#15694,#15691,#8836,.T.);
#19272=EDGE_CURVE('',#15695,#15692,#8837,.T.);
#19273=EDGE_CURVE('',#15690,#15695,#8838,.T.);
#19274=EDGE_CURVE('',#15696,#15693,#8839,.T.);
#19275=EDGE_CURVE('',#15694,#15696,#8840,.T.);
#19276=EDGE_CURVE('',#14898,#15696,#8841,.T.);
#19277=EDGE_CURVE('',#15693,#14899,#8842,.T.);
#19278=EDGE_CURVE('',#15697,#15698,#8843,.T.);
#19279=EDGE_CURVE('',#15699,#15697,#8844,.T.);
#19280=EDGE_CURVE('',#15698,#15699,#8845,.T.);
#19281=EDGE_CURVE('',#14896,#15699,#8846,.T.);
#19282=EDGE_CURVE('',#15697,#14897,#8847,.T.);
#19283=EDGE_CURVE('',#15692,#15698,#8848,.T.);
#19284=EDGE_CURVE('',#15699,#15695,#8849,.T.);
#19285=EDGE_CURVE('',#15698,#15694,#8850,.T.);
#19286=EDGE_CURVE('',#15696,#15697,#8851,.T.);
#19287=EDGE_CURVE('',#15695,#14895,#8852,.T.);
#19288=EDGE_CURVE('',#15700,#15701,#8853,.T.);
#19289=EDGE_CURVE('',#15702,#15700,#8854,.T.);
#19290=EDGE_CURVE('',#15701,#15702,#8855,.T.);
#19291=EDGE_CURVE('',#15703,#15704,#8856,.T.);
#19292=EDGE_CURVE('',#15705,#15703,#8857,.T.);
#19293=EDGE_CURVE('',#15704,#15705,#8858,.T.);
#19294=EDGE_CURVE('',#15706,#15707,#8859,.T.);
#19295=EDGE_CURVE('',#15708,#15706,#8860,.T.);
#19296=EDGE_CURVE('',#15707,#15708,#8861,.T.);
#19297=EDGE_CURVE('',#14906,#15708,#8862,.T.);
#19298=EDGE_CURVE('',#15706,#14907,#8863,.T.);
#19299=EDGE_CURVE('',#15709,#15710,#8864,.T.);
#19300=EDGE_CURVE('',#15711,#15709,#8865,.T.);
#19301=EDGE_CURVE('',#15710,#15711,#8866,.T.);
#19302=EDGE_CURVE('',#14904,#15711,#8867,.T.);
#19303=EDGE_CURVE('',#15709,#14905,#8868,.T.);
#19304=EDGE_CURVE('',#15703,#15710,#8869,.T.);
#19305=EDGE_CURVE('',#15711,#15705,#8870,.T.);
#19306=EDGE_CURVE('',#15710,#15707,#8871,.T.);
#19307=EDGE_CURVE('',#15708,#15709,#8872,.T.);
#19308=EDGE_CURVE('',#15700,#15706,#8873,.T.);
#19309=EDGE_CURVE('',#15707,#15702,#8874,.T.);
#19310=EDGE_CURVE('',#14910,#15704,#8875,.T.);
#19311=EDGE_CURVE('',#15705,#14903,#8876,.T.);
#19312=EDGE_CURVE('',#15704,#15701,#8877,.T.);
#19313=EDGE_CURVE('',#15702,#15703,#8878,.T.);
#19314=EDGE_CURVE('',#14908,#15700,#8879,.T.);
#19315=EDGE_CURVE('',#15701,#14909,#8880,.T.);
#19316=EDGE_CURVE('',#15712,#15713,#8881,.T.);
#19317=EDGE_CURVE('',#15714,#15712,#8882,.T.);
#19318=EDGE_CURVE('',#15713,#15714,#8883,.T.);
#19319=EDGE_CURVE('',#15715,#15716,#8884,.T.);
#19320=EDGE_CURVE('',#15716,#15714,#8885,.T.);
#19321=EDGE_CURVE('',#15712,#15717,#8886,.T.);
#19322=EDGE_CURVE('',#15717,#15715,#8887,.T.);
#19323=EDGE_CURVE('',#14918,#15713,#8888,.T.);
#19324=EDGE_CURVE('',#15714,#14911,#8889,.T.);
#19325=EDGE_CURVE('',#15718,#15719,#8890,.T.);
#19326=EDGE_CURVE('',#15720,#15718,#8891,.T.);
#19327=EDGE_CURVE('',#15719,#15720,#8892,.T.);
#19328=EDGE_CURVE('',#15721,#15722,#8893,.T.);
#19329=EDGE_CURVE('',#15722,#15720,#8894,.T.);
#19330=EDGE_CURVE('',#15718,#15723,#8895,.T.);
#19331=EDGE_CURVE('',#15723,#15721,#8896,.T.);
#19332=EDGE_CURVE('',#15713,#15719,#8897,.T.);
#19333=EDGE_CURVE('',#15720,#15712,#8898,.T.);
#19334=EDGE_CURVE('',#14916,#15718,#8899,.T.);
#19335=EDGE_CURVE('',#15719,#14917,#8900,.T.);
#19336=EDGE_CURVE('',#15715,#15724,#8901,.T.);
#19337=EDGE_CURVE('',#15724,#14913,#8902,.T.);
#19338=EDGE_CURVE('',#14912,#15716,#8903,.T.);
#19339=EDGE_CURVE('',#15717,#15722,#8904,.T.);
#19340=EDGE_CURVE('',#15725,#15721,#8905,.T.);
#19341=EDGE_CURVE('',#15725,#15724,#8906,.T.);
#19342=EDGE_CURVE('',#15723,#14915,#8907,.T.);
#19343=EDGE_CURVE('',#14914,#15725,#8908,.T.);
#19344=EDGE_CURVE('',#15726,#15727,#8909,.T.);
#19345=EDGE_CURVE('',#15728,#15726,#8910,.T.);
#19346=EDGE_CURVE('',#15727,#15728,#8911,.T.);
#19347=EDGE_CURVE('',#15729,#15730,#8912,.T.);
#19348=EDGE_CURVE('',#15731,#15729,#8913,.T.);
#19349=EDGE_CURVE('',#15730,#15731,#8914,.T.);
#19350=EDGE_CURVE('',#15732,#15733,#8915,.T.);
#19351=EDGE_CURVE('',#15734,#15732,#8916,.T.);
#19352=EDGE_CURVE('',#15733,#15734,#8917,.T.);
#19353=EDGE_CURVE('',#14922,#15734,#8918,.T.);
#19354=EDGE_CURVE('',#15732,#14923,#8919,.T.);
#19355=EDGE_CURVE('',#15735,#15736,#8920,.T.);
#19356=EDGE_CURVE('',#15737,#15735,#8921,.T.);
#19357=EDGE_CURVE('',#15736,#15737,#8922,.T.);
#19358=EDGE_CURVE('',#14920,#15737,#8923,.T.);
#19359=EDGE_CURVE('',#15735,#14921,#8924,.T.);
#19360=EDGE_CURVE('',#15729,#15736,#8925,.T.);
#19361=EDGE_CURVE('',#15737,#15731,#8926,.T.);
#19362=EDGE_CURVE('',#15736,#15733,#8927,.T.);
#19363=EDGE_CURVE('',#15734,#15735,#8928,.T.);
#19364=EDGE_CURVE('',#15726,#15732,#8929,.T.);
#19365=EDGE_CURVE('',#15733,#15728,#8930,.T.);
#19366=EDGE_CURVE('',#14926,#15730,#8931,.T.);
#19367=EDGE_CURVE('',#15731,#14919,#8932,.T.);
#19368=EDGE_CURVE('',#15730,#15727,#8933,.T.);
#19369=EDGE_CURVE('',#15728,#15729,#8934,.T.);
#19370=EDGE_CURVE('',#14924,#15726,#8935,.T.);
#19371=EDGE_CURVE('',#15727,#14925,#8936,.T.);
#19372=EDGE_CURVE('',#15738,#15739,#8937,.T.);
#19373=EDGE_CURVE('',#15740,#15738,#8938,.T.);
#19374=EDGE_CURVE('',#15739,#15740,#8939,.T.);
#19375=EDGE_CURVE('',#15741,#15742,#8940,.T.);
#19376=EDGE_CURVE('',#15743,#15741,#8941,.T.);
#19377=EDGE_CURVE('',#15742,#15743,#8942,.T.);
#19378=EDGE_CURVE('',#15744,#15745,#8943,.T.);
#19379=EDGE_CURVE('',#15746,#15744,#8944,.T.);
#19380=EDGE_CURVE('',#15745,#15746,#8945,.T.);
#19381=EDGE_CURVE('',#14930,#15746,#8946,.T.);
#19382=EDGE_CURVE('',#15744,#14931,#8947,.T.);
#19383=EDGE_CURVE('',#15747,#15748,#8948,.T.);
#19384=EDGE_CURVE('',#15749,#15747,#8949,.T.);
#19385=EDGE_CURVE('',#15748,#15749,#8950,.T.);
#19386=EDGE_CURVE('',#14928,#15749,#8951,.T.);
#19387=EDGE_CURVE('',#15747,#14929,#8952,.T.);
#19388=EDGE_CURVE('',#15741,#15748,#8953,.T.);
#19389=EDGE_CURVE('',#15749,#15743,#8954,.T.);
#19390=EDGE_CURVE('',#15748,#15745,#8955,.T.);
#19391=EDGE_CURVE('',#15746,#15747,#8956,.T.);
#19392=EDGE_CURVE('',#15738,#15744,#8957,.T.);
#19393=EDGE_CURVE('',#15745,#15740,#8958,.T.);
#19394=EDGE_CURVE('',#14934,#15742,#8959,.T.);
#19395=EDGE_CURVE('',#15743,#14927,#8960,.T.);
#19396=EDGE_CURVE('',#15742,#15739,#8961,.T.);
#19397=EDGE_CURVE('',#15740,#15741,#8962,.T.);
#19398=EDGE_CURVE('',#14932,#15738,#8963,.T.);
#19399=EDGE_CURVE('',#15739,#14933,#8964,.T.);
#19400=EDGE_CURVE('',#15750,#15751,#8965,.T.);
#19401=EDGE_CURVE('',#15751,#14941,#8966,.T.);
#19402=EDGE_CURVE('',#14940,#15752,#8967,.T.);
#19403=EDGE_CURVE('',#15752,#15750,#8968,.T.);
#19404=EDGE_CURVE('',#15753,#15751,#8969,.T.);
#19405=EDGE_CURVE('',#14942,#15753,#8970,.T.);
#19406=EDGE_CURVE('',#15754,#15750,#8971,.T.);
#19407=EDGE_CURVE('',#15754,#15755,#8972,.T.);
#19408=EDGE_CURVE('',#15755,#15753,#8973,.T.);
#19409=EDGE_CURVE('',#15752,#15756,#8974,.T.);
#19410=EDGE_CURVE('',#15756,#15757,#8975,.T.);
#19411=EDGE_CURVE('',#15757,#15754,#8976,.T.);
#19412=EDGE_CURVE('',#15758,#15755,#8977,.T.);
#19413=EDGE_CURVE('',#15753,#15758,#8978,.T.);
#19414=EDGE_CURVE('',#15759,#15756,#8979,.T.);
#19415=EDGE_CURVE('',#15757,#15759,#8980,.T.);
#19416=EDGE_CURVE('',#14938,#15759,#8981,.T.);
#19417=EDGE_CURVE('',#15756,#14939,#8982,.T.);
#19418=EDGE_CURVE('',#15760,#15761,#8983,.T.);
#19419=EDGE_CURVE('',#15762,#15760,#8984,.T.);
#19420=EDGE_CURVE('',#15761,#15762,#8985,.T.);
#19421=EDGE_CURVE('',#14936,#15762,#8986,.T.);
#19422=EDGE_CURVE('',#15760,#14937,#8987,.T.);
#19423=EDGE_CURVE('',#15755,#15761,#8988,.T.);
#19424=EDGE_CURVE('',#15762,#15758,#8989,.T.);
#19425=EDGE_CURVE('',#15761,#15757,#8990,.T.);
#19426=EDGE_CURVE('',#15759,#15760,#8991,.T.);
#19427=EDGE_CURVE('',#15758,#14935,#8992,.T.);
#19428=EDGE_CURVE('',#15763,#15764,#8993,.T.);
#19429=EDGE_CURVE('',#15765,#15763,#8994,.T.);
#19430=EDGE_CURVE('',#15764,#15765,#8995,.T.);
#19431=EDGE_CURVE('',#15766,#15767,#8996,.T.);
#19432=EDGE_CURVE('',#15768,#15766,#8997,.T.);
#19433=EDGE_CURVE('',#15767,#15768,#8998,.T.);
#19434=EDGE_CURVE('',#15769,#15770,#8999,.T.);
#19435=EDGE_CURVE('',#15771,#15769,#9000,.T.);
#19436=EDGE_CURVE('',#15770,#15771,#9001,.T.);
#19437=EDGE_CURVE('',#14946,#15771,#9002,.T.);
#19438=EDGE_CURVE('',#15769,#14947,#9003,.T.);
#19439=EDGE_CURVE('',#15772,#15773,#9004,.T.);
#19440=EDGE_CURVE('',#15774,#15772,#9005,.T.);
#19441=EDGE_CURVE('',#15773,#15774,#9006,.T.);
#19442=EDGE_CURVE('',#14944,#15774,#9007,.T.);
#19443=EDGE_CURVE('',#15772,#14945,#9008,.T.);
#19444=EDGE_CURVE('',#15766,#15773,#9009,.T.);
#19445=EDGE_CURVE('',#15774,#15768,#9010,.T.);
#19446=EDGE_CURVE('',#15773,#15770,#9011,.T.);
#19447=EDGE_CURVE('',#15771,#15772,#9012,.T.);
#19448=EDGE_CURVE('',#15763,#15769,#9013,.T.);
#19449=EDGE_CURVE('',#15770,#15765,#9014,.T.);
#19450=EDGE_CURVE('',#14950,#15767,#9015,.T.);
#19451=EDGE_CURVE('',#15768,#14943,#9016,.T.);
#19452=EDGE_CURVE('',#15767,#15764,#9017,.T.);
#19453=EDGE_CURVE('',#15765,#15766,#9018,.T.);
#19454=EDGE_CURVE('',#14948,#15763,#9019,.T.);
#19455=EDGE_CURVE('',#15764,#14949,#9020,.T.);
#19456=EDGE_CURVE('',#15775,#15776,#9021,.T.);
#19457=EDGE_CURVE('',#15777,#15775,#9022,.T.);
#19458=EDGE_CURVE('',#15776,#15777,#9023,.T.);
#19459=EDGE_CURVE('',#15778,#15779,#9024,.T.);
#19460=EDGE_CURVE('',#15779,#15777,#9025,.T.);
#19461=EDGE_CURVE('',#15775,#15780,#9026,.T.);
#19462=EDGE_CURVE('',#15780,#15778,#9027,.T.);
#19463=EDGE_CURVE('',#14958,#15776,#9028,.T.);
#19464=EDGE_CURVE('',#15777,#14951,#9029,.T.);
#19465=EDGE_CURVE('',#15781,#15782,#9030,.T.);
#19466=EDGE_CURVE('',#15783,#15781,#9031,.T.);
#19467=EDGE_CURVE('',#15782,#15783,#9032,.T.);
#19468=EDGE_CURVE('',#15784,#15785,#9033,.T.);
#19469=EDGE_CURVE('',#15785,#15783,#9034,.T.);
#19470=EDGE_CURVE('',#15781,#15786,#9035,.T.);
#19471=EDGE_CURVE('',#15786,#15784,#9036,.T.);
#19472=EDGE_CURVE('',#15776,#15782,#9037,.T.);
#19473=EDGE_CURVE('',#15783,#15775,#9038,.T.);
#19474=EDGE_CURVE('',#14956,#15781,#9039,.T.);
#19475=EDGE_CURVE('',#15782,#14957,#9040,.T.);
#19476=EDGE_CURVE('',#15778,#15787,#9041,.T.);
#19477=EDGE_CURVE('',#15787,#14953,#9042,.T.);
#19478=EDGE_CURVE('',#14952,#15779,#9043,.T.);
#19479=EDGE_CURVE('',#15780,#15785,#9044,.T.);
#19480=EDGE_CURVE('',#15788,#15784,#9045,.T.);
#19481=EDGE_CURVE('',#15788,#15787,#9046,.T.);
#19482=EDGE_CURVE('',#15786,#14955,#9047,.T.);
#19483=EDGE_CURVE('',#14954,#15788,#9048,.T.);
#19484=EDGE_CURVE('',#15789,#15790,#9049,.T.);
#19485=EDGE_CURVE('',#15791,#15789,#9050,.T.);
#19486=EDGE_CURVE('',#15790,#15791,#9051,.T.);
#19487=EDGE_CURVE('',#15792,#15793,#9052,.T.);
#19488=EDGE_CURVE('',#15794,#15792,#9053,.T.);
#19489=EDGE_CURVE('',#15793,#15794,#9054,.T.);
#19490=EDGE_CURVE('',#15795,#15796,#9055,.T.);
#19491=EDGE_CURVE('',#15797,#15795,#9056,.T.);
#19492=EDGE_CURVE('',#15796,#15797,#9057,.T.);
#19493=EDGE_CURVE('',#14962,#15797,#9058,.T.);
#19494=EDGE_CURVE('',#15795,#14963,#9059,.T.);
#19495=EDGE_CURVE('',#15798,#15799,#9060,.T.);
#19496=EDGE_CURVE('',#15800,#15798,#9061,.T.);
#19497=EDGE_CURVE('',#15799,#15800,#9062,.T.);
#19498=EDGE_CURVE('',#14960,#15800,#9063,.T.);
#19499=EDGE_CURVE('',#15798,#14961,#9064,.T.);
#19500=EDGE_CURVE('',#15792,#15799,#9065,.T.);
#19501=EDGE_CURVE('',#15800,#15794,#9066,.T.);
#19502=EDGE_CURVE('',#15799,#15796,#9067,.T.);
#19503=EDGE_CURVE('',#15797,#15798,#9068,.T.);
#19504=EDGE_CURVE('',#15789,#15795,#9069,.T.);
#19505=EDGE_CURVE('',#15796,#15791,#9070,.T.);
#19506=EDGE_CURVE('',#14966,#15793,#9071,.T.);
#19507=EDGE_CURVE('',#15794,#14959,#9072,.T.);
#19508=EDGE_CURVE('',#15793,#15790,#9073,.T.);
#19509=EDGE_CURVE('',#15791,#15792,#9074,.T.);
#19510=EDGE_CURVE('',#14964,#15789,#9075,.T.);
#19511=EDGE_CURVE('',#15790,#14965,#9076,.T.);
#19512=EDGE_CURVE('',#15801,#15802,#9077,.T.);
#19513=EDGE_CURVE('',#15803,#15801,#9078,.T.);
#19514=EDGE_CURVE('',#15802,#15803,#9079,.T.);
#19515=EDGE_CURVE('',#15804,#15805,#9080,.T.);
#19516=EDGE_CURVE('',#15806,#15804,#9081,.T.);
#19517=EDGE_CURVE('',#15805,#15806,#9082,.T.);
#19518=EDGE_CURVE('',#15807,#15808,#9083,.T.);
#19519=EDGE_CURVE('',#15809,#15807,#9084,.T.);
#19520=EDGE_CURVE('',#15808,#15809,#9085,.T.);
#19521=EDGE_CURVE('',#14970,#15809,#9086,.T.);
#19522=EDGE_CURVE('',#15807,#14971,#9087,.T.);
#19523=EDGE_CURVE('',#15810,#15811,#9088,.T.);
#19524=EDGE_CURVE('',#15812,#15810,#9089,.T.);
#19525=EDGE_CURVE('',#15811,#15812,#9090,.T.);
#19526=EDGE_CURVE('',#14968,#15812,#9091,.T.);
#19527=EDGE_CURVE('',#15810,#14969,#9092,.T.);
#19528=EDGE_CURVE('',#15804,#15811,#9093,.T.);
#19529=EDGE_CURVE('',#15812,#15806,#9094,.T.);
#19530=EDGE_CURVE('',#15811,#15808,#9095,.T.);
#19531=EDGE_CURVE('',#15809,#15810,#9096,.T.);
#19532=EDGE_CURVE('',#15801,#15807,#9097,.T.);
#19533=EDGE_CURVE('',#15808,#15803,#9098,.T.);
#19534=EDGE_CURVE('',#14974,#15805,#9099,.T.);
#19535=EDGE_CURVE('',#15806,#14967,#9100,.T.);
#19536=EDGE_CURVE('',#15805,#15802,#9101,.T.);
#19537=EDGE_CURVE('',#15803,#15804,#9102,.T.);
#19538=EDGE_CURVE('',#14972,#15801,#9103,.T.);
#19539=EDGE_CURVE('',#15802,#14973,#9104,.T.);
#19540=EDGE_CURVE('',#15813,#15814,#9105,.T.);
#19541=EDGE_CURVE('',#15814,#14981,#9106,.T.);
#19542=EDGE_CURVE('',#14980,#15815,#9107,.T.);
#19543=EDGE_CURVE('',#15815,#15813,#9108,.T.);
#19544=EDGE_CURVE('',#15816,#15814,#9109,.T.);
#19545=EDGE_CURVE('',#14982,#15816,#9110,.T.);
#19546=EDGE_CURVE('',#15817,#15813,#9111,.T.);
#19547=EDGE_CURVE('',#15817,#15818,#9112,.T.);
#19548=EDGE_CURVE('',#15818,#15816,#9113,.T.);
#19549=EDGE_CURVE('',#15815,#15819,#9114,.T.);
#19550=EDGE_CURVE('',#15819,#15820,#9115,.T.);
#19551=EDGE_CURVE('',#15820,#15817,#9116,.T.);
#19552=EDGE_CURVE('',#15821,#15818,#9117,.T.);
#19553=EDGE_CURVE('',#15816,#15821,#9118,.T.);
#19554=EDGE_CURVE('',#15822,#15819,#9119,.T.);
#19555=EDGE_CURVE('',#15820,#15822,#9120,.T.);
#19556=EDGE_CURVE('',#14978,#15822,#9121,.T.);
#19557=EDGE_CURVE('',#15819,#14979,#9122,.T.);
#19558=EDGE_CURVE('',#15823,#15824,#9123,.T.);
#19559=EDGE_CURVE('',#15825,#15823,#9124,.T.);
#19560=EDGE_CURVE('',#15824,#15825,#9125,.T.);
#19561=EDGE_CURVE('',#14976,#15825,#9126,.T.);
#19562=EDGE_CURVE('',#15823,#14977,#9127,.T.);
#19563=EDGE_CURVE('',#15818,#15824,#9128,.T.);
#19564=EDGE_CURVE('',#15825,#15821,#9129,.T.);
#19565=EDGE_CURVE('',#15824,#15820,#9130,.T.);
#19566=EDGE_CURVE('',#15822,#15823,#9131,.T.);
#19567=EDGE_CURVE('',#15821,#14975,#9132,.T.);
#19568=EDGE_CURVE('',#15826,#15827,#9133,.T.);
#19569=EDGE_CURVE('',#15828,#15826,#9134,.T.);
#19570=EDGE_CURVE('',#15827,#15828,#9135,.T.);
#19571=EDGE_CURVE('',#15829,#15830,#9136,.T.);
#19572=EDGE_CURVE('',#15831,#15829,#9137,.T.);
#19573=EDGE_CURVE('',#15830,#15831,#9138,.T.);
#19574=EDGE_CURVE('',#15832,#15833,#9139,.T.);
#19575=EDGE_CURVE('',#15834,#15832,#9140,.T.);
#19576=EDGE_CURVE('',#15833,#15834,#9141,.T.);
#19577=EDGE_CURVE('',#14986,#15834,#9142,.T.);
#19578=EDGE_CURVE('',#15832,#14987,#9143,.T.);
#19579=EDGE_CURVE('',#15835,#15836,#9144,.T.);
#19580=EDGE_CURVE('',#15837,#15835,#9145,.T.);
#19581=EDGE_CURVE('',#15836,#15837,#9146,.T.);
#19582=EDGE_CURVE('',#14984,#15837,#9147,.T.);
#19583=EDGE_CURVE('',#15835,#14985,#9148,.T.);
#19584=EDGE_CURVE('',#15829,#15836,#9149,.T.);
#19585=EDGE_CURVE('',#15837,#15831,#9150,.T.);
#19586=EDGE_CURVE('',#15836,#15833,#9151,.T.);
#19587=EDGE_CURVE('',#15834,#15835,#9152,.T.);
#19588=EDGE_CURVE('',#15826,#15832,#9153,.T.);
#19589=EDGE_CURVE('',#15833,#15828,#9154,.T.);
#19590=EDGE_CURVE('',#14990,#15830,#9155,.T.);
#19591=EDGE_CURVE('',#15831,#14983,#9156,.T.);
#19592=EDGE_CURVE('',#15830,#15827,#9157,.T.);
#19593=EDGE_CURVE('',#15828,#15829,#9158,.T.);
#19594=EDGE_CURVE('',#14988,#15826,#9159,.T.);
#19595=EDGE_CURVE('',#15827,#14989,#9160,.T.);
#19596=EDGE_CURVE('',#15838,#15839,#9161,.T.);
#19597=EDGE_CURVE('',#15840,#15838,#9162,.T.);
#19598=EDGE_CURVE('',#15839,#15840,#9163,.T.);
#19599=EDGE_CURVE('',#15841,#15842,#9164,.T.);
#19600=EDGE_CURVE('',#15842,#15840,#9165,.T.);
#19601=EDGE_CURVE('',#15838,#15843,#9166,.T.);
#19602=EDGE_CURVE('',#15843,#15841,#9167,.T.);
#19603=EDGE_CURVE('',#14998,#15839,#9168,.T.);
#19604=EDGE_CURVE('',#15840,#14991,#9169,.T.);
#19605=EDGE_CURVE('',#15844,#15845,#9170,.T.);
#19606=EDGE_CURVE('',#15846,#15844,#9171,.T.);
#19607=EDGE_CURVE('',#15845,#15846,#9172,.T.);
#19608=EDGE_CURVE('',#15847,#15848,#9173,.T.);
#19609=EDGE_CURVE('',#15848,#15846,#9174,.T.);
#19610=EDGE_CURVE('',#15844,#15849,#9175,.T.);
#19611=EDGE_CURVE('',#15849,#15847,#9176,.T.);
#19612=EDGE_CURVE('',#15839,#15845,#9177,.T.);
#19613=EDGE_CURVE('',#15846,#15838,#9178,.T.);
#19614=EDGE_CURVE('',#14996,#15844,#9179,.T.);
#19615=EDGE_CURVE('',#15845,#14997,#9180,.T.);
#19616=EDGE_CURVE('',#15841,#15850,#9181,.T.);
#19617=EDGE_CURVE('',#15850,#14993,#9182,.T.);
#19618=EDGE_CURVE('',#14992,#15842,#9183,.T.);
#19619=EDGE_CURVE('',#15843,#15848,#9184,.T.);
#19620=EDGE_CURVE('',#15851,#15847,#9185,.T.);
#19621=EDGE_CURVE('',#15851,#15850,#9186,.T.);
#19622=EDGE_CURVE('',#15849,#14995,#9187,.T.);
#19623=EDGE_CURVE('',#14994,#15851,#9188,.T.);
#19624=EDGE_CURVE('',#15852,#15853,#9189,.T.);
#19625=EDGE_CURVE('',#15854,#15852,#9190,.T.);
#19626=EDGE_CURVE('',#15853,#15854,#9191,.T.);
#19627=EDGE_CURVE('',#15855,#15856,#9192,.T.);
#19628=EDGE_CURVE('',#15857,#15855,#9193,.T.);
#19629=EDGE_CURVE('',#15856,#15857,#9194,.T.);
#19630=EDGE_CURVE('',#15858,#15859,#9195,.T.);
#19631=EDGE_CURVE('',#15860,#15858,#9196,.T.);
#19632=EDGE_CURVE('',#15859,#15860,#9197,.T.);
#19633=EDGE_CURVE('',#15002,#15860,#9198,.T.);
#19634=EDGE_CURVE('',#15858,#15003,#9199,.T.);
#19635=EDGE_CURVE('',#15861,#15862,#9200,.T.);
#19636=EDGE_CURVE('',#15863,#15861,#9201,.T.);
#19637=EDGE_CURVE('',#15862,#15863,#9202,.T.);
#19638=EDGE_CURVE('',#15000,#15863,#9203,.T.);
#19639=EDGE_CURVE('',#15861,#15001,#9204,.T.);
#19640=EDGE_CURVE('',#15855,#15862,#9205,.T.);
#19641=EDGE_CURVE('',#15863,#15857,#9206,.T.);
#19642=EDGE_CURVE('',#15862,#15859,#9207,.T.);
#19643=EDGE_CURVE('',#15860,#15861,#9208,.T.);
#19644=EDGE_CURVE('',#15852,#15858,#9209,.T.);
#19645=EDGE_CURVE('',#15859,#15854,#9210,.T.);
#19646=EDGE_CURVE('',#15006,#15856,#9211,.T.);
#19647=EDGE_CURVE('',#15857,#14999,#9212,.T.);
#19648=EDGE_CURVE('',#15856,#15853,#9213,.T.);
#19649=EDGE_CURVE('',#15854,#15855,#9214,.T.);
#19650=EDGE_CURVE('',#15004,#15852,#9215,.T.);
#19651=EDGE_CURVE('',#15853,#15005,#9216,.T.);
#19652=EDGE_CURVE('',#15864,#15865,#9217,.T.);
#19653=EDGE_CURVE('',#15866,#15864,#9218,.T.);
#19654=EDGE_CURVE('',#15865,#15866,#9219,.T.);
#19655=EDGE_CURVE('',#15867,#15868,#9220,.T.);
#19656=EDGE_CURVE('',#15869,#15867,#9221,.T.);
#19657=EDGE_CURVE('',#15868,#15869,#9222,.T.);
#19658=EDGE_CURVE('',#15870,#15871,#9223,.T.);
#19659=EDGE_CURVE('',#15872,#15870,#9224,.T.);
#19660=EDGE_CURVE('',#15871,#15872,#9225,.T.);
#19661=EDGE_CURVE('',#15010,#15872,#9226,.T.);
#19662=EDGE_CURVE('',#15870,#15011,#9227,.T.);
#19663=EDGE_CURVE('',#15873,#15874,#9228,.T.);
#19664=EDGE_CURVE('',#15875,#15873,#9229,.T.);
#19665=EDGE_CURVE('',#15874,#15875,#9230,.T.);
#19666=EDGE_CURVE('',#15008,#15875,#9231,.T.);
#19667=EDGE_CURVE('',#15873,#15009,#9232,.T.);
#19668=EDGE_CURVE('',#15867,#15874,#9233,.T.);
#19669=EDGE_CURVE('',#15875,#15869,#9234,.T.);
#19670=EDGE_CURVE('',#15874,#15871,#9235,.T.);
#19671=EDGE_CURVE('',#15872,#15873,#9236,.T.);
#19672=EDGE_CURVE('',#15864,#15870,#9237,.T.);
#19673=EDGE_CURVE('',#15871,#15866,#9238,.T.);
#19674=EDGE_CURVE('',#15014,#15868,#9239,.T.);
#19675=EDGE_CURVE('',#15869,#15007,#9240,.T.);
#19676=EDGE_CURVE('',#15868,#15865,#9241,.T.);
#19677=EDGE_CURVE('',#15866,#15867,#9242,.T.);
#19678=EDGE_CURVE('',#15012,#15864,#9243,.T.);
#19679=EDGE_CURVE('',#15865,#15013,#9244,.T.);
#19680=EDGE_CURVE('',#15876,#15877,#9245,.T.);
#19681=EDGE_CURVE('',#15877,#15021,#9246,.T.);
#19682=EDGE_CURVE('',#15020,#15878,#9247,.T.);
#19683=EDGE_CURVE('',#15878,#15876,#9248,.T.);
#19684=EDGE_CURVE('',#15879,#15877,#9249,.T.);
#19685=EDGE_CURVE('',#15022,#15879,#9250,.T.);
#19686=EDGE_CURVE('',#15880,#15876,#9251,.T.);
#19687=EDGE_CURVE('',#15880,#15881,#9252,.T.);
#19688=EDGE_CURVE('',#15881,#15879,#9253,.T.);
#19689=EDGE_CURVE('',#15878,#15882,#9254,.T.);
#19690=EDGE_CURVE('',#15882,#15883,#9255,.T.);
#19691=EDGE_CURVE('',#15883,#15880,#9256,.T.);
#19692=EDGE_CURVE('',#15884,#15881,#9257,.T.);
#19693=EDGE_CURVE('',#15879,#15884,#9258,.T.);
#19694=EDGE_CURVE('',#15885,#15882,#9259,.T.);
#19695=EDGE_CURVE('',#15883,#15885,#9260,.T.);
#19696=EDGE_CURVE('',#15018,#15885,#9261,.T.);
#19697=EDGE_CURVE('',#15882,#15019,#9262,.T.);
#19698=EDGE_CURVE('',#15886,#15887,#9263,.T.);
#19699=EDGE_CURVE('',#15888,#15886,#9264,.T.);
#19700=EDGE_CURVE('',#15887,#15888,#9265,.T.);
#19701=EDGE_CURVE('',#15016,#15888,#9266,.T.);
#19702=EDGE_CURVE('',#15886,#15017,#9267,.T.);
#19703=EDGE_CURVE('',#15881,#15887,#9268,.T.);
#19704=EDGE_CURVE('',#15888,#15884,#9269,.T.);
#19705=EDGE_CURVE('',#15887,#15883,#9270,.T.);
#19706=EDGE_CURVE('',#15885,#15886,#9271,.T.);
#19707=EDGE_CURVE('',#15884,#15015,#9272,.T.);
#19708=EDGE_CURVE('',#15889,#15890,#9273,.T.);
#19709=EDGE_CURVE('',#15891,#15889,#9274,.T.);
#19710=EDGE_CURVE('',#15890,#15891,#9275,.T.);
#19711=EDGE_CURVE('',#15892,#15893,#9276,.T.);
#19712=EDGE_CURVE('',#15894,#15892,#9277,.T.);
#19713=EDGE_CURVE('',#15893,#15894,#9278,.T.);
#19714=EDGE_CURVE('',#15895,#15896,#9279,.T.);
#19715=EDGE_CURVE('',#15897,#15895,#9280,.T.);
#19716=EDGE_CURVE('',#15896,#15897,#9281,.T.);
#19717=EDGE_CURVE('',#15026,#15897,#9282,.T.);
#19718=EDGE_CURVE('',#15895,#15027,#9283,.T.);
#19719=EDGE_CURVE('',#15898,#15899,#9284,.T.);
#19720=EDGE_CURVE('',#15900,#15898,#9285,.T.);
#19721=EDGE_CURVE('',#15899,#15900,#9286,.T.);
#19722=EDGE_CURVE('',#15024,#15900,#9287,.T.);
#19723=EDGE_CURVE('',#15898,#15025,#9288,.T.);
#19724=EDGE_CURVE('',#15892,#15899,#9289,.T.);
#19725=EDGE_CURVE('',#15900,#15894,#9290,.T.);
#19726=EDGE_CURVE('',#15899,#15896,#9291,.T.);
#19727=EDGE_CURVE('',#15897,#15898,#9292,.T.);
#19728=EDGE_CURVE('',#15889,#15895,#9293,.T.);
#19729=EDGE_CURVE('',#15896,#15891,#9294,.T.);
#19730=EDGE_CURVE('',#15030,#15893,#9295,.T.);
#19731=EDGE_CURVE('',#15894,#15023,#9296,.T.);
#19732=EDGE_CURVE('',#15893,#15890,#9297,.T.);
#19733=EDGE_CURVE('',#15891,#15892,#9298,.T.);
#19734=EDGE_CURVE('',#15028,#15889,#9299,.T.);
#19735=EDGE_CURVE('',#15890,#15029,#9300,.T.);
#19736=EDGE_CURVE('',#15901,#15902,#9301,.T.);
#19737=EDGE_CURVE('',#15903,#15901,#9302,.T.);
#19738=EDGE_CURVE('',#15902,#15903,#9303,.T.);
#19739=EDGE_CURVE('',#15904,#15905,#9304,.T.);
#19740=EDGE_CURVE('',#15905,#15903,#9305,.T.);
#19741=EDGE_CURVE('',#15901,#15906,#9306,.T.);
#19742=EDGE_CURVE('',#15906,#15904,#9307,.T.);
#19743=EDGE_CURVE('',#15038,#15902,#9308,.T.);
#19744=EDGE_CURVE('',#15903,#15031,#9309,.T.);
#19745=EDGE_CURVE('',#15907,#15908,#9310,.T.);
#19746=EDGE_CURVE('',#15909,#15907,#9311,.T.);
#19747=EDGE_CURVE('',#15908,#15909,#9312,.T.);
#19748=EDGE_CURVE('',#15910,#15911,#9313,.T.);
#19749=EDGE_CURVE('',#15911,#15909,#9314,.T.);
#19750=EDGE_CURVE('',#15907,#15912,#9315,.T.);
#19751=EDGE_CURVE('',#15912,#15910,#9316,.T.);
#19752=EDGE_CURVE('',#15902,#15908,#9317,.T.);
#19753=EDGE_CURVE('',#15909,#15901,#9318,.T.);
#19754=EDGE_CURVE('',#15036,#15907,#9319,.T.);
#19755=EDGE_CURVE('',#15908,#15037,#9320,.T.);
#19756=EDGE_CURVE('',#15904,#15913,#9321,.T.);
#19757=EDGE_CURVE('',#15913,#15033,#9322,.T.);
#19758=EDGE_CURVE('',#15032,#15905,#9323,.T.);
#19759=EDGE_CURVE('',#15906,#15911,#9324,.T.);
#19760=EDGE_CURVE('',#15914,#15910,#9325,.T.);
#19761=EDGE_CURVE('',#15914,#15913,#9326,.T.);
#19762=EDGE_CURVE('',#15912,#15035,#9327,.T.);
#19763=EDGE_CURVE('',#15034,#15914,#9328,.T.);
#19764=EDGE_CURVE('',#15915,#15916,#9329,.T.);
#19765=EDGE_CURVE('',#15917,#15915,#9330,.T.);
#19766=EDGE_CURVE('',#15916,#15917,#9331,.T.);
#19767=EDGE_CURVE('',#15918,#15919,#9332,.T.);
#19768=EDGE_CURVE('',#15920,#15918,#9333,.T.);
#19769=EDGE_CURVE('',#15919,#15920,#9334,.T.);
#19770=EDGE_CURVE('',#15921,#15922,#9335,.T.);
#19771=EDGE_CURVE('',#15923,#15921,#9336,.T.);
#19772=EDGE_CURVE('',#15922,#15923,#9337,.T.);
#19773=EDGE_CURVE('',#15042,#15923,#9338,.T.);
#19774=EDGE_CURVE('',#15921,#15043,#9339,.T.);
#19775=EDGE_CURVE('',#15924,#15925,#9340,.T.);
#19776=EDGE_CURVE('',#15926,#15924,#9341,.T.);
#19777=EDGE_CURVE('',#15925,#15926,#9342,.T.);
#19778=EDGE_CURVE('',#15040,#15926,#9343,.T.);
#19779=EDGE_CURVE('',#15924,#15041,#9344,.T.);
#19780=EDGE_CURVE('',#15918,#15925,#9345,.T.);
#19781=EDGE_CURVE('',#15926,#15920,#9346,.T.);
#19782=EDGE_CURVE('',#15925,#15922,#9347,.T.);
#19783=EDGE_CURVE('',#15923,#15924,#9348,.T.);
#19784=EDGE_CURVE('',#15915,#15921,#9349,.T.);
#19785=EDGE_CURVE('',#15922,#15917,#9350,.T.);
#19786=EDGE_CURVE('',#15046,#15919,#9351,.T.);
#19787=EDGE_CURVE('',#15920,#15039,#9352,.T.);
#19788=EDGE_CURVE('',#15919,#15916,#9353,.T.);
#19789=EDGE_CURVE('',#15917,#15918,#9354,.T.);
#19790=EDGE_CURVE('',#15044,#15915,#9355,.T.);
#19791=EDGE_CURVE('',#15916,#15045,#9356,.T.);
#19792=EDGE_CURVE('',#15927,#15928,#9357,.T.);
#19793=EDGE_CURVE('',#15929,#15927,#9358,.T.);
#19794=EDGE_CURVE('',#15928,#15929,#9359,.T.);
#19795=EDGE_CURVE('',#15930,#15931,#9360,.T.);
#19796=EDGE_CURVE('',#15932,#15930,#9361,.T.);
#19797=EDGE_CURVE('',#15931,#15932,#9362,.T.);
#19798=EDGE_CURVE('',#15933,#15934,#9363,.T.);
#19799=EDGE_CURVE('',#15935,#15933,#9364,.T.);
#19800=EDGE_CURVE('',#15934,#15935,#9365,.T.);
#19801=EDGE_CURVE('',#15050,#15935,#9366,.T.);
#19802=EDGE_CURVE('',#15933,#15051,#9367,.T.);
#19803=EDGE_CURVE('',#15936,#15937,#9368,.T.);
#19804=EDGE_CURVE('',#15938,#15936,#9369,.T.);
#19805=EDGE_CURVE('',#15937,#15938,#9370,.T.);
#19806=EDGE_CURVE('',#15048,#15938,#9371,.T.);
#19807=EDGE_CURVE('',#15936,#15049,#9372,.T.);
#19808=EDGE_CURVE('',#15930,#15937,#9373,.T.);
#19809=EDGE_CURVE('',#15938,#15932,#9374,.T.);
#19810=EDGE_CURVE('',#15937,#15934,#9375,.T.);
#19811=EDGE_CURVE('',#15935,#15936,#9376,.T.);
#19812=EDGE_CURVE('',#15927,#15933,#9377,.T.);
#19813=EDGE_CURVE('',#15934,#15929,#9378,.T.);
#19814=EDGE_CURVE('',#15054,#15931,#9379,.T.);
#19815=EDGE_CURVE('',#15932,#15047,#9380,.T.);
#19816=EDGE_CURVE('',#15931,#15928,#9381,.T.);
#19817=EDGE_CURVE('',#15929,#15930,#9382,.T.);
#19818=EDGE_CURVE('',#15052,#15927,#9383,.T.);
#19819=EDGE_CURVE('',#15928,#15053,#9384,.T.);
#19820=EDGE_CURVE('',#15939,#15940,#9385,.T.);
#19821=EDGE_CURVE('',#15940,#15061,#9386,.T.);
#19822=EDGE_CURVE('',#15060,#15941,#9387,.T.);
#19823=EDGE_CURVE('',#15941,#15939,#9388,.T.);
#19824=EDGE_CURVE('',#15942,#15940,#9389,.T.);
#19825=EDGE_CURVE('',#15062,#15942,#9390,.T.);
#19826=EDGE_CURVE('',#15943,#15939,#9391,.T.);
#19827=EDGE_CURVE('',#15943,#15944,#9392,.T.);
#19828=EDGE_CURVE('',#15944,#15942,#9393,.T.);
#19829=EDGE_CURVE('',#15941,#15945,#9394,.T.);
#19830=EDGE_CURVE('',#15945,#15946,#9395,.T.);
#19831=EDGE_CURVE('',#15946,#15943,#9396,.T.);
#19832=EDGE_CURVE('',#15947,#15944,#9397,.T.);
#19833=EDGE_CURVE('',#15942,#15947,#9398,.T.);
#19834=EDGE_CURVE('',#15948,#15945,#9399,.T.);
#19835=EDGE_CURVE('',#15946,#15948,#9400,.T.);
#19836=EDGE_CURVE('',#15058,#15948,#9401,.T.);
#19837=EDGE_CURVE('',#15945,#15059,#9402,.T.);
#19838=EDGE_CURVE('',#15949,#15950,#9403,.T.);
#19839=EDGE_CURVE('',#15951,#15949,#9404,.T.);
#19840=EDGE_CURVE('',#15950,#15951,#9405,.T.);
#19841=EDGE_CURVE('',#15056,#15951,#9406,.T.);
#19842=EDGE_CURVE('',#15949,#15057,#9407,.T.);
#19843=EDGE_CURVE('',#15944,#15950,#9408,.T.);
#19844=EDGE_CURVE('',#15951,#15947,#9409,.T.);
#19845=EDGE_CURVE('',#15950,#15946,#9410,.T.);
#19846=EDGE_CURVE('',#15948,#15949,#9411,.T.);
#19847=EDGE_CURVE('',#15947,#15055,#9412,.T.);
#19848=EDGE_CURVE('',#15952,#15953,#9413,.T.);
#19849=EDGE_CURVE('',#15954,#15952,#9414,.T.);
#19850=EDGE_CURVE('',#15953,#15954,#9415,.T.);
#19851=EDGE_CURVE('',#15955,#15956,#9416,.T.);
#19852=EDGE_CURVE('',#15957,#15955,#9417,.T.);
#19853=EDGE_CURVE('',#15956,#15957,#9418,.T.);
#19854=EDGE_CURVE('',#15958,#15959,#9419,.T.);
#19855=EDGE_CURVE('',#15960,#15958,#9420,.T.);
#19856=EDGE_CURVE('',#15959,#15960,#9421,.T.);
#19857=EDGE_CURVE('',#15066,#15960,#9422,.T.);
#19858=EDGE_CURVE('',#15958,#15067,#9423,.T.);
#19859=EDGE_CURVE('',#15961,#15962,#9424,.T.);
#19860=EDGE_CURVE('',#15963,#15961,#9425,.T.);
#19861=EDGE_CURVE('',#15962,#15963,#9426,.T.);
#19862=EDGE_CURVE('',#15064,#15963,#9427,.T.);
#19863=EDGE_CURVE('',#15961,#15065,#9428,.T.);
#19864=EDGE_CURVE('',#15955,#15962,#9429,.T.);
#19865=EDGE_CURVE('',#15963,#15957,#9430,.T.);
#19866=EDGE_CURVE('',#15962,#15959,#9431,.T.);
#19867=EDGE_CURVE('',#15960,#15961,#9432,.T.);
#19868=EDGE_CURVE('',#15952,#15958,#9433,.T.);
#19869=EDGE_CURVE('',#15959,#15954,#9434,.T.);
#19870=EDGE_CURVE('',#15070,#15956,#9435,.T.);
#19871=EDGE_CURVE('',#15957,#15063,#9436,.T.);
#19872=EDGE_CURVE('',#15956,#15953,#9437,.T.);
#19873=EDGE_CURVE('',#15954,#15955,#9438,.T.);
#19874=EDGE_CURVE('',#15068,#15952,#9439,.T.);
#19875=EDGE_CURVE('',#15953,#15069,#9440,.T.);
#19876=EDGE_CURVE('',#15964,#15965,#9441,.T.);
#19877=EDGE_CURVE('',#15966,#15964,#9442,.T.);
#19878=EDGE_CURVE('',#15965,#15966,#9443,.T.);
#19879=EDGE_CURVE('',#15967,#15968,#9444,.T.);
#19880=EDGE_CURVE('',#15968,#15966,#9445,.T.);
#19881=EDGE_CURVE('',#15964,#15969,#9446,.T.);
#19882=EDGE_CURVE('',#15969,#15967,#9447,.T.);
#19883=EDGE_CURVE('',#15078,#15965,#9448,.T.);
#19884=EDGE_CURVE('',#15966,#15071,#9449,.T.);
#19885=EDGE_CURVE('',#15970,#15971,#9450,.T.);
#19886=EDGE_CURVE('',#15972,#15970,#9451,.T.);
#19887=EDGE_CURVE('',#15971,#15972,#9452,.T.);
#19888=EDGE_CURVE('',#15973,#15974,#9453,.T.);
#19889=EDGE_CURVE('',#15974,#15972,#9454,.T.);
#19890=EDGE_CURVE('',#15970,#15975,#9455,.T.);
#19891=EDGE_CURVE('',#15975,#15973,#9456,.T.);
#19892=EDGE_CURVE('',#15965,#15971,#9457,.T.);
#19893=EDGE_CURVE('',#15972,#15964,#9458,.T.);
#19894=EDGE_CURVE('',#15076,#15970,#9459,.T.);
#19895=EDGE_CURVE('',#15971,#15077,#9460,.T.);
#19896=EDGE_CURVE('',#15967,#15976,#9461,.T.);
#19897=EDGE_CURVE('',#15976,#15073,#9462,.T.);
#19898=EDGE_CURVE('',#15072,#15968,#9463,.T.);
#19899=EDGE_CURVE('',#15969,#15974,#9464,.T.);
#19900=EDGE_CURVE('',#15977,#15973,#9465,.T.);
#19901=EDGE_CURVE('',#15977,#15976,#9466,.T.);
#19902=EDGE_CURVE('',#15975,#15075,#9467,.T.);
#19903=EDGE_CURVE('',#15074,#15977,#9468,.T.);
#19904=EDGE_CURVE('',#15978,#15979,#9469,.T.);
#19905=EDGE_CURVE('',#15980,#15978,#9470,.T.);
#19906=EDGE_CURVE('',#15979,#15980,#9471,.T.);
#19907=EDGE_CURVE('',#15981,#15982,#9472,.T.);
#19908=EDGE_CURVE('',#15983,#15981,#9473,.T.);
#19909=EDGE_CURVE('',#15982,#15983,#9474,.T.);
#19910=EDGE_CURVE('',#15984,#15985,#9475,.T.);
#19911=EDGE_CURVE('',#15986,#15984,#9476,.T.);
#19912=EDGE_CURVE('',#15985,#15986,#9477,.T.);
#19913=EDGE_CURVE('',#15082,#15986,#9478,.T.);
#19914=EDGE_CURVE('',#15984,#15083,#9479,.T.);
#19915=EDGE_CURVE('',#15987,#15988,#9480,.T.);
#19916=EDGE_CURVE('',#15989,#15987,#9481,.T.);
#19917=EDGE_CURVE('',#15988,#15989,#9482,.T.);
#19918=EDGE_CURVE('',#15080,#15989,#9483,.T.);
#19919=EDGE_CURVE('',#15987,#15081,#9484,.T.);
#19920=EDGE_CURVE('',#15981,#15988,#9485,.T.);
#19921=EDGE_CURVE('',#15989,#15983,#9486,.T.);
#19922=EDGE_CURVE('',#15988,#15985,#9487,.T.);
#19923=EDGE_CURVE('',#15986,#15987,#9488,.T.);
#19924=EDGE_CURVE('',#15978,#15984,#9489,.T.);
#19925=EDGE_CURVE('',#15985,#15980,#9490,.T.);
#19926=EDGE_CURVE('',#15086,#15982,#9491,.T.);
#19927=EDGE_CURVE('',#15983,#15079,#9492,.T.);
#19928=EDGE_CURVE('',#15982,#15979,#9493,.T.);
#19929=EDGE_CURVE('',#15980,#15981,#9494,.T.);
#19930=EDGE_CURVE('',#15084,#15978,#9495,.T.);
#19931=EDGE_CURVE('',#15979,#15085,#9496,.T.);
#19932=EDGE_CURVE('',#15990,#15991,#9497,.T.);
#19933=EDGE_CURVE('',#15992,#15990,#9498,.T.);
#19934=EDGE_CURVE('',#15991,#15992,#9499,.T.);
#19935=EDGE_CURVE('',#15993,#15994,#9500,.T.);
#19936=EDGE_CURVE('',#15995,#15993,#9501,.T.);
#19937=EDGE_CURVE('',#15994,#15995,#9502,.T.);
#19938=EDGE_CURVE('',#15996,#15997,#9503,.T.);
#19939=EDGE_CURVE('',#15998,#15996,#9504,.T.);
#19940=EDGE_CURVE('',#15997,#15998,#9505,.T.);
#19941=EDGE_CURVE('',#15090,#15998,#9506,.T.);
#19942=EDGE_CURVE('',#15996,#15091,#9507,.T.);
#19943=EDGE_CURVE('',#15999,#16000,#9508,.T.);
#19944=EDGE_CURVE('',#16001,#15999,#9509,.T.);
#19945=EDGE_CURVE('',#16000,#16001,#9510,.T.);
#19946=EDGE_CURVE('',#15088,#16001,#9511,.T.);
#19947=EDGE_CURVE('',#15999,#15089,#9512,.T.);
#19948=EDGE_CURVE('',#15993,#16000,#9513,.T.);
#19949=EDGE_CURVE('',#16001,#15995,#9514,.T.);
#19950=EDGE_CURVE('',#16000,#15997,#9515,.T.);
#19951=EDGE_CURVE('',#15998,#15999,#9516,.T.);
#19952=EDGE_CURVE('',#15990,#15996,#9517,.T.);
#19953=EDGE_CURVE('',#15997,#15992,#9518,.T.);
#19954=EDGE_CURVE('',#15094,#15994,#9519,.T.);
#19955=EDGE_CURVE('',#15995,#15087,#9520,.T.);
#19956=EDGE_CURVE('',#15994,#15991,#9521,.T.);
#19957=EDGE_CURVE('',#15992,#15993,#9522,.T.);
#19958=EDGE_CURVE('',#15092,#15990,#9523,.T.);
#19959=EDGE_CURVE('',#15991,#15093,#9524,.T.);
#19960=EDGE_CURVE('',#16002,#16003,#9525,.T.);
#19961=EDGE_CURVE('',#16003,#15101,#9526,.T.);
#19962=EDGE_CURVE('',#15100,#16004,#9527,.T.);
#19963=EDGE_CURVE('',#16004,#16002,#9528,.T.);
#19964=EDGE_CURVE('',#16005,#16003,#9529,.T.);
#19965=EDGE_CURVE('',#15102,#16005,#9530,.T.);
#19966=EDGE_CURVE('',#16006,#16002,#9531,.T.);
#19967=EDGE_CURVE('',#16006,#16007,#9532,.T.);
#19968=EDGE_CURVE('',#16007,#16005,#9533,.T.);
#19969=EDGE_CURVE('',#16004,#16008,#9534,.T.);
#19970=EDGE_CURVE('',#16008,#16009,#9535,.T.);
#19971=EDGE_CURVE('',#16009,#16006,#9536,.T.);
#19972=EDGE_CURVE('',#16010,#16007,#9537,.T.);
#19973=EDGE_CURVE('',#16005,#16010,#9538,.T.);
#19974=EDGE_CURVE('',#16011,#16008,#9539,.T.);
#19975=EDGE_CURVE('',#16009,#16011,#9540,.T.);
#19976=EDGE_CURVE('',#15098,#16011,#9541,.T.);
#19977=EDGE_CURVE('',#16008,#15099,#9542,.T.);
#19978=EDGE_CURVE('',#16012,#16013,#9543,.T.);
#19979=EDGE_CURVE('',#16014,#16012,#9544,.T.);
#19980=EDGE_CURVE('',#16013,#16014,#9545,.T.);
#19981=EDGE_CURVE('',#15096,#16014,#9546,.T.);
#19982=EDGE_CURVE('',#16012,#15097,#9547,.T.);
#19983=EDGE_CURVE('',#16007,#16013,#9548,.T.);
#19984=EDGE_CURVE('',#16014,#16010,#9549,.T.);
#19985=EDGE_CURVE('',#16013,#16009,#9550,.T.);
#19986=EDGE_CURVE('',#16011,#16012,#9551,.T.);
#19987=EDGE_CURVE('',#16010,#15095,#9552,.T.);
#19988=EDGE_CURVE('',#16015,#16016,#9553,.T.);
#19989=EDGE_CURVE('',#16017,#16015,#9554,.T.);
#19990=EDGE_CURVE('',#16016,#16017,#9555,.T.);
#19991=EDGE_CURVE('',#16018,#16019,#9556,.T.);
#19992=EDGE_CURVE('',#16020,#16018,#9557,.T.);
#19993=EDGE_CURVE('',#16019,#16020,#9558,.T.);
#19994=EDGE_CURVE('',#16021,#16022,#9559,.T.);
#19995=EDGE_CURVE('',#16023,#16021,#9560,.T.);
#19996=EDGE_CURVE('',#16022,#16023,#9561,.T.);
#19997=EDGE_CURVE('',#15106,#16023,#9562,.T.);
#19998=EDGE_CURVE('',#16021,#15107,#9563,.T.);
#19999=EDGE_CURVE('',#16024,#16025,#9564,.T.);
#20000=EDGE_CURVE('',#16026,#16024,#9565,.T.);
#20001=EDGE_CURVE('',#16025,#16026,#9566,.T.);
#20002=EDGE_CURVE('',#15104,#16026,#9567,.T.);
#20003=EDGE_CURVE('',#16024,#15105,#9568,.T.);
#20004=EDGE_CURVE('',#16018,#16025,#9569,.T.);
#20005=EDGE_CURVE('',#16026,#16020,#9570,.T.);
#20006=EDGE_CURVE('',#16025,#16022,#9571,.T.);
#20007=EDGE_CURVE('',#16023,#16024,#9572,.T.);
#20008=EDGE_CURVE('',#16015,#16021,#9573,.T.);
#20009=EDGE_CURVE('',#16022,#16017,#9574,.T.);
#20010=EDGE_CURVE('',#15110,#16019,#9575,.T.);
#20011=EDGE_CURVE('',#16020,#15103,#9576,.T.);
#20012=EDGE_CURVE('',#16019,#16016,#9577,.T.);
#20013=EDGE_CURVE('',#16017,#16018,#9578,.T.);
#20014=EDGE_CURVE('',#15108,#16015,#9579,.T.);
#20015=EDGE_CURVE('',#16016,#15109,#9580,.T.);
#20016=EDGE_CURVE('',#16027,#16028,#9581,.T.);
#20017=EDGE_CURVE('',#16029,#16027,#9582,.T.);
#20018=EDGE_CURVE('',#16028,#16029,#9583,.T.);
#20019=EDGE_CURVE('',#16030,#16031,#9584,.T.);
#20020=EDGE_CURVE('',#16031,#16029,#9585,.T.);
#20021=EDGE_CURVE('',#16027,#16032,#9586,.T.);
#20022=EDGE_CURVE('',#16032,#16030,#9587,.T.);
#20023=EDGE_CURVE('',#15118,#16028,#9588,.T.);
#20024=EDGE_CURVE('',#16029,#15111,#9589,.T.);
#20025=EDGE_CURVE('',#16033,#16034,#9590,.T.);
#20026=EDGE_CURVE('',#16035,#16033,#9591,.T.);
#20027=EDGE_CURVE('',#16034,#16035,#9592,.T.);
#20028=EDGE_CURVE('',#16036,#16037,#9593,.T.);
#20029=EDGE_CURVE('',#16037,#16035,#9594,.T.);
#20030=EDGE_CURVE('',#16033,#16038,#9595,.T.);
#20031=EDGE_CURVE('',#16038,#16036,#9596,.T.);
#20032=EDGE_CURVE('',#16028,#16034,#9597,.T.);
#20033=EDGE_CURVE('',#16035,#16027,#9598,.T.);
#20034=EDGE_CURVE('',#15116,#16033,#9599,.T.);
#20035=EDGE_CURVE('',#16034,#15117,#9600,.T.);
#20036=EDGE_CURVE('',#16030,#16039,#9601,.T.);
#20037=EDGE_CURVE('',#16039,#15113,#9602,.T.);
#20038=EDGE_CURVE('',#15112,#16031,#9603,.T.);
#20039=EDGE_CURVE('',#16032,#16037,#9604,.T.);
#20040=EDGE_CURVE('',#16040,#16036,#9605,.T.);
#20041=EDGE_CURVE('',#16040,#16039,#9606,.T.);
#20042=EDGE_CURVE('',#16038,#15115,#9607,.T.);
#20043=EDGE_CURVE('',#15114,#16040,#9608,.T.);
#20044=EDGE_CURVE('',#16041,#16042,#9609,.T.);
#20045=EDGE_CURVE('',#16043,#16041,#9610,.T.);
#20046=EDGE_CURVE('',#16042,#16043,#9611,.T.);
#20047=EDGE_CURVE('',#16044,#16045,#9612,.T.);
#20048=EDGE_CURVE('',#16046,#16044,#9613,.T.);
#20049=EDGE_CURVE('',#16045,#16046,#9614,.T.);
#20050=EDGE_CURVE('',#16047,#16048,#9615,.T.);
#20051=EDGE_CURVE('',#16049,#16047,#9616,.T.);
#20052=EDGE_CURVE('',#16048,#16049,#9617,.T.);
#20053=EDGE_CURVE('',#15122,#16049,#9618,.T.);
#20054=EDGE_CURVE('',#16047,#15123,#9619,.T.);
#20055=EDGE_CURVE('',#16050,#16051,#9620,.T.);
#20056=EDGE_CURVE('',#16052,#16050,#9621,.T.);
#20057=EDGE_CURVE('',#16051,#16052,#9622,.T.);
#20058=EDGE_CURVE('',#15120,#16052,#9623,.T.);
#20059=EDGE_CURVE('',#16050,#15121,#9624,.T.);
#20060=EDGE_CURVE('',#16044,#16051,#9625,.T.);
#20061=EDGE_CURVE('',#16052,#16046,#9626,.T.);
#20062=EDGE_CURVE('',#16051,#16048,#9627,.T.);
#20063=EDGE_CURVE('',#16049,#16050,#9628,.T.);
#20064=EDGE_CURVE('',#16041,#16047,#9629,.T.);
#20065=EDGE_CURVE('',#16048,#16043,#9630,.T.);
#20066=EDGE_CURVE('',#15126,#16045,#9631,.T.);
#20067=EDGE_CURVE('',#16046,#15119,#9632,.T.);
#20068=EDGE_CURVE('',#16045,#16042,#9633,.T.);
#20069=EDGE_CURVE('',#16043,#16044,#9634,.T.);
#20070=EDGE_CURVE('',#15124,#16041,#9635,.T.);
#20071=EDGE_CURVE('',#16042,#15125,#9636,.T.);
#20072=EDGE_CURVE('',#16053,#16054,#9637,.T.);
#20073=EDGE_CURVE('',#16055,#16053,#9638,.T.);
#20074=EDGE_CURVE('',#16054,#16055,#9639,.T.);
#20075=EDGE_CURVE('',#16056,#16057,#9640,.T.);
#20076=EDGE_CURVE('',#16058,#16056,#9641,.T.);
#20077=EDGE_CURVE('',#16057,#16058,#9642,.T.);
#20078=EDGE_CURVE('',#16059,#16060,#9643,.T.);
#20079=EDGE_CURVE('',#16061,#16059,#9644,.T.);
#20080=EDGE_CURVE('',#16060,#16061,#9645,.T.);
#20081=EDGE_CURVE('',#15130,#16061,#9646,.T.);
#20082=EDGE_CURVE('',#16059,#15131,#9647,.T.);
#20083=EDGE_CURVE('',#16062,#16063,#9648,.T.);
#20084=EDGE_CURVE('',#16064,#16062,#9649,.T.);
#20085=EDGE_CURVE('',#16063,#16064,#9650,.T.);
#20086=EDGE_CURVE('',#15128,#16064,#9651,.T.);
#20087=EDGE_CURVE('',#16062,#15129,#9652,.T.);
#20088=EDGE_CURVE('',#16056,#16063,#9653,.T.);
#20089=EDGE_CURVE('',#16064,#16058,#9654,.T.);
#20090=EDGE_CURVE('',#16063,#16060,#9655,.T.);
#20091=EDGE_CURVE('',#16061,#16062,#9656,.T.);
#20092=EDGE_CURVE('',#16053,#16059,#9657,.T.);
#20093=EDGE_CURVE('',#16060,#16055,#9658,.T.);
#20094=EDGE_CURVE('',#15134,#16057,#9659,.T.);
#20095=EDGE_CURVE('',#16058,#15127,#9660,.T.);
#20096=EDGE_CURVE('',#16057,#16054,#9661,.T.);
#20097=EDGE_CURVE('',#16055,#16056,#9662,.T.);
#20098=EDGE_CURVE('',#15132,#16053,#9663,.T.);
#20099=EDGE_CURVE('',#16054,#15133,#9664,.T.);
#20100=EDGE_CURVE('',#16065,#16066,#13852,.T.);
#20101=EDGE_CURVE('',#16066,#16065,#13853,.T.);
#20102=EDGE_CURVE('',#16065,#16067,#9665,.T.);
#20103=EDGE_CURVE('',#16067,#16068,#13854,.T.);
#20104=EDGE_CURVE('',#16068,#16067,#13855,.T.);
#20105=EDGE_CURVE('',#16066,#16069,#9666,.T.);
#20106=EDGE_CURVE('',#16070,#16069,#13856,.T.);
#20107=EDGE_CURVE('',#16069,#16070,#13857,.T.);
#20108=EDGE_CURVE('',#16071,#16071,#13858,.T.);
#20109=EDGE_CURVE('',#16071,#16068,#9667,.T.);
#20110=EDGE_CURVE('',#16072,#16073,#9668,.T.);
#20111=EDGE_CURVE('',#16074,#16072,#9669,.T.);
#20112=EDGE_CURVE('',#16073,#16074,#9670,.T.);
#20113=EDGE_CURVE('',#16075,#16076,#9671,.T.);
#20114=EDGE_CURVE('',#16077,#16075,#9672,.T.);
#20115=EDGE_CURVE('',#16076,#16077,#9673,.T.);
#20116=EDGE_CURVE('',#16078,#16079,#9674,.T.);
#20117=EDGE_CURVE('',#16080,#16078,#9675,.T.);
#20118=EDGE_CURVE('',#16079,#16080,#9676,.T.);
#20119=EDGE_CURVE('',#15138,#16080,#9677,.T.);
#20120=EDGE_CURVE('',#16078,#15139,#9678,.T.);
#20121=EDGE_CURVE('',#16081,#16082,#9679,.T.);
#20122=EDGE_CURVE('',#16083,#16081,#9680,.T.);
#20123=EDGE_CURVE('',#16082,#16083,#9681,.T.);
#20124=EDGE_CURVE('',#15136,#16083,#9682,.T.);
#20125=EDGE_CURVE('',#16081,#15137,#9683,.T.);
#20126=EDGE_CURVE('',#16075,#16082,#9684,.T.);
#20127=EDGE_CURVE('',#16083,#16077,#9685,.T.);
#20128=EDGE_CURVE('',#16082,#16079,#9686,.T.);
#20129=EDGE_CURVE('',#16080,#16081,#9687,.T.);
#20130=EDGE_CURVE('',#16072,#16078,#9688,.T.);
#20131=EDGE_CURVE('',#16079,#16074,#9689,.T.);
#20132=EDGE_CURVE('',#15142,#16076,#9690,.T.);
#20133=EDGE_CURVE('',#16077,#15135,#9691,.T.);
#20134=EDGE_CURVE('',#16076,#16073,#9692,.T.);
#20135=EDGE_CURVE('',#16074,#16075,#9693,.T.);
#20136=EDGE_CURVE('',#15140,#16072,#9694,.T.);
#20137=EDGE_CURVE('',#16073,#15141,#9695,.T.);
#20138=EDGE_CURVE('',#16084,#16085,#9696,.T.);
#20139=EDGE_CURVE('',#16086,#16084,#9697,.T.);
#20140=EDGE_CURVE('',#16085,#16086,#9698,.T.);
#20141=EDGE_CURVE('',#16087,#16088,#9699,.T.);
#20142=EDGE_CURVE('',#16089,#16087,#9700,.T.);
#20143=EDGE_CURVE('',#16088,#16089,#9701,.T.);
#20144=EDGE_CURVE('',#16090,#16091,#9702,.T.);
#20145=EDGE_CURVE('',#16092,#16090,#9703,.T.);
#20146=EDGE_CURVE('',#16091,#16092,#9704,.T.);
#20147=EDGE_CURVE('',#15146,#16092,#9705,.T.);
#20148=EDGE_CURVE('',#16090,#15147,#9706,.T.);
#20149=EDGE_CURVE('',#16093,#16094,#9707,.T.);
#20150=EDGE_CURVE('',#16095,#16093,#9708,.T.);
#20151=EDGE_CURVE('',#16094,#16095,#9709,.T.);
#20152=EDGE_CURVE('',#15144,#16095,#9710,.T.);
#20153=EDGE_CURVE('',#16093,#15145,#9711,.T.);
#20154=EDGE_CURVE('',#16087,#16094,#9712,.T.);
#20155=EDGE_CURVE('',#16095,#16089,#9713,.T.);
#20156=EDGE_CURVE('',#16094,#16091,#9714,.T.);
#20157=EDGE_CURVE('',#16092,#16093,#9715,.T.);
#20158=EDGE_CURVE('',#16084,#16090,#9716,.T.);
#20159=EDGE_CURVE('',#16091,#16086,#9717,.T.);
#20160=EDGE_CURVE('',#15150,#16088,#9718,.T.);
#20161=EDGE_CURVE('',#16089,#15143,#9719,.T.);
#20162=EDGE_CURVE('',#16088,#16085,#9720,.T.);
#20163=EDGE_CURVE('',#16086,#16087,#9721,.T.);
#20164=EDGE_CURVE('',#15148,#16084,#9722,.T.);
#20165=EDGE_CURVE('',#16085,#15149,#9723,.T.);
#20166=EDGE_CURVE('',#16096,#16097,#13859,.T.);
#20167=EDGE_CURVE('',#16097,#16096,#13860,.T.);
#20168=EDGE_CURVE('',#16096,#16098,#9724,.T.);
#20169=EDGE_CURVE('',#16098,#16099,#13861,.T.);
#20170=EDGE_CURVE('',#16099,#16098,#13862,.T.);
#20171=EDGE_CURVE('',#16099,#16100,#9725,.T.);
#20172=EDGE_CURVE('',#16101,#16100,#13863,.T.);
#20173=EDGE_CURVE('',#16100,#16101,#13864,.T.);
#20174=EDGE_CURVE('',#14578,#16097,#9726,.T.);
#20175=EDGE_CURVE('',#16102,#16102,#13865,.T.);
#20176=EDGE_CURVE('',#16102,#16070,#9727,.T.);
#20177=EDGE_CURVE('',#16103,#16103,#13866,.T.);
#20178=EDGE_CURVE('',#16104,#16104,#13867,.T.);
#20179=EDGE_CURVE('',#16104,#16101,#9728,.T.);
#20180=EDGE_CURVE('',#16104,#16105,#9729,.T.);
#20181=EDGE_CURVE('',#16105,#16105,#13868,.T.);
#20182=EDGE_CURVE('',#16105,#16103,#9730,.T.);
#20183=EDGE_CURVE('',#15178,#16106,#9731,.T.);
#20184=EDGE_CURVE('',#16106,#16106,#13869,.T.);
#20185=EDGE_CURVE('',#15179,#16107,#9732,.T.);
#20186=EDGE_CURVE('',#16107,#16107,#13870,.T.);
#20187=EDGE_CURVE('',#15180,#16108,#9733,.T.);
#20188=EDGE_CURVE('',#16108,#16108,#13871,.T.);
#20189=EDGE_CURVE('',#15181,#16109,#9734,.T.);
#20190=EDGE_CURVE('',#16109,#16109,#13872,.T.);
#20191=EDGE_CURVE('',#15182,#16110,#9735,.T.);
#20192=EDGE_CURVE('',#16110,#16110,#13873,.T.);
#20193=EDGE_CURVE('',#16111,#16111,#13874,.T.);
#20194=EDGE_CURVE('',#16111,#16112,#9736,.T.);
#20195=EDGE_CURVE('',#16112,#16112,#13875,.T.);
#20196=EDGE_CURVE('',#16112,#16113,#9737,.T.);
#20197=EDGE_CURVE('',#16113,#16113,#13876,.T.);
#20198=EDGE_CURVE('',#16114,#15156,#9738,.T.);
#20199=EDGE_CURVE('',#15177,#16114,#13877,.T.);
#20200=EDGE_CURVE('',#16115,#15158,#9739,.T.);
#20201=EDGE_CURVE('',#16114,#16115,#13878,.T.);
#20202=EDGE_CURVE('',#16116,#15160,#9740,.T.);
#20203=EDGE_CURVE('',#16115,#16116,#13879,.T.);
#20204=EDGE_CURVE('',#16116,#15172,#13880,.T.);
#20205=EDGE_CURVE('',#14551,#16117,#9741,.T.);
#20206=EDGE_CURVE('',#16117,#16117,#13881,.T.);
#20207=EDGE_CURVE('',#16111,#16118,#9742,.T.);
#20208=EDGE_CURVE('',#16118,#16118,#13882,.T.);
#20209=EDGE_CURVE('',#14545,#16119,#9743,.T.);
#20210=EDGE_CURVE('',#16119,#16119,#13883,.T.);
#20211=EDGE_CURVE('',#16120,#16120,#13884,.T.);
#20212=EDGE_CURVE('',#16120,#16121,#9744,.T.);
#20213=EDGE_CURVE('',#16121,#16121,#13885,.T.);
#20214=EDGE_CURVE('',#16121,#14540,#9745,.T.);
#20215=EDGE_CURVE('',#16122,#16122,#13886,.T.);
#20216=EDGE_CURVE('',#16122,#14538,#9746,.T.);
#20217=EDGE_CURVE('',#16123,#16123,#13887,.T.);
#20218=EDGE_CURVE('',#16123,#16124,#9747,.T.);
#20219=EDGE_CURVE('',#16124,#16124,#13888,.T.);
#20220=EDGE_CURVE('',#16124,#16071,#9748,.T.);
#22278=ORIENTED_EDGE('',*,*,#17453,.T.);
#22279=ORIENTED_EDGE('',*,*,#17454,.T.);
#22280=ORIENTED_EDGE('',*,*,#17455,.T.);
#22281=ORIENTED_EDGE('',*,*,#17456,.T.);
#22282=ORIENTED_EDGE('',*,*,#17457,.T.);
#22283=ORIENTED_EDGE('',*,*,#17455,.F.);
#22284=ORIENTED_EDGE('',*,*,#17456,.F.);
#22285=ORIENTED_EDGE('',*,*,#17457,.F.);
#22286=ORIENTED_EDGE('',*,*,#17458,.T.);
#22287=ORIENTED_EDGE('',*,*,#17459,.F.);
#22288=ORIENTED_EDGE('',*,*,#17460,.F.);
#22289=ORIENTED_EDGE('',*,*,#17458,.F.);
#22290=ORIENTED_EDGE('',*,*,#17461,.F.);
#22291=ORIENTED_EDGE('',*,*,#17462,.T.);
#22292=ORIENTED_EDGE('',*,*,#17453,.F.);
#22293=ORIENTED_EDGE('',*,*,#17454,.F.);
#22294=ORIENTED_EDGE('',*,*,#17462,.F.);
#22295=ORIENTED_EDGE('',*,*,#17459,.T.);
#22296=ORIENTED_EDGE('',*,*,#17460,.T.);
#22297=ORIENTED_EDGE('',*,*,#17463,.T.);
#22298=ORIENTED_EDGE('',*,*,#17464,.T.);
#22299=ORIENTED_EDGE('',*,*,#17463,.F.);
#22300=ORIENTED_EDGE('',*,*,#17464,.F.);
#22301=ORIENTED_EDGE('',*,*,#17465,.T.);
#22302=ORIENTED_EDGE('',*,*,#17466,.T.);
#22303=ORIENTED_EDGE('',*,*,#17467,.T.);
#22304=ORIENTED_EDGE('',*,*,#17468,.T.);
#22305=ORIENTED_EDGE('',*,*,#17469,.T.);
#22306=ORIENTED_EDGE('',*,*,#17467,.F.);
#22307=ORIENTED_EDGE('',*,*,#17470,.T.);
#22308=ORIENTED_EDGE('',*,*,#17471,.T.);
#22309=ORIENTED_EDGE('',*,*,#17468,.F.);
#22310=ORIENTED_EDGE('',*,*,#17469,.F.);
#22311=ORIENTED_EDGE('',*,*,#17471,.F.);
#22312=ORIENTED_EDGE('',*,*,#17472,.F.);
#22313=ORIENTED_EDGE('',*,*,#17466,.F.);
#22314=ORIENTED_EDGE('',*,*,#17473,.T.);
#22315=ORIENTED_EDGE('',*,*,#17474,.T.);
#22316=ORIENTED_EDGE('',*,*,#17475,.T.);
#22317=ORIENTED_EDGE('',*,*,#17476,.T.);
#22318=ORIENTED_EDGE('',*,*,#17474,.F.);
#22319=ORIENTED_EDGE('',*,*,#17475,.F.);
#22320=ORIENTED_EDGE('',*,*,#17476,.F.);
#22321=ORIENTED_EDGE('',*,*,#17477,.T.);
#22322=ORIENTED_EDGE('',*,*,#17478,.F.);
#22323=ORIENTED_EDGE('',*,*,#17479,.F.);
#22324=ORIENTED_EDGE('',*,*,#17477,.F.);
#22325=ORIENTED_EDGE('',*,*,#17473,.F.);
#22326=ORIENTED_EDGE('',*,*,#17480,.F.);
#22327=ORIENTED_EDGE('',*,*,#17478,.T.);
#22328=ORIENTED_EDGE('',*,*,#17479,.T.);
#22329=ORIENTED_EDGE('',*,*,#17481,.T.);
#22330=ORIENTED_EDGE('',*,*,#17482,.T.);
#22331=ORIENTED_EDGE('',*,*,#17483,.T.);
#22332=ORIENTED_EDGE('',*,*,#17481,.F.);
#22333=ORIENTED_EDGE('',*,*,#17482,.F.);
#22334=ORIENTED_EDGE('',*,*,#17483,.F.);
#22335=ORIENTED_EDGE('',*,*,#17484,.T.);
#22336=ORIENTED_EDGE('',*,*,#17485,.T.);
#22337=ORIENTED_EDGE('',*,*,#17484,.F.);
#22338=ORIENTED_EDGE('',*,*,#17486,.T.);
#22339=ORIENTED_EDGE('',*,*,#17487,.T.);
#22340=ORIENTED_EDGE('',*,*,#17488,.T.);
#22341=ORIENTED_EDGE('',*,*,#17489,.T.);
#22342=ORIENTED_EDGE('',*,*,#17490,.T.);
#22343=ORIENTED_EDGE('',*,*,#17488,.F.);
#22344=ORIENTED_EDGE('',*,*,#17489,.F.);
#22345=ORIENTED_EDGE('',*,*,#17490,.F.);
#22346=ORIENTED_EDGE('',*,*,#17491,.T.);
#22347=ORIENTED_EDGE('',*,*,#17492,.F.);
#22348=ORIENTED_EDGE('',*,*,#17493,.F.);
#22349=ORIENTED_EDGE('',*,*,#17491,.F.);
#22350=ORIENTED_EDGE('',*,*,#17494,.F.);
#22351=ORIENTED_EDGE('',*,*,#17495,.T.);
#22352=ORIENTED_EDGE('',*,*,#17486,.F.);
#22353=ORIENTED_EDGE('',*,*,#17487,.F.);
#22354=ORIENTED_EDGE('',*,*,#17495,.F.);
#22355=ORIENTED_EDGE('',*,*,#17492,.T.);
#22356=ORIENTED_EDGE('',*,*,#17493,.T.);
#22357=ORIENTED_EDGE('',*,*,#17496,.T.);
#22358=ORIENTED_EDGE('',*,*,#17497,.T.);
#22359=ORIENTED_EDGE('',*,*,#17498,.T.);
#22360=ORIENTED_EDGE('',*,*,#17496,.F.);
#22361=ORIENTED_EDGE('',*,*,#17497,.F.);
#22362=ORIENTED_EDGE('',*,*,#17498,.F.);
#22363=ORIENTED_EDGE('',*,*,#17499,.T.);
#22364=ORIENTED_EDGE('',*,*,#17500,.F.);
#22365=ORIENTED_EDGE('',*,*,#17501,.F.);
#22366=ORIENTED_EDGE('',*,*,#17499,.F.);
#22367=ORIENTED_EDGE('',*,*,#17500,.T.);
#22368=ORIENTED_EDGE('',*,*,#17501,.T.);
#22369=ORIENTED_EDGE('',*,*,#17502,.T.);
#22370=ORIENTED_EDGE('',*,*,#17503,.T.);
#22371=ORIENTED_EDGE('',*,*,#17504,.T.);
#22372=ORIENTED_EDGE('',*,*,#17502,.F.);
#22373=ORIENTED_EDGE('',*,*,#17503,.F.);
#22374=ORIENTED_EDGE('',*,*,#17504,.F.);
#22375=ORIENTED_EDGE('',*,*,#17505,.T.);
#22376=ORIENTED_EDGE('',*,*,#17506,.F.);
#22377=ORIENTED_EDGE('',*,*,#17507,.F.);
#22378=ORIENTED_EDGE('',*,*,#17505,.F.);
#22379=ORIENTED_EDGE('',*,*,#17506,.T.);
#22380=ORIENTED_EDGE('',*,*,#17507,.T.);
#22381=ORIENTED_EDGE('',*,*,#17508,.T.);
#22382=ORIENTED_EDGE('',*,*,#17509,.T.);
#22383=ORIENTED_EDGE('',*,*,#17510,.T.);
#22384=ORIENTED_EDGE('',*,*,#17508,.F.);
#22385=ORIENTED_EDGE('',*,*,#17509,.F.);
#22386=ORIENTED_EDGE('',*,*,#17510,.F.);
#22387=ORIENTED_EDGE('',*,*,#17511,.T.);
#22388=ORIENTED_EDGE('',*,*,#17512,.T.);
#22389=ORIENTED_EDGE('',*,*,#17513,.F.);
#22390=ORIENTED_EDGE('',*,*,#17514,.T.);
#22391=ORIENTED_EDGE('',*,*,#17515,.F.);
#22392=ORIENTED_EDGE('',*,*,#17516,.T.);
#22393=ORIENTED_EDGE('',*,*,#17517,.T.);
#22394=ORIENTED_EDGE('',*,*,#17518,.T.);
#22395=ORIENTED_EDGE('',*,*,#17517,.F.);
#22396=ORIENTED_EDGE('',*,*,#17519,.T.);
#22397=ORIENTED_EDGE('',*,*,#17520,.F.);
#22398=ORIENTED_EDGE('',*,*,#17521,.T.);
#22399=ORIENTED_EDGE('',*,*,#17522,.F.);
#22400=ORIENTED_EDGE('',*,*,#17523,.T.);
#22401=ORIENTED_EDGE('',*,*,#17511,.F.);
#22402=ORIENTED_EDGE('',*,*,#17524,.T.);
#22403=ORIENTED_EDGE('',*,*,#17525,.F.);
#22404=ORIENTED_EDGE('',*,*,#17526,.T.);
#22405=ORIENTED_EDGE('',*,*,#17527,.F.);
#22406=ORIENTED_EDGE('',*,*,#17528,.T.);
#22407=ORIENTED_EDGE('',*,*,#17529,.F.);
#22408=ORIENTED_EDGE('',*,*,#17530,.T.);
#22409=ORIENTED_EDGE('',*,*,#17531,.F.);
#22410=ORIENTED_EDGE('',*,*,#17532,.T.);
#22411=ORIENTED_EDGE('',*,*,#17533,.F.);
#22412=ORIENTED_EDGE('',*,*,#17534,.T.);
#22413=ORIENTED_EDGE('',*,*,#17535,.F.);
#22414=ORIENTED_EDGE('',*,*,#17536,.T.);
#22415=ORIENTED_EDGE('',*,*,#17537,.F.);
#22416=ORIENTED_EDGE('',*,*,#17538,.T.);
#22417=ORIENTED_EDGE('',*,*,#17539,.F.);
#22418=ORIENTED_EDGE('',*,*,#17540,.T.);
#22419=ORIENTED_EDGE('',*,*,#17541,.F.);
#22420=ORIENTED_EDGE('',*,*,#17542,.T.);
#22421=ORIENTED_EDGE('',*,*,#17543,.F.);
#22422=ORIENTED_EDGE('',*,*,#17544,.T.);
#22423=ORIENTED_EDGE('',*,*,#17545,.F.);
#22424=ORIENTED_EDGE('',*,*,#17546,.T.);
#22425=ORIENTED_EDGE('',*,*,#17547,.F.);
#22426=ORIENTED_EDGE('',*,*,#17548,.T.);
#22427=ORIENTED_EDGE('',*,*,#17549,.F.);
#22428=ORIENTED_EDGE('',*,*,#17550,.T.);
#22429=ORIENTED_EDGE('',*,*,#17551,.F.);
#22430=ORIENTED_EDGE('',*,*,#17552,.T.);
#22431=ORIENTED_EDGE('',*,*,#17553,.F.);
#22432=ORIENTED_EDGE('',*,*,#17554,.T.);
#22433=ORIENTED_EDGE('',*,*,#17555,.F.);
#22434=ORIENTED_EDGE('',*,*,#17556,.T.);
#22435=ORIENTED_EDGE('',*,*,#17557,.F.);
#22436=ORIENTED_EDGE('',*,*,#17558,.T.);
#22437=ORIENTED_EDGE('',*,*,#17559,.F.);
#22438=ORIENTED_EDGE('',*,*,#17560,.T.);
#22439=ORIENTED_EDGE('',*,*,#17561,.F.);
#22440=ORIENTED_EDGE('',*,*,#17562,.T.);
#22441=ORIENTED_EDGE('',*,*,#17563,.F.);
#22442=ORIENTED_EDGE('',*,*,#17564,.T.);
#22443=ORIENTED_EDGE('',*,*,#17565,.F.);
#22444=ORIENTED_EDGE('',*,*,#17566,.T.);
#22445=ORIENTED_EDGE('',*,*,#17567,.F.);
#22446=ORIENTED_EDGE('',*,*,#17568,.T.);
#22447=ORIENTED_EDGE('',*,*,#17569,.F.);
#22448=ORIENTED_EDGE('',*,*,#17570,.T.);
#22449=ORIENTED_EDGE('',*,*,#17571,.F.);
#22450=ORIENTED_EDGE('',*,*,#17572,.T.);
#22451=ORIENTED_EDGE('',*,*,#17573,.F.);
#22452=ORIENTED_EDGE('',*,*,#17574,.T.);
#22453=ORIENTED_EDGE('',*,*,#17575,.F.);
#22454=ORIENTED_EDGE('',*,*,#17576,.T.);
#22455=ORIENTED_EDGE('',*,*,#17577,.F.);
#22456=ORIENTED_EDGE('',*,*,#17578,.T.);
#22457=ORIENTED_EDGE('',*,*,#17579,.F.);
#22458=ORIENTED_EDGE('',*,*,#17580,.T.);
#22459=ORIENTED_EDGE('',*,*,#17581,.F.);
#22460=ORIENTED_EDGE('',*,*,#17582,.T.);
#22461=ORIENTED_EDGE('',*,*,#17583,.F.);
#22462=ORIENTED_EDGE('',*,*,#17584,.T.);
#22463=ORIENTED_EDGE('',*,*,#17585,.F.);
#22464=ORIENTED_EDGE('',*,*,#17586,.T.);
#22465=ORIENTED_EDGE('',*,*,#17587,.F.);
#22466=ORIENTED_EDGE('',*,*,#17588,.T.);
#22467=ORIENTED_EDGE('',*,*,#17589,.F.);
#22468=ORIENTED_EDGE('',*,*,#17590,.T.);
#22469=ORIENTED_EDGE('',*,*,#17591,.F.);
#22470=ORIENTED_EDGE('',*,*,#17592,.T.);
#22471=ORIENTED_EDGE('',*,*,#17593,.F.);
#22472=ORIENTED_EDGE('',*,*,#17594,.T.);
#22473=ORIENTED_EDGE('',*,*,#17595,.F.);
#22474=ORIENTED_EDGE('',*,*,#17596,.T.);
#22475=ORIENTED_EDGE('',*,*,#17597,.F.);
#22476=ORIENTED_EDGE('',*,*,#17598,.T.);
#22477=ORIENTED_EDGE('',*,*,#17599,.F.);
#22478=ORIENTED_EDGE('',*,*,#17600,.T.);
#22479=ORIENTED_EDGE('',*,*,#17601,.F.);
#22480=ORIENTED_EDGE('',*,*,#17602,.T.);
#22481=ORIENTED_EDGE('',*,*,#17603,.F.);
#22482=ORIENTED_EDGE('',*,*,#17604,.T.);
#22483=ORIENTED_EDGE('',*,*,#17605,.F.);
#22484=ORIENTED_EDGE('',*,*,#17606,.T.);
#22485=ORIENTED_EDGE('',*,*,#17607,.F.);
#22486=ORIENTED_EDGE('',*,*,#17608,.T.);
#22487=ORIENTED_EDGE('',*,*,#17609,.F.);
#22488=ORIENTED_EDGE('',*,*,#17610,.T.);
#22489=ORIENTED_EDGE('',*,*,#17611,.F.);
#22490=ORIENTED_EDGE('',*,*,#17612,.T.);
#22491=ORIENTED_EDGE('',*,*,#17613,.F.);
#22492=ORIENTED_EDGE('',*,*,#17614,.T.);
#22493=ORIENTED_EDGE('',*,*,#17615,.F.);
#22494=ORIENTED_EDGE('',*,*,#17616,.T.);
#22495=ORIENTED_EDGE('',*,*,#17617,.F.);
#22496=ORIENTED_EDGE('',*,*,#17618,.T.);
#22497=ORIENTED_EDGE('',*,*,#17619,.F.);
#22498=ORIENTED_EDGE('',*,*,#17620,.T.);
#22499=ORIENTED_EDGE('',*,*,#17621,.F.);
#22500=ORIENTED_EDGE('',*,*,#17622,.T.);
#22501=ORIENTED_EDGE('',*,*,#17623,.F.);
#22502=ORIENTED_EDGE('',*,*,#17624,.T.);
#22503=ORIENTED_EDGE('',*,*,#17625,.F.);
#22504=ORIENTED_EDGE('',*,*,#17626,.T.);
#22505=ORIENTED_EDGE('',*,*,#17627,.F.);
#22506=ORIENTED_EDGE('',*,*,#17628,.T.);
#22507=ORIENTED_EDGE('',*,*,#17629,.F.);
#22508=ORIENTED_EDGE('',*,*,#17630,.T.);
#22509=ORIENTED_EDGE('',*,*,#17631,.F.);
#22510=ORIENTED_EDGE('',*,*,#17632,.T.);
#22511=ORIENTED_EDGE('',*,*,#17633,.F.);
#22512=ORIENTED_EDGE('',*,*,#17634,.T.);
#22513=ORIENTED_EDGE('',*,*,#17635,.F.);
#22514=ORIENTED_EDGE('',*,*,#17636,.T.);
#22515=ORIENTED_EDGE('',*,*,#17637,.F.);
#22516=ORIENTED_EDGE('',*,*,#17638,.T.);
#22517=ORIENTED_EDGE('',*,*,#17639,.F.);
#22518=ORIENTED_EDGE('',*,*,#17640,.T.);
#22519=ORIENTED_EDGE('',*,*,#17641,.F.);
#22520=ORIENTED_EDGE('',*,*,#17642,.T.);
#22521=ORIENTED_EDGE('',*,*,#17643,.F.);
#22522=ORIENTED_EDGE('',*,*,#17644,.T.);
#22523=ORIENTED_EDGE('',*,*,#17645,.F.);
#22524=ORIENTED_EDGE('',*,*,#17646,.T.);
#22525=ORIENTED_EDGE('',*,*,#17647,.F.);
#22526=ORIENTED_EDGE('',*,*,#17648,.T.);
#22527=ORIENTED_EDGE('',*,*,#17649,.F.);
#22528=ORIENTED_EDGE('',*,*,#17650,.T.);
#22529=ORIENTED_EDGE('',*,*,#17651,.F.);
#22530=ORIENTED_EDGE('',*,*,#17652,.T.);
#22531=ORIENTED_EDGE('',*,*,#17653,.F.);
#22532=ORIENTED_EDGE('',*,*,#17654,.T.);
#22533=ORIENTED_EDGE('',*,*,#17655,.F.);
#22534=ORIENTED_EDGE('',*,*,#17656,.T.);
#22535=ORIENTED_EDGE('',*,*,#17657,.F.);
#22536=ORIENTED_EDGE('',*,*,#17658,.T.);
#22537=ORIENTED_EDGE('',*,*,#17659,.F.);
#22538=ORIENTED_EDGE('',*,*,#17660,.T.);
#22539=ORIENTED_EDGE('',*,*,#17661,.F.);
#22540=ORIENTED_EDGE('',*,*,#17662,.T.);
#22541=ORIENTED_EDGE('',*,*,#17663,.F.);
#22542=ORIENTED_EDGE('',*,*,#17664,.T.);
#22543=ORIENTED_EDGE('',*,*,#17665,.F.);
#22544=ORIENTED_EDGE('',*,*,#17666,.T.);
#22545=ORIENTED_EDGE('',*,*,#17667,.F.);
#22546=ORIENTED_EDGE('',*,*,#17668,.T.);
#22547=ORIENTED_EDGE('',*,*,#17669,.F.);
#22548=ORIENTED_EDGE('',*,*,#17670,.T.);
#22549=ORIENTED_EDGE('',*,*,#17671,.F.);
#22550=ORIENTED_EDGE('',*,*,#17672,.T.);
#22551=ORIENTED_EDGE('',*,*,#17673,.F.);
#22552=ORIENTED_EDGE('',*,*,#17674,.T.);
#22553=ORIENTED_EDGE('',*,*,#17675,.F.);
#22554=ORIENTED_EDGE('',*,*,#17676,.T.);
#22555=ORIENTED_EDGE('',*,*,#17677,.F.);
#22556=ORIENTED_EDGE('',*,*,#17678,.T.);
#22557=ORIENTED_EDGE('',*,*,#17679,.F.);
#22558=ORIENTED_EDGE('',*,*,#17680,.T.);
#22559=ORIENTED_EDGE('',*,*,#17681,.F.);
#22560=ORIENTED_EDGE('',*,*,#17682,.T.);
#22561=ORIENTED_EDGE('',*,*,#17683,.F.);
#22562=ORIENTED_EDGE('',*,*,#17684,.T.);
#22563=ORIENTED_EDGE('',*,*,#17685,.F.);
#22564=ORIENTED_EDGE('',*,*,#17686,.T.);
#22565=ORIENTED_EDGE('',*,*,#17687,.F.);
#22566=ORIENTED_EDGE('',*,*,#17688,.T.);
#22567=ORIENTED_EDGE('',*,*,#17689,.F.);
#22568=ORIENTED_EDGE('',*,*,#17690,.T.);
#22569=ORIENTED_EDGE('',*,*,#17691,.F.);
#22570=ORIENTED_EDGE('',*,*,#17692,.T.);
#22571=ORIENTED_EDGE('',*,*,#17693,.F.);
#22572=ORIENTED_EDGE('',*,*,#17694,.T.);
#22573=ORIENTED_EDGE('',*,*,#17695,.F.);
#22574=ORIENTED_EDGE('',*,*,#17696,.T.);
#22575=ORIENTED_EDGE('',*,*,#17697,.F.);
#22576=ORIENTED_EDGE('',*,*,#17698,.T.);
#22577=ORIENTED_EDGE('',*,*,#17699,.F.);
#22578=ORIENTED_EDGE('',*,*,#17700,.T.);
#22579=ORIENTED_EDGE('',*,*,#17701,.F.);
#22580=ORIENTED_EDGE('',*,*,#17702,.T.);
#22581=ORIENTED_EDGE('',*,*,#17703,.F.);
#22582=ORIENTED_EDGE('',*,*,#17704,.T.);
#22583=ORIENTED_EDGE('',*,*,#17705,.F.);
#22584=ORIENTED_EDGE('',*,*,#17706,.T.);
#22585=ORIENTED_EDGE('',*,*,#17707,.F.);
#22586=ORIENTED_EDGE('',*,*,#17708,.T.);
#22587=ORIENTED_EDGE('',*,*,#17709,.F.);
#22588=ORIENTED_EDGE('',*,*,#17710,.T.);
#22589=ORIENTED_EDGE('',*,*,#17711,.F.);
#22590=ORIENTED_EDGE('',*,*,#17712,.T.);
#22591=ORIENTED_EDGE('',*,*,#17713,.F.);
#22592=ORIENTED_EDGE('',*,*,#17714,.T.);
#22593=ORIENTED_EDGE('',*,*,#17715,.F.);
#22594=ORIENTED_EDGE('',*,*,#17716,.T.);
#22595=ORIENTED_EDGE('',*,*,#17717,.F.);
#22596=ORIENTED_EDGE('',*,*,#17718,.T.);
#22597=ORIENTED_EDGE('',*,*,#17719,.F.);
#22598=ORIENTED_EDGE('',*,*,#17720,.T.);
#22599=ORIENTED_EDGE('',*,*,#17721,.F.);
#22600=ORIENTED_EDGE('',*,*,#17722,.T.);
#22601=ORIENTED_EDGE('',*,*,#17723,.F.);
#22602=ORIENTED_EDGE('',*,*,#17724,.T.);
#22603=ORIENTED_EDGE('',*,*,#17725,.F.);
#22604=ORIENTED_EDGE('',*,*,#17726,.T.);
#22605=ORIENTED_EDGE('',*,*,#17727,.F.);
#22606=ORIENTED_EDGE('',*,*,#17728,.T.);
#22607=ORIENTED_EDGE('',*,*,#17729,.F.);
#22608=ORIENTED_EDGE('',*,*,#17730,.T.);
#22609=ORIENTED_EDGE('',*,*,#17731,.F.);
#22610=ORIENTED_EDGE('',*,*,#17732,.T.);
#22611=ORIENTED_EDGE('',*,*,#17733,.F.);
#22612=ORIENTED_EDGE('',*,*,#17734,.T.);
#22613=ORIENTED_EDGE('',*,*,#17735,.F.);
#22614=ORIENTED_EDGE('',*,*,#17736,.T.);
#22615=ORIENTED_EDGE('',*,*,#17737,.F.);
#22616=ORIENTED_EDGE('',*,*,#17738,.T.);
#22617=ORIENTED_EDGE('',*,*,#17739,.F.);
#22618=ORIENTED_EDGE('',*,*,#17740,.T.);
#22619=ORIENTED_EDGE('',*,*,#17741,.F.);
#22620=ORIENTED_EDGE('',*,*,#17742,.T.);
#22621=ORIENTED_EDGE('',*,*,#17743,.F.);
#22622=ORIENTED_EDGE('',*,*,#17744,.T.);
#22623=ORIENTED_EDGE('',*,*,#17745,.F.);
#22624=ORIENTED_EDGE('',*,*,#17746,.T.);
#22625=ORIENTED_EDGE('',*,*,#17747,.F.);
#22626=ORIENTED_EDGE('',*,*,#17748,.T.);
#22627=ORIENTED_EDGE('',*,*,#17749,.F.);
#22628=ORIENTED_EDGE('',*,*,#17750,.T.);
#22629=ORIENTED_EDGE('',*,*,#17751,.F.);
#22630=ORIENTED_EDGE('',*,*,#17752,.T.);
#22631=ORIENTED_EDGE('',*,*,#17753,.F.);
#22632=ORIENTED_EDGE('',*,*,#17754,.T.);
#22633=ORIENTED_EDGE('',*,*,#17755,.F.);
#22634=ORIENTED_EDGE('',*,*,#17756,.T.);
#22635=ORIENTED_EDGE('',*,*,#17757,.F.);
#22636=ORIENTED_EDGE('',*,*,#17758,.T.);
#22637=ORIENTED_EDGE('',*,*,#17759,.F.);
#22638=ORIENTED_EDGE('',*,*,#17760,.T.);
#22639=ORIENTED_EDGE('',*,*,#17761,.F.);
#22640=ORIENTED_EDGE('',*,*,#17762,.T.);
#22641=ORIENTED_EDGE('',*,*,#17763,.F.);
#22642=ORIENTED_EDGE('',*,*,#17764,.T.);
#22643=ORIENTED_EDGE('',*,*,#17765,.F.);
#22644=ORIENTED_EDGE('',*,*,#17766,.T.);
#22645=ORIENTED_EDGE('',*,*,#17767,.F.);
#22646=ORIENTED_EDGE('',*,*,#17768,.T.);
#22647=ORIENTED_EDGE('',*,*,#17769,.F.);
#22648=ORIENTED_EDGE('',*,*,#17770,.T.);
#22649=ORIENTED_EDGE('',*,*,#17771,.F.);
#22650=ORIENTED_EDGE('',*,*,#17772,.T.);
#22651=ORIENTED_EDGE('',*,*,#17773,.F.);
#22652=ORIENTED_EDGE('',*,*,#17774,.T.);
#22653=ORIENTED_EDGE('',*,*,#17775,.F.);
#22654=ORIENTED_EDGE('',*,*,#17776,.T.);
#22655=ORIENTED_EDGE('',*,*,#17777,.F.);
#22656=ORIENTED_EDGE('',*,*,#17778,.T.);
#22657=ORIENTED_EDGE('',*,*,#17779,.F.);
#22658=ORIENTED_EDGE('',*,*,#17780,.T.);
#22659=ORIENTED_EDGE('',*,*,#17781,.F.);
#22660=ORIENTED_EDGE('',*,*,#17782,.T.);
#22661=ORIENTED_EDGE('',*,*,#17783,.F.);
#22662=ORIENTED_EDGE('',*,*,#17784,.T.);
#22663=ORIENTED_EDGE('',*,*,#17785,.F.);
#22664=ORIENTED_EDGE('',*,*,#17786,.T.);
#22665=ORIENTED_EDGE('',*,*,#17787,.F.);
#22666=ORIENTED_EDGE('',*,*,#17788,.T.);
#22667=ORIENTED_EDGE('',*,*,#17789,.F.);
#22668=ORIENTED_EDGE('',*,*,#17790,.T.);
#22669=ORIENTED_EDGE('',*,*,#17791,.F.);
#22670=ORIENTED_EDGE('',*,*,#17792,.T.);
#22671=ORIENTED_EDGE('',*,*,#17793,.F.);
#22672=ORIENTED_EDGE('',*,*,#17794,.T.);
#22673=ORIENTED_EDGE('',*,*,#17795,.F.);
#22674=ORIENTED_EDGE('',*,*,#17796,.T.);
#22675=ORIENTED_EDGE('',*,*,#17797,.F.);
#22676=ORIENTED_EDGE('',*,*,#17798,.T.);
#22677=ORIENTED_EDGE('',*,*,#17799,.F.);
#22678=ORIENTED_EDGE('',*,*,#17800,.T.);
#22679=ORIENTED_EDGE('',*,*,#17801,.F.);
#22680=ORIENTED_EDGE('',*,*,#17802,.T.);
#22681=ORIENTED_EDGE('',*,*,#17803,.F.);
#22682=ORIENTED_EDGE('',*,*,#17804,.T.);
#22683=ORIENTED_EDGE('',*,*,#17805,.F.);
#22684=ORIENTED_EDGE('',*,*,#17806,.T.);
#22685=ORIENTED_EDGE('',*,*,#17807,.F.);
#22686=ORIENTED_EDGE('',*,*,#17808,.T.);
#22687=ORIENTED_EDGE('',*,*,#17809,.F.);
#22688=ORIENTED_EDGE('',*,*,#17810,.T.);
#22689=ORIENTED_EDGE('',*,*,#17811,.F.);
#22690=ORIENTED_EDGE('',*,*,#17812,.T.);
#22691=ORIENTED_EDGE('',*,*,#17813,.F.);
#22692=ORIENTED_EDGE('',*,*,#17814,.T.);
#22693=ORIENTED_EDGE('',*,*,#17815,.F.);
#22694=ORIENTED_EDGE('',*,*,#17816,.T.);
#22695=ORIENTED_EDGE('',*,*,#17817,.F.);
#22696=ORIENTED_EDGE('',*,*,#17818,.T.);
#22697=ORIENTED_EDGE('',*,*,#17819,.F.);
#22698=ORIENTED_EDGE('',*,*,#17820,.T.);
#22699=ORIENTED_EDGE('',*,*,#17821,.F.);
#22700=ORIENTED_EDGE('',*,*,#17822,.T.);
#22701=ORIENTED_EDGE('',*,*,#17823,.F.);
#22702=ORIENTED_EDGE('',*,*,#17824,.T.);
#22703=ORIENTED_EDGE('',*,*,#17825,.F.);
#22704=ORIENTED_EDGE('',*,*,#17826,.T.);
#22705=ORIENTED_EDGE('',*,*,#17827,.F.);
#22706=ORIENTED_EDGE('',*,*,#17828,.T.);
#22707=ORIENTED_EDGE('',*,*,#17829,.F.);
#22708=ORIENTED_EDGE('',*,*,#17830,.T.);
#22709=ORIENTED_EDGE('',*,*,#17831,.F.);
#22710=ORIENTED_EDGE('',*,*,#17832,.T.);
#22711=ORIENTED_EDGE('',*,*,#17833,.F.);
#22712=ORIENTED_EDGE('',*,*,#17834,.T.);
#22713=ORIENTED_EDGE('',*,*,#17835,.F.);
#22714=ORIENTED_EDGE('',*,*,#17836,.T.);
#22715=ORIENTED_EDGE('',*,*,#17837,.F.);
#22716=ORIENTED_EDGE('',*,*,#17838,.T.);
#22717=ORIENTED_EDGE('',*,*,#17839,.F.);
#22718=ORIENTED_EDGE('',*,*,#17840,.T.);
#22719=ORIENTED_EDGE('',*,*,#17841,.F.);
#22720=ORIENTED_EDGE('',*,*,#17842,.T.);
#22721=ORIENTED_EDGE('',*,*,#17843,.F.);
#22722=ORIENTED_EDGE('',*,*,#17844,.T.);
#22723=ORIENTED_EDGE('',*,*,#17845,.F.);
#22724=ORIENTED_EDGE('',*,*,#17846,.T.);
#22725=ORIENTED_EDGE('',*,*,#17847,.F.);
#22726=ORIENTED_EDGE('',*,*,#17848,.T.);
#22727=ORIENTED_EDGE('',*,*,#17849,.F.);
#22728=ORIENTED_EDGE('',*,*,#17850,.T.);
#22729=ORIENTED_EDGE('',*,*,#17851,.F.);
#22730=ORIENTED_EDGE('',*,*,#17852,.T.);
#22731=ORIENTED_EDGE('',*,*,#17853,.F.);
#22732=ORIENTED_EDGE('',*,*,#17854,.T.);
#22733=ORIENTED_EDGE('',*,*,#17855,.F.);
#22734=ORIENTED_EDGE('',*,*,#17856,.T.);
#22735=ORIENTED_EDGE('',*,*,#17857,.F.);
#22736=ORIENTED_EDGE('',*,*,#17858,.T.);
#22737=ORIENTED_EDGE('',*,*,#17859,.F.);
#22738=ORIENTED_EDGE('',*,*,#17860,.T.);
#22739=ORIENTED_EDGE('',*,*,#17861,.F.);
#22740=ORIENTED_EDGE('',*,*,#17862,.T.);
#22741=ORIENTED_EDGE('',*,*,#17863,.F.);
#22742=ORIENTED_EDGE('',*,*,#17864,.T.);
#22743=ORIENTED_EDGE('',*,*,#17865,.F.);
#22744=ORIENTED_EDGE('',*,*,#17866,.T.);
#22745=ORIENTED_EDGE('',*,*,#17867,.F.);
#22746=ORIENTED_EDGE('',*,*,#17868,.T.);
#22747=ORIENTED_EDGE('',*,*,#17869,.F.);
#22748=ORIENTED_EDGE('',*,*,#17870,.T.);
#22749=ORIENTED_EDGE('',*,*,#17871,.F.);
#22750=ORIENTED_EDGE('',*,*,#17872,.T.);
#22751=ORIENTED_EDGE('',*,*,#17873,.F.);
#22752=ORIENTED_EDGE('',*,*,#17874,.T.);
#22753=ORIENTED_EDGE('',*,*,#17875,.F.);
#22754=ORIENTED_EDGE('',*,*,#17876,.T.);
#22755=ORIENTED_EDGE('',*,*,#17877,.F.);
#22756=ORIENTED_EDGE('',*,*,#17878,.T.);
#22757=ORIENTED_EDGE('',*,*,#17879,.F.);
#22758=ORIENTED_EDGE('',*,*,#17880,.T.);
#22759=ORIENTED_EDGE('',*,*,#17881,.F.);
#22760=ORIENTED_EDGE('',*,*,#17882,.T.);
#22761=ORIENTED_EDGE('',*,*,#17883,.F.);
#22762=ORIENTED_EDGE('',*,*,#17884,.T.);
#22763=ORIENTED_EDGE('',*,*,#17885,.F.);
#22764=ORIENTED_EDGE('',*,*,#17886,.T.);
#22765=ORIENTED_EDGE('',*,*,#17887,.F.);
#22766=ORIENTED_EDGE('',*,*,#17888,.T.);
#22767=ORIENTED_EDGE('',*,*,#17889,.F.);
#22768=ORIENTED_EDGE('',*,*,#17890,.T.);
#22769=ORIENTED_EDGE('',*,*,#17891,.F.);
#22770=ORIENTED_EDGE('',*,*,#17892,.T.);
#22771=ORIENTED_EDGE('',*,*,#17893,.F.);
#22772=ORIENTED_EDGE('',*,*,#17894,.T.);
#22773=ORIENTED_EDGE('',*,*,#17895,.F.);
#22774=ORIENTED_EDGE('',*,*,#17896,.T.);
#22775=ORIENTED_EDGE('',*,*,#17897,.F.);
#22776=ORIENTED_EDGE('',*,*,#17898,.T.);
#22777=ORIENTED_EDGE('',*,*,#17899,.F.);
#22778=ORIENTED_EDGE('',*,*,#17900,.T.);
#22779=ORIENTED_EDGE('',*,*,#17901,.F.);
#22780=ORIENTED_EDGE('',*,*,#17902,.T.);
#22781=ORIENTED_EDGE('',*,*,#17903,.F.);
#22782=ORIENTED_EDGE('',*,*,#17904,.T.);
#22783=ORIENTED_EDGE('',*,*,#17905,.F.);
#22784=ORIENTED_EDGE('',*,*,#17906,.T.);
#22785=ORIENTED_EDGE('',*,*,#17907,.F.);
#22786=ORIENTED_EDGE('',*,*,#17908,.T.);
#22787=ORIENTED_EDGE('',*,*,#17909,.F.);
#22788=ORIENTED_EDGE('',*,*,#17910,.T.);
#22789=ORIENTED_EDGE('',*,*,#17911,.F.);
#22790=ORIENTED_EDGE('',*,*,#17912,.T.);
#22791=ORIENTED_EDGE('',*,*,#17913,.F.);
#22792=ORIENTED_EDGE('',*,*,#17914,.T.);
#22793=ORIENTED_EDGE('',*,*,#17915,.F.);
#22794=ORIENTED_EDGE('',*,*,#17916,.T.);
#22795=ORIENTED_EDGE('',*,*,#17917,.F.);
#22796=ORIENTED_EDGE('',*,*,#17918,.T.);
#22797=ORIENTED_EDGE('',*,*,#17919,.F.);
#22798=ORIENTED_EDGE('',*,*,#17920,.T.);
#22799=ORIENTED_EDGE('',*,*,#17921,.F.);
#22800=ORIENTED_EDGE('',*,*,#17922,.T.);
#22801=ORIENTED_EDGE('',*,*,#17923,.F.);
#22802=ORIENTED_EDGE('',*,*,#17924,.T.);
#22803=ORIENTED_EDGE('',*,*,#17925,.F.);
#22804=ORIENTED_EDGE('',*,*,#17926,.T.);
#22805=ORIENTED_EDGE('',*,*,#17927,.F.);
#22806=ORIENTED_EDGE('',*,*,#17928,.T.);
#22807=ORIENTED_EDGE('',*,*,#17929,.F.);
#22808=ORIENTED_EDGE('',*,*,#17930,.T.);
#22809=ORIENTED_EDGE('',*,*,#17931,.F.);
#22810=ORIENTED_EDGE('',*,*,#17932,.T.);
#22811=ORIENTED_EDGE('',*,*,#17933,.F.);
#22812=ORIENTED_EDGE('',*,*,#17934,.T.);
#22813=ORIENTED_EDGE('',*,*,#17935,.F.);
#22814=ORIENTED_EDGE('',*,*,#17936,.T.);
#22815=ORIENTED_EDGE('',*,*,#17937,.F.);
#22816=ORIENTED_EDGE('',*,*,#17938,.T.);
#22817=ORIENTED_EDGE('',*,*,#17939,.F.);
#22818=ORIENTED_EDGE('',*,*,#17940,.T.);
#22819=ORIENTED_EDGE('',*,*,#17941,.F.);
#22820=ORIENTED_EDGE('',*,*,#17942,.T.);
#22821=ORIENTED_EDGE('',*,*,#17943,.F.);
#22822=ORIENTED_EDGE('',*,*,#17944,.T.);
#22823=ORIENTED_EDGE('',*,*,#17945,.F.);
#22824=ORIENTED_EDGE('',*,*,#17946,.T.);
#22825=ORIENTED_EDGE('',*,*,#17947,.F.);
#22826=ORIENTED_EDGE('',*,*,#17948,.T.);
#22827=ORIENTED_EDGE('',*,*,#17949,.F.);
#22828=ORIENTED_EDGE('',*,*,#17950,.T.);
#22829=ORIENTED_EDGE('',*,*,#17951,.F.);
#22830=ORIENTED_EDGE('',*,*,#17952,.T.);
#22831=ORIENTED_EDGE('',*,*,#17953,.F.);
#22832=ORIENTED_EDGE('',*,*,#17954,.T.);
#22833=ORIENTED_EDGE('',*,*,#17955,.F.);
#22834=ORIENTED_EDGE('',*,*,#17956,.T.);
#22835=ORIENTED_EDGE('',*,*,#17957,.F.);
#22836=ORIENTED_EDGE('',*,*,#17958,.T.);
#22837=ORIENTED_EDGE('',*,*,#17959,.F.);
#22838=ORIENTED_EDGE('',*,*,#17960,.T.);
#22839=ORIENTED_EDGE('',*,*,#17961,.F.);
#22840=ORIENTED_EDGE('',*,*,#17962,.T.);
#22841=ORIENTED_EDGE('',*,*,#17963,.F.);
#22842=ORIENTED_EDGE('',*,*,#17964,.T.);
#22843=ORIENTED_EDGE('',*,*,#17965,.F.);
#22844=ORIENTED_EDGE('',*,*,#17966,.T.);
#22845=ORIENTED_EDGE('',*,*,#17967,.F.);
#22846=ORIENTED_EDGE('',*,*,#17968,.T.);
#22847=ORIENTED_EDGE('',*,*,#17969,.F.);
#22848=ORIENTED_EDGE('',*,*,#17970,.T.);
#22849=ORIENTED_EDGE('',*,*,#17971,.F.);
#22850=ORIENTED_EDGE('',*,*,#17972,.T.);
#22851=ORIENTED_EDGE('',*,*,#17973,.F.);
#22852=ORIENTED_EDGE('',*,*,#17974,.T.);
#22853=ORIENTED_EDGE('',*,*,#17975,.F.);
#22854=ORIENTED_EDGE('',*,*,#17976,.T.);
#22855=ORIENTED_EDGE('',*,*,#17977,.F.);
#22856=ORIENTED_EDGE('',*,*,#17978,.T.);
#22857=ORIENTED_EDGE('',*,*,#17979,.F.);
#22858=ORIENTED_EDGE('',*,*,#17980,.T.);
#22859=ORIENTED_EDGE('',*,*,#17981,.F.);
#22860=ORIENTED_EDGE('',*,*,#17982,.T.);
#22861=ORIENTED_EDGE('',*,*,#17983,.F.);
#22862=ORIENTED_EDGE('',*,*,#17984,.T.);
#22863=ORIENTED_EDGE('',*,*,#17985,.F.);
#22864=ORIENTED_EDGE('',*,*,#17986,.T.);
#22865=ORIENTED_EDGE('',*,*,#17987,.F.);
#22866=ORIENTED_EDGE('',*,*,#17988,.T.);
#22867=ORIENTED_EDGE('',*,*,#17989,.F.);
#22868=ORIENTED_EDGE('',*,*,#17990,.T.);
#22869=ORIENTED_EDGE('',*,*,#17991,.F.);
#22870=ORIENTED_EDGE('',*,*,#17992,.T.);
#22871=ORIENTED_EDGE('',*,*,#17993,.F.);
#22872=ORIENTED_EDGE('',*,*,#17994,.T.);
#22873=ORIENTED_EDGE('',*,*,#17995,.F.);
#22874=ORIENTED_EDGE('',*,*,#17996,.T.);
#22875=ORIENTED_EDGE('',*,*,#17997,.F.);
#22876=ORIENTED_EDGE('',*,*,#17998,.T.);
#22877=ORIENTED_EDGE('',*,*,#17999,.F.);
#22878=ORIENTED_EDGE('',*,*,#18000,.T.);
#22879=ORIENTED_EDGE('',*,*,#18001,.F.);
#22880=ORIENTED_EDGE('',*,*,#18002,.T.);
#22881=ORIENTED_EDGE('',*,*,#18003,.F.);
#22882=ORIENTED_EDGE('',*,*,#18004,.T.);
#22883=ORIENTED_EDGE('',*,*,#18005,.F.);
#22884=ORIENTED_EDGE('',*,*,#18006,.T.);
#22885=ORIENTED_EDGE('',*,*,#18007,.F.);
#22886=ORIENTED_EDGE('',*,*,#18008,.T.);
#22887=ORIENTED_EDGE('',*,*,#18009,.F.);
#22888=ORIENTED_EDGE('',*,*,#18010,.T.);
#22889=ORIENTED_EDGE('',*,*,#18011,.F.);
#22890=ORIENTED_EDGE('',*,*,#18012,.T.);
#22891=ORIENTED_EDGE('',*,*,#18013,.F.);
#22892=ORIENTED_EDGE('',*,*,#18014,.T.);
#22893=ORIENTED_EDGE('',*,*,#18015,.F.);
#22894=ORIENTED_EDGE('',*,*,#18016,.T.);
#22895=ORIENTED_EDGE('',*,*,#18017,.F.);
#22896=ORIENTED_EDGE('',*,*,#18018,.T.);
#22897=ORIENTED_EDGE('',*,*,#18019,.F.);
#22898=ORIENTED_EDGE('',*,*,#18020,.T.);
#22899=ORIENTED_EDGE('',*,*,#18021,.F.);
#22900=ORIENTED_EDGE('',*,*,#18022,.T.);
#22901=ORIENTED_EDGE('',*,*,#18023,.F.);
#22902=ORIENTED_EDGE('',*,*,#18024,.T.);
#22903=ORIENTED_EDGE('',*,*,#18025,.F.);
#22904=ORIENTED_EDGE('',*,*,#18026,.T.);
#22905=ORIENTED_EDGE('',*,*,#18027,.F.);
#22906=ORIENTED_EDGE('',*,*,#18028,.T.);
#22907=ORIENTED_EDGE('',*,*,#18029,.F.);
#22908=ORIENTED_EDGE('',*,*,#18030,.T.);
#22909=ORIENTED_EDGE('',*,*,#18031,.F.);
#22910=ORIENTED_EDGE('',*,*,#18032,.T.);
#22911=ORIENTED_EDGE('',*,*,#18033,.F.);
#22912=ORIENTED_EDGE('',*,*,#18034,.T.);
#22913=ORIENTED_EDGE('',*,*,#18035,.F.);
#22914=ORIENTED_EDGE('',*,*,#18036,.T.);
#22915=ORIENTED_EDGE('',*,*,#18037,.F.);
#22916=ORIENTED_EDGE('',*,*,#18038,.T.);
#22917=ORIENTED_EDGE('',*,*,#18039,.F.);
#22918=ORIENTED_EDGE('',*,*,#18040,.T.);
#22919=ORIENTED_EDGE('',*,*,#18041,.F.);
#22920=ORIENTED_EDGE('',*,*,#18042,.T.);
#22921=ORIENTED_EDGE('',*,*,#18043,.F.);
#22922=ORIENTED_EDGE('',*,*,#18044,.T.);
#22923=ORIENTED_EDGE('',*,*,#18045,.F.);
#22924=ORIENTED_EDGE('',*,*,#18046,.T.);
#22925=ORIENTED_EDGE('',*,*,#18047,.F.);
#22926=ORIENTED_EDGE('',*,*,#18048,.T.);
#22927=ORIENTED_EDGE('',*,*,#18049,.F.);
#22928=ORIENTED_EDGE('',*,*,#18050,.T.);
#22929=ORIENTED_EDGE('',*,*,#18051,.F.);
#22930=ORIENTED_EDGE('',*,*,#18052,.T.);
#22931=ORIENTED_EDGE('',*,*,#18053,.F.);
#22932=ORIENTED_EDGE('',*,*,#18054,.T.);
#22933=ORIENTED_EDGE('',*,*,#18055,.F.);
#22934=ORIENTED_EDGE('',*,*,#18056,.T.);
#22935=ORIENTED_EDGE('',*,*,#18057,.F.);
#22936=ORIENTED_EDGE('',*,*,#18058,.T.);
#22937=ORIENTED_EDGE('',*,*,#18059,.F.);
#22938=ORIENTED_EDGE('',*,*,#18060,.T.);
#22939=ORIENTED_EDGE('',*,*,#18061,.F.);
#22940=ORIENTED_EDGE('',*,*,#18062,.T.);
#22941=ORIENTED_EDGE('',*,*,#18063,.F.);
#22942=ORIENTED_EDGE('',*,*,#18064,.T.);
#22943=ORIENTED_EDGE('',*,*,#18065,.F.);
#22944=ORIENTED_EDGE('',*,*,#18066,.T.);
#22945=ORIENTED_EDGE('',*,*,#18067,.F.);
#22946=ORIENTED_EDGE('',*,*,#18068,.T.);
#22947=ORIENTED_EDGE('',*,*,#18069,.F.);
#22948=ORIENTED_EDGE('',*,*,#18070,.T.);
#22949=ORIENTED_EDGE('',*,*,#18071,.F.);
#22950=ORIENTED_EDGE('',*,*,#18072,.T.);
#22951=ORIENTED_EDGE('',*,*,#18073,.F.);
#22952=ORIENTED_EDGE('',*,*,#18074,.T.);
#22953=ORIENTED_EDGE('',*,*,#18075,.F.);
#22954=ORIENTED_EDGE('',*,*,#18076,.T.);
#22955=ORIENTED_EDGE('',*,*,#18077,.F.);
#22956=ORIENTED_EDGE('',*,*,#18078,.T.);
#22957=ORIENTED_EDGE('',*,*,#18079,.F.);
#22958=ORIENTED_EDGE('',*,*,#18080,.T.);
#22959=ORIENTED_EDGE('',*,*,#18081,.F.);
#22960=ORIENTED_EDGE('',*,*,#18082,.T.);
#22961=ORIENTED_EDGE('',*,*,#18083,.F.);
#22962=ORIENTED_EDGE('',*,*,#18084,.T.);
#22963=ORIENTED_EDGE('',*,*,#18085,.F.);
#22964=ORIENTED_EDGE('',*,*,#18086,.T.);
#22965=ORIENTED_EDGE('',*,*,#18087,.F.);
#22966=ORIENTED_EDGE('',*,*,#18088,.T.);
#22967=ORIENTED_EDGE('',*,*,#18089,.F.);
#22968=ORIENTED_EDGE('',*,*,#18090,.T.);
#22969=ORIENTED_EDGE('',*,*,#18091,.F.);
#22970=ORIENTED_EDGE('',*,*,#18092,.T.);
#22971=ORIENTED_EDGE('',*,*,#18093,.T.);
#22972=ORIENTED_EDGE('',*,*,#18094,.T.);
#22973=ORIENTED_EDGE('',*,*,#18095,.F.);
#22974=ORIENTED_EDGE('',*,*,#18096,.T.);
#22975=ORIENTED_EDGE('',*,*,#18097,.T.);
#22976=ORIENTED_EDGE('',*,*,#18098,.T.);
#22977=ORIENTED_EDGE('',*,*,#18093,.F.);
#22978=ORIENTED_EDGE('',*,*,#18099,.T.);
#22979=ORIENTED_EDGE('',*,*,#18100,.T.);
#22980=ORIENTED_EDGE('',*,*,#18101,.T.);
#22981=ORIENTED_EDGE('',*,*,#18097,.F.);
#22982=ORIENTED_EDGE('',*,*,#18102,.T.);
#22983=ORIENTED_EDGE('',*,*,#18103,.T.);
#22984=ORIENTED_EDGE('',*,*,#18104,.T.);
#22985=ORIENTED_EDGE('',*,*,#18100,.F.);
#22986=ORIENTED_EDGE('',*,*,#18105,.T.);
#22987=ORIENTED_EDGE('',*,*,#18106,.T.);
#22988=ORIENTED_EDGE('',*,*,#18107,.T.);
#22989=ORIENTED_EDGE('',*,*,#18103,.F.);
#22990=ORIENTED_EDGE('',*,*,#18108,.T.);
#22991=ORIENTED_EDGE('',*,*,#18109,.T.);
#22992=ORIENTED_EDGE('',*,*,#18110,.T.);
#22993=ORIENTED_EDGE('',*,*,#18106,.F.);
#22994=ORIENTED_EDGE('',*,*,#18111,.T.);
#22995=ORIENTED_EDGE('',*,*,#18109,.F.);
#22996=ORIENTED_EDGE('',*,*,#18112,.T.);
#22997=ORIENTED_EDGE('',*,*,#18113,.T.);
#22998=ORIENTED_EDGE('',*,*,#18114,.T.);
#22999=ORIENTED_EDGE('',*,*,#18113,.F.);
#23000=ORIENTED_EDGE('',*,*,#18115,.T.);
#23001=ORIENTED_EDGE('',*,*,#18116,.T.);
#23002=ORIENTED_EDGE('',*,*,#18117,.T.);
#23003=ORIENTED_EDGE('',*,*,#18116,.F.);
#23004=ORIENTED_EDGE('',*,*,#18118,.T.);
#23005=ORIENTED_EDGE('',*,*,#18119,.T.);
#23006=ORIENTED_EDGE('',*,*,#18120,.T.);
#23007=ORIENTED_EDGE('',*,*,#18119,.F.);
#23008=ORIENTED_EDGE('',*,*,#18121,.T.);
#23009=ORIENTED_EDGE('',*,*,#18095,.T.);
#23010=ORIENTED_EDGE('',*,*,#18110,.F.);
#23011=ORIENTED_EDGE('',*,*,#18122,.F.);
#23012=ORIENTED_EDGE('',*,*,#18123,.F.);
#23013=ORIENTED_EDGE('',*,*,#18124,.T.);
#23014=ORIENTED_EDGE('',*,*,#18111,.F.);
#23015=ORIENTED_EDGE('',*,*,#18125,.F.);
#23016=ORIENTED_EDGE('',*,*,#18126,.F.);
#23017=ORIENTED_EDGE('',*,*,#18122,.T.);
#23018=ORIENTED_EDGE('',*,*,#18114,.F.);
#23019=ORIENTED_EDGE('',*,*,#18127,.F.);
#23020=ORIENTED_EDGE('',*,*,#18128,.F.);
#23021=ORIENTED_EDGE('',*,*,#18125,.T.);
#23022=ORIENTED_EDGE('',*,*,#18117,.F.);
#23023=ORIENTED_EDGE('',*,*,#18129,.F.);
#23024=ORIENTED_EDGE('',*,*,#18130,.F.);
#23025=ORIENTED_EDGE('',*,*,#18127,.T.);
#23026=ORIENTED_EDGE('',*,*,#18120,.F.);
#23027=ORIENTED_EDGE('',*,*,#18131,.F.);
#23028=ORIENTED_EDGE('',*,*,#18132,.F.);
#23029=ORIENTED_EDGE('',*,*,#18129,.T.);
#23030=ORIENTED_EDGE('',*,*,#18094,.F.);
#23031=ORIENTED_EDGE('',*,*,#18133,.F.);
#23032=ORIENTED_EDGE('',*,*,#18134,.F.);
#23033=ORIENTED_EDGE('',*,*,#18131,.T.);
#23034=ORIENTED_EDGE('',*,*,#18108,.F.);
#23035=ORIENTED_EDGE('',*,*,#18105,.F.);
#23036=ORIENTED_EDGE('',*,*,#18102,.F.);
#23037=ORIENTED_EDGE('',*,*,#18099,.F.);
#23038=ORIENTED_EDGE('',*,*,#18096,.F.);
#23039=ORIENTED_EDGE('',*,*,#18092,.F.);
#23040=ORIENTED_EDGE('',*,*,#18121,.F.);
#23041=ORIENTED_EDGE('',*,*,#18118,.F.);
#23042=ORIENTED_EDGE('',*,*,#18115,.F.);
#23043=ORIENTED_EDGE('',*,*,#18112,.F.);
#23044=ORIENTED_EDGE('',*,*,#18135,.T.);
#23045=ORIENTED_EDGE('',*,*,#18136,.T.);
#23046=ORIENTED_EDGE('',*,*,#18137,.T.);
#23047=ORIENTED_EDGE('',*,*,#18138,.T.);
#23048=ORIENTED_EDGE('',*,*,#18139,.T.);
#23049=ORIENTED_EDGE('',*,*,#17485,.F.);
#23050=ORIENTED_EDGE('',*,*,#18140,.T.);
#23051=ORIENTED_EDGE('',*,*,#18141,.T.);
#23052=ORIENTED_EDGE('',*,*,#17529,.T.);
#23053=ORIENTED_EDGE('',*,*,#18142,.T.);
#23054=ORIENTED_EDGE('',*,*,#18143,.T.);
#23055=ORIENTED_EDGE('',*,*,#18141,.F.);
#23056=ORIENTED_EDGE('',*,*,#18144,.F.);
#23057=ORIENTED_EDGE('',*,*,#18145,.F.);
#23058=ORIENTED_EDGE('',*,*,#17530,.F.);
#23059=ORIENTED_EDGE('',*,*,#18140,.F.);
#23060=ORIENTED_EDGE('',*,*,#18146,.F.);
#23061=ORIENTED_EDGE('',*,*,#18147,.T.);
#23062=ORIENTED_EDGE('',*,*,#18148,.T.);
#23063=ORIENTED_EDGE('',*,*,#18144,.T.);
#23064=ORIENTED_EDGE('',*,*,#18143,.F.);
#23065=ORIENTED_EDGE('',*,*,#18149,.T.);
#23066=ORIENTED_EDGE('',*,*,#18150,.T.);
#23067=ORIENTED_EDGE('',*,*,#18151,.T.);
#23068=ORIENTED_EDGE('',*,*,#18146,.T.);
#23069=ORIENTED_EDGE('',*,*,#18148,.F.);
#23070=ORIENTED_EDGE('',*,*,#18152,.F.);
#23071=ORIENTED_EDGE('',*,*,#18153,.F.);
#23072=ORIENTED_EDGE('',*,*,#18150,.F.);
#23073=ORIENTED_EDGE('',*,*,#18154,.F.);
#23074=ORIENTED_EDGE('',*,*,#18155,.F.);
#23075=ORIENTED_EDGE('',*,*,#17527,.T.);
#23076=ORIENTED_EDGE('',*,*,#18156,.T.);
#23077=ORIENTED_EDGE('',*,*,#18154,.T.);
#23078=ORIENTED_EDGE('',*,*,#18157,.T.);
#23079=ORIENTED_EDGE('',*,*,#18158,.F.);
#23080=ORIENTED_EDGE('',*,*,#18159,.F.);
#23081=ORIENTED_EDGE('',*,*,#18160,.F.);
#23082=ORIENTED_EDGE('',*,*,#17525,.T.);
#23083=ORIENTED_EDGE('',*,*,#18161,.T.);
#23084=ORIENTED_EDGE('',*,*,#18159,.T.);
#23085=ORIENTED_EDGE('',*,*,#18162,.T.);
#23086=ORIENTED_EDGE('',*,*,#18152,.T.);
#23087=ORIENTED_EDGE('',*,*,#18163,.T.);
#23088=ORIENTED_EDGE('',*,*,#18160,.T.);
#23089=ORIENTED_EDGE('',*,*,#18164,.T.);
#23090=ORIENTED_EDGE('',*,*,#18158,.T.);
#23091=ORIENTED_EDGE('',*,*,#18165,.T.);
#23092=ORIENTED_EDGE('',*,*,#18155,.T.);
#23093=ORIENTED_EDGE('',*,*,#18166,.T.);
#23094=ORIENTED_EDGE('',*,*,#17531,.T.);
#23095=ORIENTED_EDGE('',*,*,#18145,.T.);
#23096=ORIENTED_EDGE('',*,*,#18153,.T.);
#23097=ORIENTED_EDGE('',*,*,#18167,.T.);
#23098=ORIENTED_EDGE('',*,*,#18142,.F.);
#23099=ORIENTED_EDGE('',*,*,#17528,.F.);
#23100=ORIENTED_EDGE('',*,*,#18157,.F.);
#23101=ORIENTED_EDGE('',*,*,#18149,.F.);
#23102=ORIENTED_EDGE('',*,*,#18163,.F.);
#23103=ORIENTED_EDGE('',*,*,#18147,.F.);
#23104=ORIENTED_EDGE('',*,*,#18151,.F.);
#23105=ORIENTED_EDGE('',*,*,#18165,.F.);
#23106=ORIENTED_EDGE('',*,*,#18168,.F.);
#23107=ORIENTED_EDGE('',*,*,#18169,.F.);
#23108=ORIENTED_EDGE('',*,*,#18170,.F.);
#23109=ORIENTED_EDGE('',*,*,#18171,.F.);
#23110=ORIENTED_EDGE('',*,*,#18172,.F.);
#23111=ORIENTED_EDGE('',*,*,#18173,.F.);
#23112=ORIENTED_EDGE('',*,*,#18174,.F.);
#23113=ORIENTED_EDGE('',*,*,#18175,.F.);
#23114=ORIENTED_EDGE('',*,*,#18176,.F.);
#23115=ORIENTED_EDGE('',*,*,#17535,.T.);
#23116=ORIENTED_EDGE('',*,*,#18177,.T.);
#23117=ORIENTED_EDGE('',*,*,#18175,.T.);
#23118=ORIENTED_EDGE('',*,*,#18178,.T.);
#23119=ORIENTED_EDGE('',*,*,#18179,.F.);
#23120=ORIENTED_EDGE('',*,*,#18180,.F.);
#23121=ORIENTED_EDGE('',*,*,#18181,.F.);
#23122=ORIENTED_EDGE('',*,*,#17533,.T.);
#23123=ORIENTED_EDGE('',*,*,#18182,.T.);
#23124=ORIENTED_EDGE('',*,*,#18180,.T.);
#23125=ORIENTED_EDGE('',*,*,#18183,.T.);
#23126=ORIENTED_EDGE('',*,*,#18172,.T.);
#23127=ORIENTED_EDGE('',*,*,#18184,.T.);
#23128=ORIENTED_EDGE('',*,*,#18181,.T.);
#23129=ORIENTED_EDGE('',*,*,#18185,.T.);
#23130=ORIENTED_EDGE('',*,*,#18179,.T.);
#23131=ORIENTED_EDGE('',*,*,#18186,.T.);
#23132=ORIENTED_EDGE('',*,*,#18176,.T.);
#23133=ORIENTED_EDGE('',*,*,#18187,.T.);
#23134=ORIENTED_EDGE('',*,*,#18169,.T.);
#23135=ORIENTED_EDGE('',*,*,#18188,.T.);
#23136=ORIENTED_EDGE('',*,*,#18174,.T.);
#23137=ORIENTED_EDGE('',*,*,#18189,.T.);
#23138=ORIENTED_EDGE('',*,*,#17539,.T.);
#23139=ORIENTED_EDGE('',*,*,#18190,.T.);
#23140=ORIENTED_EDGE('',*,*,#18173,.T.);
#23141=ORIENTED_EDGE('',*,*,#18191,.T.);
#23142=ORIENTED_EDGE('',*,*,#18171,.T.);
#23143=ORIENTED_EDGE('',*,*,#18192,.T.);
#23144=ORIENTED_EDGE('',*,*,#18170,.T.);
#23145=ORIENTED_EDGE('',*,*,#18193,.T.);
#23146=ORIENTED_EDGE('',*,*,#17537,.T.);
#23147=ORIENTED_EDGE('',*,*,#18194,.T.);
#23148=ORIENTED_EDGE('',*,*,#18168,.T.);
#23149=ORIENTED_EDGE('',*,*,#18195,.T.);
#23150=ORIENTED_EDGE('',*,*,#18183,.F.);
#23151=ORIENTED_EDGE('',*,*,#18187,.F.);
#23152=ORIENTED_EDGE('',*,*,#18177,.F.);
#23153=ORIENTED_EDGE('',*,*,#17534,.F.);
#23154=ORIENTED_EDGE('',*,*,#18178,.F.);
#23155=ORIENTED_EDGE('',*,*,#18188,.F.);
#23156=ORIENTED_EDGE('',*,*,#18194,.F.);
#23157=ORIENTED_EDGE('',*,*,#17536,.F.);
#23158=ORIENTED_EDGE('',*,*,#18184,.F.);
#23159=ORIENTED_EDGE('',*,*,#18193,.F.);
#23160=ORIENTED_EDGE('',*,*,#18189,.F.);
#23161=ORIENTED_EDGE('',*,*,#18186,.F.);
#23162=ORIENTED_EDGE('',*,*,#18196,.F.);
#23163=ORIENTED_EDGE('',*,*,#18197,.F.);
#23164=ORIENTED_EDGE('',*,*,#18198,.F.);
#23165=ORIENTED_EDGE('',*,*,#18199,.T.);
#23166=ORIENTED_EDGE('',*,*,#18200,.T.);
#23167=ORIENTED_EDGE('',*,*,#18197,.T.);
#23168=ORIENTED_EDGE('',*,*,#18201,.T.);
#23169=ORIENTED_EDGE('',*,*,#18202,.T.);
#23170=ORIENTED_EDGE('',*,*,#17547,.T.);
#23171=ORIENTED_EDGE('',*,*,#18203,.T.);
#23172=ORIENTED_EDGE('',*,*,#18198,.T.);
#23173=ORIENTED_EDGE('',*,*,#18204,.T.);
#23174=ORIENTED_EDGE('',*,*,#18205,.F.);
#23175=ORIENTED_EDGE('',*,*,#18206,.F.);
#23176=ORIENTED_EDGE('',*,*,#18207,.F.);
#23177=ORIENTED_EDGE('',*,*,#18208,.T.);
#23178=ORIENTED_EDGE('',*,*,#18209,.T.);
#23179=ORIENTED_EDGE('',*,*,#18206,.T.);
#23180=ORIENTED_EDGE('',*,*,#18210,.T.);
#23181=ORIENTED_EDGE('',*,*,#18211,.T.);
#23182=ORIENTED_EDGE('',*,*,#18196,.T.);
#23183=ORIENTED_EDGE('',*,*,#18212,.T.);
#23184=ORIENTED_EDGE('',*,*,#18207,.T.);
#23185=ORIENTED_EDGE('',*,*,#18213,.T.);
#23186=ORIENTED_EDGE('',*,*,#17545,.T.);
#23187=ORIENTED_EDGE('',*,*,#18214,.T.);
#23188=ORIENTED_EDGE('',*,*,#18205,.T.);
#23189=ORIENTED_EDGE('',*,*,#18215,.T.);
#23190=ORIENTED_EDGE('',*,*,#18199,.F.);
#23191=ORIENTED_EDGE('',*,*,#18216,.T.);
#23192=ORIENTED_EDGE('',*,*,#18217,.T.);
#23193=ORIENTED_EDGE('',*,*,#17541,.T.);
#23194=ORIENTED_EDGE('',*,*,#18218,.T.);
#23195=ORIENTED_EDGE('',*,*,#18201,.F.);
#23196=ORIENTED_EDGE('',*,*,#18213,.F.);
#23197=ORIENTED_EDGE('',*,*,#18209,.F.);
#23198=ORIENTED_EDGE('',*,*,#18219,.F.);
#23199=ORIENTED_EDGE('',*,*,#18202,.F.);
#23200=ORIENTED_EDGE('',*,*,#18219,.T.);
#23201=ORIENTED_EDGE('',*,*,#18208,.F.);
#23202=ORIENTED_EDGE('',*,*,#18220,.F.);
#23203=ORIENTED_EDGE('',*,*,#18221,.T.);
#23204=ORIENTED_EDGE('',*,*,#18216,.F.);
#23205=ORIENTED_EDGE('',*,*,#18211,.F.);
#23206=ORIENTED_EDGE('',*,*,#18222,.T.);
#23207=ORIENTED_EDGE('',*,*,#17543,.T.);
#23208=ORIENTED_EDGE('',*,*,#18223,.T.);
#23209=ORIENTED_EDGE('',*,*,#18220,.T.);
#23210=ORIENTED_EDGE('',*,*,#18210,.F.);
#23211=ORIENTED_EDGE('',*,*,#18214,.F.);
#23212=ORIENTED_EDGE('',*,*,#17544,.F.);
#23213=ORIENTED_EDGE('',*,*,#18222,.F.);
#23214=ORIENTED_EDGE('',*,*,#18200,.F.);
#23215=ORIENTED_EDGE('',*,*,#18218,.F.);
#23216=ORIENTED_EDGE('',*,*,#17540,.F.);
#23217=ORIENTED_EDGE('',*,*,#18204,.F.);
#23218=ORIENTED_EDGE('',*,*,#18224,.F.);
#23219=ORIENTED_EDGE('',*,*,#18225,.F.);
#23220=ORIENTED_EDGE('',*,*,#18226,.F.);
#23221=ORIENTED_EDGE('',*,*,#18227,.F.);
#23222=ORIENTED_EDGE('',*,*,#18228,.F.);
#23223=ORIENTED_EDGE('',*,*,#18229,.F.);
#23224=ORIENTED_EDGE('',*,*,#18230,.F.);
#23225=ORIENTED_EDGE('',*,*,#18231,.F.);
#23226=ORIENTED_EDGE('',*,*,#18232,.F.);
#23227=ORIENTED_EDGE('',*,*,#17551,.T.);
#23228=ORIENTED_EDGE('',*,*,#18233,.T.);
#23229=ORIENTED_EDGE('',*,*,#18231,.T.);
#23230=ORIENTED_EDGE('',*,*,#18234,.T.);
#23231=ORIENTED_EDGE('',*,*,#18235,.F.);
#23232=ORIENTED_EDGE('',*,*,#18236,.F.);
#23233=ORIENTED_EDGE('',*,*,#18237,.F.);
#23234=ORIENTED_EDGE('',*,*,#17549,.T.);
#23235=ORIENTED_EDGE('',*,*,#18238,.T.);
#23236=ORIENTED_EDGE('',*,*,#18236,.T.);
#23237=ORIENTED_EDGE('',*,*,#18239,.T.);
#23238=ORIENTED_EDGE('',*,*,#18228,.T.);
#23239=ORIENTED_EDGE('',*,*,#18240,.T.);
#23240=ORIENTED_EDGE('',*,*,#18237,.T.);
#23241=ORIENTED_EDGE('',*,*,#18241,.T.);
#23242=ORIENTED_EDGE('',*,*,#18235,.T.);
#23243=ORIENTED_EDGE('',*,*,#18242,.T.);
#23244=ORIENTED_EDGE('',*,*,#18232,.T.);
#23245=ORIENTED_EDGE('',*,*,#18243,.T.);
#23246=ORIENTED_EDGE('',*,*,#18225,.T.);
#23247=ORIENTED_EDGE('',*,*,#18244,.T.);
#23248=ORIENTED_EDGE('',*,*,#18230,.T.);
#23249=ORIENTED_EDGE('',*,*,#18245,.T.);
#23250=ORIENTED_EDGE('',*,*,#17555,.T.);
#23251=ORIENTED_EDGE('',*,*,#18246,.T.);
#23252=ORIENTED_EDGE('',*,*,#18229,.T.);
#23253=ORIENTED_EDGE('',*,*,#18247,.T.);
#23254=ORIENTED_EDGE('',*,*,#18227,.T.);
#23255=ORIENTED_EDGE('',*,*,#18248,.T.);
#23256=ORIENTED_EDGE('',*,*,#18226,.T.);
#23257=ORIENTED_EDGE('',*,*,#18249,.T.);
#23258=ORIENTED_EDGE('',*,*,#17553,.T.);
#23259=ORIENTED_EDGE('',*,*,#18250,.T.);
#23260=ORIENTED_EDGE('',*,*,#18224,.T.);
#23261=ORIENTED_EDGE('',*,*,#18251,.T.);
#23262=ORIENTED_EDGE('',*,*,#18239,.F.);
#23263=ORIENTED_EDGE('',*,*,#18243,.F.);
#23264=ORIENTED_EDGE('',*,*,#18233,.F.);
#23265=ORIENTED_EDGE('',*,*,#17550,.F.);
#23266=ORIENTED_EDGE('',*,*,#18234,.F.);
#23267=ORIENTED_EDGE('',*,*,#18244,.F.);
#23268=ORIENTED_EDGE('',*,*,#18250,.F.);
#23269=ORIENTED_EDGE('',*,*,#17552,.F.);
#23270=ORIENTED_EDGE('',*,*,#18240,.F.);
#23271=ORIENTED_EDGE('',*,*,#18249,.F.);
#23272=ORIENTED_EDGE('',*,*,#18245,.F.);
#23273=ORIENTED_EDGE('',*,*,#18242,.F.);
#23274=ORIENTED_EDGE('',*,*,#18252,.F.);
#23275=ORIENTED_EDGE('',*,*,#18253,.F.);
#23276=ORIENTED_EDGE('',*,*,#18254,.F.);
#23277=ORIENTED_EDGE('',*,*,#18255,.F.);
#23278=ORIENTED_EDGE('',*,*,#18256,.F.);
#23279=ORIENTED_EDGE('',*,*,#18257,.F.);
#23280=ORIENTED_EDGE('',*,*,#18258,.F.);
#23281=ORIENTED_EDGE('',*,*,#18259,.F.);
#23282=ORIENTED_EDGE('',*,*,#18260,.F.);
#23283=ORIENTED_EDGE('',*,*,#17559,.T.);
#23284=ORIENTED_EDGE('',*,*,#18261,.T.);
#23285=ORIENTED_EDGE('',*,*,#18259,.T.);
#23286=ORIENTED_EDGE('',*,*,#18262,.T.);
#23287=ORIENTED_EDGE('',*,*,#18263,.F.);
#23288=ORIENTED_EDGE('',*,*,#18264,.F.);
#23289=ORIENTED_EDGE('',*,*,#18265,.F.);
#23290=ORIENTED_EDGE('',*,*,#17557,.T.);
#23291=ORIENTED_EDGE('',*,*,#18266,.T.);
#23292=ORIENTED_EDGE('',*,*,#18264,.T.);
#23293=ORIENTED_EDGE('',*,*,#18267,.T.);
#23294=ORIENTED_EDGE('',*,*,#18256,.T.);
#23295=ORIENTED_EDGE('',*,*,#18268,.T.);
#23296=ORIENTED_EDGE('',*,*,#18265,.T.);
#23297=ORIENTED_EDGE('',*,*,#18269,.T.);
#23298=ORIENTED_EDGE('',*,*,#18263,.T.);
#23299=ORIENTED_EDGE('',*,*,#18270,.T.);
#23300=ORIENTED_EDGE('',*,*,#18260,.T.);
#23301=ORIENTED_EDGE('',*,*,#18271,.T.);
#23302=ORIENTED_EDGE('',*,*,#18253,.T.);
#23303=ORIENTED_EDGE('',*,*,#18272,.T.);
#23304=ORIENTED_EDGE('',*,*,#18258,.T.);
#23305=ORIENTED_EDGE('',*,*,#18273,.T.);
#23306=ORIENTED_EDGE('',*,*,#17563,.T.);
#23307=ORIENTED_EDGE('',*,*,#18274,.T.);
#23308=ORIENTED_EDGE('',*,*,#18257,.T.);
#23309=ORIENTED_EDGE('',*,*,#18275,.T.);
#23310=ORIENTED_EDGE('',*,*,#18255,.T.);
#23311=ORIENTED_EDGE('',*,*,#18276,.T.);
#23312=ORIENTED_EDGE('',*,*,#18254,.T.);
#23313=ORIENTED_EDGE('',*,*,#18277,.T.);
#23314=ORIENTED_EDGE('',*,*,#17561,.T.);
#23315=ORIENTED_EDGE('',*,*,#18278,.T.);
#23316=ORIENTED_EDGE('',*,*,#18252,.T.);
#23317=ORIENTED_EDGE('',*,*,#18279,.T.);
#23318=ORIENTED_EDGE('',*,*,#18267,.F.);
#23319=ORIENTED_EDGE('',*,*,#18271,.F.);
#23320=ORIENTED_EDGE('',*,*,#18261,.F.);
#23321=ORIENTED_EDGE('',*,*,#17558,.F.);
#23322=ORIENTED_EDGE('',*,*,#18262,.F.);
#23323=ORIENTED_EDGE('',*,*,#18272,.F.);
#23324=ORIENTED_EDGE('',*,*,#18278,.F.);
#23325=ORIENTED_EDGE('',*,*,#17560,.F.);
#23326=ORIENTED_EDGE('',*,*,#18268,.F.);
#23327=ORIENTED_EDGE('',*,*,#18277,.F.);
#23328=ORIENTED_EDGE('',*,*,#18273,.F.);
#23329=ORIENTED_EDGE('',*,*,#18270,.F.);
#23330=ORIENTED_EDGE('',*,*,#18280,.T.);
#23331=ORIENTED_EDGE('',*,*,#18281,.T.);
#23332=ORIENTED_EDGE('',*,*,#17569,.T.);
#23333=ORIENTED_EDGE('',*,*,#18282,.T.);
#23334=ORIENTED_EDGE('',*,*,#18283,.T.);
#23335=ORIENTED_EDGE('',*,*,#18281,.F.);
#23336=ORIENTED_EDGE('',*,*,#18284,.F.);
#23337=ORIENTED_EDGE('',*,*,#18285,.F.);
#23338=ORIENTED_EDGE('',*,*,#17570,.F.);
#23339=ORIENTED_EDGE('',*,*,#18280,.F.);
#23340=ORIENTED_EDGE('',*,*,#18286,.F.);
#23341=ORIENTED_EDGE('',*,*,#18287,.T.);
#23342=ORIENTED_EDGE('',*,*,#18288,.T.);
#23343=ORIENTED_EDGE('',*,*,#18284,.T.);
#23344=ORIENTED_EDGE('',*,*,#18283,.F.);
#23345=ORIENTED_EDGE('',*,*,#18289,.T.);
#23346=ORIENTED_EDGE('',*,*,#18290,.T.);
#23347=ORIENTED_EDGE('',*,*,#18291,.T.);
#23348=ORIENTED_EDGE('',*,*,#18286,.T.);
#23349=ORIENTED_EDGE('',*,*,#18288,.F.);
#23350=ORIENTED_EDGE('',*,*,#18292,.F.);
#23351=ORIENTED_EDGE('',*,*,#18293,.F.);
#23352=ORIENTED_EDGE('',*,*,#18290,.F.);
#23353=ORIENTED_EDGE('',*,*,#18294,.F.);
#23354=ORIENTED_EDGE('',*,*,#18295,.F.);
#23355=ORIENTED_EDGE('',*,*,#17567,.T.);
#23356=ORIENTED_EDGE('',*,*,#18296,.T.);
#23357=ORIENTED_EDGE('',*,*,#18294,.T.);
#23358=ORIENTED_EDGE('',*,*,#18297,.T.);
#23359=ORIENTED_EDGE('',*,*,#18298,.F.);
#23360=ORIENTED_EDGE('',*,*,#18299,.F.);
#23361=ORIENTED_EDGE('',*,*,#18300,.F.);
#23362=ORIENTED_EDGE('',*,*,#17565,.T.);
#23363=ORIENTED_EDGE('',*,*,#18301,.T.);
#23364=ORIENTED_EDGE('',*,*,#18299,.T.);
#23365=ORIENTED_EDGE('',*,*,#18302,.T.);
#23366=ORIENTED_EDGE('',*,*,#18292,.T.);
#23367=ORIENTED_EDGE('',*,*,#18303,.T.);
#23368=ORIENTED_EDGE('',*,*,#18300,.T.);
#23369=ORIENTED_EDGE('',*,*,#18304,.T.);
#23370=ORIENTED_EDGE('',*,*,#18298,.T.);
#23371=ORIENTED_EDGE('',*,*,#18305,.T.);
#23372=ORIENTED_EDGE('',*,*,#18295,.T.);
#23373=ORIENTED_EDGE('',*,*,#18306,.T.);
#23374=ORIENTED_EDGE('',*,*,#17571,.T.);
#23375=ORIENTED_EDGE('',*,*,#18285,.T.);
#23376=ORIENTED_EDGE('',*,*,#18293,.T.);
#23377=ORIENTED_EDGE('',*,*,#18307,.T.);
#23378=ORIENTED_EDGE('',*,*,#18282,.F.);
#23379=ORIENTED_EDGE('',*,*,#17568,.F.);
#23380=ORIENTED_EDGE('',*,*,#18297,.F.);
#23381=ORIENTED_EDGE('',*,*,#18289,.F.);
#23382=ORIENTED_EDGE('',*,*,#18303,.F.);
#23383=ORIENTED_EDGE('',*,*,#18287,.F.);
#23384=ORIENTED_EDGE('',*,*,#18291,.F.);
#23385=ORIENTED_EDGE('',*,*,#18305,.F.);
#23386=ORIENTED_EDGE('',*,*,#18308,.F.);
#23387=ORIENTED_EDGE('',*,*,#18309,.F.);
#23388=ORIENTED_EDGE('',*,*,#18310,.F.);
#23389=ORIENTED_EDGE('',*,*,#18311,.F.);
#23390=ORIENTED_EDGE('',*,*,#18312,.F.);
#23391=ORIENTED_EDGE('',*,*,#18313,.F.);
#23392=ORIENTED_EDGE('',*,*,#18314,.F.);
#23393=ORIENTED_EDGE('',*,*,#18315,.F.);
#23394=ORIENTED_EDGE('',*,*,#18316,.F.);
#23395=ORIENTED_EDGE('',*,*,#17575,.T.);
#23396=ORIENTED_EDGE('',*,*,#18317,.T.);
#23397=ORIENTED_EDGE('',*,*,#18315,.T.);
#23398=ORIENTED_EDGE('',*,*,#18318,.T.);
#23399=ORIENTED_EDGE('',*,*,#18319,.F.);
#23400=ORIENTED_EDGE('',*,*,#18320,.F.);
#23401=ORIENTED_EDGE('',*,*,#18321,.F.);
#23402=ORIENTED_EDGE('',*,*,#17573,.T.);
#23403=ORIENTED_EDGE('',*,*,#18322,.T.);
#23404=ORIENTED_EDGE('',*,*,#18320,.T.);
#23405=ORIENTED_EDGE('',*,*,#18323,.T.);
#23406=ORIENTED_EDGE('',*,*,#18312,.T.);
#23407=ORIENTED_EDGE('',*,*,#18324,.T.);
#23408=ORIENTED_EDGE('',*,*,#18321,.T.);
#23409=ORIENTED_EDGE('',*,*,#18325,.T.);
#23410=ORIENTED_EDGE('',*,*,#18319,.T.);
#23411=ORIENTED_EDGE('',*,*,#18326,.T.);
#23412=ORIENTED_EDGE('',*,*,#18316,.T.);
#23413=ORIENTED_EDGE('',*,*,#18327,.T.);
#23414=ORIENTED_EDGE('',*,*,#18309,.T.);
#23415=ORIENTED_EDGE('',*,*,#18328,.T.);
#23416=ORIENTED_EDGE('',*,*,#18314,.T.);
#23417=ORIENTED_EDGE('',*,*,#18329,.T.);
#23418=ORIENTED_EDGE('',*,*,#17579,.T.);
#23419=ORIENTED_EDGE('',*,*,#18330,.T.);
#23420=ORIENTED_EDGE('',*,*,#18313,.T.);
#23421=ORIENTED_EDGE('',*,*,#18331,.T.);
#23422=ORIENTED_EDGE('',*,*,#18311,.T.);
#23423=ORIENTED_EDGE('',*,*,#18332,.T.);
#23424=ORIENTED_EDGE('',*,*,#18310,.T.);
#23425=ORIENTED_EDGE('',*,*,#18333,.T.);
#23426=ORIENTED_EDGE('',*,*,#17577,.T.);
#23427=ORIENTED_EDGE('',*,*,#18334,.T.);
#23428=ORIENTED_EDGE('',*,*,#18308,.T.);
#23429=ORIENTED_EDGE('',*,*,#18335,.T.);
#23430=ORIENTED_EDGE('',*,*,#18323,.F.);
#23431=ORIENTED_EDGE('',*,*,#18327,.F.);
#23432=ORIENTED_EDGE('',*,*,#18317,.F.);
#23433=ORIENTED_EDGE('',*,*,#17574,.F.);
#23434=ORIENTED_EDGE('',*,*,#18318,.F.);
#23435=ORIENTED_EDGE('',*,*,#18328,.F.);
#23436=ORIENTED_EDGE('',*,*,#18334,.F.);
#23437=ORIENTED_EDGE('',*,*,#17576,.F.);
#23438=ORIENTED_EDGE('',*,*,#18324,.F.);
#23439=ORIENTED_EDGE('',*,*,#18333,.F.);
#23440=ORIENTED_EDGE('',*,*,#18329,.F.);
#23441=ORIENTED_EDGE('',*,*,#18326,.F.);
#23442=ORIENTED_EDGE('',*,*,#18336,.F.);
#23443=ORIENTED_EDGE('',*,*,#18337,.F.);
#23444=ORIENTED_EDGE('',*,*,#18338,.F.);
#23445=ORIENTED_EDGE('',*,*,#18339,.T.);
#23446=ORIENTED_EDGE('',*,*,#18340,.T.);
#23447=ORIENTED_EDGE('',*,*,#18337,.T.);
#23448=ORIENTED_EDGE('',*,*,#18341,.T.);
#23449=ORIENTED_EDGE('',*,*,#18342,.T.);
#23450=ORIENTED_EDGE('',*,*,#17587,.T.);
#23451=ORIENTED_EDGE('',*,*,#18343,.T.);
#23452=ORIENTED_EDGE('',*,*,#18338,.T.);
#23453=ORIENTED_EDGE('',*,*,#18344,.T.);
#23454=ORIENTED_EDGE('',*,*,#18345,.F.);
#23455=ORIENTED_EDGE('',*,*,#18346,.F.);
#23456=ORIENTED_EDGE('',*,*,#18347,.F.);
#23457=ORIENTED_EDGE('',*,*,#18348,.T.);
#23458=ORIENTED_EDGE('',*,*,#18349,.T.);
#23459=ORIENTED_EDGE('',*,*,#18346,.T.);
#23460=ORIENTED_EDGE('',*,*,#18350,.T.);
#23461=ORIENTED_EDGE('',*,*,#18351,.T.);
#23462=ORIENTED_EDGE('',*,*,#18336,.T.);
#23463=ORIENTED_EDGE('',*,*,#18352,.T.);
#23464=ORIENTED_EDGE('',*,*,#18347,.T.);
#23465=ORIENTED_EDGE('',*,*,#18353,.T.);
#23466=ORIENTED_EDGE('',*,*,#17585,.T.);
#23467=ORIENTED_EDGE('',*,*,#18354,.T.);
#23468=ORIENTED_EDGE('',*,*,#18345,.T.);
#23469=ORIENTED_EDGE('',*,*,#18355,.T.);
#23470=ORIENTED_EDGE('',*,*,#18339,.F.);
#23471=ORIENTED_EDGE('',*,*,#18356,.T.);
#23472=ORIENTED_EDGE('',*,*,#18357,.T.);
#23473=ORIENTED_EDGE('',*,*,#17581,.T.);
#23474=ORIENTED_EDGE('',*,*,#18358,.T.);
#23475=ORIENTED_EDGE('',*,*,#18341,.F.);
#23476=ORIENTED_EDGE('',*,*,#18353,.F.);
#23477=ORIENTED_EDGE('',*,*,#18349,.F.);
#23478=ORIENTED_EDGE('',*,*,#18359,.F.);
#23479=ORIENTED_EDGE('',*,*,#18342,.F.);
#23480=ORIENTED_EDGE('',*,*,#18359,.T.);
#23481=ORIENTED_EDGE('',*,*,#18348,.F.);
#23482=ORIENTED_EDGE('',*,*,#18360,.F.);
#23483=ORIENTED_EDGE('',*,*,#18361,.T.);
#23484=ORIENTED_EDGE('',*,*,#18356,.F.);
#23485=ORIENTED_EDGE('',*,*,#18351,.F.);
#23486=ORIENTED_EDGE('',*,*,#18362,.T.);
#23487=ORIENTED_EDGE('',*,*,#17583,.T.);
#23488=ORIENTED_EDGE('',*,*,#18363,.T.);
#23489=ORIENTED_EDGE('',*,*,#18360,.T.);
#23490=ORIENTED_EDGE('',*,*,#18350,.F.);
#23491=ORIENTED_EDGE('',*,*,#18354,.F.);
#23492=ORIENTED_EDGE('',*,*,#17584,.F.);
#23493=ORIENTED_EDGE('',*,*,#18362,.F.);
#23494=ORIENTED_EDGE('',*,*,#18340,.F.);
#23495=ORIENTED_EDGE('',*,*,#18358,.F.);
#23496=ORIENTED_EDGE('',*,*,#17580,.F.);
#23497=ORIENTED_EDGE('',*,*,#18344,.F.);
#23498=ORIENTED_EDGE('',*,*,#18364,.F.);
#23499=ORIENTED_EDGE('',*,*,#18365,.F.);
#23500=ORIENTED_EDGE('',*,*,#18366,.F.);
#23501=ORIENTED_EDGE('',*,*,#18367,.F.);
#23502=ORIENTED_EDGE('',*,*,#18368,.F.);
#23503=ORIENTED_EDGE('',*,*,#18369,.F.);
#23504=ORIENTED_EDGE('',*,*,#18370,.F.);
#23505=ORIENTED_EDGE('',*,*,#18371,.F.);
#23506=ORIENTED_EDGE('',*,*,#18372,.F.);
#23507=ORIENTED_EDGE('',*,*,#17591,.T.);
#23508=ORIENTED_EDGE('',*,*,#18373,.T.);
#23509=ORIENTED_EDGE('',*,*,#18371,.T.);
#23510=ORIENTED_EDGE('',*,*,#18374,.T.);
#23511=ORIENTED_EDGE('',*,*,#18375,.F.);
#23512=ORIENTED_EDGE('',*,*,#18376,.F.);
#23513=ORIENTED_EDGE('',*,*,#18377,.F.);
#23514=ORIENTED_EDGE('',*,*,#17589,.T.);
#23515=ORIENTED_EDGE('',*,*,#18378,.T.);
#23516=ORIENTED_EDGE('',*,*,#18376,.T.);
#23517=ORIENTED_EDGE('',*,*,#18379,.T.);
#23518=ORIENTED_EDGE('',*,*,#18368,.T.);
#23519=ORIENTED_EDGE('',*,*,#18380,.T.);
#23520=ORIENTED_EDGE('',*,*,#18377,.T.);
#23521=ORIENTED_EDGE('',*,*,#18381,.T.);
#23522=ORIENTED_EDGE('',*,*,#18375,.T.);
#23523=ORIENTED_EDGE('',*,*,#18382,.T.);
#23524=ORIENTED_EDGE('',*,*,#18372,.T.);
#23525=ORIENTED_EDGE('',*,*,#18383,.T.);
#23526=ORIENTED_EDGE('',*,*,#18365,.T.);
#23527=ORIENTED_EDGE('',*,*,#18384,.T.);
#23528=ORIENTED_EDGE('',*,*,#18370,.T.);
#23529=ORIENTED_EDGE('',*,*,#18385,.T.);
#23530=ORIENTED_EDGE('',*,*,#17595,.T.);
#23531=ORIENTED_EDGE('',*,*,#18386,.T.);
#23532=ORIENTED_EDGE('',*,*,#18369,.T.);
#23533=ORIENTED_EDGE('',*,*,#18387,.T.);
#23534=ORIENTED_EDGE('',*,*,#18367,.T.);
#23535=ORIENTED_EDGE('',*,*,#18388,.T.);
#23536=ORIENTED_EDGE('',*,*,#18366,.T.);
#23537=ORIENTED_EDGE('',*,*,#18389,.T.);
#23538=ORIENTED_EDGE('',*,*,#17593,.T.);
#23539=ORIENTED_EDGE('',*,*,#18390,.T.);
#23540=ORIENTED_EDGE('',*,*,#18364,.T.);
#23541=ORIENTED_EDGE('',*,*,#18391,.T.);
#23542=ORIENTED_EDGE('',*,*,#18379,.F.);
#23543=ORIENTED_EDGE('',*,*,#18383,.F.);
#23544=ORIENTED_EDGE('',*,*,#18373,.F.);
#23545=ORIENTED_EDGE('',*,*,#17590,.F.);
#23546=ORIENTED_EDGE('',*,*,#18374,.F.);
#23547=ORIENTED_EDGE('',*,*,#18384,.F.);
#23548=ORIENTED_EDGE('',*,*,#18390,.F.);
#23549=ORIENTED_EDGE('',*,*,#17592,.F.);
#23550=ORIENTED_EDGE('',*,*,#18380,.F.);
#23551=ORIENTED_EDGE('',*,*,#18389,.F.);
#23552=ORIENTED_EDGE('',*,*,#18385,.F.);
#23553=ORIENTED_EDGE('',*,*,#18382,.F.);
#23554=ORIENTED_EDGE('',*,*,#18392,.F.);
#23555=ORIENTED_EDGE('',*,*,#18393,.F.);
#23556=ORIENTED_EDGE('',*,*,#18394,.F.);
#23557=ORIENTED_EDGE('',*,*,#18395,.F.);
#23558=ORIENTED_EDGE('',*,*,#18396,.F.);
#23559=ORIENTED_EDGE('',*,*,#18397,.F.);
#23560=ORIENTED_EDGE('',*,*,#18398,.F.);
#23561=ORIENTED_EDGE('',*,*,#18399,.F.);
#23562=ORIENTED_EDGE('',*,*,#18400,.F.);
#23563=ORIENTED_EDGE('',*,*,#17599,.T.);
#23564=ORIENTED_EDGE('',*,*,#18401,.T.);
#23565=ORIENTED_EDGE('',*,*,#18399,.T.);
#23566=ORIENTED_EDGE('',*,*,#18402,.T.);
#23567=ORIENTED_EDGE('',*,*,#18403,.F.);
#23568=ORIENTED_EDGE('',*,*,#18404,.F.);
#23569=ORIENTED_EDGE('',*,*,#18405,.F.);
#23570=ORIENTED_EDGE('',*,*,#17597,.T.);
#23571=ORIENTED_EDGE('',*,*,#18406,.T.);
#23572=ORIENTED_EDGE('',*,*,#18404,.T.);
#23573=ORIENTED_EDGE('',*,*,#18407,.T.);
#23574=ORIENTED_EDGE('',*,*,#18396,.T.);
#23575=ORIENTED_EDGE('',*,*,#18408,.T.);
#23576=ORIENTED_EDGE('',*,*,#18405,.T.);
#23577=ORIENTED_EDGE('',*,*,#18409,.T.);
#23578=ORIENTED_EDGE('',*,*,#18403,.T.);
#23579=ORIENTED_EDGE('',*,*,#18410,.T.);
#23580=ORIENTED_EDGE('',*,*,#18400,.T.);
#23581=ORIENTED_EDGE('',*,*,#18411,.T.);
#23582=ORIENTED_EDGE('',*,*,#18393,.T.);
#23583=ORIENTED_EDGE('',*,*,#18412,.T.);
#23584=ORIENTED_EDGE('',*,*,#18398,.T.);
#23585=ORIENTED_EDGE('',*,*,#18413,.T.);
#23586=ORIENTED_EDGE('',*,*,#17603,.T.);
#23587=ORIENTED_EDGE('',*,*,#18414,.T.);
#23588=ORIENTED_EDGE('',*,*,#18397,.T.);
#23589=ORIENTED_EDGE('',*,*,#18415,.T.);
#23590=ORIENTED_EDGE('',*,*,#18395,.T.);
#23591=ORIENTED_EDGE('',*,*,#18416,.T.);
#23592=ORIENTED_EDGE('',*,*,#18394,.T.);
#23593=ORIENTED_EDGE('',*,*,#18417,.T.);
#23594=ORIENTED_EDGE('',*,*,#17601,.T.);
#23595=ORIENTED_EDGE('',*,*,#18418,.T.);
#23596=ORIENTED_EDGE('',*,*,#18392,.T.);
#23597=ORIENTED_EDGE('',*,*,#18419,.T.);
#23598=ORIENTED_EDGE('',*,*,#18407,.F.);
#23599=ORIENTED_EDGE('',*,*,#18411,.F.);
#23600=ORIENTED_EDGE('',*,*,#18401,.F.);
#23601=ORIENTED_EDGE('',*,*,#17598,.F.);
#23602=ORIENTED_EDGE('',*,*,#18402,.F.);
#23603=ORIENTED_EDGE('',*,*,#18412,.F.);
#23604=ORIENTED_EDGE('',*,*,#18418,.F.);
#23605=ORIENTED_EDGE('',*,*,#17600,.F.);
#23606=ORIENTED_EDGE('',*,*,#18408,.F.);
#23607=ORIENTED_EDGE('',*,*,#18417,.F.);
#23608=ORIENTED_EDGE('',*,*,#18413,.F.);
#23609=ORIENTED_EDGE('',*,*,#18410,.F.);
#23610=ORIENTED_EDGE('',*,*,#18420,.T.);
#23611=ORIENTED_EDGE('',*,*,#18421,.T.);
#23612=ORIENTED_EDGE('',*,*,#17609,.T.);
#23613=ORIENTED_EDGE('',*,*,#18422,.T.);
#23614=ORIENTED_EDGE('',*,*,#18423,.T.);
#23615=ORIENTED_EDGE('',*,*,#18421,.F.);
#23616=ORIENTED_EDGE('',*,*,#18424,.F.);
#23617=ORIENTED_EDGE('',*,*,#18425,.F.);
#23618=ORIENTED_EDGE('',*,*,#17610,.F.);
#23619=ORIENTED_EDGE('',*,*,#18420,.F.);
#23620=ORIENTED_EDGE('',*,*,#18426,.F.);
#23621=ORIENTED_EDGE('',*,*,#18427,.T.);
#23622=ORIENTED_EDGE('',*,*,#18428,.T.);
#23623=ORIENTED_EDGE('',*,*,#18424,.T.);
#23624=ORIENTED_EDGE('',*,*,#18423,.F.);
#23625=ORIENTED_EDGE('',*,*,#18429,.T.);
#23626=ORIENTED_EDGE('',*,*,#18430,.T.);
#23627=ORIENTED_EDGE('',*,*,#18431,.T.);
#23628=ORIENTED_EDGE('',*,*,#18426,.T.);
#23629=ORIENTED_EDGE('',*,*,#18428,.F.);
#23630=ORIENTED_EDGE('',*,*,#18432,.F.);
#23631=ORIENTED_EDGE('',*,*,#18433,.F.);
#23632=ORIENTED_EDGE('',*,*,#18430,.F.);
#23633=ORIENTED_EDGE('',*,*,#18434,.F.);
#23634=ORIENTED_EDGE('',*,*,#18435,.F.);
#23635=ORIENTED_EDGE('',*,*,#17607,.T.);
#23636=ORIENTED_EDGE('',*,*,#18436,.T.);
#23637=ORIENTED_EDGE('',*,*,#18434,.T.);
#23638=ORIENTED_EDGE('',*,*,#18437,.T.);
#23639=ORIENTED_EDGE('',*,*,#18438,.F.);
#23640=ORIENTED_EDGE('',*,*,#18439,.F.);
#23641=ORIENTED_EDGE('',*,*,#18440,.F.);
#23642=ORIENTED_EDGE('',*,*,#17605,.T.);
#23643=ORIENTED_EDGE('',*,*,#18441,.T.);
#23644=ORIENTED_EDGE('',*,*,#18439,.T.);
#23645=ORIENTED_EDGE('',*,*,#18442,.T.);
#23646=ORIENTED_EDGE('',*,*,#18432,.T.);
#23647=ORIENTED_EDGE('',*,*,#18443,.T.);
#23648=ORIENTED_EDGE('',*,*,#18440,.T.);
#23649=ORIENTED_EDGE('',*,*,#18444,.T.);
#23650=ORIENTED_EDGE('',*,*,#18438,.T.);
#23651=ORIENTED_EDGE('',*,*,#18445,.T.);
#23652=ORIENTED_EDGE('',*,*,#18435,.T.);
#23653=ORIENTED_EDGE('',*,*,#18446,.T.);
#23654=ORIENTED_EDGE('',*,*,#17611,.T.);
#23655=ORIENTED_EDGE('',*,*,#18425,.T.);
#23656=ORIENTED_EDGE('',*,*,#18433,.T.);
#23657=ORIENTED_EDGE('',*,*,#18447,.T.);
#23658=ORIENTED_EDGE('',*,*,#18422,.F.);
#23659=ORIENTED_EDGE('',*,*,#17608,.F.);
#23660=ORIENTED_EDGE('',*,*,#18437,.F.);
#23661=ORIENTED_EDGE('',*,*,#18429,.F.);
#23662=ORIENTED_EDGE('',*,*,#18443,.F.);
#23663=ORIENTED_EDGE('',*,*,#18427,.F.);
#23664=ORIENTED_EDGE('',*,*,#18431,.F.);
#23665=ORIENTED_EDGE('',*,*,#18445,.F.);
#23666=ORIENTED_EDGE('',*,*,#18448,.F.);
#23667=ORIENTED_EDGE('',*,*,#18449,.F.);
#23668=ORIENTED_EDGE('',*,*,#18450,.F.);
#23669=ORIENTED_EDGE('',*,*,#18451,.F.);
#23670=ORIENTED_EDGE('',*,*,#18452,.F.);
#23671=ORIENTED_EDGE('',*,*,#18453,.F.);
#23672=ORIENTED_EDGE('',*,*,#18454,.F.);
#23673=ORIENTED_EDGE('',*,*,#18455,.F.);
#23674=ORIENTED_EDGE('',*,*,#18456,.F.);
#23675=ORIENTED_EDGE('',*,*,#17615,.T.);
#23676=ORIENTED_EDGE('',*,*,#18457,.T.);
#23677=ORIENTED_EDGE('',*,*,#18455,.T.);
#23678=ORIENTED_EDGE('',*,*,#18458,.T.);
#23679=ORIENTED_EDGE('',*,*,#18459,.F.);
#23680=ORIENTED_EDGE('',*,*,#18460,.F.);
#23681=ORIENTED_EDGE('',*,*,#18461,.F.);
#23682=ORIENTED_EDGE('',*,*,#17613,.T.);
#23683=ORIENTED_EDGE('',*,*,#18462,.T.);
#23684=ORIENTED_EDGE('',*,*,#18460,.T.);
#23685=ORIENTED_EDGE('',*,*,#18463,.T.);
#23686=ORIENTED_EDGE('',*,*,#18452,.T.);
#23687=ORIENTED_EDGE('',*,*,#18464,.T.);
#23688=ORIENTED_EDGE('',*,*,#18461,.T.);
#23689=ORIENTED_EDGE('',*,*,#18465,.T.);
#23690=ORIENTED_EDGE('',*,*,#18459,.T.);
#23691=ORIENTED_EDGE('',*,*,#18466,.T.);
#23692=ORIENTED_EDGE('',*,*,#18456,.T.);
#23693=ORIENTED_EDGE('',*,*,#18467,.T.);
#23694=ORIENTED_EDGE('',*,*,#18449,.T.);
#23695=ORIENTED_EDGE('',*,*,#18468,.T.);
#23696=ORIENTED_EDGE('',*,*,#18454,.T.);
#23697=ORIENTED_EDGE('',*,*,#18469,.T.);
#23698=ORIENTED_EDGE('',*,*,#17619,.T.);
#23699=ORIENTED_EDGE('',*,*,#18470,.T.);
#23700=ORIENTED_EDGE('',*,*,#18453,.T.);
#23701=ORIENTED_EDGE('',*,*,#18471,.T.);
#23702=ORIENTED_EDGE('',*,*,#18451,.T.);
#23703=ORIENTED_EDGE('',*,*,#18472,.T.);
#23704=ORIENTED_EDGE('',*,*,#18450,.T.);
#23705=ORIENTED_EDGE('',*,*,#18473,.T.);
#23706=ORIENTED_EDGE('',*,*,#17617,.T.);
#23707=ORIENTED_EDGE('',*,*,#18474,.T.);
#23708=ORIENTED_EDGE('',*,*,#18448,.T.);
#23709=ORIENTED_EDGE('',*,*,#18475,.T.);
#23710=ORIENTED_EDGE('',*,*,#18463,.F.);
#23711=ORIENTED_EDGE('',*,*,#18467,.F.);
#23712=ORIENTED_EDGE('',*,*,#18457,.F.);
#23713=ORIENTED_EDGE('',*,*,#17614,.F.);
#23714=ORIENTED_EDGE('',*,*,#18458,.F.);
#23715=ORIENTED_EDGE('',*,*,#18468,.F.);
#23716=ORIENTED_EDGE('',*,*,#18474,.F.);
#23717=ORIENTED_EDGE('',*,*,#17616,.F.);
#23718=ORIENTED_EDGE('',*,*,#18464,.F.);
#23719=ORIENTED_EDGE('',*,*,#18473,.F.);
#23720=ORIENTED_EDGE('',*,*,#18469,.F.);
#23721=ORIENTED_EDGE('',*,*,#18466,.F.);
#23722=ORIENTED_EDGE('',*,*,#18476,.F.);
#23723=ORIENTED_EDGE('',*,*,#18477,.F.);
#23724=ORIENTED_EDGE('',*,*,#18478,.F.);
#23725=ORIENTED_EDGE('',*,*,#18479,.T.);
#23726=ORIENTED_EDGE('',*,*,#18480,.T.);
#23727=ORIENTED_EDGE('',*,*,#18477,.T.);
#23728=ORIENTED_EDGE('',*,*,#18481,.T.);
#23729=ORIENTED_EDGE('',*,*,#18482,.T.);
#23730=ORIENTED_EDGE('',*,*,#17627,.T.);
#23731=ORIENTED_EDGE('',*,*,#18483,.T.);
#23732=ORIENTED_EDGE('',*,*,#18478,.T.);
#23733=ORIENTED_EDGE('',*,*,#18484,.T.);
#23734=ORIENTED_EDGE('',*,*,#18485,.F.);
#23735=ORIENTED_EDGE('',*,*,#18486,.F.);
#23736=ORIENTED_EDGE('',*,*,#18487,.F.);
#23737=ORIENTED_EDGE('',*,*,#18488,.T.);
#23738=ORIENTED_EDGE('',*,*,#18489,.T.);
#23739=ORIENTED_EDGE('',*,*,#18486,.T.);
#23740=ORIENTED_EDGE('',*,*,#18490,.T.);
#23741=ORIENTED_EDGE('',*,*,#18491,.T.);
#23742=ORIENTED_EDGE('',*,*,#18476,.T.);
#23743=ORIENTED_EDGE('',*,*,#18492,.T.);
#23744=ORIENTED_EDGE('',*,*,#18487,.T.);
#23745=ORIENTED_EDGE('',*,*,#18493,.T.);
#23746=ORIENTED_EDGE('',*,*,#17625,.T.);
#23747=ORIENTED_EDGE('',*,*,#18494,.T.);
#23748=ORIENTED_EDGE('',*,*,#18485,.T.);
#23749=ORIENTED_EDGE('',*,*,#18495,.T.);
#23750=ORIENTED_EDGE('',*,*,#18479,.F.);
#23751=ORIENTED_EDGE('',*,*,#18496,.T.);
#23752=ORIENTED_EDGE('',*,*,#18497,.T.);
#23753=ORIENTED_EDGE('',*,*,#17621,.T.);
#23754=ORIENTED_EDGE('',*,*,#18498,.T.);
#23755=ORIENTED_EDGE('',*,*,#18481,.F.);
#23756=ORIENTED_EDGE('',*,*,#18493,.F.);
#23757=ORIENTED_EDGE('',*,*,#18489,.F.);
#23758=ORIENTED_EDGE('',*,*,#18499,.F.);
#23759=ORIENTED_EDGE('',*,*,#18482,.F.);
#23760=ORIENTED_EDGE('',*,*,#18499,.T.);
#23761=ORIENTED_EDGE('',*,*,#18488,.F.);
#23762=ORIENTED_EDGE('',*,*,#18500,.F.);
#23763=ORIENTED_EDGE('',*,*,#18501,.T.);
#23764=ORIENTED_EDGE('',*,*,#18496,.F.);
#23765=ORIENTED_EDGE('',*,*,#18491,.F.);
#23766=ORIENTED_EDGE('',*,*,#18502,.T.);
#23767=ORIENTED_EDGE('',*,*,#17623,.T.);
#23768=ORIENTED_EDGE('',*,*,#18503,.T.);
#23769=ORIENTED_EDGE('',*,*,#18500,.T.);
#23770=ORIENTED_EDGE('',*,*,#18490,.F.);
#23771=ORIENTED_EDGE('',*,*,#18494,.F.);
#23772=ORIENTED_EDGE('',*,*,#17624,.F.);
#23773=ORIENTED_EDGE('',*,*,#18502,.F.);
#23774=ORIENTED_EDGE('',*,*,#18480,.F.);
#23775=ORIENTED_EDGE('',*,*,#18498,.F.);
#23776=ORIENTED_EDGE('',*,*,#17620,.F.);
#23777=ORIENTED_EDGE('',*,*,#18484,.F.);
#23778=ORIENTED_EDGE('',*,*,#18504,.F.);
#23779=ORIENTED_EDGE('',*,*,#18505,.F.);
#23780=ORIENTED_EDGE('',*,*,#18506,.F.);
#23781=ORIENTED_EDGE('',*,*,#18507,.F.);
#23782=ORIENTED_EDGE('',*,*,#18508,.F.);
#23783=ORIENTED_EDGE('',*,*,#18509,.F.);
#23784=ORIENTED_EDGE('',*,*,#18510,.F.);
#23785=ORIENTED_EDGE('',*,*,#18511,.F.);
#23786=ORIENTED_EDGE('',*,*,#18512,.F.);
#23787=ORIENTED_EDGE('',*,*,#17631,.T.);
#23788=ORIENTED_EDGE('',*,*,#18513,.T.);
#23789=ORIENTED_EDGE('',*,*,#18511,.T.);
#23790=ORIENTED_EDGE('',*,*,#18514,.T.);
#23791=ORIENTED_EDGE('',*,*,#18515,.F.);
#23792=ORIENTED_EDGE('',*,*,#18516,.F.);
#23793=ORIENTED_EDGE('',*,*,#18517,.F.);
#23794=ORIENTED_EDGE('',*,*,#17629,.T.);
#23795=ORIENTED_EDGE('',*,*,#18518,.T.);
#23796=ORIENTED_EDGE('',*,*,#18516,.T.);
#23797=ORIENTED_EDGE('',*,*,#18519,.T.);
#23798=ORIENTED_EDGE('',*,*,#18508,.T.);
#23799=ORIENTED_EDGE('',*,*,#18520,.T.);
#23800=ORIENTED_EDGE('',*,*,#18517,.T.);
#23801=ORIENTED_EDGE('',*,*,#18521,.T.);
#23802=ORIENTED_EDGE('',*,*,#18515,.T.);
#23803=ORIENTED_EDGE('',*,*,#18522,.T.);
#23804=ORIENTED_EDGE('',*,*,#18512,.T.);
#23805=ORIENTED_EDGE('',*,*,#18523,.T.);
#23806=ORIENTED_EDGE('',*,*,#18505,.T.);
#23807=ORIENTED_EDGE('',*,*,#18524,.T.);
#23808=ORIENTED_EDGE('',*,*,#18510,.T.);
#23809=ORIENTED_EDGE('',*,*,#18525,.T.);
#23810=ORIENTED_EDGE('',*,*,#17635,.T.);
#23811=ORIENTED_EDGE('',*,*,#18526,.T.);
#23812=ORIENTED_EDGE('',*,*,#18509,.T.);
#23813=ORIENTED_EDGE('',*,*,#18527,.T.);
#23814=ORIENTED_EDGE('',*,*,#18507,.T.);
#23815=ORIENTED_EDGE('',*,*,#18528,.T.);
#23816=ORIENTED_EDGE('',*,*,#18506,.T.);
#23817=ORIENTED_EDGE('',*,*,#18529,.T.);
#23818=ORIENTED_EDGE('',*,*,#17633,.T.);
#23819=ORIENTED_EDGE('',*,*,#18530,.T.);
#23820=ORIENTED_EDGE('',*,*,#18504,.T.);
#23821=ORIENTED_EDGE('',*,*,#18531,.T.);
#23822=ORIENTED_EDGE('',*,*,#18519,.F.);
#23823=ORIENTED_EDGE('',*,*,#18523,.F.);
#23824=ORIENTED_EDGE('',*,*,#18513,.F.);
#23825=ORIENTED_EDGE('',*,*,#17630,.F.);
#23826=ORIENTED_EDGE('',*,*,#18514,.F.);
#23827=ORIENTED_EDGE('',*,*,#18524,.F.);
#23828=ORIENTED_EDGE('',*,*,#18530,.F.);
#23829=ORIENTED_EDGE('',*,*,#17632,.F.);
#23830=ORIENTED_EDGE('',*,*,#18520,.F.);
#23831=ORIENTED_EDGE('',*,*,#18529,.F.);
#23832=ORIENTED_EDGE('',*,*,#18525,.F.);
#23833=ORIENTED_EDGE('',*,*,#18522,.F.);
#23834=ORIENTED_EDGE('',*,*,#18532,.F.);
#23835=ORIENTED_EDGE('',*,*,#18533,.F.);
#23836=ORIENTED_EDGE('',*,*,#18534,.F.);
#23837=ORIENTED_EDGE('',*,*,#18535,.F.);
#23838=ORIENTED_EDGE('',*,*,#18536,.F.);
#23839=ORIENTED_EDGE('',*,*,#18537,.F.);
#23840=ORIENTED_EDGE('',*,*,#18538,.F.);
#23841=ORIENTED_EDGE('',*,*,#18539,.F.);
#23842=ORIENTED_EDGE('',*,*,#18540,.F.);
#23843=ORIENTED_EDGE('',*,*,#17639,.T.);
#23844=ORIENTED_EDGE('',*,*,#18541,.T.);
#23845=ORIENTED_EDGE('',*,*,#18539,.T.);
#23846=ORIENTED_EDGE('',*,*,#18542,.T.);
#23847=ORIENTED_EDGE('',*,*,#18543,.F.);
#23848=ORIENTED_EDGE('',*,*,#18544,.F.);
#23849=ORIENTED_EDGE('',*,*,#18545,.F.);
#23850=ORIENTED_EDGE('',*,*,#17637,.T.);
#23851=ORIENTED_EDGE('',*,*,#18546,.T.);
#23852=ORIENTED_EDGE('',*,*,#18544,.T.);
#23853=ORIENTED_EDGE('',*,*,#18547,.T.);
#23854=ORIENTED_EDGE('',*,*,#18536,.T.);
#23855=ORIENTED_EDGE('',*,*,#18548,.T.);
#23856=ORIENTED_EDGE('',*,*,#18545,.T.);
#23857=ORIENTED_EDGE('',*,*,#18549,.T.);
#23858=ORIENTED_EDGE('',*,*,#18543,.T.);
#23859=ORIENTED_EDGE('',*,*,#18550,.T.);
#23860=ORIENTED_EDGE('',*,*,#18540,.T.);
#23861=ORIENTED_EDGE('',*,*,#18551,.T.);
#23862=ORIENTED_EDGE('',*,*,#18533,.T.);
#23863=ORIENTED_EDGE('',*,*,#18552,.T.);
#23864=ORIENTED_EDGE('',*,*,#18538,.T.);
#23865=ORIENTED_EDGE('',*,*,#18553,.T.);
#23866=ORIENTED_EDGE('',*,*,#17643,.T.);
#23867=ORIENTED_EDGE('',*,*,#18554,.T.);
#23868=ORIENTED_EDGE('',*,*,#18537,.T.);
#23869=ORIENTED_EDGE('',*,*,#18555,.T.);
#23870=ORIENTED_EDGE('',*,*,#18535,.T.);
#23871=ORIENTED_EDGE('',*,*,#18556,.T.);
#23872=ORIENTED_EDGE('',*,*,#18534,.T.);
#23873=ORIENTED_EDGE('',*,*,#18557,.T.);
#23874=ORIENTED_EDGE('',*,*,#17641,.T.);
#23875=ORIENTED_EDGE('',*,*,#18558,.T.);
#23876=ORIENTED_EDGE('',*,*,#18532,.T.);
#23877=ORIENTED_EDGE('',*,*,#18559,.T.);
#23878=ORIENTED_EDGE('',*,*,#18547,.F.);
#23879=ORIENTED_EDGE('',*,*,#18551,.F.);
#23880=ORIENTED_EDGE('',*,*,#18541,.F.);
#23881=ORIENTED_EDGE('',*,*,#17638,.F.);
#23882=ORIENTED_EDGE('',*,*,#18542,.F.);
#23883=ORIENTED_EDGE('',*,*,#18552,.F.);
#23884=ORIENTED_EDGE('',*,*,#18558,.F.);
#23885=ORIENTED_EDGE('',*,*,#17640,.F.);
#23886=ORIENTED_EDGE('',*,*,#18548,.F.);
#23887=ORIENTED_EDGE('',*,*,#18557,.F.);
#23888=ORIENTED_EDGE('',*,*,#18553,.F.);
#23889=ORIENTED_EDGE('',*,*,#18550,.F.);
#23890=ORIENTED_EDGE('',*,*,#18560,.T.);
#23891=ORIENTED_EDGE('',*,*,#18561,.T.);
#23892=ORIENTED_EDGE('',*,*,#17649,.T.);
#23893=ORIENTED_EDGE('',*,*,#18562,.T.);
#23894=ORIENTED_EDGE('',*,*,#18563,.T.);
#23895=ORIENTED_EDGE('',*,*,#18561,.F.);
#23896=ORIENTED_EDGE('',*,*,#18564,.F.);
#23897=ORIENTED_EDGE('',*,*,#18565,.F.);
#23898=ORIENTED_EDGE('',*,*,#17650,.F.);
#23899=ORIENTED_EDGE('',*,*,#18560,.F.);
#23900=ORIENTED_EDGE('',*,*,#18566,.F.);
#23901=ORIENTED_EDGE('',*,*,#18567,.T.);
#23902=ORIENTED_EDGE('',*,*,#18568,.T.);
#23903=ORIENTED_EDGE('',*,*,#18564,.T.);
#23904=ORIENTED_EDGE('',*,*,#18563,.F.);
#23905=ORIENTED_EDGE('',*,*,#18569,.T.);
#23906=ORIENTED_EDGE('',*,*,#18570,.T.);
#23907=ORIENTED_EDGE('',*,*,#18571,.T.);
#23908=ORIENTED_EDGE('',*,*,#18566,.T.);
#23909=ORIENTED_EDGE('',*,*,#18568,.F.);
#23910=ORIENTED_EDGE('',*,*,#18572,.F.);
#23911=ORIENTED_EDGE('',*,*,#18573,.F.);
#23912=ORIENTED_EDGE('',*,*,#18570,.F.);
#23913=ORIENTED_EDGE('',*,*,#18574,.F.);
#23914=ORIENTED_EDGE('',*,*,#18575,.F.);
#23915=ORIENTED_EDGE('',*,*,#17647,.T.);
#23916=ORIENTED_EDGE('',*,*,#18576,.T.);
#23917=ORIENTED_EDGE('',*,*,#18574,.T.);
#23918=ORIENTED_EDGE('',*,*,#18577,.T.);
#23919=ORIENTED_EDGE('',*,*,#18578,.F.);
#23920=ORIENTED_EDGE('',*,*,#18579,.F.);
#23921=ORIENTED_EDGE('',*,*,#18580,.F.);
#23922=ORIENTED_EDGE('',*,*,#17645,.T.);
#23923=ORIENTED_EDGE('',*,*,#18581,.T.);
#23924=ORIENTED_EDGE('',*,*,#18579,.T.);
#23925=ORIENTED_EDGE('',*,*,#18582,.T.);
#23926=ORIENTED_EDGE('',*,*,#18572,.T.);
#23927=ORIENTED_EDGE('',*,*,#18583,.T.);
#23928=ORIENTED_EDGE('',*,*,#18580,.T.);
#23929=ORIENTED_EDGE('',*,*,#18584,.T.);
#23930=ORIENTED_EDGE('',*,*,#18578,.T.);
#23931=ORIENTED_EDGE('',*,*,#18585,.T.);
#23932=ORIENTED_EDGE('',*,*,#18575,.T.);
#23933=ORIENTED_EDGE('',*,*,#18586,.T.);
#23934=ORIENTED_EDGE('',*,*,#17651,.T.);
#23935=ORIENTED_EDGE('',*,*,#18565,.T.);
#23936=ORIENTED_EDGE('',*,*,#18573,.T.);
#23937=ORIENTED_EDGE('',*,*,#18587,.T.);
#23938=ORIENTED_EDGE('',*,*,#18562,.F.);
#23939=ORIENTED_EDGE('',*,*,#17648,.F.);
#23940=ORIENTED_EDGE('',*,*,#18577,.F.);
#23941=ORIENTED_EDGE('',*,*,#18569,.F.);
#23942=ORIENTED_EDGE('',*,*,#18583,.F.);
#23943=ORIENTED_EDGE('',*,*,#18567,.F.);
#23944=ORIENTED_EDGE('',*,*,#18571,.F.);
#23945=ORIENTED_EDGE('',*,*,#18585,.F.);
#23946=ORIENTED_EDGE('',*,*,#18588,.F.);
#23947=ORIENTED_EDGE('',*,*,#18589,.F.);
#23948=ORIENTED_EDGE('',*,*,#18590,.F.);
#23949=ORIENTED_EDGE('',*,*,#18591,.F.);
#23950=ORIENTED_EDGE('',*,*,#18592,.F.);
#23951=ORIENTED_EDGE('',*,*,#18593,.F.);
#23952=ORIENTED_EDGE('',*,*,#18594,.F.);
#23953=ORIENTED_EDGE('',*,*,#18595,.F.);
#23954=ORIENTED_EDGE('',*,*,#18596,.F.);
#23955=ORIENTED_EDGE('',*,*,#17655,.T.);
#23956=ORIENTED_EDGE('',*,*,#18597,.T.);
#23957=ORIENTED_EDGE('',*,*,#18595,.T.);
#23958=ORIENTED_EDGE('',*,*,#18598,.T.);
#23959=ORIENTED_EDGE('',*,*,#18599,.F.);
#23960=ORIENTED_EDGE('',*,*,#18600,.F.);
#23961=ORIENTED_EDGE('',*,*,#18601,.F.);
#23962=ORIENTED_EDGE('',*,*,#17653,.T.);
#23963=ORIENTED_EDGE('',*,*,#18602,.T.);
#23964=ORIENTED_EDGE('',*,*,#18600,.T.);
#23965=ORIENTED_EDGE('',*,*,#18603,.T.);
#23966=ORIENTED_EDGE('',*,*,#18592,.T.);
#23967=ORIENTED_EDGE('',*,*,#18604,.T.);
#23968=ORIENTED_EDGE('',*,*,#18601,.T.);
#23969=ORIENTED_EDGE('',*,*,#18605,.T.);
#23970=ORIENTED_EDGE('',*,*,#18599,.T.);
#23971=ORIENTED_EDGE('',*,*,#18606,.T.);
#23972=ORIENTED_EDGE('',*,*,#18596,.T.);
#23973=ORIENTED_EDGE('',*,*,#18607,.T.);
#23974=ORIENTED_EDGE('',*,*,#18589,.T.);
#23975=ORIENTED_EDGE('',*,*,#18608,.T.);
#23976=ORIENTED_EDGE('',*,*,#18594,.T.);
#23977=ORIENTED_EDGE('',*,*,#18609,.T.);
#23978=ORIENTED_EDGE('',*,*,#17659,.T.);
#23979=ORIENTED_EDGE('',*,*,#18610,.T.);
#23980=ORIENTED_EDGE('',*,*,#18593,.T.);
#23981=ORIENTED_EDGE('',*,*,#18611,.T.);
#23982=ORIENTED_EDGE('',*,*,#18591,.T.);
#23983=ORIENTED_EDGE('',*,*,#18612,.T.);
#23984=ORIENTED_EDGE('',*,*,#18590,.T.);
#23985=ORIENTED_EDGE('',*,*,#18613,.T.);
#23986=ORIENTED_EDGE('',*,*,#17657,.T.);
#23987=ORIENTED_EDGE('',*,*,#18614,.T.);
#23988=ORIENTED_EDGE('',*,*,#18588,.T.);
#23989=ORIENTED_EDGE('',*,*,#18615,.T.);
#23990=ORIENTED_EDGE('',*,*,#18603,.F.);
#23991=ORIENTED_EDGE('',*,*,#18607,.F.);
#23992=ORIENTED_EDGE('',*,*,#18597,.F.);
#23993=ORIENTED_EDGE('',*,*,#17654,.F.);
#23994=ORIENTED_EDGE('',*,*,#18598,.F.);
#23995=ORIENTED_EDGE('',*,*,#18608,.F.);
#23996=ORIENTED_EDGE('',*,*,#18614,.F.);
#23997=ORIENTED_EDGE('',*,*,#17656,.F.);
#23998=ORIENTED_EDGE('',*,*,#18604,.F.);
#23999=ORIENTED_EDGE('',*,*,#18613,.F.);
#24000=ORIENTED_EDGE('',*,*,#18609,.F.);
#24001=ORIENTED_EDGE('',*,*,#18606,.F.);
#24002=ORIENTED_EDGE('',*,*,#18616,.F.);
#24003=ORIENTED_EDGE('',*,*,#18617,.F.);
#24004=ORIENTED_EDGE('',*,*,#18618,.F.);
#24005=ORIENTED_EDGE('',*,*,#18619,.T.);
#24006=ORIENTED_EDGE('',*,*,#18620,.T.);
#24007=ORIENTED_EDGE('',*,*,#18617,.T.);
#24008=ORIENTED_EDGE('',*,*,#18621,.T.);
#24009=ORIENTED_EDGE('',*,*,#18622,.T.);
#24010=ORIENTED_EDGE('',*,*,#17667,.T.);
#24011=ORIENTED_EDGE('',*,*,#18623,.T.);
#24012=ORIENTED_EDGE('',*,*,#18618,.T.);
#24013=ORIENTED_EDGE('',*,*,#18624,.T.);
#24014=ORIENTED_EDGE('',*,*,#18625,.F.);
#24015=ORIENTED_EDGE('',*,*,#18626,.F.);
#24016=ORIENTED_EDGE('',*,*,#18627,.F.);
#24017=ORIENTED_EDGE('',*,*,#18628,.T.);
#24018=ORIENTED_EDGE('',*,*,#18629,.T.);
#24019=ORIENTED_EDGE('',*,*,#18626,.T.);
#24020=ORIENTED_EDGE('',*,*,#18630,.T.);
#24021=ORIENTED_EDGE('',*,*,#18631,.T.);
#24022=ORIENTED_EDGE('',*,*,#18616,.T.);
#24023=ORIENTED_EDGE('',*,*,#18632,.T.);
#24024=ORIENTED_EDGE('',*,*,#18627,.T.);
#24025=ORIENTED_EDGE('',*,*,#18633,.T.);
#24026=ORIENTED_EDGE('',*,*,#17665,.T.);
#24027=ORIENTED_EDGE('',*,*,#18634,.T.);
#24028=ORIENTED_EDGE('',*,*,#18625,.T.);
#24029=ORIENTED_EDGE('',*,*,#18635,.T.);
#24030=ORIENTED_EDGE('',*,*,#18619,.F.);
#24031=ORIENTED_EDGE('',*,*,#18636,.T.);
#24032=ORIENTED_EDGE('',*,*,#18637,.T.);
#24033=ORIENTED_EDGE('',*,*,#17661,.T.);
#24034=ORIENTED_EDGE('',*,*,#18638,.T.);
#24035=ORIENTED_EDGE('',*,*,#18621,.F.);
#24036=ORIENTED_EDGE('',*,*,#18633,.F.);
#24037=ORIENTED_EDGE('',*,*,#18629,.F.);
#24038=ORIENTED_EDGE('',*,*,#18639,.F.);
#24039=ORIENTED_EDGE('',*,*,#18622,.F.);
#24040=ORIENTED_EDGE('',*,*,#18639,.T.);
#24041=ORIENTED_EDGE('',*,*,#18628,.F.);
#24042=ORIENTED_EDGE('',*,*,#18640,.F.);
#24043=ORIENTED_EDGE('',*,*,#18641,.T.);
#24044=ORIENTED_EDGE('',*,*,#18636,.F.);
#24045=ORIENTED_EDGE('',*,*,#18631,.F.);
#24046=ORIENTED_EDGE('',*,*,#18642,.T.);
#24047=ORIENTED_EDGE('',*,*,#17663,.T.);
#24048=ORIENTED_EDGE('',*,*,#18643,.T.);
#24049=ORIENTED_EDGE('',*,*,#18640,.T.);
#24050=ORIENTED_EDGE('',*,*,#18630,.F.);
#24051=ORIENTED_EDGE('',*,*,#18634,.F.);
#24052=ORIENTED_EDGE('',*,*,#17664,.F.);
#24053=ORIENTED_EDGE('',*,*,#18642,.F.);
#24054=ORIENTED_EDGE('',*,*,#18620,.F.);
#24055=ORIENTED_EDGE('',*,*,#18638,.F.);
#24056=ORIENTED_EDGE('',*,*,#17660,.F.);
#24057=ORIENTED_EDGE('',*,*,#18624,.F.);
#24058=ORIENTED_EDGE('',*,*,#18644,.F.);
#24059=ORIENTED_EDGE('',*,*,#18645,.F.);
#24060=ORIENTED_EDGE('',*,*,#18646,.F.);
#24061=ORIENTED_EDGE('',*,*,#18647,.F.);
#24062=ORIENTED_EDGE('',*,*,#18648,.F.);
#24063=ORIENTED_EDGE('',*,*,#18649,.F.);
#24064=ORIENTED_EDGE('',*,*,#18650,.F.);
#24065=ORIENTED_EDGE('',*,*,#18651,.F.);
#24066=ORIENTED_EDGE('',*,*,#18652,.F.);
#24067=ORIENTED_EDGE('',*,*,#17520,.T.);
#24068=ORIENTED_EDGE('',*,*,#18653,.T.);
#24069=ORIENTED_EDGE('',*,*,#18651,.T.);
#24070=ORIENTED_EDGE('',*,*,#18654,.T.);
#24071=ORIENTED_EDGE('',*,*,#18655,.F.);
#24072=ORIENTED_EDGE('',*,*,#18656,.F.);
#24073=ORIENTED_EDGE('',*,*,#18657,.F.);
#24074=ORIENTED_EDGE('',*,*,#17515,.T.);
#24075=ORIENTED_EDGE('',*,*,#18658,.T.);
#24076=ORIENTED_EDGE('',*,*,#18656,.T.);
#24077=ORIENTED_EDGE('',*,*,#18659,.T.);
#24078=ORIENTED_EDGE('',*,*,#18648,.T.);
#24079=ORIENTED_EDGE('',*,*,#18660,.T.);
#24080=ORIENTED_EDGE('',*,*,#18657,.T.);
#24081=ORIENTED_EDGE('',*,*,#18661,.T.);
#24082=ORIENTED_EDGE('',*,*,#18655,.T.);
#24083=ORIENTED_EDGE('',*,*,#18662,.T.);
#24084=ORIENTED_EDGE('',*,*,#18652,.T.);
#24085=ORIENTED_EDGE('',*,*,#18663,.T.);
#24086=ORIENTED_EDGE('',*,*,#18645,.T.);
#24087=ORIENTED_EDGE('',*,*,#18664,.T.);
#24088=ORIENTED_EDGE('',*,*,#18650,.T.);
#24089=ORIENTED_EDGE('',*,*,#18665,.T.);
#24090=ORIENTED_EDGE('',*,*,#17513,.T.);
#24091=ORIENTED_EDGE('',*,*,#18666,.T.);
#24092=ORIENTED_EDGE('',*,*,#18649,.T.);
#24093=ORIENTED_EDGE('',*,*,#18667,.T.);
#24094=ORIENTED_EDGE('',*,*,#18647,.T.);
#24095=ORIENTED_EDGE('',*,*,#18668,.T.);
#24096=ORIENTED_EDGE('',*,*,#18646,.T.);
#24097=ORIENTED_EDGE('',*,*,#18669,.T.);
#24098=ORIENTED_EDGE('',*,*,#17522,.T.);
#24099=ORIENTED_EDGE('',*,*,#18670,.T.);
#24100=ORIENTED_EDGE('',*,*,#18644,.T.);
#24101=ORIENTED_EDGE('',*,*,#18671,.T.);
#24102=ORIENTED_EDGE('',*,*,#18659,.F.);
#24103=ORIENTED_EDGE('',*,*,#18663,.F.);
#24104=ORIENTED_EDGE('',*,*,#18653,.F.);
#24105=ORIENTED_EDGE('',*,*,#17519,.F.);
#24106=ORIENTED_EDGE('',*,*,#17516,.F.);
#24107=ORIENTED_EDGE('',*,*,#18654,.F.);
#24108=ORIENTED_EDGE('',*,*,#18664,.F.);
#24109=ORIENTED_EDGE('',*,*,#18670,.F.);
#24110=ORIENTED_EDGE('',*,*,#17521,.F.);
#24111=ORIENTED_EDGE('',*,*,#18660,.F.);
#24112=ORIENTED_EDGE('',*,*,#18669,.F.);
#24113=ORIENTED_EDGE('',*,*,#18665,.F.);
#24114=ORIENTED_EDGE('',*,*,#18662,.F.);
#24115=ORIENTED_EDGE('',*,*,#18672,.F.);
#24116=ORIENTED_EDGE('',*,*,#18673,.F.);
#24117=ORIENTED_EDGE('',*,*,#18674,.F.);
#24118=ORIENTED_EDGE('',*,*,#18675,.F.);
#24119=ORIENTED_EDGE('',*,*,#18676,.F.);
#24120=ORIENTED_EDGE('',*,*,#18677,.F.);
#24121=ORIENTED_EDGE('',*,*,#18678,.F.);
#24122=ORIENTED_EDGE('',*,*,#18679,.F.);
#24123=ORIENTED_EDGE('',*,*,#18680,.F.);
#24124=ORIENTED_EDGE('',*,*,#17671,.T.);
#24125=ORIENTED_EDGE('',*,*,#18681,.T.);
#24126=ORIENTED_EDGE('',*,*,#18679,.T.);
#24127=ORIENTED_EDGE('',*,*,#18682,.T.);
#24128=ORIENTED_EDGE('',*,*,#18683,.F.);
#24129=ORIENTED_EDGE('',*,*,#18684,.F.);
#24130=ORIENTED_EDGE('',*,*,#18685,.F.);
#24131=ORIENTED_EDGE('',*,*,#17669,.T.);
#24132=ORIENTED_EDGE('',*,*,#18686,.T.);
#24133=ORIENTED_EDGE('',*,*,#18684,.T.);
#24134=ORIENTED_EDGE('',*,*,#18687,.T.);
#24135=ORIENTED_EDGE('',*,*,#18676,.T.);
#24136=ORIENTED_EDGE('',*,*,#18688,.T.);
#24137=ORIENTED_EDGE('',*,*,#18685,.T.);
#24138=ORIENTED_EDGE('',*,*,#18689,.T.);
#24139=ORIENTED_EDGE('',*,*,#18683,.T.);
#24140=ORIENTED_EDGE('',*,*,#18690,.T.);
#24141=ORIENTED_EDGE('',*,*,#18680,.T.);
#24142=ORIENTED_EDGE('',*,*,#18691,.T.);
#24143=ORIENTED_EDGE('',*,*,#18673,.T.);
#24144=ORIENTED_EDGE('',*,*,#18692,.T.);
#24145=ORIENTED_EDGE('',*,*,#18678,.T.);
#24146=ORIENTED_EDGE('',*,*,#18693,.T.);
#24147=ORIENTED_EDGE('',*,*,#17675,.T.);
#24148=ORIENTED_EDGE('',*,*,#18694,.T.);
#24149=ORIENTED_EDGE('',*,*,#18677,.T.);
#24150=ORIENTED_EDGE('',*,*,#18695,.T.);
#24151=ORIENTED_EDGE('',*,*,#18675,.T.);
#24152=ORIENTED_EDGE('',*,*,#18696,.T.);
#24153=ORIENTED_EDGE('',*,*,#18674,.T.);
#24154=ORIENTED_EDGE('',*,*,#18697,.T.);
#24155=ORIENTED_EDGE('',*,*,#17673,.T.);
#24156=ORIENTED_EDGE('',*,*,#18698,.T.);
#24157=ORIENTED_EDGE('',*,*,#18672,.T.);
#24158=ORIENTED_EDGE('',*,*,#18699,.T.);
#24159=ORIENTED_EDGE('',*,*,#18687,.F.);
#24160=ORIENTED_EDGE('',*,*,#18691,.F.);
#24161=ORIENTED_EDGE('',*,*,#18681,.F.);
#24162=ORIENTED_EDGE('',*,*,#17670,.F.);
#24163=ORIENTED_EDGE('',*,*,#18682,.F.);
#24164=ORIENTED_EDGE('',*,*,#18692,.F.);
#24165=ORIENTED_EDGE('',*,*,#18698,.F.);
#24166=ORIENTED_EDGE('',*,*,#17672,.F.);
#24167=ORIENTED_EDGE('',*,*,#18688,.F.);
#24168=ORIENTED_EDGE('',*,*,#18697,.F.);
#24169=ORIENTED_EDGE('',*,*,#18693,.F.);
#24170=ORIENTED_EDGE('',*,*,#18690,.F.);
#24171=ORIENTED_EDGE('',*,*,#18700,.T.);
#24172=ORIENTED_EDGE('',*,*,#18701,.T.);
#24173=ORIENTED_EDGE('',*,*,#17681,.T.);
#24174=ORIENTED_EDGE('',*,*,#18702,.T.);
#24175=ORIENTED_EDGE('',*,*,#18703,.T.);
#24176=ORIENTED_EDGE('',*,*,#18701,.F.);
#24177=ORIENTED_EDGE('',*,*,#18704,.F.);
#24178=ORIENTED_EDGE('',*,*,#18705,.F.);
#24179=ORIENTED_EDGE('',*,*,#17682,.F.);
#24180=ORIENTED_EDGE('',*,*,#18700,.F.);
#24181=ORIENTED_EDGE('',*,*,#18706,.F.);
#24182=ORIENTED_EDGE('',*,*,#18707,.T.);
#24183=ORIENTED_EDGE('',*,*,#18708,.T.);
#24184=ORIENTED_EDGE('',*,*,#18704,.T.);
#24185=ORIENTED_EDGE('',*,*,#18703,.F.);
#24186=ORIENTED_EDGE('',*,*,#18709,.T.);
#24187=ORIENTED_EDGE('',*,*,#18710,.T.);
#24188=ORIENTED_EDGE('',*,*,#18711,.T.);
#24189=ORIENTED_EDGE('',*,*,#18706,.T.);
#24190=ORIENTED_EDGE('',*,*,#18708,.F.);
#24191=ORIENTED_EDGE('',*,*,#18712,.F.);
#24192=ORIENTED_EDGE('',*,*,#18713,.F.);
#24193=ORIENTED_EDGE('',*,*,#18710,.F.);
#24194=ORIENTED_EDGE('',*,*,#18714,.F.);
#24195=ORIENTED_EDGE('',*,*,#18715,.F.);
#24196=ORIENTED_EDGE('',*,*,#17679,.T.);
#24197=ORIENTED_EDGE('',*,*,#18716,.T.);
#24198=ORIENTED_EDGE('',*,*,#18714,.T.);
#24199=ORIENTED_EDGE('',*,*,#18717,.T.);
#24200=ORIENTED_EDGE('',*,*,#18718,.F.);
#24201=ORIENTED_EDGE('',*,*,#18719,.F.);
#24202=ORIENTED_EDGE('',*,*,#18720,.F.);
#24203=ORIENTED_EDGE('',*,*,#17677,.T.);
#24204=ORIENTED_EDGE('',*,*,#18721,.T.);
#24205=ORIENTED_EDGE('',*,*,#18719,.T.);
#24206=ORIENTED_EDGE('',*,*,#18722,.T.);
#24207=ORIENTED_EDGE('',*,*,#18712,.T.);
#24208=ORIENTED_EDGE('',*,*,#18723,.T.);
#24209=ORIENTED_EDGE('',*,*,#18720,.T.);
#24210=ORIENTED_EDGE('',*,*,#18724,.T.);
#24211=ORIENTED_EDGE('',*,*,#18718,.T.);
#24212=ORIENTED_EDGE('',*,*,#18725,.T.);
#24213=ORIENTED_EDGE('',*,*,#18715,.T.);
#24214=ORIENTED_EDGE('',*,*,#18726,.T.);
#24215=ORIENTED_EDGE('',*,*,#17683,.T.);
#24216=ORIENTED_EDGE('',*,*,#18705,.T.);
#24217=ORIENTED_EDGE('',*,*,#18713,.T.);
#24218=ORIENTED_EDGE('',*,*,#18727,.T.);
#24219=ORIENTED_EDGE('',*,*,#18702,.F.);
#24220=ORIENTED_EDGE('',*,*,#17680,.F.);
#24221=ORIENTED_EDGE('',*,*,#18717,.F.);
#24222=ORIENTED_EDGE('',*,*,#18709,.F.);
#24223=ORIENTED_EDGE('',*,*,#18723,.F.);
#24224=ORIENTED_EDGE('',*,*,#18707,.F.);
#24225=ORIENTED_EDGE('',*,*,#18711,.F.);
#24226=ORIENTED_EDGE('',*,*,#18725,.F.);
#24227=ORIENTED_EDGE('',*,*,#18728,.F.);
#24228=ORIENTED_EDGE('',*,*,#18729,.F.);
#24229=ORIENTED_EDGE('',*,*,#18730,.F.);
#24230=ORIENTED_EDGE('',*,*,#18731,.F.);
#24231=ORIENTED_EDGE('',*,*,#18732,.F.);
#24232=ORIENTED_EDGE('',*,*,#18733,.F.);
#24233=ORIENTED_EDGE('',*,*,#18734,.F.);
#24234=ORIENTED_EDGE('',*,*,#18735,.F.);
#24235=ORIENTED_EDGE('',*,*,#18736,.F.);
#24236=ORIENTED_EDGE('',*,*,#17687,.T.);
#24237=ORIENTED_EDGE('',*,*,#18737,.T.);
#24238=ORIENTED_EDGE('',*,*,#18735,.T.);
#24239=ORIENTED_EDGE('',*,*,#18738,.T.);
#24240=ORIENTED_EDGE('',*,*,#18739,.F.);
#24241=ORIENTED_EDGE('',*,*,#18740,.F.);
#24242=ORIENTED_EDGE('',*,*,#18741,.F.);
#24243=ORIENTED_EDGE('',*,*,#17685,.T.);
#24244=ORIENTED_EDGE('',*,*,#18742,.T.);
#24245=ORIENTED_EDGE('',*,*,#18740,.T.);
#24246=ORIENTED_EDGE('',*,*,#18743,.T.);
#24247=ORIENTED_EDGE('',*,*,#18732,.T.);
#24248=ORIENTED_EDGE('',*,*,#18744,.T.);
#24249=ORIENTED_EDGE('',*,*,#18741,.T.);
#24250=ORIENTED_EDGE('',*,*,#18745,.T.);
#24251=ORIENTED_EDGE('',*,*,#18739,.T.);
#24252=ORIENTED_EDGE('',*,*,#18746,.T.);
#24253=ORIENTED_EDGE('',*,*,#18736,.T.);
#24254=ORIENTED_EDGE('',*,*,#18747,.T.);
#24255=ORIENTED_EDGE('',*,*,#18729,.T.);
#24256=ORIENTED_EDGE('',*,*,#18748,.T.);
#24257=ORIENTED_EDGE('',*,*,#18734,.T.);
#24258=ORIENTED_EDGE('',*,*,#18749,.T.);
#24259=ORIENTED_EDGE('',*,*,#17691,.T.);
#24260=ORIENTED_EDGE('',*,*,#18750,.T.);
#24261=ORIENTED_EDGE('',*,*,#18733,.T.);
#24262=ORIENTED_EDGE('',*,*,#18751,.T.);
#24263=ORIENTED_EDGE('',*,*,#18731,.T.);
#24264=ORIENTED_EDGE('',*,*,#18752,.T.);
#24265=ORIENTED_EDGE('',*,*,#18730,.T.);
#24266=ORIENTED_EDGE('',*,*,#18753,.T.);
#24267=ORIENTED_EDGE('',*,*,#17689,.T.);
#24268=ORIENTED_EDGE('',*,*,#18754,.T.);
#24269=ORIENTED_EDGE('',*,*,#18728,.T.);
#24270=ORIENTED_EDGE('',*,*,#18755,.T.);
#24271=ORIENTED_EDGE('',*,*,#18743,.F.);
#24272=ORIENTED_EDGE('',*,*,#18747,.F.);
#24273=ORIENTED_EDGE('',*,*,#18737,.F.);
#24274=ORIENTED_EDGE('',*,*,#17686,.F.);
#24275=ORIENTED_EDGE('',*,*,#18738,.F.);
#24276=ORIENTED_EDGE('',*,*,#18748,.F.);
#24277=ORIENTED_EDGE('',*,*,#18754,.F.);
#24278=ORIENTED_EDGE('',*,*,#17688,.F.);
#24279=ORIENTED_EDGE('',*,*,#18744,.F.);
#24280=ORIENTED_EDGE('',*,*,#18753,.F.);
#24281=ORIENTED_EDGE('',*,*,#18749,.F.);
#24282=ORIENTED_EDGE('',*,*,#18746,.F.);
#24283=ORIENTED_EDGE('',*,*,#18756,.F.);
#24284=ORIENTED_EDGE('',*,*,#18757,.F.);
#24285=ORIENTED_EDGE('',*,*,#18758,.F.);
#24286=ORIENTED_EDGE('',*,*,#18759,.T.);
#24287=ORIENTED_EDGE('',*,*,#18760,.T.);
#24288=ORIENTED_EDGE('',*,*,#18757,.T.);
#24289=ORIENTED_EDGE('',*,*,#18761,.T.);
#24290=ORIENTED_EDGE('',*,*,#18762,.T.);
#24291=ORIENTED_EDGE('',*,*,#17699,.T.);
#24292=ORIENTED_EDGE('',*,*,#18763,.T.);
#24293=ORIENTED_EDGE('',*,*,#18758,.T.);
#24294=ORIENTED_EDGE('',*,*,#18764,.T.);
#24295=ORIENTED_EDGE('',*,*,#18765,.F.);
#24296=ORIENTED_EDGE('',*,*,#18766,.F.);
#24297=ORIENTED_EDGE('',*,*,#18767,.F.);
#24298=ORIENTED_EDGE('',*,*,#18768,.T.);
#24299=ORIENTED_EDGE('',*,*,#18769,.T.);
#24300=ORIENTED_EDGE('',*,*,#18766,.T.);
#24301=ORIENTED_EDGE('',*,*,#18770,.T.);
#24302=ORIENTED_EDGE('',*,*,#18771,.T.);
#24303=ORIENTED_EDGE('',*,*,#18756,.T.);
#24304=ORIENTED_EDGE('',*,*,#18772,.T.);
#24305=ORIENTED_EDGE('',*,*,#18767,.T.);
#24306=ORIENTED_EDGE('',*,*,#18773,.T.);
#24307=ORIENTED_EDGE('',*,*,#17697,.T.);
#24308=ORIENTED_EDGE('',*,*,#18774,.T.);
#24309=ORIENTED_EDGE('',*,*,#18765,.T.);
#24310=ORIENTED_EDGE('',*,*,#18775,.T.);
#24311=ORIENTED_EDGE('',*,*,#18759,.F.);
#24312=ORIENTED_EDGE('',*,*,#18776,.T.);
#24313=ORIENTED_EDGE('',*,*,#18777,.T.);
#24314=ORIENTED_EDGE('',*,*,#17693,.T.);
#24315=ORIENTED_EDGE('',*,*,#18778,.T.);
#24316=ORIENTED_EDGE('',*,*,#18761,.F.);
#24317=ORIENTED_EDGE('',*,*,#18773,.F.);
#24318=ORIENTED_EDGE('',*,*,#18769,.F.);
#24319=ORIENTED_EDGE('',*,*,#18779,.F.);
#24320=ORIENTED_EDGE('',*,*,#18762,.F.);
#24321=ORIENTED_EDGE('',*,*,#18779,.T.);
#24322=ORIENTED_EDGE('',*,*,#18768,.F.);
#24323=ORIENTED_EDGE('',*,*,#18780,.F.);
#24324=ORIENTED_EDGE('',*,*,#18781,.T.);
#24325=ORIENTED_EDGE('',*,*,#18776,.F.);
#24326=ORIENTED_EDGE('',*,*,#18771,.F.);
#24327=ORIENTED_EDGE('',*,*,#18782,.T.);
#24328=ORIENTED_EDGE('',*,*,#17695,.T.);
#24329=ORIENTED_EDGE('',*,*,#18783,.T.);
#24330=ORIENTED_EDGE('',*,*,#18780,.T.);
#24331=ORIENTED_EDGE('',*,*,#18770,.F.);
#24332=ORIENTED_EDGE('',*,*,#18774,.F.);
#24333=ORIENTED_EDGE('',*,*,#17696,.F.);
#24334=ORIENTED_EDGE('',*,*,#18782,.F.);
#24335=ORIENTED_EDGE('',*,*,#18760,.F.);
#24336=ORIENTED_EDGE('',*,*,#18778,.F.);
#24337=ORIENTED_EDGE('',*,*,#17692,.F.);
#24338=ORIENTED_EDGE('',*,*,#18764,.F.);
#24339=ORIENTED_EDGE('',*,*,#18784,.F.);
#24340=ORIENTED_EDGE('',*,*,#18785,.F.);
#24341=ORIENTED_EDGE('',*,*,#18786,.F.);
#24342=ORIENTED_EDGE('',*,*,#18787,.F.);
#24343=ORIENTED_EDGE('',*,*,#18788,.F.);
#24344=ORIENTED_EDGE('',*,*,#18789,.F.);
#24345=ORIENTED_EDGE('',*,*,#18790,.F.);
#24346=ORIENTED_EDGE('',*,*,#18791,.F.);
#24347=ORIENTED_EDGE('',*,*,#18792,.F.);
#24348=ORIENTED_EDGE('',*,*,#17703,.T.);
#24349=ORIENTED_EDGE('',*,*,#18793,.T.);
#24350=ORIENTED_EDGE('',*,*,#18791,.T.);
#24351=ORIENTED_EDGE('',*,*,#18794,.T.);
#24352=ORIENTED_EDGE('',*,*,#18795,.F.);
#24353=ORIENTED_EDGE('',*,*,#18796,.F.);
#24354=ORIENTED_EDGE('',*,*,#18797,.F.);
#24355=ORIENTED_EDGE('',*,*,#17701,.T.);
#24356=ORIENTED_EDGE('',*,*,#18798,.T.);
#24357=ORIENTED_EDGE('',*,*,#18796,.T.);
#24358=ORIENTED_EDGE('',*,*,#18799,.T.);
#24359=ORIENTED_EDGE('',*,*,#18788,.T.);
#24360=ORIENTED_EDGE('',*,*,#18800,.T.);
#24361=ORIENTED_EDGE('',*,*,#18797,.T.);
#24362=ORIENTED_EDGE('',*,*,#18801,.T.);
#24363=ORIENTED_EDGE('',*,*,#18795,.T.);
#24364=ORIENTED_EDGE('',*,*,#18802,.T.);
#24365=ORIENTED_EDGE('',*,*,#18792,.T.);
#24366=ORIENTED_EDGE('',*,*,#18803,.T.);
#24367=ORIENTED_EDGE('',*,*,#18785,.T.);
#24368=ORIENTED_EDGE('',*,*,#18804,.T.);
#24369=ORIENTED_EDGE('',*,*,#18790,.T.);
#24370=ORIENTED_EDGE('',*,*,#18805,.T.);
#24371=ORIENTED_EDGE('',*,*,#17707,.T.);
#24372=ORIENTED_EDGE('',*,*,#18806,.T.);
#24373=ORIENTED_EDGE('',*,*,#18789,.T.);
#24374=ORIENTED_EDGE('',*,*,#18807,.T.);
#24375=ORIENTED_EDGE('',*,*,#18787,.T.);
#24376=ORIENTED_EDGE('',*,*,#18808,.T.);
#24377=ORIENTED_EDGE('',*,*,#18786,.T.);
#24378=ORIENTED_EDGE('',*,*,#18809,.T.);
#24379=ORIENTED_EDGE('',*,*,#17705,.T.);
#24380=ORIENTED_EDGE('',*,*,#18810,.T.);
#24381=ORIENTED_EDGE('',*,*,#18784,.T.);
#24382=ORIENTED_EDGE('',*,*,#18811,.T.);
#24383=ORIENTED_EDGE('',*,*,#18799,.F.);
#24384=ORIENTED_EDGE('',*,*,#18803,.F.);
#24385=ORIENTED_EDGE('',*,*,#18793,.F.);
#24386=ORIENTED_EDGE('',*,*,#17702,.F.);
#24387=ORIENTED_EDGE('',*,*,#18794,.F.);
#24388=ORIENTED_EDGE('',*,*,#18804,.F.);
#24389=ORIENTED_EDGE('',*,*,#18810,.F.);
#24390=ORIENTED_EDGE('',*,*,#17704,.F.);
#24391=ORIENTED_EDGE('',*,*,#18800,.F.);
#24392=ORIENTED_EDGE('',*,*,#18809,.F.);
#24393=ORIENTED_EDGE('',*,*,#18805,.F.);
#24394=ORIENTED_EDGE('',*,*,#18802,.F.);
#24395=ORIENTED_EDGE('',*,*,#18812,.F.);
#24396=ORIENTED_EDGE('',*,*,#18813,.F.);
#24397=ORIENTED_EDGE('',*,*,#18814,.F.);
#24398=ORIENTED_EDGE('',*,*,#18815,.F.);
#24399=ORIENTED_EDGE('',*,*,#18816,.F.);
#24400=ORIENTED_EDGE('',*,*,#18817,.F.);
#24401=ORIENTED_EDGE('',*,*,#18818,.F.);
#24402=ORIENTED_EDGE('',*,*,#18819,.F.);
#24403=ORIENTED_EDGE('',*,*,#18820,.F.);
#24404=ORIENTED_EDGE('',*,*,#17711,.T.);
#24405=ORIENTED_EDGE('',*,*,#18821,.T.);
#24406=ORIENTED_EDGE('',*,*,#18819,.T.);
#24407=ORIENTED_EDGE('',*,*,#18822,.T.);
#24408=ORIENTED_EDGE('',*,*,#18823,.F.);
#24409=ORIENTED_EDGE('',*,*,#18824,.F.);
#24410=ORIENTED_EDGE('',*,*,#18825,.F.);
#24411=ORIENTED_EDGE('',*,*,#17709,.T.);
#24412=ORIENTED_EDGE('',*,*,#18826,.T.);
#24413=ORIENTED_EDGE('',*,*,#18824,.T.);
#24414=ORIENTED_EDGE('',*,*,#18827,.T.);
#24415=ORIENTED_EDGE('',*,*,#18816,.T.);
#24416=ORIENTED_EDGE('',*,*,#18828,.T.);
#24417=ORIENTED_EDGE('',*,*,#18825,.T.);
#24418=ORIENTED_EDGE('',*,*,#18829,.T.);
#24419=ORIENTED_EDGE('',*,*,#18823,.T.);
#24420=ORIENTED_EDGE('',*,*,#18830,.T.);
#24421=ORIENTED_EDGE('',*,*,#18820,.T.);
#24422=ORIENTED_EDGE('',*,*,#18831,.T.);
#24423=ORIENTED_EDGE('',*,*,#18813,.T.);
#24424=ORIENTED_EDGE('',*,*,#18832,.T.);
#24425=ORIENTED_EDGE('',*,*,#18818,.T.);
#24426=ORIENTED_EDGE('',*,*,#18833,.T.);
#24427=ORIENTED_EDGE('',*,*,#17715,.T.);
#24428=ORIENTED_EDGE('',*,*,#18834,.T.);
#24429=ORIENTED_EDGE('',*,*,#18817,.T.);
#24430=ORIENTED_EDGE('',*,*,#18835,.T.);
#24431=ORIENTED_EDGE('',*,*,#18815,.T.);
#24432=ORIENTED_EDGE('',*,*,#18836,.T.);
#24433=ORIENTED_EDGE('',*,*,#18814,.T.);
#24434=ORIENTED_EDGE('',*,*,#18837,.T.);
#24435=ORIENTED_EDGE('',*,*,#17713,.T.);
#24436=ORIENTED_EDGE('',*,*,#18838,.T.);
#24437=ORIENTED_EDGE('',*,*,#18812,.T.);
#24438=ORIENTED_EDGE('',*,*,#18839,.T.);
#24439=ORIENTED_EDGE('',*,*,#18827,.F.);
#24440=ORIENTED_EDGE('',*,*,#18831,.F.);
#24441=ORIENTED_EDGE('',*,*,#18821,.F.);
#24442=ORIENTED_EDGE('',*,*,#17710,.F.);
#24443=ORIENTED_EDGE('',*,*,#18822,.F.);
#24444=ORIENTED_EDGE('',*,*,#18832,.F.);
#24445=ORIENTED_EDGE('',*,*,#18838,.F.);
#24446=ORIENTED_EDGE('',*,*,#17712,.F.);
#24447=ORIENTED_EDGE('',*,*,#18828,.F.);
#24448=ORIENTED_EDGE('',*,*,#18837,.F.);
#24449=ORIENTED_EDGE('',*,*,#18833,.F.);
#24450=ORIENTED_EDGE('',*,*,#18830,.F.);
#24451=ORIENTED_EDGE('',*,*,#18840,.T.);
#24452=ORIENTED_EDGE('',*,*,#18841,.T.);
#24453=ORIENTED_EDGE('',*,*,#17721,.T.);
#24454=ORIENTED_EDGE('',*,*,#18842,.T.);
#24455=ORIENTED_EDGE('',*,*,#18843,.T.);
#24456=ORIENTED_EDGE('',*,*,#18841,.F.);
#24457=ORIENTED_EDGE('',*,*,#18844,.F.);
#24458=ORIENTED_EDGE('',*,*,#18845,.F.);
#24459=ORIENTED_EDGE('',*,*,#17722,.F.);
#24460=ORIENTED_EDGE('',*,*,#18840,.F.);
#24461=ORIENTED_EDGE('',*,*,#18846,.F.);
#24462=ORIENTED_EDGE('',*,*,#18847,.T.);
#24463=ORIENTED_EDGE('',*,*,#18848,.T.);
#24464=ORIENTED_EDGE('',*,*,#18844,.T.);
#24465=ORIENTED_EDGE('',*,*,#18843,.F.);
#24466=ORIENTED_EDGE('',*,*,#18849,.T.);
#24467=ORIENTED_EDGE('',*,*,#18850,.T.);
#24468=ORIENTED_EDGE('',*,*,#18851,.T.);
#24469=ORIENTED_EDGE('',*,*,#18846,.T.);
#24470=ORIENTED_EDGE('',*,*,#18848,.F.);
#24471=ORIENTED_EDGE('',*,*,#18852,.F.);
#24472=ORIENTED_EDGE('',*,*,#18853,.F.);
#24473=ORIENTED_EDGE('',*,*,#18850,.F.);
#24474=ORIENTED_EDGE('',*,*,#18854,.F.);
#24475=ORIENTED_EDGE('',*,*,#18855,.F.);
#24476=ORIENTED_EDGE('',*,*,#17719,.T.);
#24477=ORIENTED_EDGE('',*,*,#18856,.T.);
#24478=ORIENTED_EDGE('',*,*,#18854,.T.);
#24479=ORIENTED_EDGE('',*,*,#18857,.T.);
#24480=ORIENTED_EDGE('',*,*,#18858,.F.);
#24481=ORIENTED_EDGE('',*,*,#18859,.F.);
#24482=ORIENTED_EDGE('',*,*,#18860,.F.);
#24483=ORIENTED_EDGE('',*,*,#17717,.T.);
#24484=ORIENTED_EDGE('',*,*,#18861,.T.);
#24485=ORIENTED_EDGE('',*,*,#18859,.T.);
#24486=ORIENTED_EDGE('',*,*,#18862,.T.);
#24487=ORIENTED_EDGE('',*,*,#18852,.T.);
#24488=ORIENTED_EDGE('',*,*,#18863,.T.);
#24489=ORIENTED_EDGE('',*,*,#18860,.T.);
#24490=ORIENTED_EDGE('',*,*,#18864,.T.);
#24491=ORIENTED_EDGE('',*,*,#18858,.T.);
#24492=ORIENTED_EDGE('',*,*,#18865,.T.);
#24493=ORIENTED_EDGE('',*,*,#18855,.T.);
#24494=ORIENTED_EDGE('',*,*,#18866,.T.);
#24495=ORIENTED_EDGE('',*,*,#17723,.T.);
#24496=ORIENTED_EDGE('',*,*,#18845,.T.);
#24497=ORIENTED_EDGE('',*,*,#18853,.T.);
#24498=ORIENTED_EDGE('',*,*,#18867,.T.);
#24499=ORIENTED_EDGE('',*,*,#18842,.F.);
#24500=ORIENTED_EDGE('',*,*,#17720,.F.);
#24501=ORIENTED_EDGE('',*,*,#18857,.F.);
#24502=ORIENTED_EDGE('',*,*,#18849,.F.);
#24503=ORIENTED_EDGE('',*,*,#18863,.F.);
#24504=ORIENTED_EDGE('',*,*,#18847,.F.);
#24505=ORIENTED_EDGE('',*,*,#18851,.F.);
#24506=ORIENTED_EDGE('',*,*,#18865,.F.);
#24507=ORIENTED_EDGE('',*,*,#18868,.F.);
#24508=ORIENTED_EDGE('',*,*,#18869,.F.);
#24509=ORIENTED_EDGE('',*,*,#18870,.F.);
#24510=ORIENTED_EDGE('',*,*,#18871,.F.);
#24511=ORIENTED_EDGE('',*,*,#18872,.F.);
#24512=ORIENTED_EDGE('',*,*,#18873,.F.);
#24513=ORIENTED_EDGE('',*,*,#18874,.F.);
#24514=ORIENTED_EDGE('',*,*,#18875,.F.);
#24515=ORIENTED_EDGE('',*,*,#18876,.F.);
#24516=ORIENTED_EDGE('',*,*,#17727,.T.);
#24517=ORIENTED_EDGE('',*,*,#18877,.T.);
#24518=ORIENTED_EDGE('',*,*,#18875,.T.);
#24519=ORIENTED_EDGE('',*,*,#18878,.T.);
#24520=ORIENTED_EDGE('',*,*,#18879,.F.);
#24521=ORIENTED_EDGE('',*,*,#18880,.F.);
#24522=ORIENTED_EDGE('',*,*,#18881,.F.);
#24523=ORIENTED_EDGE('',*,*,#17725,.T.);
#24524=ORIENTED_EDGE('',*,*,#18882,.T.);
#24525=ORIENTED_EDGE('',*,*,#18880,.T.);
#24526=ORIENTED_EDGE('',*,*,#18883,.T.);
#24527=ORIENTED_EDGE('',*,*,#18872,.T.);
#24528=ORIENTED_EDGE('',*,*,#18884,.T.);
#24529=ORIENTED_EDGE('',*,*,#18881,.T.);
#24530=ORIENTED_EDGE('',*,*,#18885,.T.);
#24531=ORIENTED_EDGE('',*,*,#18879,.T.);
#24532=ORIENTED_EDGE('',*,*,#18886,.T.);
#24533=ORIENTED_EDGE('',*,*,#18876,.T.);
#24534=ORIENTED_EDGE('',*,*,#18887,.T.);
#24535=ORIENTED_EDGE('',*,*,#18869,.T.);
#24536=ORIENTED_EDGE('',*,*,#18888,.T.);
#24537=ORIENTED_EDGE('',*,*,#18874,.T.);
#24538=ORIENTED_EDGE('',*,*,#18889,.T.);
#24539=ORIENTED_EDGE('',*,*,#17731,.T.);
#24540=ORIENTED_EDGE('',*,*,#18890,.T.);
#24541=ORIENTED_EDGE('',*,*,#18873,.T.);
#24542=ORIENTED_EDGE('',*,*,#18891,.T.);
#24543=ORIENTED_EDGE('',*,*,#18871,.T.);
#24544=ORIENTED_EDGE('',*,*,#18892,.T.);
#24545=ORIENTED_EDGE('',*,*,#18870,.T.);
#24546=ORIENTED_EDGE('',*,*,#18893,.T.);
#24547=ORIENTED_EDGE('',*,*,#17729,.T.);
#24548=ORIENTED_EDGE('',*,*,#18894,.T.);
#24549=ORIENTED_EDGE('',*,*,#18868,.T.);
#24550=ORIENTED_EDGE('',*,*,#18895,.T.);
#24551=ORIENTED_EDGE('',*,*,#18883,.F.);
#24552=ORIENTED_EDGE('',*,*,#18887,.F.);
#24553=ORIENTED_EDGE('',*,*,#18877,.F.);
#24554=ORIENTED_EDGE('',*,*,#17726,.F.);
#24555=ORIENTED_EDGE('',*,*,#18878,.F.);
#24556=ORIENTED_EDGE('',*,*,#18888,.F.);
#24557=ORIENTED_EDGE('',*,*,#18894,.F.);
#24558=ORIENTED_EDGE('',*,*,#17728,.F.);
#24559=ORIENTED_EDGE('',*,*,#18884,.F.);
#24560=ORIENTED_EDGE('',*,*,#18893,.F.);
#24561=ORIENTED_EDGE('',*,*,#18889,.F.);
#24562=ORIENTED_EDGE('',*,*,#18886,.F.);
#24563=ORIENTED_EDGE('',*,*,#18896,.F.);
#24564=ORIENTED_EDGE('',*,*,#18897,.F.);
#24565=ORIENTED_EDGE('',*,*,#18898,.F.);
#24566=ORIENTED_EDGE('',*,*,#18899,.T.);
#24567=ORIENTED_EDGE('',*,*,#18900,.T.);
#24568=ORIENTED_EDGE('',*,*,#18897,.T.);
#24569=ORIENTED_EDGE('',*,*,#18901,.T.);
#24570=ORIENTED_EDGE('',*,*,#18902,.T.);
#24571=ORIENTED_EDGE('',*,*,#17739,.T.);
#24572=ORIENTED_EDGE('',*,*,#18903,.T.);
#24573=ORIENTED_EDGE('',*,*,#18898,.T.);
#24574=ORIENTED_EDGE('',*,*,#18904,.T.);
#24575=ORIENTED_EDGE('',*,*,#18905,.F.);
#24576=ORIENTED_EDGE('',*,*,#18906,.F.);
#24577=ORIENTED_EDGE('',*,*,#18907,.F.);
#24578=ORIENTED_EDGE('',*,*,#18908,.T.);
#24579=ORIENTED_EDGE('',*,*,#18909,.T.);
#24580=ORIENTED_EDGE('',*,*,#18906,.T.);
#24581=ORIENTED_EDGE('',*,*,#18910,.T.);
#24582=ORIENTED_EDGE('',*,*,#18911,.T.);
#24583=ORIENTED_EDGE('',*,*,#18896,.T.);
#24584=ORIENTED_EDGE('',*,*,#18912,.T.);
#24585=ORIENTED_EDGE('',*,*,#18907,.T.);
#24586=ORIENTED_EDGE('',*,*,#18913,.T.);
#24587=ORIENTED_EDGE('',*,*,#17737,.T.);
#24588=ORIENTED_EDGE('',*,*,#18914,.T.);
#24589=ORIENTED_EDGE('',*,*,#18905,.T.);
#24590=ORIENTED_EDGE('',*,*,#18915,.T.);
#24591=ORIENTED_EDGE('',*,*,#18899,.F.);
#24592=ORIENTED_EDGE('',*,*,#18916,.T.);
#24593=ORIENTED_EDGE('',*,*,#18917,.T.);
#24594=ORIENTED_EDGE('',*,*,#17733,.T.);
#24595=ORIENTED_EDGE('',*,*,#18918,.T.);
#24596=ORIENTED_EDGE('',*,*,#18901,.F.);
#24597=ORIENTED_EDGE('',*,*,#18913,.F.);
#24598=ORIENTED_EDGE('',*,*,#18909,.F.);
#24599=ORIENTED_EDGE('',*,*,#18919,.F.);
#24600=ORIENTED_EDGE('',*,*,#18902,.F.);
#24601=ORIENTED_EDGE('',*,*,#18919,.T.);
#24602=ORIENTED_EDGE('',*,*,#18908,.F.);
#24603=ORIENTED_EDGE('',*,*,#18920,.F.);
#24604=ORIENTED_EDGE('',*,*,#18921,.T.);
#24605=ORIENTED_EDGE('',*,*,#18916,.F.);
#24606=ORIENTED_EDGE('',*,*,#18911,.F.);
#24607=ORIENTED_EDGE('',*,*,#18922,.T.);
#24608=ORIENTED_EDGE('',*,*,#17735,.T.);
#24609=ORIENTED_EDGE('',*,*,#18923,.T.);
#24610=ORIENTED_EDGE('',*,*,#18920,.T.);
#24611=ORIENTED_EDGE('',*,*,#18910,.F.);
#24612=ORIENTED_EDGE('',*,*,#18914,.F.);
#24613=ORIENTED_EDGE('',*,*,#17736,.F.);
#24614=ORIENTED_EDGE('',*,*,#18922,.F.);
#24615=ORIENTED_EDGE('',*,*,#18900,.F.);
#24616=ORIENTED_EDGE('',*,*,#18918,.F.);
#24617=ORIENTED_EDGE('',*,*,#17732,.F.);
#24618=ORIENTED_EDGE('',*,*,#18904,.F.);
#24619=ORIENTED_EDGE('',*,*,#18924,.F.);
#24620=ORIENTED_EDGE('',*,*,#18925,.F.);
#24621=ORIENTED_EDGE('',*,*,#18926,.F.);
#24622=ORIENTED_EDGE('',*,*,#18927,.F.);
#24623=ORIENTED_EDGE('',*,*,#18928,.F.);
#24624=ORIENTED_EDGE('',*,*,#18929,.F.);
#24625=ORIENTED_EDGE('',*,*,#18930,.F.);
#24626=ORIENTED_EDGE('',*,*,#18931,.F.);
#24627=ORIENTED_EDGE('',*,*,#18932,.F.);
#24628=ORIENTED_EDGE('',*,*,#17743,.T.);
#24629=ORIENTED_EDGE('',*,*,#18933,.T.);
#24630=ORIENTED_EDGE('',*,*,#18931,.T.);
#24631=ORIENTED_EDGE('',*,*,#18934,.T.);
#24632=ORIENTED_EDGE('',*,*,#18935,.F.);
#24633=ORIENTED_EDGE('',*,*,#18936,.F.);
#24634=ORIENTED_EDGE('',*,*,#18937,.F.);
#24635=ORIENTED_EDGE('',*,*,#17741,.T.);
#24636=ORIENTED_EDGE('',*,*,#18938,.T.);
#24637=ORIENTED_EDGE('',*,*,#18936,.T.);
#24638=ORIENTED_EDGE('',*,*,#18939,.T.);
#24639=ORIENTED_EDGE('',*,*,#18928,.T.);
#24640=ORIENTED_EDGE('',*,*,#18940,.T.);
#24641=ORIENTED_EDGE('',*,*,#18937,.T.);
#24642=ORIENTED_EDGE('',*,*,#18941,.T.);
#24643=ORIENTED_EDGE('',*,*,#18935,.T.);
#24644=ORIENTED_EDGE('',*,*,#18942,.T.);
#24645=ORIENTED_EDGE('',*,*,#18932,.T.);
#24646=ORIENTED_EDGE('',*,*,#18943,.T.);
#24647=ORIENTED_EDGE('',*,*,#18925,.T.);
#24648=ORIENTED_EDGE('',*,*,#18944,.T.);
#24649=ORIENTED_EDGE('',*,*,#18930,.T.);
#24650=ORIENTED_EDGE('',*,*,#18945,.T.);
#24651=ORIENTED_EDGE('',*,*,#17747,.T.);
#24652=ORIENTED_EDGE('',*,*,#18946,.T.);
#24653=ORIENTED_EDGE('',*,*,#18929,.T.);
#24654=ORIENTED_EDGE('',*,*,#18947,.T.);
#24655=ORIENTED_EDGE('',*,*,#18927,.T.);
#24656=ORIENTED_EDGE('',*,*,#18948,.T.);
#24657=ORIENTED_EDGE('',*,*,#18926,.T.);
#24658=ORIENTED_EDGE('',*,*,#18949,.T.);
#24659=ORIENTED_EDGE('',*,*,#17745,.T.);
#24660=ORIENTED_EDGE('',*,*,#18950,.T.);
#24661=ORIENTED_EDGE('',*,*,#18924,.T.);
#24662=ORIENTED_EDGE('',*,*,#18951,.T.);
#24663=ORIENTED_EDGE('',*,*,#18939,.F.);
#24664=ORIENTED_EDGE('',*,*,#18943,.F.);
#24665=ORIENTED_EDGE('',*,*,#18933,.F.);
#24666=ORIENTED_EDGE('',*,*,#17742,.F.);
#24667=ORIENTED_EDGE('',*,*,#18934,.F.);
#24668=ORIENTED_EDGE('',*,*,#18944,.F.);
#24669=ORIENTED_EDGE('',*,*,#18950,.F.);
#24670=ORIENTED_EDGE('',*,*,#17744,.F.);
#24671=ORIENTED_EDGE('',*,*,#18940,.F.);
#24672=ORIENTED_EDGE('',*,*,#18949,.F.);
#24673=ORIENTED_EDGE('',*,*,#18945,.F.);
#24674=ORIENTED_EDGE('',*,*,#18942,.F.);
#24675=ORIENTED_EDGE('',*,*,#18952,.F.);
#24676=ORIENTED_EDGE('',*,*,#18953,.F.);
#24677=ORIENTED_EDGE('',*,*,#18954,.F.);
#24678=ORIENTED_EDGE('',*,*,#18955,.F.);
#24679=ORIENTED_EDGE('',*,*,#18956,.F.);
#24680=ORIENTED_EDGE('',*,*,#18957,.F.);
#24681=ORIENTED_EDGE('',*,*,#18958,.F.);
#24682=ORIENTED_EDGE('',*,*,#18959,.F.);
#24683=ORIENTED_EDGE('',*,*,#18960,.F.);
#24684=ORIENTED_EDGE('',*,*,#17751,.T.);
#24685=ORIENTED_EDGE('',*,*,#18961,.T.);
#24686=ORIENTED_EDGE('',*,*,#18959,.T.);
#24687=ORIENTED_EDGE('',*,*,#18962,.T.);
#24688=ORIENTED_EDGE('',*,*,#18963,.F.);
#24689=ORIENTED_EDGE('',*,*,#18964,.F.);
#24690=ORIENTED_EDGE('',*,*,#18965,.F.);
#24691=ORIENTED_EDGE('',*,*,#17749,.T.);
#24692=ORIENTED_EDGE('',*,*,#18966,.T.);
#24693=ORIENTED_EDGE('',*,*,#18964,.T.);
#24694=ORIENTED_EDGE('',*,*,#18967,.T.);
#24695=ORIENTED_EDGE('',*,*,#18956,.T.);
#24696=ORIENTED_EDGE('',*,*,#18968,.T.);
#24697=ORIENTED_EDGE('',*,*,#18965,.T.);
#24698=ORIENTED_EDGE('',*,*,#18969,.T.);
#24699=ORIENTED_EDGE('',*,*,#18963,.T.);
#24700=ORIENTED_EDGE('',*,*,#18970,.T.);
#24701=ORIENTED_EDGE('',*,*,#18960,.T.);
#24702=ORIENTED_EDGE('',*,*,#18971,.T.);
#24703=ORIENTED_EDGE('',*,*,#18953,.T.);
#24704=ORIENTED_EDGE('',*,*,#18972,.T.);
#24705=ORIENTED_EDGE('',*,*,#18958,.T.);
#24706=ORIENTED_EDGE('',*,*,#18973,.T.);
#24707=ORIENTED_EDGE('',*,*,#17755,.T.);
#24708=ORIENTED_EDGE('',*,*,#18974,.T.);
#24709=ORIENTED_EDGE('',*,*,#18957,.T.);
#24710=ORIENTED_EDGE('',*,*,#18975,.T.);
#24711=ORIENTED_EDGE('',*,*,#18955,.T.);
#24712=ORIENTED_EDGE('',*,*,#18976,.T.);
#24713=ORIENTED_EDGE('',*,*,#18954,.T.);
#24714=ORIENTED_EDGE('',*,*,#18977,.T.);
#24715=ORIENTED_EDGE('',*,*,#17753,.T.);
#24716=ORIENTED_EDGE('',*,*,#18978,.T.);
#24717=ORIENTED_EDGE('',*,*,#18952,.T.);
#24718=ORIENTED_EDGE('',*,*,#18979,.T.);
#24719=ORIENTED_EDGE('',*,*,#18967,.F.);
#24720=ORIENTED_EDGE('',*,*,#18971,.F.);
#24721=ORIENTED_EDGE('',*,*,#18961,.F.);
#24722=ORIENTED_EDGE('',*,*,#17750,.F.);
#24723=ORIENTED_EDGE('',*,*,#18962,.F.);
#24724=ORIENTED_EDGE('',*,*,#18972,.F.);
#24725=ORIENTED_EDGE('',*,*,#18978,.F.);
#24726=ORIENTED_EDGE('',*,*,#17752,.F.);
#24727=ORIENTED_EDGE('',*,*,#18968,.F.);
#24728=ORIENTED_EDGE('',*,*,#18977,.F.);
#24729=ORIENTED_EDGE('',*,*,#18973,.F.);
#24730=ORIENTED_EDGE('',*,*,#18970,.F.);
#24731=ORIENTED_EDGE('',*,*,#18980,.T.);
#24732=ORIENTED_EDGE('',*,*,#18981,.T.);
#24733=ORIENTED_EDGE('',*,*,#17761,.T.);
#24734=ORIENTED_EDGE('',*,*,#18982,.T.);
#24735=ORIENTED_EDGE('',*,*,#18983,.T.);
#24736=ORIENTED_EDGE('',*,*,#18981,.F.);
#24737=ORIENTED_EDGE('',*,*,#18984,.F.);
#24738=ORIENTED_EDGE('',*,*,#18985,.F.);
#24739=ORIENTED_EDGE('',*,*,#17762,.F.);
#24740=ORIENTED_EDGE('',*,*,#18980,.F.);
#24741=ORIENTED_EDGE('',*,*,#18986,.F.);
#24742=ORIENTED_EDGE('',*,*,#18987,.T.);
#24743=ORIENTED_EDGE('',*,*,#18988,.T.);
#24744=ORIENTED_EDGE('',*,*,#18984,.T.);
#24745=ORIENTED_EDGE('',*,*,#18983,.F.);
#24746=ORIENTED_EDGE('',*,*,#18989,.T.);
#24747=ORIENTED_EDGE('',*,*,#18990,.T.);
#24748=ORIENTED_EDGE('',*,*,#18991,.T.);
#24749=ORIENTED_EDGE('',*,*,#18986,.T.);
#24750=ORIENTED_EDGE('',*,*,#18988,.F.);
#24751=ORIENTED_EDGE('',*,*,#18992,.F.);
#24752=ORIENTED_EDGE('',*,*,#18993,.F.);
#24753=ORIENTED_EDGE('',*,*,#18990,.F.);
#24754=ORIENTED_EDGE('',*,*,#18994,.F.);
#24755=ORIENTED_EDGE('',*,*,#18995,.F.);
#24756=ORIENTED_EDGE('',*,*,#17759,.T.);
#24757=ORIENTED_EDGE('',*,*,#18996,.T.);
#24758=ORIENTED_EDGE('',*,*,#18994,.T.);
#24759=ORIENTED_EDGE('',*,*,#18997,.T.);
#24760=ORIENTED_EDGE('',*,*,#18998,.F.);
#24761=ORIENTED_EDGE('',*,*,#18999,.F.);
#24762=ORIENTED_EDGE('',*,*,#19000,.F.);
#24763=ORIENTED_EDGE('',*,*,#17757,.T.);
#24764=ORIENTED_EDGE('',*,*,#19001,.T.);
#24765=ORIENTED_EDGE('',*,*,#18999,.T.);
#24766=ORIENTED_EDGE('',*,*,#19002,.T.);
#24767=ORIENTED_EDGE('',*,*,#18992,.T.);
#24768=ORIENTED_EDGE('',*,*,#19003,.T.);
#24769=ORIENTED_EDGE('',*,*,#19000,.T.);
#24770=ORIENTED_EDGE('',*,*,#19004,.T.);
#24771=ORIENTED_EDGE('',*,*,#18998,.T.);
#24772=ORIENTED_EDGE('',*,*,#19005,.T.);
#24773=ORIENTED_EDGE('',*,*,#18995,.T.);
#24774=ORIENTED_EDGE('',*,*,#19006,.T.);
#24775=ORIENTED_EDGE('',*,*,#17763,.T.);
#24776=ORIENTED_EDGE('',*,*,#18985,.T.);
#24777=ORIENTED_EDGE('',*,*,#18993,.T.);
#24778=ORIENTED_EDGE('',*,*,#19007,.T.);
#24779=ORIENTED_EDGE('',*,*,#18982,.F.);
#24780=ORIENTED_EDGE('',*,*,#17760,.F.);
#24781=ORIENTED_EDGE('',*,*,#18997,.F.);
#24782=ORIENTED_EDGE('',*,*,#18989,.F.);
#24783=ORIENTED_EDGE('',*,*,#19003,.F.);
#24784=ORIENTED_EDGE('',*,*,#18987,.F.);
#24785=ORIENTED_EDGE('',*,*,#18991,.F.);
#24786=ORIENTED_EDGE('',*,*,#19005,.F.);
#24787=ORIENTED_EDGE('',*,*,#19008,.F.);
#24788=ORIENTED_EDGE('',*,*,#19009,.F.);
#24789=ORIENTED_EDGE('',*,*,#19010,.F.);
#24790=ORIENTED_EDGE('',*,*,#19011,.F.);
#24791=ORIENTED_EDGE('',*,*,#19012,.F.);
#24792=ORIENTED_EDGE('',*,*,#19013,.F.);
#24793=ORIENTED_EDGE('',*,*,#19014,.F.);
#24794=ORIENTED_EDGE('',*,*,#19015,.F.);
#24795=ORIENTED_EDGE('',*,*,#19016,.F.);
#24796=ORIENTED_EDGE('',*,*,#17767,.T.);
#24797=ORIENTED_EDGE('',*,*,#19017,.T.);
#24798=ORIENTED_EDGE('',*,*,#19015,.T.);
#24799=ORIENTED_EDGE('',*,*,#19018,.T.);
#24800=ORIENTED_EDGE('',*,*,#19019,.F.);
#24801=ORIENTED_EDGE('',*,*,#19020,.F.);
#24802=ORIENTED_EDGE('',*,*,#19021,.F.);
#24803=ORIENTED_EDGE('',*,*,#17765,.T.);
#24804=ORIENTED_EDGE('',*,*,#19022,.T.);
#24805=ORIENTED_EDGE('',*,*,#19020,.T.);
#24806=ORIENTED_EDGE('',*,*,#19023,.T.);
#24807=ORIENTED_EDGE('',*,*,#19012,.T.);
#24808=ORIENTED_EDGE('',*,*,#19024,.T.);
#24809=ORIENTED_EDGE('',*,*,#19021,.T.);
#24810=ORIENTED_EDGE('',*,*,#19025,.T.);
#24811=ORIENTED_EDGE('',*,*,#19019,.T.);
#24812=ORIENTED_EDGE('',*,*,#19026,.T.);
#24813=ORIENTED_EDGE('',*,*,#19016,.T.);
#24814=ORIENTED_EDGE('',*,*,#19027,.T.);
#24815=ORIENTED_EDGE('',*,*,#19009,.T.);
#24816=ORIENTED_EDGE('',*,*,#19028,.T.);
#24817=ORIENTED_EDGE('',*,*,#19014,.T.);
#24818=ORIENTED_EDGE('',*,*,#19029,.T.);
#24819=ORIENTED_EDGE('',*,*,#17771,.T.);
#24820=ORIENTED_EDGE('',*,*,#19030,.T.);
#24821=ORIENTED_EDGE('',*,*,#19013,.T.);
#24822=ORIENTED_EDGE('',*,*,#19031,.T.);
#24823=ORIENTED_EDGE('',*,*,#19011,.T.);
#24824=ORIENTED_EDGE('',*,*,#19032,.T.);
#24825=ORIENTED_EDGE('',*,*,#19010,.T.);
#24826=ORIENTED_EDGE('',*,*,#19033,.T.);
#24827=ORIENTED_EDGE('',*,*,#17769,.T.);
#24828=ORIENTED_EDGE('',*,*,#19034,.T.);
#24829=ORIENTED_EDGE('',*,*,#19008,.T.);
#24830=ORIENTED_EDGE('',*,*,#19035,.T.);
#24831=ORIENTED_EDGE('',*,*,#19023,.F.);
#24832=ORIENTED_EDGE('',*,*,#19027,.F.);
#24833=ORIENTED_EDGE('',*,*,#19017,.F.);
#24834=ORIENTED_EDGE('',*,*,#17766,.F.);
#24835=ORIENTED_EDGE('',*,*,#19018,.F.);
#24836=ORIENTED_EDGE('',*,*,#19028,.F.);
#24837=ORIENTED_EDGE('',*,*,#19034,.F.);
#24838=ORIENTED_EDGE('',*,*,#17768,.F.);
#24839=ORIENTED_EDGE('',*,*,#19024,.F.);
#24840=ORIENTED_EDGE('',*,*,#19033,.F.);
#24841=ORIENTED_EDGE('',*,*,#19029,.F.);
#24842=ORIENTED_EDGE('',*,*,#19026,.F.);
#24843=ORIENTED_EDGE('',*,*,#19036,.F.);
#24844=ORIENTED_EDGE('',*,*,#19037,.F.);
#24845=ORIENTED_EDGE('',*,*,#19038,.F.);
#24846=ORIENTED_EDGE('',*,*,#19039,.T.);
#24847=ORIENTED_EDGE('',*,*,#19040,.T.);
#24848=ORIENTED_EDGE('',*,*,#19037,.T.);
#24849=ORIENTED_EDGE('',*,*,#19041,.T.);
#24850=ORIENTED_EDGE('',*,*,#19042,.T.);
#24851=ORIENTED_EDGE('',*,*,#17779,.T.);
#24852=ORIENTED_EDGE('',*,*,#19043,.T.);
#24853=ORIENTED_EDGE('',*,*,#19038,.T.);
#24854=ORIENTED_EDGE('',*,*,#19044,.T.);
#24855=ORIENTED_EDGE('',*,*,#19045,.F.);
#24856=ORIENTED_EDGE('',*,*,#19046,.F.);
#24857=ORIENTED_EDGE('',*,*,#19047,.F.);
#24858=ORIENTED_EDGE('',*,*,#19048,.T.);
#24859=ORIENTED_EDGE('',*,*,#19049,.T.);
#24860=ORIENTED_EDGE('',*,*,#19046,.T.);
#24861=ORIENTED_EDGE('',*,*,#19050,.T.);
#24862=ORIENTED_EDGE('',*,*,#19051,.T.);
#24863=ORIENTED_EDGE('',*,*,#19036,.T.);
#24864=ORIENTED_EDGE('',*,*,#19052,.T.);
#24865=ORIENTED_EDGE('',*,*,#19047,.T.);
#24866=ORIENTED_EDGE('',*,*,#19053,.T.);
#24867=ORIENTED_EDGE('',*,*,#17777,.T.);
#24868=ORIENTED_EDGE('',*,*,#19054,.T.);
#24869=ORIENTED_EDGE('',*,*,#19045,.T.);
#24870=ORIENTED_EDGE('',*,*,#19055,.T.);
#24871=ORIENTED_EDGE('',*,*,#19039,.F.);
#24872=ORIENTED_EDGE('',*,*,#19056,.T.);
#24873=ORIENTED_EDGE('',*,*,#19057,.T.);
#24874=ORIENTED_EDGE('',*,*,#17773,.T.);
#24875=ORIENTED_EDGE('',*,*,#19058,.T.);
#24876=ORIENTED_EDGE('',*,*,#19041,.F.);
#24877=ORIENTED_EDGE('',*,*,#19053,.F.);
#24878=ORIENTED_EDGE('',*,*,#19049,.F.);
#24879=ORIENTED_EDGE('',*,*,#19059,.F.);
#24880=ORIENTED_EDGE('',*,*,#19042,.F.);
#24881=ORIENTED_EDGE('',*,*,#19059,.T.);
#24882=ORIENTED_EDGE('',*,*,#19048,.F.);
#24883=ORIENTED_EDGE('',*,*,#19060,.F.);
#24884=ORIENTED_EDGE('',*,*,#19061,.T.);
#24885=ORIENTED_EDGE('',*,*,#19056,.F.);
#24886=ORIENTED_EDGE('',*,*,#19051,.F.);
#24887=ORIENTED_EDGE('',*,*,#19062,.T.);
#24888=ORIENTED_EDGE('',*,*,#17775,.T.);
#24889=ORIENTED_EDGE('',*,*,#19063,.T.);
#24890=ORIENTED_EDGE('',*,*,#19060,.T.);
#24891=ORIENTED_EDGE('',*,*,#19050,.F.);
#24892=ORIENTED_EDGE('',*,*,#19054,.F.);
#24893=ORIENTED_EDGE('',*,*,#17776,.F.);
#24894=ORIENTED_EDGE('',*,*,#19062,.F.);
#24895=ORIENTED_EDGE('',*,*,#19040,.F.);
#24896=ORIENTED_EDGE('',*,*,#19058,.F.);
#24897=ORIENTED_EDGE('',*,*,#17772,.F.);
#24898=ORIENTED_EDGE('',*,*,#19044,.F.);
#24899=ORIENTED_EDGE('',*,*,#19064,.F.);
#24900=ORIENTED_EDGE('',*,*,#19065,.F.);
#24901=ORIENTED_EDGE('',*,*,#19066,.F.);
#24902=ORIENTED_EDGE('',*,*,#19067,.F.);
#24903=ORIENTED_EDGE('',*,*,#19068,.F.);
#24904=ORIENTED_EDGE('',*,*,#19069,.F.);
#24905=ORIENTED_EDGE('',*,*,#19070,.F.);
#24906=ORIENTED_EDGE('',*,*,#19071,.F.);
#24907=ORIENTED_EDGE('',*,*,#19072,.F.);
#24908=ORIENTED_EDGE('',*,*,#17783,.T.);
#24909=ORIENTED_EDGE('',*,*,#19073,.T.);
#24910=ORIENTED_EDGE('',*,*,#19071,.T.);
#24911=ORIENTED_EDGE('',*,*,#19074,.T.);
#24912=ORIENTED_EDGE('',*,*,#19075,.F.);
#24913=ORIENTED_EDGE('',*,*,#19076,.F.);
#24914=ORIENTED_EDGE('',*,*,#19077,.F.);
#24915=ORIENTED_EDGE('',*,*,#17781,.T.);
#24916=ORIENTED_EDGE('',*,*,#19078,.T.);
#24917=ORIENTED_EDGE('',*,*,#19076,.T.);
#24918=ORIENTED_EDGE('',*,*,#19079,.T.);
#24919=ORIENTED_EDGE('',*,*,#19068,.T.);
#24920=ORIENTED_EDGE('',*,*,#19080,.T.);
#24921=ORIENTED_EDGE('',*,*,#19077,.T.);
#24922=ORIENTED_EDGE('',*,*,#19081,.T.);
#24923=ORIENTED_EDGE('',*,*,#19075,.T.);
#24924=ORIENTED_EDGE('',*,*,#19082,.T.);
#24925=ORIENTED_EDGE('',*,*,#19072,.T.);
#24926=ORIENTED_EDGE('',*,*,#19083,.T.);
#24927=ORIENTED_EDGE('',*,*,#19065,.T.);
#24928=ORIENTED_EDGE('',*,*,#19084,.T.);
#24929=ORIENTED_EDGE('',*,*,#19070,.T.);
#24930=ORIENTED_EDGE('',*,*,#19085,.T.);
#24931=ORIENTED_EDGE('',*,*,#17787,.T.);
#24932=ORIENTED_EDGE('',*,*,#19086,.T.);
#24933=ORIENTED_EDGE('',*,*,#19069,.T.);
#24934=ORIENTED_EDGE('',*,*,#19087,.T.);
#24935=ORIENTED_EDGE('',*,*,#19067,.T.);
#24936=ORIENTED_EDGE('',*,*,#19088,.T.);
#24937=ORIENTED_EDGE('',*,*,#19066,.T.);
#24938=ORIENTED_EDGE('',*,*,#19089,.T.);
#24939=ORIENTED_EDGE('',*,*,#17785,.T.);
#24940=ORIENTED_EDGE('',*,*,#19090,.T.);
#24941=ORIENTED_EDGE('',*,*,#19064,.T.);
#24942=ORIENTED_EDGE('',*,*,#19091,.T.);
#24943=ORIENTED_EDGE('',*,*,#19079,.F.);
#24944=ORIENTED_EDGE('',*,*,#19083,.F.);
#24945=ORIENTED_EDGE('',*,*,#19073,.F.);
#24946=ORIENTED_EDGE('',*,*,#17782,.F.);
#24947=ORIENTED_EDGE('',*,*,#19074,.F.);
#24948=ORIENTED_EDGE('',*,*,#19084,.F.);
#24949=ORIENTED_EDGE('',*,*,#19090,.F.);
#24950=ORIENTED_EDGE('',*,*,#17784,.F.);
#24951=ORIENTED_EDGE('',*,*,#19080,.F.);
#24952=ORIENTED_EDGE('',*,*,#19089,.F.);
#24953=ORIENTED_EDGE('',*,*,#19085,.F.);
#24954=ORIENTED_EDGE('',*,*,#19082,.F.);
#24955=ORIENTED_EDGE('',*,*,#19092,.F.);
#24956=ORIENTED_EDGE('',*,*,#19093,.F.);
#24957=ORIENTED_EDGE('',*,*,#19094,.F.);
#24958=ORIENTED_EDGE('',*,*,#19095,.F.);
#24959=ORIENTED_EDGE('',*,*,#19096,.F.);
#24960=ORIENTED_EDGE('',*,*,#19097,.F.);
#24961=ORIENTED_EDGE('',*,*,#19098,.F.);
#24962=ORIENTED_EDGE('',*,*,#19099,.F.);
#24963=ORIENTED_EDGE('',*,*,#19100,.F.);
#24964=ORIENTED_EDGE('',*,*,#17791,.T.);
#24965=ORIENTED_EDGE('',*,*,#19101,.T.);
#24966=ORIENTED_EDGE('',*,*,#19099,.T.);
#24967=ORIENTED_EDGE('',*,*,#19102,.T.);
#24968=ORIENTED_EDGE('',*,*,#19103,.F.);
#24969=ORIENTED_EDGE('',*,*,#19104,.F.);
#24970=ORIENTED_EDGE('',*,*,#19105,.F.);
#24971=ORIENTED_EDGE('',*,*,#17789,.T.);
#24972=ORIENTED_EDGE('',*,*,#19106,.T.);
#24973=ORIENTED_EDGE('',*,*,#19104,.T.);
#24974=ORIENTED_EDGE('',*,*,#19107,.T.);
#24975=ORIENTED_EDGE('',*,*,#19096,.T.);
#24976=ORIENTED_EDGE('',*,*,#19108,.T.);
#24977=ORIENTED_EDGE('',*,*,#19105,.T.);
#24978=ORIENTED_EDGE('',*,*,#19109,.T.);
#24979=ORIENTED_EDGE('',*,*,#19103,.T.);
#24980=ORIENTED_EDGE('',*,*,#19110,.T.);
#24981=ORIENTED_EDGE('',*,*,#19100,.T.);
#24982=ORIENTED_EDGE('',*,*,#19111,.T.);
#24983=ORIENTED_EDGE('',*,*,#19093,.T.);
#24984=ORIENTED_EDGE('',*,*,#19112,.T.);
#24985=ORIENTED_EDGE('',*,*,#19098,.T.);
#24986=ORIENTED_EDGE('',*,*,#19113,.T.);
#24987=ORIENTED_EDGE('',*,*,#17795,.T.);
#24988=ORIENTED_EDGE('',*,*,#19114,.T.);
#24989=ORIENTED_EDGE('',*,*,#19097,.T.);
#24990=ORIENTED_EDGE('',*,*,#19115,.T.);
#24991=ORIENTED_EDGE('',*,*,#19095,.T.);
#24992=ORIENTED_EDGE('',*,*,#19116,.T.);
#24993=ORIENTED_EDGE('',*,*,#19094,.T.);
#24994=ORIENTED_EDGE('',*,*,#19117,.T.);
#24995=ORIENTED_EDGE('',*,*,#17793,.T.);
#24996=ORIENTED_EDGE('',*,*,#19118,.T.);
#24997=ORIENTED_EDGE('',*,*,#19092,.T.);
#24998=ORIENTED_EDGE('',*,*,#19119,.T.);
#24999=ORIENTED_EDGE('',*,*,#19107,.F.);
#25000=ORIENTED_EDGE('',*,*,#19111,.F.);
#25001=ORIENTED_EDGE('',*,*,#19101,.F.);
#25002=ORIENTED_EDGE('',*,*,#17790,.F.);
#25003=ORIENTED_EDGE('',*,*,#19102,.F.);
#25004=ORIENTED_EDGE('',*,*,#19112,.F.);
#25005=ORIENTED_EDGE('',*,*,#19118,.F.);
#25006=ORIENTED_EDGE('',*,*,#17792,.F.);
#25007=ORIENTED_EDGE('',*,*,#19108,.F.);
#25008=ORIENTED_EDGE('',*,*,#19117,.F.);
#25009=ORIENTED_EDGE('',*,*,#19113,.F.);
#25010=ORIENTED_EDGE('',*,*,#19110,.F.);
#25011=ORIENTED_EDGE('',*,*,#19120,.T.);
#25012=ORIENTED_EDGE('',*,*,#19121,.T.);
#25013=ORIENTED_EDGE('',*,*,#17801,.T.);
#25014=ORIENTED_EDGE('',*,*,#19122,.T.);
#25015=ORIENTED_EDGE('',*,*,#19123,.T.);
#25016=ORIENTED_EDGE('',*,*,#19121,.F.);
#25017=ORIENTED_EDGE('',*,*,#19124,.F.);
#25018=ORIENTED_EDGE('',*,*,#19125,.F.);
#25019=ORIENTED_EDGE('',*,*,#17802,.F.);
#25020=ORIENTED_EDGE('',*,*,#19120,.F.);
#25021=ORIENTED_EDGE('',*,*,#19126,.F.);
#25022=ORIENTED_EDGE('',*,*,#19127,.T.);
#25023=ORIENTED_EDGE('',*,*,#19128,.T.);
#25024=ORIENTED_EDGE('',*,*,#19124,.T.);
#25025=ORIENTED_EDGE('',*,*,#19123,.F.);
#25026=ORIENTED_EDGE('',*,*,#19129,.T.);
#25027=ORIENTED_EDGE('',*,*,#19130,.T.);
#25028=ORIENTED_EDGE('',*,*,#19131,.T.);
#25029=ORIENTED_EDGE('',*,*,#19126,.T.);
#25030=ORIENTED_EDGE('',*,*,#19128,.F.);
#25031=ORIENTED_EDGE('',*,*,#19132,.F.);
#25032=ORIENTED_EDGE('',*,*,#19133,.F.);
#25033=ORIENTED_EDGE('',*,*,#19130,.F.);
#25034=ORIENTED_EDGE('',*,*,#19134,.F.);
#25035=ORIENTED_EDGE('',*,*,#19135,.F.);
#25036=ORIENTED_EDGE('',*,*,#17799,.T.);
#25037=ORIENTED_EDGE('',*,*,#19136,.T.);
#25038=ORIENTED_EDGE('',*,*,#19134,.T.);
#25039=ORIENTED_EDGE('',*,*,#19137,.T.);
#25040=ORIENTED_EDGE('',*,*,#19138,.F.);
#25041=ORIENTED_EDGE('',*,*,#19139,.F.);
#25042=ORIENTED_EDGE('',*,*,#19140,.F.);
#25043=ORIENTED_EDGE('',*,*,#17797,.T.);
#25044=ORIENTED_EDGE('',*,*,#19141,.T.);
#25045=ORIENTED_EDGE('',*,*,#19139,.T.);
#25046=ORIENTED_EDGE('',*,*,#19142,.T.);
#25047=ORIENTED_EDGE('',*,*,#19132,.T.);
#25048=ORIENTED_EDGE('',*,*,#19143,.T.);
#25049=ORIENTED_EDGE('',*,*,#19140,.T.);
#25050=ORIENTED_EDGE('',*,*,#19144,.T.);
#25051=ORIENTED_EDGE('',*,*,#19138,.T.);
#25052=ORIENTED_EDGE('',*,*,#19145,.T.);
#25053=ORIENTED_EDGE('',*,*,#19135,.T.);
#25054=ORIENTED_EDGE('',*,*,#19146,.T.);
#25055=ORIENTED_EDGE('',*,*,#17803,.T.);
#25056=ORIENTED_EDGE('',*,*,#19125,.T.);
#25057=ORIENTED_EDGE('',*,*,#19133,.T.);
#25058=ORIENTED_EDGE('',*,*,#19147,.T.);
#25059=ORIENTED_EDGE('',*,*,#19122,.F.);
#25060=ORIENTED_EDGE('',*,*,#17800,.F.);
#25061=ORIENTED_EDGE('',*,*,#19137,.F.);
#25062=ORIENTED_EDGE('',*,*,#19129,.F.);
#25063=ORIENTED_EDGE('',*,*,#19143,.F.);
#25064=ORIENTED_EDGE('',*,*,#19127,.F.);
#25065=ORIENTED_EDGE('',*,*,#19131,.F.);
#25066=ORIENTED_EDGE('',*,*,#19145,.F.);
#25067=ORIENTED_EDGE('',*,*,#19148,.F.);
#25068=ORIENTED_EDGE('',*,*,#19149,.F.);
#25069=ORIENTED_EDGE('',*,*,#19150,.F.);
#25070=ORIENTED_EDGE('',*,*,#19151,.F.);
#25071=ORIENTED_EDGE('',*,*,#19152,.F.);
#25072=ORIENTED_EDGE('',*,*,#19153,.F.);
#25073=ORIENTED_EDGE('',*,*,#19154,.F.);
#25074=ORIENTED_EDGE('',*,*,#19155,.F.);
#25075=ORIENTED_EDGE('',*,*,#19156,.F.);
#25076=ORIENTED_EDGE('',*,*,#17807,.T.);
#25077=ORIENTED_EDGE('',*,*,#19157,.T.);
#25078=ORIENTED_EDGE('',*,*,#19155,.T.);
#25079=ORIENTED_EDGE('',*,*,#19158,.T.);
#25080=ORIENTED_EDGE('',*,*,#19159,.F.);
#25081=ORIENTED_EDGE('',*,*,#19160,.F.);
#25082=ORIENTED_EDGE('',*,*,#19161,.F.);
#25083=ORIENTED_EDGE('',*,*,#17805,.T.);
#25084=ORIENTED_EDGE('',*,*,#19162,.T.);
#25085=ORIENTED_EDGE('',*,*,#19160,.T.);
#25086=ORIENTED_EDGE('',*,*,#19163,.T.);
#25087=ORIENTED_EDGE('',*,*,#19152,.T.);
#25088=ORIENTED_EDGE('',*,*,#19164,.T.);
#25089=ORIENTED_EDGE('',*,*,#19161,.T.);
#25090=ORIENTED_EDGE('',*,*,#19165,.T.);
#25091=ORIENTED_EDGE('',*,*,#19159,.T.);
#25092=ORIENTED_EDGE('',*,*,#19166,.T.);
#25093=ORIENTED_EDGE('',*,*,#19156,.T.);
#25094=ORIENTED_EDGE('',*,*,#19167,.T.);
#25095=ORIENTED_EDGE('',*,*,#19149,.T.);
#25096=ORIENTED_EDGE('',*,*,#19168,.T.);
#25097=ORIENTED_EDGE('',*,*,#19154,.T.);
#25098=ORIENTED_EDGE('',*,*,#19169,.T.);
#25099=ORIENTED_EDGE('',*,*,#17811,.T.);
#25100=ORIENTED_EDGE('',*,*,#19170,.T.);
#25101=ORIENTED_EDGE('',*,*,#19153,.T.);
#25102=ORIENTED_EDGE('',*,*,#19171,.T.);
#25103=ORIENTED_EDGE('',*,*,#19151,.T.);
#25104=ORIENTED_EDGE('',*,*,#19172,.T.);
#25105=ORIENTED_EDGE('',*,*,#19150,.T.);
#25106=ORIENTED_EDGE('',*,*,#19173,.T.);
#25107=ORIENTED_EDGE('',*,*,#17809,.T.);
#25108=ORIENTED_EDGE('',*,*,#19174,.T.);
#25109=ORIENTED_EDGE('',*,*,#19148,.T.);
#25110=ORIENTED_EDGE('',*,*,#19175,.T.);
#25111=ORIENTED_EDGE('',*,*,#19163,.F.);
#25112=ORIENTED_EDGE('',*,*,#19167,.F.);
#25113=ORIENTED_EDGE('',*,*,#19157,.F.);
#25114=ORIENTED_EDGE('',*,*,#17806,.F.);
#25115=ORIENTED_EDGE('',*,*,#19158,.F.);
#25116=ORIENTED_EDGE('',*,*,#19168,.F.);
#25117=ORIENTED_EDGE('',*,*,#19174,.F.);
#25118=ORIENTED_EDGE('',*,*,#17808,.F.);
#25119=ORIENTED_EDGE('',*,*,#19164,.F.);
#25120=ORIENTED_EDGE('',*,*,#19173,.F.);
#25121=ORIENTED_EDGE('',*,*,#19169,.F.);
#25122=ORIENTED_EDGE('',*,*,#19166,.F.);
#25123=ORIENTED_EDGE('',*,*,#19176,.F.);
#25124=ORIENTED_EDGE('',*,*,#19177,.F.);
#25125=ORIENTED_EDGE('',*,*,#19178,.F.);
#25126=ORIENTED_EDGE('',*,*,#19179,.T.);
#25127=ORIENTED_EDGE('',*,*,#19180,.T.);
#25128=ORIENTED_EDGE('',*,*,#19177,.T.);
#25129=ORIENTED_EDGE('',*,*,#19181,.T.);
#25130=ORIENTED_EDGE('',*,*,#19182,.T.);
#25131=ORIENTED_EDGE('',*,*,#17819,.T.);
#25132=ORIENTED_EDGE('',*,*,#19183,.T.);
#25133=ORIENTED_EDGE('',*,*,#19178,.T.);
#25134=ORIENTED_EDGE('',*,*,#19184,.T.);
#25135=ORIENTED_EDGE('',*,*,#19185,.F.);
#25136=ORIENTED_EDGE('',*,*,#19186,.F.);
#25137=ORIENTED_EDGE('',*,*,#19187,.F.);
#25138=ORIENTED_EDGE('',*,*,#19188,.T.);
#25139=ORIENTED_EDGE('',*,*,#19189,.T.);
#25140=ORIENTED_EDGE('',*,*,#19186,.T.);
#25141=ORIENTED_EDGE('',*,*,#19190,.T.);
#25142=ORIENTED_EDGE('',*,*,#19191,.T.);
#25143=ORIENTED_EDGE('',*,*,#19176,.T.);
#25144=ORIENTED_EDGE('',*,*,#19192,.T.);
#25145=ORIENTED_EDGE('',*,*,#19187,.T.);
#25146=ORIENTED_EDGE('',*,*,#19193,.T.);
#25147=ORIENTED_EDGE('',*,*,#17817,.T.);
#25148=ORIENTED_EDGE('',*,*,#19194,.T.);
#25149=ORIENTED_EDGE('',*,*,#19185,.T.);
#25150=ORIENTED_EDGE('',*,*,#19195,.T.);
#25151=ORIENTED_EDGE('',*,*,#19179,.F.);
#25152=ORIENTED_EDGE('',*,*,#19196,.T.);
#25153=ORIENTED_EDGE('',*,*,#19197,.T.);
#25154=ORIENTED_EDGE('',*,*,#17813,.T.);
#25155=ORIENTED_EDGE('',*,*,#19198,.T.);
#25156=ORIENTED_EDGE('',*,*,#19181,.F.);
#25157=ORIENTED_EDGE('',*,*,#19193,.F.);
#25158=ORIENTED_EDGE('',*,*,#19189,.F.);
#25159=ORIENTED_EDGE('',*,*,#19199,.F.);
#25160=ORIENTED_EDGE('',*,*,#19182,.F.);
#25161=ORIENTED_EDGE('',*,*,#19199,.T.);
#25162=ORIENTED_EDGE('',*,*,#19188,.F.);
#25163=ORIENTED_EDGE('',*,*,#19200,.F.);
#25164=ORIENTED_EDGE('',*,*,#19201,.T.);
#25165=ORIENTED_EDGE('',*,*,#19196,.F.);
#25166=ORIENTED_EDGE('',*,*,#19191,.F.);
#25167=ORIENTED_EDGE('',*,*,#19202,.T.);
#25168=ORIENTED_EDGE('',*,*,#17815,.T.);
#25169=ORIENTED_EDGE('',*,*,#19203,.T.);
#25170=ORIENTED_EDGE('',*,*,#19200,.T.);
#25171=ORIENTED_EDGE('',*,*,#19190,.F.);
#25172=ORIENTED_EDGE('',*,*,#19194,.F.);
#25173=ORIENTED_EDGE('',*,*,#17816,.F.);
#25174=ORIENTED_EDGE('',*,*,#19202,.F.);
#25175=ORIENTED_EDGE('',*,*,#19180,.F.);
#25176=ORIENTED_EDGE('',*,*,#19198,.F.);
#25177=ORIENTED_EDGE('',*,*,#17812,.F.);
#25178=ORIENTED_EDGE('',*,*,#19184,.F.);
#25179=ORIENTED_EDGE('',*,*,#19204,.F.);
#25180=ORIENTED_EDGE('',*,*,#19205,.F.);
#25181=ORIENTED_EDGE('',*,*,#19206,.F.);
#25182=ORIENTED_EDGE('',*,*,#19207,.F.);
#25183=ORIENTED_EDGE('',*,*,#19208,.F.);
#25184=ORIENTED_EDGE('',*,*,#19209,.F.);
#25185=ORIENTED_EDGE('',*,*,#19210,.F.);
#25186=ORIENTED_EDGE('',*,*,#19211,.F.);
#25187=ORIENTED_EDGE('',*,*,#19212,.F.);
#25188=ORIENTED_EDGE('',*,*,#17823,.T.);
#25189=ORIENTED_EDGE('',*,*,#19213,.T.);
#25190=ORIENTED_EDGE('',*,*,#19211,.T.);
#25191=ORIENTED_EDGE('',*,*,#19214,.T.);
#25192=ORIENTED_EDGE('',*,*,#19215,.F.);
#25193=ORIENTED_EDGE('',*,*,#19216,.F.);
#25194=ORIENTED_EDGE('',*,*,#19217,.F.);
#25195=ORIENTED_EDGE('',*,*,#17821,.T.);
#25196=ORIENTED_EDGE('',*,*,#19218,.T.);
#25197=ORIENTED_EDGE('',*,*,#19216,.T.);
#25198=ORIENTED_EDGE('',*,*,#19219,.T.);
#25199=ORIENTED_EDGE('',*,*,#19208,.T.);
#25200=ORIENTED_EDGE('',*,*,#19220,.T.);
#25201=ORIENTED_EDGE('',*,*,#19217,.T.);
#25202=ORIENTED_EDGE('',*,*,#19221,.T.);
#25203=ORIENTED_EDGE('',*,*,#19215,.T.);
#25204=ORIENTED_EDGE('',*,*,#19222,.T.);
#25205=ORIENTED_EDGE('',*,*,#19212,.T.);
#25206=ORIENTED_EDGE('',*,*,#19223,.T.);
#25207=ORIENTED_EDGE('',*,*,#19205,.T.);
#25208=ORIENTED_EDGE('',*,*,#19224,.T.);
#25209=ORIENTED_EDGE('',*,*,#19210,.T.);
#25210=ORIENTED_EDGE('',*,*,#19225,.T.);
#25211=ORIENTED_EDGE('',*,*,#17827,.T.);
#25212=ORIENTED_EDGE('',*,*,#19226,.T.);
#25213=ORIENTED_EDGE('',*,*,#19209,.T.);
#25214=ORIENTED_EDGE('',*,*,#19227,.T.);
#25215=ORIENTED_EDGE('',*,*,#19207,.T.);
#25216=ORIENTED_EDGE('',*,*,#19228,.T.);
#25217=ORIENTED_EDGE('',*,*,#19206,.T.);
#25218=ORIENTED_EDGE('',*,*,#19229,.T.);
#25219=ORIENTED_EDGE('',*,*,#17825,.T.);
#25220=ORIENTED_EDGE('',*,*,#19230,.T.);
#25221=ORIENTED_EDGE('',*,*,#19204,.T.);
#25222=ORIENTED_EDGE('',*,*,#19231,.T.);
#25223=ORIENTED_EDGE('',*,*,#19219,.F.);
#25224=ORIENTED_EDGE('',*,*,#19223,.F.);
#25225=ORIENTED_EDGE('',*,*,#19213,.F.);
#25226=ORIENTED_EDGE('',*,*,#17822,.F.);
#25227=ORIENTED_EDGE('',*,*,#19214,.F.);
#25228=ORIENTED_EDGE('',*,*,#19224,.F.);
#25229=ORIENTED_EDGE('',*,*,#19230,.F.);
#25230=ORIENTED_EDGE('',*,*,#17824,.F.);
#25231=ORIENTED_EDGE('',*,*,#19220,.F.);
#25232=ORIENTED_EDGE('',*,*,#19229,.F.);
#25233=ORIENTED_EDGE('',*,*,#19225,.F.);
#25234=ORIENTED_EDGE('',*,*,#19222,.F.);
#25235=ORIENTED_EDGE('',*,*,#19232,.F.);
#25236=ORIENTED_EDGE('',*,*,#19233,.F.);
#25237=ORIENTED_EDGE('',*,*,#19234,.F.);
#25238=ORIENTED_EDGE('',*,*,#19235,.F.);
#25239=ORIENTED_EDGE('',*,*,#19236,.F.);
#25240=ORIENTED_EDGE('',*,*,#19237,.F.);
#25241=ORIENTED_EDGE('',*,*,#19238,.F.);
#25242=ORIENTED_EDGE('',*,*,#19239,.F.);
#25243=ORIENTED_EDGE('',*,*,#19240,.F.);
#25244=ORIENTED_EDGE('',*,*,#17831,.T.);
#25245=ORIENTED_EDGE('',*,*,#19241,.T.);
#25246=ORIENTED_EDGE('',*,*,#19239,.T.);
#25247=ORIENTED_EDGE('',*,*,#19242,.T.);
#25248=ORIENTED_EDGE('',*,*,#19243,.F.);
#25249=ORIENTED_EDGE('',*,*,#19244,.F.);
#25250=ORIENTED_EDGE('',*,*,#19245,.F.);
#25251=ORIENTED_EDGE('',*,*,#17829,.T.);
#25252=ORIENTED_EDGE('',*,*,#19246,.T.);
#25253=ORIENTED_EDGE('',*,*,#19244,.T.);
#25254=ORIENTED_EDGE('',*,*,#19247,.T.);
#25255=ORIENTED_EDGE('',*,*,#19236,.T.);
#25256=ORIENTED_EDGE('',*,*,#19248,.T.);
#25257=ORIENTED_EDGE('',*,*,#19245,.T.);
#25258=ORIENTED_EDGE('',*,*,#19249,.T.);
#25259=ORIENTED_EDGE('',*,*,#19243,.T.);
#25260=ORIENTED_EDGE('',*,*,#19250,.T.);
#25261=ORIENTED_EDGE('',*,*,#19240,.T.);
#25262=ORIENTED_EDGE('',*,*,#19251,.T.);
#25263=ORIENTED_EDGE('',*,*,#19233,.T.);
#25264=ORIENTED_EDGE('',*,*,#19252,.T.);
#25265=ORIENTED_EDGE('',*,*,#19238,.T.);
#25266=ORIENTED_EDGE('',*,*,#19253,.T.);
#25267=ORIENTED_EDGE('',*,*,#17835,.T.);
#25268=ORIENTED_EDGE('',*,*,#19254,.T.);
#25269=ORIENTED_EDGE('',*,*,#19237,.T.);
#25270=ORIENTED_EDGE('',*,*,#19255,.T.);
#25271=ORIENTED_EDGE('',*,*,#19235,.T.);
#25272=ORIENTED_EDGE('',*,*,#19256,.T.);
#25273=ORIENTED_EDGE('',*,*,#19234,.T.);
#25274=ORIENTED_EDGE('',*,*,#19257,.T.);
#25275=ORIENTED_EDGE('',*,*,#17833,.T.);
#25276=ORIENTED_EDGE('',*,*,#19258,.T.);
#25277=ORIENTED_EDGE('',*,*,#19232,.T.);
#25278=ORIENTED_EDGE('',*,*,#19259,.T.);
#25279=ORIENTED_EDGE('',*,*,#19247,.F.);
#25280=ORIENTED_EDGE('',*,*,#19251,.F.);
#25281=ORIENTED_EDGE('',*,*,#19241,.F.);
#25282=ORIENTED_EDGE('',*,*,#17830,.F.);
#25283=ORIENTED_EDGE('',*,*,#19242,.F.);
#25284=ORIENTED_EDGE('',*,*,#19252,.F.);
#25285=ORIENTED_EDGE('',*,*,#19258,.F.);
#25286=ORIENTED_EDGE('',*,*,#17832,.F.);
#25287=ORIENTED_EDGE('',*,*,#19248,.F.);
#25288=ORIENTED_EDGE('',*,*,#19257,.F.);
#25289=ORIENTED_EDGE('',*,*,#19253,.F.);
#25290=ORIENTED_EDGE('',*,*,#19250,.F.);
#25291=ORIENTED_EDGE('',*,*,#19260,.T.);
#25292=ORIENTED_EDGE('',*,*,#19261,.T.);
#25293=ORIENTED_EDGE('',*,*,#17841,.T.);
#25294=ORIENTED_EDGE('',*,*,#19262,.T.);
#25295=ORIENTED_EDGE('',*,*,#19263,.T.);
#25296=ORIENTED_EDGE('',*,*,#19261,.F.);
#25297=ORIENTED_EDGE('',*,*,#19264,.F.);
#25298=ORIENTED_EDGE('',*,*,#19265,.F.);
#25299=ORIENTED_EDGE('',*,*,#17842,.F.);
#25300=ORIENTED_EDGE('',*,*,#19260,.F.);
#25301=ORIENTED_EDGE('',*,*,#19266,.F.);
#25302=ORIENTED_EDGE('',*,*,#19267,.T.);
#25303=ORIENTED_EDGE('',*,*,#19268,.T.);
#25304=ORIENTED_EDGE('',*,*,#19264,.T.);
#25305=ORIENTED_EDGE('',*,*,#19263,.F.);
#25306=ORIENTED_EDGE('',*,*,#19269,.T.);
#25307=ORIENTED_EDGE('',*,*,#19270,.T.);
#25308=ORIENTED_EDGE('',*,*,#19271,.T.);
#25309=ORIENTED_EDGE('',*,*,#19266,.T.);
#25310=ORIENTED_EDGE('',*,*,#19268,.F.);
#25311=ORIENTED_EDGE('',*,*,#19272,.F.);
#25312=ORIENTED_EDGE('',*,*,#19273,.F.);
#25313=ORIENTED_EDGE('',*,*,#19270,.F.);
#25314=ORIENTED_EDGE('',*,*,#19274,.F.);
#25315=ORIENTED_EDGE('',*,*,#19275,.F.);
#25316=ORIENTED_EDGE('',*,*,#17839,.T.);
#25317=ORIENTED_EDGE('',*,*,#19276,.T.);
#25318=ORIENTED_EDGE('',*,*,#19274,.T.);
#25319=ORIENTED_EDGE('',*,*,#19277,.T.);
#25320=ORIENTED_EDGE('',*,*,#19278,.F.);
#25321=ORIENTED_EDGE('',*,*,#19279,.F.);
#25322=ORIENTED_EDGE('',*,*,#19280,.F.);
#25323=ORIENTED_EDGE('',*,*,#17837,.T.);
#25324=ORIENTED_EDGE('',*,*,#19281,.T.);
#25325=ORIENTED_EDGE('',*,*,#19279,.T.);
#25326=ORIENTED_EDGE('',*,*,#19282,.T.);
#25327=ORIENTED_EDGE('',*,*,#19272,.T.);
#25328=ORIENTED_EDGE('',*,*,#19283,.T.);
#25329=ORIENTED_EDGE('',*,*,#19280,.T.);
#25330=ORIENTED_EDGE('',*,*,#19284,.T.);
#25331=ORIENTED_EDGE('',*,*,#19278,.T.);
#25332=ORIENTED_EDGE('',*,*,#19285,.T.);
#25333=ORIENTED_EDGE('',*,*,#19275,.T.);
#25334=ORIENTED_EDGE('',*,*,#19286,.T.);
#25335=ORIENTED_EDGE('',*,*,#17843,.T.);
#25336=ORIENTED_EDGE('',*,*,#19265,.T.);
#25337=ORIENTED_EDGE('',*,*,#19273,.T.);
#25338=ORIENTED_EDGE('',*,*,#19287,.T.);
#25339=ORIENTED_EDGE('',*,*,#19262,.F.);
#25340=ORIENTED_EDGE('',*,*,#17840,.F.);
#25341=ORIENTED_EDGE('',*,*,#19277,.F.);
#25342=ORIENTED_EDGE('',*,*,#19269,.F.);
#25343=ORIENTED_EDGE('',*,*,#19283,.F.);
#25344=ORIENTED_EDGE('',*,*,#19267,.F.);
#25345=ORIENTED_EDGE('',*,*,#19271,.F.);
#25346=ORIENTED_EDGE('',*,*,#19285,.F.);
#25347=ORIENTED_EDGE('',*,*,#19288,.F.);
#25348=ORIENTED_EDGE('',*,*,#19289,.F.);
#25349=ORIENTED_EDGE('',*,*,#19290,.F.);
#25350=ORIENTED_EDGE('',*,*,#19291,.F.);
#25351=ORIENTED_EDGE('',*,*,#19292,.F.);
#25352=ORIENTED_EDGE('',*,*,#19293,.F.);
#25353=ORIENTED_EDGE('',*,*,#19294,.F.);
#25354=ORIENTED_EDGE('',*,*,#19295,.F.);
#25355=ORIENTED_EDGE('',*,*,#19296,.F.);
#25356=ORIENTED_EDGE('',*,*,#17847,.T.);
#25357=ORIENTED_EDGE('',*,*,#19297,.T.);
#25358=ORIENTED_EDGE('',*,*,#19295,.T.);
#25359=ORIENTED_EDGE('',*,*,#19298,.T.);
#25360=ORIENTED_EDGE('',*,*,#19299,.F.);
#25361=ORIENTED_EDGE('',*,*,#19300,.F.);
#25362=ORIENTED_EDGE('',*,*,#19301,.F.);
#25363=ORIENTED_EDGE('',*,*,#17845,.T.);
#25364=ORIENTED_EDGE('',*,*,#19302,.T.);
#25365=ORIENTED_EDGE('',*,*,#19300,.T.);
#25366=ORIENTED_EDGE('',*,*,#19303,.T.);
#25367=ORIENTED_EDGE('',*,*,#19292,.T.);
#25368=ORIENTED_EDGE('',*,*,#19304,.T.);
#25369=ORIENTED_EDGE('',*,*,#19301,.T.);
#25370=ORIENTED_EDGE('',*,*,#19305,.T.);
#25371=ORIENTED_EDGE('',*,*,#19299,.T.);
#25372=ORIENTED_EDGE('',*,*,#19306,.T.);
#25373=ORIENTED_EDGE('',*,*,#19296,.T.);
#25374=ORIENTED_EDGE('',*,*,#19307,.T.);
#25375=ORIENTED_EDGE('',*,*,#19289,.T.);
#25376=ORIENTED_EDGE('',*,*,#19308,.T.);
#25377=ORIENTED_EDGE('',*,*,#19294,.T.);
#25378=ORIENTED_EDGE('',*,*,#19309,.T.);
#25379=ORIENTED_EDGE('',*,*,#17851,.T.);
#25380=ORIENTED_EDGE('',*,*,#19310,.T.);
#25381=ORIENTED_EDGE('',*,*,#19293,.T.);
#25382=ORIENTED_EDGE('',*,*,#19311,.T.);
#25383=ORIENTED_EDGE('',*,*,#19291,.T.);
#25384=ORIENTED_EDGE('',*,*,#19312,.T.);
#25385=ORIENTED_EDGE('',*,*,#19290,.T.);
#25386=ORIENTED_EDGE('',*,*,#19313,.T.);
#25387=ORIENTED_EDGE('',*,*,#17849,.T.);
#25388=ORIENTED_EDGE('',*,*,#19314,.T.);
#25389=ORIENTED_EDGE('',*,*,#19288,.T.);
#25390=ORIENTED_EDGE('',*,*,#19315,.T.);
#25391=ORIENTED_EDGE('',*,*,#19303,.F.);
#25392=ORIENTED_EDGE('',*,*,#19307,.F.);
#25393=ORIENTED_EDGE('',*,*,#19297,.F.);
#25394=ORIENTED_EDGE('',*,*,#17846,.F.);
#25395=ORIENTED_EDGE('',*,*,#19298,.F.);
#25396=ORIENTED_EDGE('',*,*,#19308,.F.);
#25397=ORIENTED_EDGE('',*,*,#19314,.F.);
#25398=ORIENTED_EDGE('',*,*,#17848,.F.);
#25399=ORIENTED_EDGE('',*,*,#19304,.F.);
#25400=ORIENTED_EDGE('',*,*,#19313,.F.);
#25401=ORIENTED_EDGE('',*,*,#19309,.F.);
#25402=ORIENTED_EDGE('',*,*,#19306,.F.);
#25403=ORIENTED_EDGE('',*,*,#19316,.F.);
#25404=ORIENTED_EDGE('',*,*,#19317,.F.);
#25405=ORIENTED_EDGE('',*,*,#19318,.F.);
#25406=ORIENTED_EDGE('',*,*,#19319,.T.);
#25407=ORIENTED_EDGE('',*,*,#19320,.T.);
#25408=ORIENTED_EDGE('',*,*,#19317,.T.);
#25409=ORIENTED_EDGE('',*,*,#19321,.T.);
#25410=ORIENTED_EDGE('',*,*,#19322,.T.);
#25411=ORIENTED_EDGE('',*,*,#17859,.T.);
#25412=ORIENTED_EDGE('',*,*,#19323,.T.);
#25413=ORIENTED_EDGE('',*,*,#19318,.T.);
#25414=ORIENTED_EDGE('',*,*,#19324,.T.);
#25415=ORIENTED_EDGE('',*,*,#19325,.F.);
#25416=ORIENTED_EDGE('',*,*,#19326,.F.);
#25417=ORIENTED_EDGE('',*,*,#19327,.F.);
#25418=ORIENTED_EDGE('',*,*,#19328,.T.);
#25419=ORIENTED_EDGE('',*,*,#19329,.T.);
#25420=ORIENTED_EDGE('',*,*,#19326,.T.);
#25421=ORIENTED_EDGE('',*,*,#19330,.T.);
#25422=ORIENTED_EDGE('',*,*,#19331,.T.);
#25423=ORIENTED_EDGE('',*,*,#19316,.T.);
#25424=ORIENTED_EDGE('',*,*,#19332,.T.);
#25425=ORIENTED_EDGE('',*,*,#19327,.T.);
#25426=ORIENTED_EDGE('',*,*,#19333,.T.);
#25427=ORIENTED_EDGE('',*,*,#17857,.T.);
#25428=ORIENTED_EDGE('',*,*,#19334,.T.);
#25429=ORIENTED_EDGE('',*,*,#19325,.T.);
#25430=ORIENTED_EDGE('',*,*,#19335,.T.);
#25431=ORIENTED_EDGE('',*,*,#19319,.F.);
#25432=ORIENTED_EDGE('',*,*,#19336,.T.);
#25433=ORIENTED_EDGE('',*,*,#19337,.T.);
#25434=ORIENTED_EDGE('',*,*,#17853,.T.);
#25435=ORIENTED_EDGE('',*,*,#19338,.T.);
#25436=ORIENTED_EDGE('',*,*,#19321,.F.);
#25437=ORIENTED_EDGE('',*,*,#19333,.F.);
#25438=ORIENTED_EDGE('',*,*,#19329,.F.);
#25439=ORIENTED_EDGE('',*,*,#19339,.F.);
#25440=ORIENTED_EDGE('',*,*,#19322,.F.);
#25441=ORIENTED_EDGE('',*,*,#19339,.T.);
#25442=ORIENTED_EDGE('',*,*,#19328,.F.);
#25443=ORIENTED_EDGE('',*,*,#19340,.F.);
#25444=ORIENTED_EDGE('',*,*,#19341,.T.);
#25445=ORIENTED_EDGE('',*,*,#19336,.F.);
#25446=ORIENTED_EDGE('',*,*,#19331,.F.);
#25447=ORIENTED_EDGE('',*,*,#19342,.T.);
#25448=ORIENTED_EDGE('',*,*,#17855,.T.);
#25449=ORIENTED_EDGE('',*,*,#19343,.T.);
#25450=ORIENTED_EDGE('',*,*,#19340,.T.);
#25451=ORIENTED_EDGE('',*,*,#19330,.F.);
#25452=ORIENTED_EDGE('',*,*,#19334,.F.);
#25453=ORIENTED_EDGE('',*,*,#17856,.F.);
#25454=ORIENTED_EDGE('',*,*,#19342,.F.);
#25455=ORIENTED_EDGE('',*,*,#19320,.F.);
#25456=ORIENTED_EDGE('',*,*,#19338,.F.);
#25457=ORIENTED_EDGE('',*,*,#17852,.F.);
#25458=ORIENTED_EDGE('',*,*,#19324,.F.);
#25459=ORIENTED_EDGE('',*,*,#19344,.F.);
#25460=ORIENTED_EDGE('',*,*,#19345,.F.);
#25461=ORIENTED_EDGE('',*,*,#19346,.F.);
#25462=ORIENTED_EDGE('',*,*,#19347,.F.);
#25463=ORIENTED_EDGE('',*,*,#19348,.F.);
#25464=ORIENTED_EDGE('',*,*,#19349,.F.);
#25465=ORIENTED_EDGE('',*,*,#19350,.F.);
#25466=ORIENTED_EDGE('',*,*,#19351,.F.);
#25467=ORIENTED_EDGE('',*,*,#19352,.F.);
#25468=ORIENTED_EDGE('',*,*,#17863,.T.);
#25469=ORIENTED_EDGE('',*,*,#19353,.T.);
#25470=ORIENTED_EDGE('',*,*,#19351,.T.);
#25471=ORIENTED_EDGE('',*,*,#19354,.T.);
#25472=ORIENTED_EDGE('',*,*,#19355,.F.);
#25473=ORIENTED_EDGE('',*,*,#19356,.F.);
#25474=ORIENTED_EDGE('',*,*,#19357,.F.);
#25475=ORIENTED_EDGE('',*,*,#17861,.T.);
#25476=ORIENTED_EDGE('',*,*,#19358,.T.);
#25477=ORIENTED_EDGE('',*,*,#19356,.T.);
#25478=ORIENTED_EDGE('',*,*,#19359,.T.);
#25479=ORIENTED_EDGE('',*,*,#19348,.T.);
#25480=ORIENTED_EDGE('',*,*,#19360,.T.);
#25481=ORIENTED_EDGE('',*,*,#19357,.T.);
#25482=ORIENTED_EDGE('',*,*,#19361,.T.);
#25483=ORIENTED_EDGE('',*,*,#19355,.T.);
#25484=ORIENTED_EDGE('',*,*,#19362,.T.);
#25485=ORIENTED_EDGE('',*,*,#19352,.T.);
#25486=ORIENTED_EDGE('',*,*,#19363,.T.);
#25487=ORIENTED_EDGE('',*,*,#19345,.T.);
#25488=ORIENTED_EDGE('',*,*,#19364,.T.);
#25489=ORIENTED_EDGE('',*,*,#19350,.T.);
#25490=ORIENTED_EDGE('',*,*,#19365,.T.);
#25491=ORIENTED_EDGE('',*,*,#17867,.T.);
#25492=ORIENTED_EDGE('',*,*,#19366,.T.);
#25493=ORIENTED_EDGE('',*,*,#19349,.T.);
#25494=ORIENTED_EDGE('',*,*,#19367,.T.);
#25495=ORIENTED_EDGE('',*,*,#19347,.T.);
#25496=ORIENTED_EDGE('',*,*,#19368,.T.);
#25497=ORIENTED_EDGE('',*,*,#19346,.T.);
#25498=ORIENTED_EDGE('',*,*,#19369,.T.);
#25499=ORIENTED_EDGE('',*,*,#17865,.T.);
#25500=ORIENTED_EDGE('',*,*,#19370,.T.);
#25501=ORIENTED_EDGE('',*,*,#19344,.T.);
#25502=ORIENTED_EDGE('',*,*,#19371,.T.);
#25503=ORIENTED_EDGE('',*,*,#19359,.F.);
#25504=ORIENTED_EDGE('',*,*,#19363,.F.);
#25505=ORIENTED_EDGE('',*,*,#19353,.F.);
#25506=ORIENTED_EDGE('',*,*,#17862,.F.);
#25507=ORIENTED_EDGE('',*,*,#19354,.F.);
#25508=ORIENTED_EDGE('',*,*,#19364,.F.);
#25509=ORIENTED_EDGE('',*,*,#19370,.F.);
#25510=ORIENTED_EDGE('',*,*,#17864,.F.);
#25511=ORIENTED_EDGE('',*,*,#19360,.F.);
#25512=ORIENTED_EDGE('',*,*,#19369,.F.);
#25513=ORIENTED_EDGE('',*,*,#19365,.F.);
#25514=ORIENTED_EDGE('',*,*,#19362,.F.);
#25515=ORIENTED_EDGE('',*,*,#19372,.F.);
#25516=ORIENTED_EDGE('',*,*,#19373,.F.);
#25517=ORIENTED_EDGE('',*,*,#19374,.F.);
#25518=ORIENTED_EDGE('',*,*,#19375,.F.);
#25519=ORIENTED_EDGE('',*,*,#19376,.F.);
#25520=ORIENTED_EDGE('',*,*,#19377,.F.);
#25521=ORIENTED_EDGE('',*,*,#19378,.F.);
#25522=ORIENTED_EDGE('',*,*,#19379,.F.);
#25523=ORIENTED_EDGE('',*,*,#19380,.F.);
#25524=ORIENTED_EDGE('',*,*,#17871,.T.);
#25525=ORIENTED_EDGE('',*,*,#19381,.T.);
#25526=ORIENTED_EDGE('',*,*,#19379,.T.);
#25527=ORIENTED_EDGE('',*,*,#19382,.T.);
#25528=ORIENTED_EDGE('',*,*,#19383,.F.);
#25529=ORIENTED_EDGE('',*,*,#19384,.F.);
#25530=ORIENTED_EDGE('',*,*,#19385,.F.);
#25531=ORIENTED_EDGE('',*,*,#17869,.T.);
#25532=ORIENTED_EDGE('',*,*,#19386,.T.);
#25533=ORIENTED_EDGE('',*,*,#19384,.T.);
#25534=ORIENTED_EDGE('',*,*,#19387,.T.);
#25535=ORIENTED_EDGE('',*,*,#19376,.T.);
#25536=ORIENTED_EDGE('',*,*,#19388,.T.);
#25537=ORIENTED_EDGE('',*,*,#19385,.T.);
#25538=ORIENTED_EDGE('',*,*,#19389,.T.);
#25539=ORIENTED_EDGE('',*,*,#19383,.T.);
#25540=ORIENTED_EDGE('',*,*,#19390,.T.);
#25541=ORIENTED_EDGE('',*,*,#19380,.T.);
#25542=ORIENTED_EDGE('',*,*,#19391,.T.);
#25543=ORIENTED_EDGE('',*,*,#19373,.T.);
#25544=ORIENTED_EDGE('',*,*,#19392,.T.);
#25545=ORIENTED_EDGE('',*,*,#19378,.T.);
#25546=ORIENTED_EDGE('',*,*,#19393,.T.);
#25547=ORIENTED_EDGE('',*,*,#17875,.T.);
#25548=ORIENTED_EDGE('',*,*,#19394,.T.);
#25549=ORIENTED_EDGE('',*,*,#19377,.T.);
#25550=ORIENTED_EDGE('',*,*,#19395,.T.);
#25551=ORIENTED_EDGE('',*,*,#19375,.T.);
#25552=ORIENTED_EDGE('',*,*,#19396,.T.);
#25553=ORIENTED_EDGE('',*,*,#19374,.T.);
#25554=ORIENTED_EDGE('',*,*,#19397,.T.);
#25555=ORIENTED_EDGE('',*,*,#17873,.T.);
#25556=ORIENTED_EDGE('',*,*,#19398,.T.);
#25557=ORIENTED_EDGE('',*,*,#19372,.T.);
#25558=ORIENTED_EDGE('',*,*,#19399,.T.);
#25559=ORIENTED_EDGE('',*,*,#19387,.F.);
#25560=ORIENTED_EDGE('',*,*,#19391,.F.);
#25561=ORIENTED_EDGE('',*,*,#19381,.F.);
#25562=ORIENTED_EDGE('',*,*,#17870,.F.);
#25563=ORIENTED_EDGE('',*,*,#19382,.F.);
#25564=ORIENTED_EDGE('',*,*,#19392,.F.);
#25565=ORIENTED_EDGE('',*,*,#19398,.F.);
#25566=ORIENTED_EDGE('',*,*,#17872,.F.);
#25567=ORIENTED_EDGE('',*,*,#19388,.F.);
#25568=ORIENTED_EDGE('',*,*,#19397,.F.);
#25569=ORIENTED_EDGE('',*,*,#19393,.F.);
#25570=ORIENTED_EDGE('',*,*,#19390,.F.);
#25571=ORIENTED_EDGE('',*,*,#19400,.T.);
#25572=ORIENTED_EDGE('',*,*,#19401,.T.);
#25573=ORIENTED_EDGE('',*,*,#17881,.T.);
#25574=ORIENTED_EDGE('',*,*,#19402,.T.);
#25575=ORIENTED_EDGE('',*,*,#19403,.T.);
#25576=ORIENTED_EDGE('',*,*,#19401,.F.);
#25577=ORIENTED_EDGE('',*,*,#19404,.F.);
#25578=ORIENTED_EDGE('',*,*,#19405,.F.);
#25579=ORIENTED_EDGE('',*,*,#17882,.F.);
#25580=ORIENTED_EDGE('',*,*,#19400,.F.);
#25581=ORIENTED_EDGE('',*,*,#19406,.F.);
#25582=ORIENTED_EDGE('',*,*,#19407,.T.);
#25583=ORIENTED_EDGE('',*,*,#19408,.T.);
#25584=ORIENTED_EDGE('',*,*,#19404,.T.);
#25585=ORIENTED_EDGE('',*,*,#19403,.F.);
#25586=ORIENTED_EDGE('',*,*,#19409,.T.);
#25587=ORIENTED_EDGE('',*,*,#19410,.T.);
#25588=ORIENTED_EDGE('',*,*,#19411,.T.);
#25589=ORIENTED_EDGE('',*,*,#19406,.T.);
#25590=ORIENTED_EDGE('',*,*,#19408,.F.);
#25591=ORIENTED_EDGE('',*,*,#19412,.F.);
#25592=ORIENTED_EDGE('',*,*,#19413,.F.);
#25593=ORIENTED_EDGE('',*,*,#19410,.F.);
#25594=ORIENTED_EDGE('',*,*,#19414,.F.);
#25595=ORIENTED_EDGE('',*,*,#19415,.F.);
#25596=ORIENTED_EDGE('',*,*,#17879,.T.);
#25597=ORIENTED_EDGE('',*,*,#19416,.T.);
#25598=ORIENTED_EDGE('',*,*,#19414,.T.);
#25599=ORIENTED_EDGE('',*,*,#19417,.T.);
#25600=ORIENTED_EDGE('',*,*,#19418,.F.);
#25601=ORIENTED_EDGE('',*,*,#19419,.F.);
#25602=ORIENTED_EDGE('',*,*,#19420,.F.);
#25603=ORIENTED_EDGE('',*,*,#17877,.T.);
#25604=ORIENTED_EDGE('',*,*,#19421,.T.);
#25605=ORIENTED_EDGE('',*,*,#19419,.T.);
#25606=ORIENTED_EDGE('',*,*,#19422,.T.);
#25607=ORIENTED_EDGE('',*,*,#19412,.T.);
#25608=ORIENTED_EDGE('',*,*,#19423,.T.);
#25609=ORIENTED_EDGE('',*,*,#19420,.T.);
#25610=ORIENTED_EDGE('',*,*,#19424,.T.);
#25611=ORIENTED_EDGE('',*,*,#19418,.T.);
#25612=ORIENTED_EDGE('',*,*,#19425,.T.);
#25613=ORIENTED_EDGE('',*,*,#19415,.T.);
#25614=ORIENTED_EDGE('',*,*,#19426,.T.);
#25615=ORIENTED_EDGE('',*,*,#17883,.T.);
#25616=ORIENTED_EDGE('',*,*,#19405,.T.);
#25617=ORIENTED_EDGE('',*,*,#19413,.T.);
#25618=ORIENTED_EDGE('',*,*,#19427,.T.);
#25619=ORIENTED_EDGE('',*,*,#19402,.F.);
#25620=ORIENTED_EDGE('',*,*,#17880,.F.);
#25621=ORIENTED_EDGE('',*,*,#19417,.F.);
#25622=ORIENTED_EDGE('',*,*,#19409,.F.);
#25623=ORIENTED_EDGE('',*,*,#19423,.F.);
#25624=ORIENTED_EDGE('',*,*,#19407,.F.);
#25625=ORIENTED_EDGE('',*,*,#19411,.F.);
#25626=ORIENTED_EDGE('',*,*,#19425,.F.);
#25627=ORIENTED_EDGE('',*,*,#19428,.F.);
#25628=ORIENTED_EDGE('',*,*,#19429,.F.);
#25629=ORIENTED_EDGE('',*,*,#19430,.F.);
#25630=ORIENTED_EDGE('',*,*,#19431,.F.);
#25631=ORIENTED_EDGE('',*,*,#19432,.F.);
#25632=ORIENTED_EDGE('',*,*,#19433,.F.);
#25633=ORIENTED_EDGE('',*,*,#19434,.F.);
#25634=ORIENTED_EDGE('',*,*,#19435,.F.);
#25635=ORIENTED_EDGE('',*,*,#19436,.F.);
#25636=ORIENTED_EDGE('',*,*,#17887,.T.);
#25637=ORIENTED_EDGE('',*,*,#19437,.T.);
#25638=ORIENTED_EDGE('',*,*,#19435,.T.);
#25639=ORIENTED_EDGE('',*,*,#19438,.T.);
#25640=ORIENTED_EDGE('',*,*,#19439,.F.);
#25641=ORIENTED_EDGE('',*,*,#19440,.F.);
#25642=ORIENTED_EDGE('',*,*,#19441,.F.);
#25643=ORIENTED_EDGE('',*,*,#17885,.T.);
#25644=ORIENTED_EDGE('',*,*,#19442,.T.);
#25645=ORIENTED_EDGE('',*,*,#19440,.T.);
#25646=ORIENTED_EDGE('',*,*,#19443,.T.);
#25647=ORIENTED_EDGE('',*,*,#19432,.T.);
#25648=ORIENTED_EDGE('',*,*,#19444,.T.);
#25649=ORIENTED_EDGE('',*,*,#19441,.T.);
#25650=ORIENTED_EDGE('',*,*,#19445,.T.);
#25651=ORIENTED_EDGE('',*,*,#19439,.T.);
#25652=ORIENTED_EDGE('',*,*,#19446,.T.);
#25653=ORIENTED_EDGE('',*,*,#19436,.T.);
#25654=ORIENTED_EDGE('',*,*,#19447,.T.);
#25655=ORIENTED_EDGE('',*,*,#19429,.T.);
#25656=ORIENTED_EDGE('',*,*,#19448,.T.);
#25657=ORIENTED_EDGE('',*,*,#19434,.T.);
#25658=ORIENTED_EDGE('',*,*,#19449,.T.);
#25659=ORIENTED_EDGE('',*,*,#17891,.T.);
#25660=ORIENTED_EDGE('',*,*,#19450,.T.);
#25661=ORIENTED_EDGE('',*,*,#19433,.T.);
#25662=ORIENTED_EDGE('',*,*,#19451,.T.);
#25663=ORIENTED_EDGE('',*,*,#19431,.T.);
#25664=ORIENTED_EDGE('',*,*,#19452,.T.);
#25665=ORIENTED_EDGE('',*,*,#19430,.T.);
#25666=ORIENTED_EDGE('',*,*,#19453,.T.);
#25667=ORIENTED_EDGE('',*,*,#17889,.T.);
#25668=ORIENTED_EDGE('',*,*,#19454,.T.);
#25669=ORIENTED_EDGE('',*,*,#19428,.T.);
#25670=ORIENTED_EDGE('',*,*,#19455,.T.);
#25671=ORIENTED_EDGE('',*,*,#19443,.F.);
#25672=ORIENTED_EDGE('',*,*,#19447,.F.);
#25673=ORIENTED_EDGE('',*,*,#19437,.F.);
#25674=ORIENTED_EDGE('',*,*,#17886,.F.);
#25675=ORIENTED_EDGE('',*,*,#19438,.F.);
#25676=ORIENTED_EDGE('',*,*,#19448,.F.);
#25677=ORIENTED_EDGE('',*,*,#19454,.F.);
#25678=ORIENTED_EDGE('',*,*,#17888,.F.);
#25679=ORIENTED_EDGE('',*,*,#19444,.F.);
#25680=ORIENTED_EDGE('',*,*,#19453,.F.);
#25681=ORIENTED_EDGE('',*,*,#19449,.F.);
#25682=ORIENTED_EDGE('',*,*,#19446,.F.);
#25683=ORIENTED_EDGE('',*,*,#19456,.F.);
#25684=ORIENTED_EDGE('',*,*,#19457,.F.);
#25685=ORIENTED_EDGE('',*,*,#19458,.F.);
#25686=ORIENTED_EDGE('',*,*,#19459,.T.);
#25687=ORIENTED_EDGE('',*,*,#19460,.T.);
#25688=ORIENTED_EDGE('',*,*,#19457,.T.);
#25689=ORIENTED_EDGE('',*,*,#19461,.T.);
#25690=ORIENTED_EDGE('',*,*,#19462,.T.);
#25691=ORIENTED_EDGE('',*,*,#17899,.T.);
#25692=ORIENTED_EDGE('',*,*,#19463,.T.);
#25693=ORIENTED_EDGE('',*,*,#19458,.T.);
#25694=ORIENTED_EDGE('',*,*,#19464,.T.);
#25695=ORIENTED_EDGE('',*,*,#19465,.F.);
#25696=ORIENTED_EDGE('',*,*,#19466,.F.);
#25697=ORIENTED_EDGE('',*,*,#19467,.F.);
#25698=ORIENTED_EDGE('',*,*,#19468,.T.);
#25699=ORIENTED_EDGE('',*,*,#19469,.T.);
#25700=ORIENTED_EDGE('',*,*,#19466,.T.);
#25701=ORIENTED_EDGE('',*,*,#19470,.T.);
#25702=ORIENTED_EDGE('',*,*,#19471,.T.);
#25703=ORIENTED_EDGE('',*,*,#19456,.T.);
#25704=ORIENTED_EDGE('',*,*,#19472,.T.);
#25705=ORIENTED_EDGE('',*,*,#19467,.T.);
#25706=ORIENTED_EDGE('',*,*,#19473,.T.);
#25707=ORIENTED_EDGE('',*,*,#17897,.T.);
#25708=ORIENTED_EDGE('',*,*,#19474,.T.);
#25709=ORIENTED_EDGE('',*,*,#19465,.T.);
#25710=ORIENTED_EDGE('',*,*,#19475,.T.);
#25711=ORIENTED_EDGE('',*,*,#19459,.F.);
#25712=ORIENTED_EDGE('',*,*,#19476,.T.);
#25713=ORIENTED_EDGE('',*,*,#19477,.T.);
#25714=ORIENTED_EDGE('',*,*,#17893,.T.);
#25715=ORIENTED_EDGE('',*,*,#19478,.T.);
#25716=ORIENTED_EDGE('',*,*,#19461,.F.);
#25717=ORIENTED_EDGE('',*,*,#19473,.F.);
#25718=ORIENTED_EDGE('',*,*,#19469,.F.);
#25719=ORIENTED_EDGE('',*,*,#19479,.F.);
#25720=ORIENTED_EDGE('',*,*,#19462,.F.);
#25721=ORIENTED_EDGE('',*,*,#19479,.T.);
#25722=ORIENTED_EDGE('',*,*,#19468,.F.);
#25723=ORIENTED_EDGE('',*,*,#19480,.F.);
#25724=ORIENTED_EDGE('',*,*,#19481,.T.);
#25725=ORIENTED_EDGE('',*,*,#19476,.F.);
#25726=ORIENTED_EDGE('',*,*,#19471,.F.);
#25727=ORIENTED_EDGE('',*,*,#19482,.T.);
#25728=ORIENTED_EDGE('',*,*,#17895,.T.);
#25729=ORIENTED_EDGE('',*,*,#19483,.T.);
#25730=ORIENTED_EDGE('',*,*,#19480,.T.);
#25731=ORIENTED_EDGE('',*,*,#19470,.F.);
#25732=ORIENTED_EDGE('',*,*,#19474,.F.);
#25733=ORIENTED_EDGE('',*,*,#17896,.F.);
#25734=ORIENTED_EDGE('',*,*,#19482,.F.);
#25735=ORIENTED_EDGE('',*,*,#19460,.F.);
#25736=ORIENTED_EDGE('',*,*,#19478,.F.);
#25737=ORIENTED_EDGE('',*,*,#17892,.F.);
#25738=ORIENTED_EDGE('',*,*,#19464,.F.);
#25739=ORIENTED_EDGE('',*,*,#19484,.F.);
#25740=ORIENTED_EDGE('',*,*,#19485,.F.);
#25741=ORIENTED_EDGE('',*,*,#19486,.F.);
#25742=ORIENTED_EDGE('',*,*,#19487,.F.);
#25743=ORIENTED_EDGE('',*,*,#19488,.F.);
#25744=ORIENTED_EDGE('',*,*,#19489,.F.);
#25745=ORIENTED_EDGE('',*,*,#19490,.F.);
#25746=ORIENTED_EDGE('',*,*,#19491,.F.);
#25747=ORIENTED_EDGE('',*,*,#19492,.F.);
#25748=ORIENTED_EDGE('',*,*,#17903,.T.);
#25749=ORIENTED_EDGE('',*,*,#19493,.T.);
#25750=ORIENTED_EDGE('',*,*,#19491,.T.);
#25751=ORIENTED_EDGE('',*,*,#19494,.T.);
#25752=ORIENTED_EDGE('',*,*,#19495,.F.);
#25753=ORIENTED_EDGE('',*,*,#19496,.F.);
#25754=ORIENTED_EDGE('',*,*,#19497,.F.);
#25755=ORIENTED_EDGE('',*,*,#17901,.T.);
#25756=ORIENTED_EDGE('',*,*,#19498,.T.);
#25757=ORIENTED_EDGE('',*,*,#19496,.T.);
#25758=ORIENTED_EDGE('',*,*,#19499,.T.);
#25759=ORIENTED_EDGE('',*,*,#19488,.T.);
#25760=ORIENTED_EDGE('',*,*,#19500,.T.);
#25761=ORIENTED_EDGE('',*,*,#19497,.T.);
#25762=ORIENTED_EDGE('',*,*,#19501,.T.);
#25763=ORIENTED_EDGE('',*,*,#19495,.T.);
#25764=ORIENTED_EDGE('',*,*,#19502,.T.);
#25765=ORIENTED_EDGE('',*,*,#19492,.T.);
#25766=ORIENTED_EDGE('',*,*,#19503,.T.);
#25767=ORIENTED_EDGE('',*,*,#19485,.T.);
#25768=ORIENTED_EDGE('',*,*,#19504,.T.);
#25769=ORIENTED_EDGE('',*,*,#19490,.T.);
#25770=ORIENTED_EDGE('',*,*,#19505,.T.);
#25771=ORIENTED_EDGE('',*,*,#17907,.T.);
#25772=ORIENTED_EDGE('',*,*,#19506,.T.);
#25773=ORIENTED_EDGE('',*,*,#19489,.T.);
#25774=ORIENTED_EDGE('',*,*,#19507,.T.);
#25775=ORIENTED_EDGE('',*,*,#19487,.T.);
#25776=ORIENTED_EDGE('',*,*,#19508,.T.);
#25777=ORIENTED_EDGE('',*,*,#19486,.T.);
#25778=ORIENTED_EDGE('',*,*,#19509,.T.);
#25779=ORIENTED_EDGE('',*,*,#17905,.T.);
#25780=ORIENTED_EDGE('',*,*,#19510,.T.);
#25781=ORIENTED_EDGE('',*,*,#19484,.T.);
#25782=ORIENTED_EDGE('',*,*,#19511,.T.);
#25783=ORIENTED_EDGE('',*,*,#19499,.F.);
#25784=ORIENTED_EDGE('',*,*,#19503,.F.);
#25785=ORIENTED_EDGE('',*,*,#19493,.F.);
#25786=ORIENTED_EDGE('',*,*,#17902,.F.);
#25787=ORIENTED_EDGE('',*,*,#19494,.F.);
#25788=ORIENTED_EDGE('',*,*,#19504,.F.);
#25789=ORIENTED_EDGE('',*,*,#19510,.F.);
#25790=ORIENTED_EDGE('',*,*,#17904,.F.);
#25791=ORIENTED_EDGE('',*,*,#19500,.F.);
#25792=ORIENTED_EDGE('',*,*,#19509,.F.);
#25793=ORIENTED_EDGE('',*,*,#19505,.F.);
#25794=ORIENTED_EDGE('',*,*,#19502,.F.);
#25795=ORIENTED_EDGE('',*,*,#19512,.F.);
#25796=ORIENTED_EDGE('',*,*,#19513,.F.);
#25797=ORIENTED_EDGE('',*,*,#19514,.F.);
#25798=ORIENTED_EDGE('',*,*,#19515,.F.);
#25799=ORIENTED_EDGE('',*,*,#19516,.F.);
#25800=ORIENTED_EDGE('',*,*,#19517,.F.);
#25801=ORIENTED_EDGE('',*,*,#19518,.F.);
#25802=ORIENTED_EDGE('',*,*,#19519,.F.);
#25803=ORIENTED_EDGE('',*,*,#19520,.F.);
#25804=ORIENTED_EDGE('',*,*,#17911,.T.);
#25805=ORIENTED_EDGE('',*,*,#19521,.T.);
#25806=ORIENTED_EDGE('',*,*,#19519,.T.);
#25807=ORIENTED_EDGE('',*,*,#19522,.T.);
#25808=ORIENTED_EDGE('',*,*,#19523,.F.);
#25809=ORIENTED_EDGE('',*,*,#19524,.F.);
#25810=ORIENTED_EDGE('',*,*,#19525,.F.);
#25811=ORIENTED_EDGE('',*,*,#17909,.T.);
#25812=ORIENTED_EDGE('',*,*,#19526,.T.);
#25813=ORIENTED_EDGE('',*,*,#19524,.T.);
#25814=ORIENTED_EDGE('',*,*,#19527,.T.);
#25815=ORIENTED_EDGE('',*,*,#19516,.T.);
#25816=ORIENTED_EDGE('',*,*,#19528,.T.);
#25817=ORIENTED_EDGE('',*,*,#19525,.T.);
#25818=ORIENTED_EDGE('',*,*,#19529,.T.);
#25819=ORIENTED_EDGE('',*,*,#19523,.T.);
#25820=ORIENTED_EDGE('',*,*,#19530,.T.);
#25821=ORIENTED_EDGE('',*,*,#19520,.T.);
#25822=ORIENTED_EDGE('',*,*,#19531,.T.);
#25823=ORIENTED_EDGE('',*,*,#19513,.T.);
#25824=ORIENTED_EDGE('',*,*,#19532,.T.);
#25825=ORIENTED_EDGE('',*,*,#19518,.T.);
#25826=ORIENTED_EDGE('',*,*,#19533,.T.);
#25827=ORIENTED_EDGE('',*,*,#17915,.T.);
#25828=ORIENTED_EDGE('',*,*,#19534,.T.);
#25829=ORIENTED_EDGE('',*,*,#19517,.T.);
#25830=ORIENTED_EDGE('',*,*,#19535,.T.);
#25831=ORIENTED_EDGE('',*,*,#19515,.T.);
#25832=ORIENTED_EDGE('',*,*,#19536,.T.);
#25833=ORIENTED_EDGE('',*,*,#19514,.T.);
#25834=ORIENTED_EDGE('',*,*,#19537,.T.);
#25835=ORIENTED_EDGE('',*,*,#17913,.T.);
#25836=ORIENTED_EDGE('',*,*,#19538,.T.);
#25837=ORIENTED_EDGE('',*,*,#19512,.T.);
#25838=ORIENTED_EDGE('',*,*,#19539,.T.);
#25839=ORIENTED_EDGE('',*,*,#19527,.F.);
#25840=ORIENTED_EDGE('',*,*,#19531,.F.);
#25841=ORIENTED_EDGE('',*,*,#19521,.F.);
#25842=ORIENTED_EDGE('',*,*,#17910,.F.);
#25843=ORIENTED_EDGE('',*,*,#19522,.F.);
#25844=ORIENTED_EDGE('',*,*,#19532,.F.);
#25845=ORIENTED_EDGE('',*,*,#19538,.F.);
#25846=ORIENTED_EDGE('',*,*,#17912,.F.);
#25847=ORIENTED_EDGE('',*,*,#19528,.F.);
#25848=ORIENTED_EDGE('',*,*,#19537,.F.);
#25849=ORIENTED_EDGE('',*,*,#19533,.F.);
#25850=ORIENTED_EDGE('',*,*,#19530,.F.);
#25851=ORIENTED_EDGE('',*,*,#19540,.T.);
#25852=ORIENTED_EDGE('',*,*,#19541,.T.);
#25853=ORIENTED_EDGE('',*,*,#17921,.T.);
#25854=ORIENTED_EDGE('',*,*,#19542,.T.);
#25855=ORIENTED_EDGE('',*,*,#19543,.T.);
#25856=ORIENTED_EDGE('',*,*,#19541,.F.);
#25857=ORIENTED_EDGE('',*,*,#19544,.F.);
#25858=ORIENTED_EDGE('',*,*,#19545,.F.);
#25859=ORIENTED_EDGE('',*,*,#17922,.F.);
#25860=ORIENTED_EDGE('',*,*,#19540,.F.);
#25861=ORIENTED_EDGE('',*,*,#19546,.F.);
#25862=ORIENTED_EDGE('',*,*,#19547,.T.);
#25863=ORIENTED_EDGE('',*,*,#19548,.T.);
#25864=ORIENTED_EDGE('',*,*,#19544,.T.);
#25865=ORIENTED_EDGE('',*,*,#19543,.F.);
#25866=ORIENTED_EDGE('',*,*,#19549,.T.);
#25867=ORIENTED_EDGE('',*,*,#19550,.T.);
#25868=ORIENTED_EDGE('',*,*,#19551,.T.);
#25869=ORIENTED_EDGE('',*,*,#19546,.T.);
#25870=ORIENTED_EDGE('',*,*,#19548,.F.);
#25871=ORIENTED_EDGE('',*,*,#19552,.F.);
#25872=ORIENTED_EDGE('',*,*,#19553,.F.);
#25873=ORIENTED_EDGE('',*,*,#19550,.F.);
#25874=ORIENTED_EDGE('',*,*,#19554,.F.);
#25875=ORIENTED_EDGE('',*,*,#19555,.F.);
#25876=ORIENTED_EDGE('',*,*,#17919,.T.);
#25877=ORIENTED_EDGE('',*,*,#19556,.T.);
#25878=ORIENTED_EDGE('',*,*,#19554,.T.);
#25879=ORIENTED_EDGE('',*,*,#19557,.T.);
#25880=ORIENTED_EDGE('',*,*,#19558,.F.);
#25881=ORIENTED_EDGE('',*,*,#19559,.F.);
#25882=ORIENTED_EDGE('',*,*,#19560,.F.);
#25883=ORIENTED_EDGE('',*,*,#17917,.T.);
#25884=ORIENTED_EDGE('',*,*,#19561,.T.);
#25885=ORIENTED_EDGE('',*,*,#19559,.T.);
#25886=ORIENTED_EDGE('',*,*,#19562,.T.);
#25887=ORIENTED_EDGE('',*,*,#19552,.T.);
#25888=ORIENTED_EDGE('',*,*,#19563,.T.);
#25889=ORIENTED_EDGE('',*,*,#19560,.T.);
#25890=ORIENTED_EDGE('',*,*,#19564,.T.);
#25891=ORIENTED_EDGE('',*,*,#19558,.T.);
#25892=ORIENTED_EDGE('',*,*,#19565,.T.);
#25893=ORIENTED_EDGE('',*,*,#19555,.T.);
#25894=ORIENTED_EDGE('',*,*,#19566,.T.);
#25895=ORIENTED_EDGE('',*,*,#17923,.T.);
#25896=ORIENTED_EDGE('',*,*,#19545,.T.);
#25897=ORIENTED_EDGE('',*,*,#19553,.T.);
#25898=ORIENTED_EDGE('',*,*,#19567,.T.);
#25899=ORIENTED_EDGE('',*,*,#19542,.F.);
#25900=ORIENTED_EDGE('',*,*,#17920,.F.);
#25901=ORIENTED_EDGE('',*,*,#19557,.F.);
#25902=ORIENTED_EDGE('',*,*,#19549,.F.);
#25903=ORIENTED_EDGE('',*,*,#19563,.F.);
#25904=ORIENTED_EDGE('',*,*,#19547,.F.);
#25905=ORIENTED_EDGE('',*,*,#19551,.F.);
#25906=ORIENTED_EDGE('',*,*,#19565,.F.);
#25907=ORIENTED_EDGE('',*,*,#19568,.F.);
#25908=ORIENTED_EDGE('',*,*,#19569,.F.);
#25909=ORIENTED_EDGE('',*,*,#19570,.F.);
#25910=ORIENTED_EDGE('',*,*,#19571,.F.);
#25911=ORIENTED_EDGE('',*,*,#19572,.F.);
#25912=ORIENTED_EDGE('',*,*,#19573,.F.);
#25913=ORIENTED_EDGE('',*,*,#19574,.F.);
#25914=ORIENTED_EDGE('',*,*,#19575,.F.);
#25915=ORIENTED_EDGE('',*,*,#19576,.F.);
#25916=ORIENTED_EDGE('',*,*,#17927,.T.);
#25917=ORIENTED_EDGE('',*,*,#19577,.T.);
#25918=ORIENTED_EDGE('',*,*,#19575,.T.);
#25919=ORIENTED_EDGE('',*,*,#19578,.T.);
#25920=ORIENTED_EDGE('',*,*,#19579,.F.);
#25921=ORIENTED_EDGE('',*,*,#19580,.F.);
#25922=ORIENTED_EDGE('',*,*,#19581,.F.);
#25923=ORIENTED_EDGE('',*,*,#17925,.T.);
#25924=ORIENTED_EDGE('',*,*,#19582,.T.);
#25925=ORIENTED_EDGE('',*,*,#19580,.T.);
#25926=ORIENTED_EDGE('',*,*,#19583,.T.);
#25927=ORIENTED_EDGE('',*,*,#19572,.T.);
#25928=ORIENTED_EDGE('',*,*,#19584,.T.);
#25929=ORIENTED_EDGE('',*,*,#19581,.T.);
#25930=ORIENTED_EDGE('',*,*,#19585,.T.);
#25931=ORIENTED_EDGE('',*,*,#19579,.T.);
#25932=ORIENTED_EDGE('',*,*,#19586,.T.);
#25933=ORIENTED_EDGE('',*,*,#19576,.T.);
#25934=ORIENTED_EDGE('',*,*,#19587,.T.);
#25935=ORIENTED_EDGE('',*,*,#19569,.T.);
#25936=ORIENTED_EDGE('',*,*,#19588,.T.);
#25937=ORIENTED_EDGE('',*,*,#19574,.T.);
#25938=ORIENTED_EDGE('',*,*,#19589,.T.);
#25939=ORIENTED_EDGE('',*,*,#17931,.T.);
#25940=ORIENTED_EDGE('',*,*,#19590,.T.);
#25941=ORIENTED_EDGE('',*,*,#19573,.T.);
#25942=ORIENTED_EDGE('',*,*,#19591,.T.);
#25943=ORIENTED_EDGE('',*,*,#19571,.T.);
#25944=ORIENTED_EDGE('',*,*,#19592,.T.);
#25945=ORIENTED_EDGE('',*,*,#19570,.T.);
#25946=ORIENTED_EDGE('',*,*,#19593,.T.);
#25947=ORIENTED_EDGE('',*,*,#17929,.T.);
#25948=ORIENTED_EDGE('',*,*,#19594,.T.);
#25949=ORIENTED_EDGE('',*,*,#19568,.T.);
#25950=ORIENTED_EDGE('',*,*,#19595,.T.);
#25951=ORIENTED_EDGE('',*,*,#19583,.F.);
#25952=ORIENTED_EDGE('',*,*,#19587,.F.);
#25953=ORIENTED_EDGE('',*,*,#19577,.F.);
#25954=ORIENTED_EDGE('',*,*,#17926,.F.);
#25955=ORIENTED_EDGE('',*,*,#19578,.F.);
#25956=ORIENTED_EDGE('',*,*,#19588,.F.);
#25957=ORIENTED_EDGE('',*,*,#19594,.F.);
#25958=ORIENTED_EDGE('',*,*,#17928,.F.);
#25959=ORIENTED_EDGE('',*,*,#19584,.F.);
#25960=ORIENTED_EDGE('',*,*,#19593,.F.);
#25961=ORIENTED_EDGE('',*,*,#19589,.F.);
#25962=ORIENTED_EDGE('',*,*,#19586,.F.);
#25963=ORIENTED_EDGE('',*,*,#19596,.F.);
#25964=ORIENTED_EDGE('',*,*,#19597,.F.);
#25965=ORIENTED_EDGE('',*,*,#19598,.F.);
#25966=ORIENTED_EDGE('',*,*,#19599,.T.);
#25967=ORIENTED_EDGE('',*,*,#19600,.T.);
#25968=ORIENTED_EDGE('',*,*,#19597,.T.);
#25969=ORIENTED_EDGE('',*,*,#19601,.T.);
#25970=ORIENTED_EDGE('',*,*,#19602,.T.);
#25971=ORIENTED_EDGE('',*,*,#17939,.T.);
#25972=ORIENTED_EDGE('',*,*,#19603,.T.);
#25973=ORIENTED_EDGE('',*,*,#19598,.T.);
#25974=ORIENTED_EDGE('',*,*,#19604,.T.);
#25975=ORIENTED_EDGE('',*,*,#19605,.F.);
#25976=ORIENTED_EDGE('',*,*,#19606,.F.);
#25977=ORIENTED_EDGE('',*,*,#19607,.F.);
#25978=ORIENTED_EDGE('',*,*,#19608,.T.);
#25979=ORIENTED_EDGE('',*,*,#19609,.T.);
#25980=ORIENTED_EDGE('',*,*,#19606,.T.);
#25981=ORIENTED_EDGE('',*,*,#19610,.T.);
#25982=ORIENTED_EDGE('',*,*,#19611,.T.);
#25983=ORIENTED_EDGE('',*,*,#19596,.T.);
#25984=ORIENTED_EDGE('',*,*,#19612,.T.);
#25985=ORIENTED_EDGE('',*,*,#19607,.T.);
#25986=ORIENTED_EDGE('',*,*,#19613,.T.);
#25987=ORIENTED_EDGE('',*,*,#17937,.T.);
#25988=ORIENTED_EDGE('',*,*,#19614,.T.);
#25989=ORIENTED_EDGE('',*,*,#19605,.T.);
#25990=ORIENTED_EDGE('',*,*,#19615,.T.);
#25991=ORIENTED_EDGE('',*,*,#19599,.F.);
#25992=ORIENTED_EDGE('',*,*,#19616,.T.);
#25993=ORIENTED_EDGE('',*,*,#19617,.T.);
#25994=ORIENTED_EDGE('',*,*,#17933,.T.);
#25995=ORIENTED_EDGE('',*,*,#19618,.T.);
#25996=ORIENTED_EDGE('',*,*,#19601,.F.);
#25997=ORIENTED_EDGE('',*,*,#19613,.F.);
#25998=ORIENTED_EDGE('',*,*,#19609,.F.);
#25999=ORIENTED_EDGE('',*,*,#19619,.F.);
#26000=ORIENTED_EDGE('',*,*,#19602,.F.);
#26001=ORIENTED_EDGE('',*,*,#19619,.T.);
#26002=ORIENTED_EDGE('',*,*,#19608,.F.);
#26003=ORIENTED_EDGE('',*,*,#19620,.F.);
#26004=ORIENTED_EDGE('',*,*,#19621,.T.);
#26005=ORIENTED_EDGE('',*,*,#19616,.F.);
#26006=ORIENTED_EDGE('',*,*,#19611,.F.);
#26007=ORIENTED_EDGE('',*,*,#19622,.T.);
#26008=ORIENTED_EDGE('',*,*,#17935,.T.);
#26009=ORIENTED_EDGE('',*,*,#19623,.T.);
#26010=ORIENTED_EDGE('',*,*,#19620,.T.);
#26011=ORIENTED_EDGE('',*,*,#19610,.F.);
#26012=ORIENTED_EDGE('',*,*,#19614,.F.);
#26013=ORIENTED_EDGE('',*,*,#17936,.F.);
#26014=ORIENTED_EDGE('',*,*,#19622,.F.);
#26015=ORIENTED_EDGE('',*,*,#19600,.F.);
#26016=ORIENTED_EDGE('',*,*,#19618,.F.);
#26017=ORIENTED_EDGE('',*,*,#17932,.F.);
#26018=ORIENTED_EDGE('',*,*,#19604,.F.);
#26019=ORIENTED_EDGE('',*,*,#19624,.F.);
#26020=ORIENTED_EDGE('',*,*,#19625,.F.);
#26021=ORIENTED_EDGE('',*,*,#19626,.F.);
#26022=ORIENTED_EDGE('',*,*,#19627,.F.);
#26023=ORIENTED_EDGE('',*,*,#19628,.F.);
#26024=ORIENTED_EDGE('',*,*,#19629,.F.);
#26025=ORIENTED_EDGE('',*,*,#19630,.F.);
#26026=ORIENTED_EDGE('',*,*,#19631,.F.);
#26027=ORIENTED_EDGE('',*,*,#19632,.F.);
#26028=ORIENTED_EDGE('',*,*,#17943,.T.);
#26029=ORIENTED_EDGE('',*,*,#19633,.T.);
#26030=ORIENTED_EDGE('',*,*,#19631,.T.);
#26031=ORIENTED_EDGE('',*,*,#19634,.T.);
#26032=ORIENTED_EDGE('',*,*,#19635,.F.);
#26033=ORIENTED_EDGE('',*,*,#19636,.F.);
#26034=ORIENTED_EDGE('',*,*,#19637,.F.);
#26035=ORIENTED_EDGE('',*,*,#17941,.T.);
#26036=ORIENTED_EDGE('',*,*,#19638,.T.);
#26037=ORIENTED_EDGE('',*,*,#19636,.T.);
#26038=ORIENTED_EDGE('',*,*,#19639,.T.);
#26039=ORIENTED_EDGE('',*,*,#19628,.T.);
#26040=ORIENTED_EDGE('',*,*,#19640,.T.);
#26041=ORIENTED_EDGE('',*,*,#19637,.T.);
#26042=ORIENTED_EDGE('',*,*,#19641,.T.);
#26043=ORIENTED_EDGE('',*,*,#19635,.T.);
#26044=ORIENTED_EDGE('',*,*,#19642,.T.);
#26045=ORIENTED_EDGE('',*,*,#19632,.T.);
#26046=ORIENTED_EDGE('',*,*,#19643,.T.);
#26047=ORIENTED_EDGE('',*,*,#19625,.T.);
#26048=ORIENTED_EDGE('',*,*,#19644,.T.);
#26049=ORIENTED_EDGE('',*,*,#19630,.T.);
#26050=ORIENTED_EDGE('',*,*,#19645,.T.);
#26051=ORIENTED_EDGE('',*,*,#17947,.T.);
#26052=ORIENTED_EDGE('',*,*,#19646,.T.);
#26053=ORIENTED_EDGE('',*,*,#19629,.T.);
#26054=ORIENTED_EDGE('',*,*,#19647,.T.);
#26055=ORIENTED_EDGE('',*,*,#19627,.T.);
#26056=ORIENTED_EDGE('',*,*,#19648,.T.);
#26057=ORIENTED_EDGE('',*,*,#19626,.T.);
#26058=ORIENTED_EDGE('',*,*,#19649,.T.);
#26059=ORIENTED_EDGE('',*,*,#17945,.T.);
#26060=ORIENTED_EDGE('',*,*,#19650,.T.);
#26061=ORIENTED_EDGE('',*,*,#19624,.T.);
#26062=ORIENTED_EDGE('',*,*,#19651,.T.);
#26063=ORIENTED_EDGE('',*,*,#19639,.F.);
#26064=ORIENTED_EDGE('',*,*,#19643,.F.);
#26065=ORIENTED_EDGE('',*,*,#19633,.F.);
#26066=ORIENTED_EDGE('',*,*,#17942,.F.);
#26067=ORIENTED_EDGE('',*,*,#19634,.F.);
#26068=ORIENTED_EDGE('',*,*,#19644,.F.);
#26069=ORIENTED_EDGE('',*,*,#19650,.F.);
#26070=ORIENTED_EDGE('',*,*,#17944,.F.);
#26071=ORIENTED_EDGE('',*,*,#19640,.F.);
#26072=ORIENTED_EDGE('',*,*,#19649,.F.);
#26073=ORIENTED_EDGE('',*,*,#19645,.F.);
#26074=ORIENTED_EDGE('',*,*,#19642,.F.);
#26075=ORIENTED_EDGE('',*,*,#19652,.F.);
#26076=ORIENTED_EDGE('',*,*,#19653,.F.);
#26077=ORIENTED_EDGE('',*,*,#19654,.F.);
#26078=ORIENTED_EDGE('',*,*,#19655,.F.);
#26079=ORIENTED_EDGE('',*,*,#19656,.F.);
#26080=ORIENTED_EDGE('',*,*,#19657,.F.);
#26081=ORIENTED_EDGE('',*,*,#19658,.F.);
#26082=ORIENTED_EDGE('',*,*,#19659,.F.);
#26083=ORIENTED_EDGE('',*,*,#19660,.F.);
#26084=ORIENTED_EDGE('',*,*,#17951,.T.);
#26085=ORIENTED_EDGE('',*,*,#19661,.T.);
#26086=ORIENTED_EDGE('',*,*,#19659,.T.);
#26087=ORIENTED_EDGE('',*,*,#19662,.T.);
#26088=ORIENTED_EDGE('',*,*,#19663,.F.);
#26089=ORIENTED_EDGE('',*,*,#19664,.F.);
#26090=ORIENTED_EDGE('',*,*,#19665,.F.);
#26091=ORIENTED_EDGE('',*,*,#17949,.T.);
#26092=ORIENTED_EDGE('',*,*,#19666,.T.);
#26093=ORIENTED_EDGE('',*,*,#19664,.T.);
#26094=ORIENTED_EDGE('',*,*,#19667,.T.);
#26095=ORIENTED_EDGE('',*,*,#19656,.T.);
#26096=ORIENTED_EDGE('',*,*,#19668,.T.);
#26097=ORIENTED_EDGE('',*,*,#19665,.T.);
#26098=ORIENTED_EDGE('',*,*,#19669,.T.);
#26099=ORIENTED_EDGE('',*,*,#19663,.T.);
#26100=ORIENTED_EDGE('',*,*,#19670,.T.);
#26101=ORIENTED_EDGE('',*,*,#19660,.T.);
#26102=ORIENTED_EDGE('',*,*,#19671,.T.);
#26103=ORIENTED_EDGE('',*,*,#19653,.T.);
#26104=ORIENTED_EDGE('',*,*,#19672,.T.);
#26105=ORIENTED_EDGE('',*,*,#19658,.T.);
#26106=ORIENTED_EDGE('',*,*,#19673,.T.);
#26107=ORIENTED_EDGE('',*,*,#17955,.T.);
#26108=ORIENTED_EDGE('',*,*,#19674,.T.);
#26109=ORIENTED_EDGE('',*,*,#19657,.T.);
#26110=ORIENTED_EDGE('',*,*,#19675,.T.);
#26111=ORIENTED_EDGE('',*,*,#19655,.T.);
#26112=ORIENTED_EDGE('',*,*,#19676,.T.);
#26113=ORIENTED_EDGE('',*,*,#19654,.T.);
#26114=ORIENTED_EDGE('',*,*,#19677,.T.);
#26115=ORIENTED_EDGE('',*,*,#17953,.T.);
#26116=ORIENTED_EDGE('',*,*,#19678,.T.);
#26117=ORIENTED_EDGE('',*,*,#19652,.T.);
#26118=ORIENTED_EDGE('',*,*,#19679,.T.);
#26119=ORIENTED_EDGE('',*,*,#19667,.F.);
#26120=ORIENTED_EDGE('',*,*,#19671,.F.);
#26121=ORIENTED_EDGE('',*,*,#19661,.F.);
#26122=ORIENTED_EDGE('',*,*,#17950,.F.);
#26123=ORIENTED_EDGE('',*,*,#19662,.F.);
#26124=ORIENTED_EDGE('',*,*,#19672,.F.);
#26125=ORIENTED_EDGE('',*,*,#19678,.F.);
#26126=ORIENTED_EDGE('',*,*,#17952,.F.);
#26127=ORIENTED_EDGE('',*,*,#19668,.F.);
#26128=ORIENTED_EDGE('',*,*,#19677,.F.);
#26129=ORIENTED_EDGE('',*,*,#19673,.F.);
#26130=ORIENTED_EDGE('',*,*,#19670,.F.);
#26131=ORIENTED_EDGE('',*,*,#19680,.T.);
#26132=ORIENTED_EDGE('',*,*,#19681,.T.);
#26133=ORIENTED_EDGE('',*,*,#17961,.T.);
#26134=ORIENTED_EDGE('',*,*,#19682,.T.);
#26135=ORIENTED_EDGE('',*,*,#19683,.T.);
#26136=ORIENTED_EDGE('',*,*,#19681,.F.);
#26137=ORIENTED_EDGE('',*,*,#19684,.F.);
#26138=ORIENTED_EDGE('',*,*,#19685,.F.);
#26139=ORIENTED_EDGE('',*,*,#17962,.F.);
#26140=ORIENTED_EDGE('',*,*,#19680,.F.);
#26141=ORIENTED_EDGE('',*,*,#19686,.F.);
#26142=ORIENTED_EDGE('',*,*,#19687,.T.);
#26143=ORIENTED_EDGE('',*,*,#19688,.T.);
#26144=ORIENTED_EDGE('',*,*,#19684,.T.);
#26145=ORIENTED_EDGE('',*,*,#19683,.F.);
#26146=ORIENTED_EDGE('',*,*,#19689,.T.);
#26147=ORIENTED_EDGE('',*,*,#19690,.T.);
#26148=ORIENTED_EDGE('',*,*,#19691,.T.);
#26149=ORIENTED_EDGE('',*,*,#19686,.T.);
#26150=ORIENTED_EDGE('',*,*,#19688,.F.);
#26151=ORIENTED_EDGE('',*,*,#19692,.F.);
#26152=ORIENTED_EDGE('',*,*,#19693,.F.);
#26153=ORIENTED_EDGE('',*,*,#19690,.F.);
#26154=ORIENTED_EDGE('',*,*,#19694,.F.);
#26155=ORIENTED_EDGE('',*,*,#19695,.F.);
#26156=ORIENTED_EDGE('',*,*,#17959,.T.);
#26157=ORIENTED_EDGE('',*,*,#19696,.T.);
#26158=ORIENTED_EDGE('',*,*,#19694,.T.);
#26159=ORIENTED_EDGE('',*,*,#19697,.T.);
#26160=ORIENTED_EDGE('',*,*,#19698,.F.);
#26161=ORIENTED_EDGE('',*,*,#19699,.F.);
#26162=ORIENTED_EDGE('',*,*,#19700,.F.);
#26163=ORIENTED_EDGE('',*,*,#17957,.T.);
#26164=ORIENTED_EDGE('',*,*,#19701,.T.);
#26165=ORIENTED_EDGE('',*,*,#19699,.T.);
#26166=ORIENTED_EDGE('',*,*,#19702,.T.);
#26167=ORIENTED_EDGE('',*,*,#19692,.T.);
#26168=ORIENTED_EDGE('',*,*,#19703,.T.);
#26169=ORIENTED_EDGE('',*,*,#19700,.T.);
#26170=ORIENTED_EDGE('',*,*,#19704,.T.);
#26171=ORIENTED_EDGE('',*,*,#19698,.T.);
#26172=ORIENTED_EDGE('',*,*,#19705,.T.);
#26173=ORIENTED_EDGE('',*,*,#19695,.T.);
#26174=ORIENTED_EDGE('',*,*,#19706,.T.);
#26175=ORIENTED_EDGE('',*,*,#17963,.T.);
#26176=ORIENTED_EDGE('',*,*,#19685,.T.);
#26177=ORIENTED_EDGE('',*,*,#19693,.T.);
#26178=ORIENTED_EDGE('',*,*,#19707,.T.);
#26179=ORIENTED_EDGE('',*,*,#19682,.F.);
#26180=ORIENTED_EDGE('',*,*,#17960,.F.);
#26181=ORIENTED_EDGE('',*,*,#19697,.F.);
#26182=ORIENTED_EDGE('',*,*,#19689,.F.);
#26183=ORIENTED_EDGE('',*,*,#19703,.F.);
#26184=ORIENTED_EDGE('',*,*,#19687,.F.);
#26185=ORIENTED_EDGE('',*,*,#19691,.F.);
#26186=ORIENTED_EDGE('',*,*,#19705,.F.);
#26187=ORIENTED_EDGE('',*,*,#19708,.F.);
#26188=ORIENTED_EDGE('',*,*,#19709,.F.);
#26189=ORIENTED_EDGE('',*,*,#19710,.F.);
#26190=ORIENTED_EDGE('',*,*,#19711,.F.);
#26191=ORIENTED_EDGE('',*,*,#19712,.F.);
#26192=ORIENTED_EDGE('',*,*,#19713,.F.);
#26193=ORIENTED_EDGE('',*,*,#19714,.F.);
#26194=ORIENTED_EDGE('',*,*,#19715,.F.);
#26195=ORIENTED_EDGE('',*,*,#19716,.F.);
#26196=ORIENTED_EDGE('',*,*,#17967,.T.);
#26197=ORIENTED_EDGE('',*,*,#19717,.T.);
#26198=ORIENTED_EDGE('',*,*,#19715,.T.);
#26199=ORIENTED_EDGE('',*,*,#19718,.T.);
#26200=ORIENTED_EDGE('',*,*,#19719,.F.);
#26201=ORIENTED_EDGE('',*,*,#19720,.F.);
#26202=ORIENTED_EDGE('',*,*,#19721,.F.);
#26203=ORIENTED_EDGE('',*,*,#17965,.T.);
#26204=ORIENTED_EDGE('',*,*,#19722,.T.);
#26205=ORIENTED_EDGE('',*,*,#19720,.T.);
#26206=ORIENTED_EDGE('',*,*,#19723,.T.);
#26207=ORIENTED_EDGE('',*,*,#19712,.T.);
#26208=ORIENTED_EDGE('',*,*,#19724,.T.);
#26209=ORIENTED_EDGE('',*,*,#19721,.T.);
#26210=ORIENTED_EDGE('',*,*,#19725,.T.);
#26211=ORIENTED_EDGE('',*,*,#19719,.T.);
#26212=ORIENTED_EDGE('',*,*,#19726,.T.);
#26213=ORIENTED_EDGE('',*,*,#19716,.T.);
#26214=ORIENTED_EDGE('',*,*,#19727,.T.);
#26215=ORIENTED_EDGE('',*,*,#19709,.T.);
#26216=ORIENTED_EDGE('',*,*,#19728,.T.);
#26217=ORIENTED_EDGE('',*,*,#19714,.T.);
#26218=ORIENTED_EDGE('',*,*,#19729,.T.);
#26219=ORIENTED_EDGE('',*,*,#17971,.T.);
#26220=ORIENTED_EDGE('',*,*,#19730,.T.);
#26221=ORIENTED_EDGE('',*,*,#19713,.T.);
#26222=ORIENTED_EDGE('',*,*,#19731,.T.);
#26223=ORIENTED_EDGE('',*,*,#19711,.T.);
#26224=ORIENTED_EDGE('',*,*,#19732,.T.);
#26225=ORIENTED_EDGE('',*,*,#19710,.T.);
#26226=ORIENTED_EDGE('',*,*,#19733,.T.);
#26227=ORIENTED_EDGE('',*,*,#17969,.T.);
#26228=ORIENTED_EDGE('',*,*,#19734,.T.);
#26229=ORIENTED_EDGE('',*,*,#19708,.T.);
#26230=ORIENTED_EDGE('',*,*,#19735,.T.);
#26231=ORIENTED_EDGE('',*,*,#19723,.F.);
#26232=ORIENTED_EDGE('',*,*,#19727,.F.);
#26233=ORIENTED_EDGE('',*,*,#19717,.F.);
#26234=ORIENTED_EDGE('',*,*,#17966,.F.);
#26235=ORIENTED_EDGE('',*,*,#19718,.F.);
#26236=ORIENTED_EDGE('',*,*,#19728,.F.);
#26237=ORIENTED_EDGE('',*,*,#19734,.F.);
#26238=ORIENTED_EDGE('',*,*,#17968,.F.);
#26239=ORIENTED_EDGE('',*,*,#19724,.F.);
#26240=ORIENTED_EDGE('',*,*,#19733,.F.);
#26241=ORIENTED_EDGE('',*,*,#19729,.F.);
#26242=ORIENTED_EDGE('',*,*,#19726,.F.);
#26243=ORIENTED_EDGE('',*,*,#19736,.F.);
#26244=ORIENTED_EDGE('',*,*,#19737,.F.);
#26245=ORIENTED_EDGE('',*,*,#19738,.F.);
#26246=ORIENTED_EDGE('',*,*,#19739,.T.);
#26247=ORIENTED_EDGE('',*,*,#19740,.T.);
#26248=ORIENTED_EDGE('',*,*,#19737,.T.);
#26249=ORIENTED_EDGE('',*,*,#19741,.T.);
#26250=ORIENTED_EDGE('',*,*,#19742,.T.);
#26251=ORIENTED_EDGE('',*,*,#17979,.T.);
#26252=ORIENTED_EDGE('',*,*,#19743,.T.);
#26253=ORIENTED_EDGE('',*,*,#19738,.T.);
#26254=ORIENTED_EDGE('',*,*,#19744,.T.);
#26255=ORIENTED_EDGE('',*,*,#19745,.F.);
#26256=ORIENTED_EDGE('',*,*,#19746,.F.);
#26257=ORIENTED_EDGE('',*,*,#19747,.F.);
#26258=ORIENTED_EDGE('',*,*,#19748,.T.);
#26259=ORIENTED_EDGE('',*,*,#19749,.T.);
#26260=ORIENTED_EDGE('',*,*,#19746,.T.);
#26261=ORIENTED_EDGE('',*,*,#19750,.T.);
#26262=ORIENTED_EDGE('',*,*,#19751,.T.);
#26263=ORIENTED_EDGE('',*,*,#19736,.T.);
#26264=ORIENTED_EDGE('',*,*,#19752,.T.);
#26265=ORIENTED_EDGE('',*,*,#19747,.T.);
#26266=ORIENTED_EDGE('',*,*,#19753,.T.);
#26267=ORIENTED_EDGE('',*,*,#17977,.T.);
#26268=ORIENTED_EDGE('',*,*,#19754,.T.);
#26269=ORIENTED_EDGE('',*,*,#19745,.T.);
#26270=ORIENTED_EDGE('',*,*,#19755,.T.);
#26271=ORIENTED_EDGE('',*,*,#19739,.F.);
#26272=ORIENTED_EDGE('',*,*,#19756,.T.);
#26273=ORIENTED_EDGE('',*,*,#19757,.T.);
#26274=ORIENTED_EDGE('',*,*,#17973,.T.);
#26275=ORIENTED_EDGE('',*,*,#19758,.T.);
#26276=ORIENTED_EDGE('',*,*,#19741,.F.);
#26277=ORIENTED_EDGE('',*,*,#19753,.F.);
#26278=ORIENTED_EDGE('',*,*,#19749,.F.);
#26279=ORIENTED_EDGE('',*,*,#19759,.F.);
#26280=ORIENTED_EDGE('',*,*,#19742,.F.);
#26281=ORIENTED_EDGE('',*,*,#19759,.T.);
#26282=ORIENTED_EDGE('',*,*,#19748,.F.);
#26283=ORIENTED_EDGE('',*,*,#19760,.F.);
#26284=ORIENTED_EDGE('',*,*,#19761,.T.);
#26285=ORIENTED_EDGE('',*,*,#19756,.F.);
#26286=ORIENTED_EDGE('',*,*,#19751,.F.);
#26287=ORIENTED_EDGE('',*,*,#19762,.T.);
#26288=ORIENTED_EDGE('',*,*,#17975,.T.);
#26289=ORIENTED_EDGE('',*,*,#19763,.T.);
#26290=ORIENTED_EDGE('',*,*,#19760,.T.);
#26291=ORIENTED_EDGE('',*,*,#19750,.F.);
#26292=ORIENTED_EDGE('',*,*,#19754,.F.);
#26293=ORIENTED_EDGE('',*,*,#17976,.F.);
#26294=ORIENTED_EDGE('',*,*,#19762,.F.);
#26295=ORIENTED_EDGE('',*,*,#19740,.F.);
#26296=ORIENTED_EDGE('',*,*,#19758,.F.);
#26297=ORIENTED_EDGE('',*,*,#17972,.F.);
#26298=ORIENTED_EDGE('',*,*,#19744,.F.);
#26299=ORIENTED_EDGE('',*,*,#19764,.F.);
#26300=ORIENTED_EDGE('',*,*,#19765,.F.);
#26301=ORIENTED_EDGE('',*,*,#19766,.F.);
#26302=ORIENTED_EDGE('',*,*,#19767,.F.);
#26303=ORIENTED_EDGE('',*,*,#19768,.F.);
#26304=ORIENTED_EDGE('',*,*,#19769,.F.);
#26305=ORIENTED_EDGE('',*,*,#19770,.F.);
#26306=ORIENTED_EDGE('',*,*,#19771,.F.);
#26307=ORIENTED_EDGE('',*,*,#19772,.F.);
#26308=ORIENTED_EDGE('',*,*,#17983,.T.);
#26309=ORIENTED_EDGE('',*,*,#19773,.T.);
#26310=ORIENTED_EDGE('',*,*,#19771,.T.);
#26311=ORIENTED_EDGE('',*,*,#19774,.T.);
#26312=ORIENTED_EDGE('',*,*,#19775,.F.);
#26313=ORIENTED_EDGE('',*,*,#19776,.F.);
#26314=ORIENTED_EDGE('',*,*,#19777,.F.);
#26315=ORIENTED_EDGE('',*,*,#17981,.T.);
#26316=ORIENTED_EDGE('',*,*,#19778,.T.);
#26317=ORIENTED_EDGE('',*,*,#19776,.T.);
#26318=ORIENTED_EDGE('',*,*,#19779,.T.);
#26319=ORIENTED_EDGE('',*,*,#19768,.T.);
#26320=ORIENTED_EDGE('',*,*,#19780,.T.);
#26321=ORIENTED_EDGE('',*,*,#19777,.T.);
#26322=ORIENTED_EDGE('',*,*,#19781,.T.);
#26323=ORIENTED_EDGE('',*,*,#19775,.T.);
#26324=ORIENTED_EDGE('',*,*,#19782,.T.);
#26325=ORIENTED_EDGE('',*,*,#19772,.T.);
#26326=ORIENTED_EDGE('',*,*,#19783,.T.);
#26327=ORIENTED_EDGE('',*,*,#19765,.T.);
#26328=ORIENTED_EDGE('',*,*,#19784,.T.);
#26329=ORIENTED_EDGE('',*,*,#19770,.T.);
#26330=ORIENTED_EDGE('',*,*,#19785,.T.);
#26331=ORIENTED_EDGE('',*,*,#17987,.T.);
#26332=ORIENTED_EDGE('',*,*,#19786,.T.);
#26333=ORIENTED_EDGE('',*,*,#19769,.T.);
#26334=ORIENTED_EDGE('',*,*,#19787,.T.);
#26335=ORIENTED_EDGE('',*,*,#19767,.T.);
#26336=ORIENTED_EDGE('',*,*,#19788,.T.);
#26337=ORIENTED_EDGE('',*,*,#19766,.T.);
#26338=ORIENTED_EDGE('',*,*,#19789,.T.);
#26339=ORIENTED_EDGE('',*,*,#17985,.T.);
#26340=ORIENTED_EDGE('',*,*,#19790,.T.);
#26341=ORIENTED_EDGE('',*,*,#19764,.T.);
#26342=ORIENTED_EDGE('',*,*,#19791,.T.);
#26343=ORIENTED_EDGE('',*,*,#19779,.F.);
#26344=ORIENTED_EDGE('',*,*,#19783,.F.);
#26345=ORIENTED_EDGE('',*,*,#19773,.F.);
#26346=ORIENTED_EDGE('',*,*,#17982,.F.);
#26347=ORIENTED_EDGE('',*,*,#19774,.F.);
#26348=ORIENTED_EDGE('',*,*,#19784,.F.);
#26349=ORIENTED_EDGE('',*,*,#19790,.F.);
#26350=ORIENTED_EDGE('',*,*,#17984,.F.);
#26351=ORIENTED_EDGE('',*,*,#19780,.F.);
#26352=ORIENTED_EDGE('',*,*,#19789,.F.);
#26353=ORIENTED_EDGE('',*,*,#19785,.F.);
#26354=ORIENTED_EDGE('',*,*,#19782,.F.);
#26355=ORIENTED_EDGE('',*,*,#19792,.F.);
#26356=ORIENTED_EDGE('',*,*,#19793,.F.);
#26357=ORIENTED_EDGE('',*,*,#19794,.F.);
#26358=ORIENTED_EDGE('',*,*,#19795,.F.);
#26359=ORIENTED_EDGE('',*,*,#19796,.F.);
#26360=ORIENTED_EDGE('',*,*,#19797,.F.);
#26361=ORIENTED_EDGE('',*,*,#19798,.F.);
#26362=ORIENTED_EDGE('',*,*,#19799,.F.);
#26363=ORIENTED_EDGE('',*,*,#19800,.F.);
#26364=ORIENTED_EDGE('',*,*,#17991,.T.);
#26365=ORIENTED_EDGE('',*,*,#19801,.T.);
#26366=ORIENTED_EDGE('',*,*,#19799,.T.);
#26367=ORIENTED_EDGE('',*,*,#19802,.T.);
#26368=ORIENTED_EDGE('',*,*,#19803,.F.);
#26369=ORIENTED_EDGE('',*,*,#19804,.F.);
#26370=ORIENTED_EDGE('',*,*,#19805,.F.);
#26371=ORIENTED_EDGE('',*,*,#17989,.T.);
#26372=ORIENTED_EDGE('',*,*,#19806,.T.);
#26373=ORIENTED_EDGE('',*,*,#19804,.T.);
#26374=ORIENTED_EDGE('',*,*,#19807,.T.);
#26375=ORIENTED_EDGE('',*,*,#19796,.T.);
#26376=ORIENTED_EDGE('',*,*,#19808,.T.);
#26377=ORIENTED_EDGE('',*,*,#19805,.T.);
#26378=ORIENTED_EDGE('',*,*,#19809,.T.);
#26379=ORIENTED_EDGE('',*,*,#19803,.T.);
#26380=ORIENTED_EDGE('',*,*,#19810,.T.);
#26381=ORIENTED_EDGE('',*,*,#19800,.T.);
#26382=ORIENTED_EDGE('',*,*,#19811,.T.);
#26383=ORIENTED_EDGE('',*,*,#19793,.T.);
#26384=ORIENTED_EDGE('',*,*,#19812,.T.);
#26385=ORIENTED_EDGE('',*,*,#19798,.T.);
#26386=ORIENTED_EDGE('',*,*,#19813,.T.);
#26387=ORIENTED_EDGE('',*,*,#17995,.T.);
#26388=ORIENTED_EDGE('',*,*,#19814,.T.);
#26389=ORIENTED_EDGE('',*,*,#19797,.T.);
#26390=ORIENTED_EDGE('',*,*,#19815,.T.);
#26391=ORIENTED_EDGE('',*,*,#19795,.T.);
#26392=ORIENTED_EDGE('',*,*,#19816,.T.);
#26393=ORIENTED_EDGE('',*,*,#19794,.T.);
#26394=ORIENTED_EDGE('',*,*,#19817,.T.);
#26395=ORIENTED_EDGE('',*,*,#17993,.T.);
#26396=ORIENTED_EDGE('',*,*,#19818,.T.);
#26397=ORIENTED_EDGE('',*,*,#19792,.T.);
#26398=ORIENTED_EDGE('',*,*,#19819,.T.);
#26399=ORIENTED_EDGE('',*,*,#19807,.F.);
#26400=ORIENTED_EDGE('',*,*,#19811,.F.);
#26401=ORIENTED_EDGE('',*,*,#19801,.F.);
#26402=ORIENTED_EDGE('',*,*,#17990,.F.);
#26403=ORIENTED_EDGE('',*,*,#19802,.F.);
#26404=ORIENTED_EDGE('',*,*,#19812,.F.);
#26405=ORIENTED_EDGE('',*,*,#19818,.F.);
#26406=ORIENTED_EDGE('',*,*,#17992,.F.);
#26407=ORIENTED_EDGE('',*,*,#19808,.F.);
#26408=ORIENTED_EDGE('',*,*,#19817,.F.);
#26409=ORIENTED_EDGE('',*,*,#19813,.F.);
#26410=ORIENTED_EDGE('',*,*,#19810,.F.);
#26411=ORIENTED_EDGE('',*,*,#19820,.T.);
#26412=ORIENTED_EDGE('',*,*,#19821,.T.);
#26413=ORIENTED_EDGE('',*,*,#18001,.T.);
#26414=ORIENTED_EDGE('',*,*,#19822,.T.);
#26415=ORIENTED_EDGE('',*,*,#19823,.T.);
#26416=ORIENTED_EDGE('',*,*,#19821,.F.);
#26417=ORIENTED_EDGE('',*,*,#19824,.F.);
#26418=ORIENTED_EDGE('',*,*,#19825,.F.);
#26419=ORIENTED_EDGE('',*,*,#18002,.F.);
#26420=ORIENTED_EDGE('',*,*,#19820,.F.);
#26421=ORIENTED_EDGE('',*,*,#19826,.F.);
#26422=ORIENTED_EDGE('',*,*,#19827,.T.);
#26423=ORIENTED_EDGE('',*,*,#19828,.T.);
#26424=ORIENTED_EDGE('',*,*,#19824,.T.);
#26425=ORIENTED_EDGE('',*,*,#19823,.F.);
#26426=ORIENTED_EDGE('',*,*,#19829,.T.);
#26427=ORIENTED_EDGE('',*,*,#19830,.T.);
#26428=ORIENTED_EDGE('',*,*,#19831,.T.);
#26429=ORIENTED_EDGE('',*,*,#19826,.T.);
#26430=ORIENTED_EDGE('',*,*,#19828,.F.);
#26431=ORIENTED_EDGE('',*,*,#19832,.F.);
#26432=ORIENTED_EDGE('',*,*,#19833,.F.);
#26433=ORIENTED_EDGE('',*,*,#19830,.F.);
#26434=ORIENTED_EDGE('',*,*,#19834,.F.);
#26435=ORIENTED_EDGE('',*,*,#19835,.F.);
#26436=ORIENTED_EDGE('',*,*,#17999,.T.);
#26437=ORIENTED_EDGE('',*,*,#19836,.T.);
#26438=ORIENTED_EDGE('',*,*,#19834,.T.);
#26439=ORIENTED_EDGE('',*,*,#19837,.T.);
#26440=ORIENTED_EDGE('',*,*,#19838,.F.);
#26441=ORIENTED_EDGE('',*,*,#19839,.F.);
#26442=ORIENTED_EDGE('',*,*,#19840,.F.);
#26443=ORIENTED_EDGE('',*,*,#17997,.T.);
#26444=ORIENTED_EDGE('',*,*,#19841,.T.);
#26445=ORIENTED_EDGE('',*,*,#19839,.T.);
#26446=ORIENTED_EDGE('',*,*,#19842,.T.);
#26447=ORIENTED_EDGE('',*,*,#19832,.T.);
#26448=ORIENTED_EDGE('',*,*,#19843,.T.);
#26449=ORIENTED_EDGE('',*,*,#19840,.T.);
#26450=ORIENTED_EDGE('',*,*,#19844,.T.);
#26451=ORIENTED_EDGE('',*,*,#19838,.T.);
#26452=ORIENTED_EDGE('',*,*,#19845,.T.);
#26453=ORIENTED_EDGE('',*,*,#19835,.T.);
#26454=ORIENTED_EDGE('',*,*,#19846,.T.);
#26455=ORIENTED_EDGE('',*,*,#18003,.T.);
#26456=ORIENTED_EDGE('',*,*,#19825,.T.);
#26457=ORIENTED_EDGE('',*,*,#19833,.T.);
#26458=ORIENTED_EDGE('',*,*,#19847,.T.);
#26459=ORIENTED_EDGE('',*,*,#19822,.F.);
#26460=ORIENTED_EDGE('',*,*,#18000,.F.);
#26461=ORIENTED_EDGE('',*,*,#19837,.F.);
#26462=ORIENTED_EDGE('',*,*,#19829,.F.);
#26463=ORIENTED_EDGE('',*,*,#19843,.F.);
#26464=ORIENTED_EDGE('',*,*,#19827,.F.);
#26465=ORIENTED_EDGE('',*,*,#19831,.F.);
#26466=ORIENTED_EDGE('',*,*,#19845,.F.);
#26467=ORIENTED_EDGE('',*,*,#19848,.F.);
#26468=ORIENTED_EDGE('',*,*,#19849,.F.);
#26469=ORIENTED_EDGE('',*,*,#19850,.F.);
#26470=ORIENTED_EDGE('',*,*,#19851,.F.);
#26471=ORIENTED_EDGE('',*,*,#19852,.F.);
#26472=ORIENTED_EDGE('',*,*,#19853,.F.);
#26473=ORIENTED_EDGE('',*,*,#19854,.F.);
#26474=ORIENTED_EDGE('',*,*,#19855,.F.);
#26475=ORIENTED_EDGE('',*,*,#19856,.F.);
#26476=ORIENTED_EDGE('',*,*,#18007,.T.);
#26477=ORIENTED_EDGE('',*,*,#19857,.T.);
#26478=ORIENTED_EDGE('',*,*,#19855,.T.);
#26479=ORIENTED_EDGE('',*,*,#19858,.T.);
#26480=ORIENTED_EDGE('',*,*,#19859,.F.);
#26481=ORIENTED_EDGE('',*,*,#19860,.F.);
#26482=ORIENTED_EDGE('',*,*,#19861,.F.);
#26483=ORIENTED_EDGE('',*,*,#18005,.T.);
#26484=ORIENTED_EDGE('',*,*,#19862,.T.);
#26485=ORIENTED_EDGE('',*,*,#19860,.T.);
#26486=ORIENTED_EDGE('',*,*,#19863,.T.);
#26487=ORIENTED_EDGE('',*,*,#19852,.T.);
#26488=ORIENTED_EDGE('',*,*,#19864,.T.);
#26489=ORIENTED_EDGE('',*,*,#19861,.T.);
#26490=ORIENTED_EDGE('',*,*,#19865,.T.);
#26491=ORIENTED_EDGE('',*,*,#19859,.T.);
#26492=ORIENTED_EDGE('',*,*,#19866,.T.);
#26493=ORIENTED_EDGE('',*,*,#19856,.T.);
#26494=ORIENTED_EDGE('',*,*,#19867,.T.);
#26495=ORIENTED_EDGE('',*,*,#19849,.T.);
#26496=ORIENTED_EDGE('',*,*,#19868,.T.);
#26497=ORIENTED_EDGE('',*,*,#19854,.T.);
#26498=ORIENTED_EDGE('',*,*,#19869,.T.);
#26499=ORIENTED_EDGE('',*,*,#18011,.T.);
#26500=ORIENTED_EDGE('',*,*,#19870,.T.);
#26501=ORIENTED_EDGE('',*,*,#19853,.T.);
#26502=ORIENTED_EDGE('',*,*,#19871,.T.);
#26503=ORIENTED_EDGE('',*,*,#19851,.T.);
#26504=ORIENTED_EDGE('',*,*,#19872,.T.);
#26505=ORIENTED_EDGE('',*,*,#19850,.T.);
#26506=ORIENTED_EDGE('',*,*,#19873,.T.);
#26507=ORIENTED_EDGE('',*,*,#18009,.T.);
#26508=ORIENTED_EDGE('',*,*,#19874,.T.);
#26509=ORIENTED_EDGE('',*,*,#19848,.T.);
#26510=ORIENTED_EDGE('',*,*,#19875,.T.);
#26511=ORIENTED_EDGE('',*,*,#19863,.F.);
#26512=ORIENTED_EDGE('',*,*,#19867,.F.);
#26513=ORIENTED_EDGE('',*,*,#19857,.F.);
#26514=ORIENTED_EDGE('',*,*,#18006,.F.);
#26515=ORIENTED_EDGE('',*,*,#19858,.F.);
#26516=ORIENTED_EDGE('',*,*,#19868,.F.);
#26517=ORIENTED_EDGE('',*,*,#19874,.F.);
#26518=ORIENTED_EDGE('',*,*,#18008,.F.);
#26519=ORIENTED_EDGE('',*,*,#19864,.F.);
#26520=ORIENTED_EDGE('',*,*,#19873,.F.);
#26521=ORIENTED_EDGE('',*,*,#19869,.F.);
#26522=ORIENTED_EDGE('',*,*,#19866,.F.);
#26523=ORIENTED_EDGE('',*,*,#19876,.F.);
#26524=ORIENTED_EDGE('',*,*,#19877,.F.);
#26525=ORIENTED_EDGE('',*,*,#19878,.F.);
#26526=ORIENTED_EDGE('',*,*,#19879,.T.);
#26527=ORIENTED_EDGE('',*,*,#19880,.T.);
#26528=ORIENTED_EDGE('',*,*,#19877,.T.);
#26529=ORIENTED_EDGE('',*,*,#19881,.T.);
#26530=ORIENTED_EDGE('',*,*,#19882,.T.);
#26531=ORIENTED_EDGE('',*,*,#18019,.T.);
#26532=ORIENTED_EDGE('',*,*,#19883,.T.);
#26533=ORIENTED_EDGE('',*,*,#19878,.T.);
#26534=ORIENTED_EDGE('',*,*,#19884,.T.);
#26535=ORIENTED_EDGE('',*,*,#19885,.F.);
#26536=ORIENTED_EDGE('',*,*,#19886,.F.);
#26537=ORIENTED_EDGE('',*,*,#19887,.F.);
#26538=ORIENTED_EDGE('',*,*,#19888,.T.);
#26539=ORIENTED_EDGE('',*,*,#19889,.T.);
#26540=ORIENTED_EDGE('',*,*,#19886,.T.);
#26541=ORIENTED_EDGE('',*,*,#19890,.T.);
#26542=ORIENTED_EDGE('',*,*,#19891,.T.);
#26543=ORIENTED_EDGE('',*,*,#19876,.T.);
#26544=ORIENTED_EDGE('',*,*,#19892,.T.);
#26545=ORIENTED_EDGE('',*,*,#19887,.T.);
#26546=ORIENTED_EDGE('',*,*,#19893,.T.);
#26547=ORIENTED_EDGE('',*,*,#18017,.T.);
#26548=ORIENTED_EDGE('',*,*,#19894,.T.);
#26549=ORIENTED_EDGE('',*,*,#19885,.T.);
#26550=ORIENTED_EDGE('',*,*,#19895,.T.);
#26551=ORIENTED_EDGE('',*,*,#19879,.F.);
#26552=ORIENTED_EDGE('',*,*,#19896,.T.);
#26553=ORIENTED_EDGE('',*,*,#19897,.T.);
#26554=ORIENTED_EDGE('',*,*,#18013,.T.);
#26555=ORIENTED_EDGE('',*,*,#19898,.T.);
#26556=ORIENTED_EDGE('',*,*,#19881,.F.);
#26557=ORIENTED_EDGE('',*,*,#19893,.F.);
#26558=ORIENTED_EDGE('',*,*,#19889,.F.);
#26559=ORIENTED_EDGE('',*,*,#19899,.F.);
#26560=ORIENTED_EDGE('',*,*,#19882,.F.);
#26561=ORIENTED_EDGE('',*,*,#19899,.T.);
#26562=ORIENTED_EDGE('',*,*,#19888,.F.);
#26563=ORIENTED_EDGE('',*,*,#19900,.F.);
#26564=ORIENTED_EDGE('',*,*,#19901,.T.);
#26565=ORIENTED_EDGE('',*,*,#19896,.F.);
#26566=ORIENTED_EDGE('',*,*,#19891,.F.);
#26567=ORIENTED_EDGE('',*,*,#19902,.T.);
#26568=ORIENTED_EDGE('',*,*,#18015,.T.);
#26569=ORIENTED_EDGE('',*,*,#19903,.T.);
#26570=ORIENTED_EDGE('',*,*,#19900,.T.);
#26571=ORIENTED_EDGE('',*,*,#19890,.F.);
#26572=ORIENTED_EDGE('',*,*,#19894,.F.);
#26573=ORIENTED_EDGE('',*,*,#18016,.F.);
#26574=ORIENTED_EDGE('',*,*,#19902,.F.);
#26575=ORIENTED_EDGE('',*,*,#19880,.F.);
#26576=ORIENTED_EDGE('',*,*,#19898,.F.);
#26577=ORIENTED_EDGE('',*,*,#18012,.F.);
#26578=ORIENTED_EDGE('',*,*,#19884,.F.);
#26579=ORIENTED_EDGE('',*,*,#19904,.F.);
#26580=ORIENTED_EDGE('',*,*,#19905,.F.);
#26581=ORIENTED_EDGE('',*,*,#19906,.F.);
#26582=ORIENTED_EDGE('',*,*,#19907,.F.);
#26583=ORIENTED_EDGE('',*,*,#19908,.F.);
#26584=ORIENTED_EDGE('',*,*,#19909,.F.);
#26585=ORIENTED_EDGE('',*,*,#19910,.F.);
#26586=ORIENTED_EDGE('',*,*,#19911,.F.);
#26587=ORIENTED_EDGE('',*,*,#19912,.F.);
#26588=ORIENTED_EDGE('',*,*,#18023,.T.);
#26589=ORIENTED_EDGE('',*,*,#19913,.T.);
#26590=ORIENTED_EDGE('',*,*,#19911,.T.);
#26591=ORIENTED_EDGE('',*,*,#19914,.T.);
#26592=ORIENTED_EDGE('',*,*,#19915,.F.);
#26593=ORIENTED_EDGE('',*,*,#19916,.F.);
#26594=ORIENTED_EDGE('',*,*,#19917,.F.);
#26595=ORIENTED_EDGE('',*,*,#18021,.T.);
#26596=ORIENTED_EDGE('',*,*,#19918,.T.);
#26597=ORIENTED_EDGE('',*,*,#19916,.T.);
#26598=ORIENTED_EDGE('',*,*,#19919,.T.);
#26599=ORIENTED_EDGE('',*,*,#19908,.T.);
#26600=ORIENTED_EDGE('',*,*,#19920,.T.);
#26601=ORIENTED_EDGE('',*,*,#19917,.T.);
#26602=ORIENTED_EDGE('',*,*,#19921,.T.);
#26603=ORIENTED_EDGE('',*,*,#19915,.T.);
#26604=ORIENTED_EDGE('',*,*,#19922,.T.);
#26605=ORIENTED_EDGE('',*,*,#19912,.T.);
#26606=ORIENTED_EDGE('',*,*,#19923,.T.);
#26607=ORIENTED_EDGE('',*,*,#19905,.T.);
#26608=ORIENTED_EDGE('',*,*,#19924,.T.);
#26609=ORIENTED_EDGE('',*,*,#19910,.T.);
#26610=ORIENTED_EDGE('',*,*,#19925,.T.);
#26611=ORIENTED_EDGE('',*,*,#18027,.T.);
#26612=ORIENTED_EDGE('',*,*,#19926,.T.);
#26613=ORIENTED_EDGE('',*,*,#19909,.T.);
#26614=ORIENTED_EDGE('',*,*,#19927,.T.);
#26615=ORIENTED_EDGE('',*,*,#19907,.T.);
#26616=ORIENTED_EDGE('',*,*,#19928,.T.);
#26617=ORIENTED_EDGE('',*,*,#19906,.T.);
#26618=ORIENTED_EDGE('',*,*,#19929,.T.);
#26619=ORIENTED_EDGE('',*,*,#18025,.T.);
#26620=ORIENTED_EDGE('',*,*,#19930,.T.);
#26621=ORIENTED_EDGE('',*,*,#19904,.T.);
#26622=ORIENTED_EDGE('',*,*,#19931,.T.);
#26623=ORIENTED_EDGE('',*,*,#19919,.F.);
#26624=ORIENTED_EDGE('',*,*,#19923,.F.);
#26625=ORIENTED_EDGE('',*,*,#19913,.F.);
#26626=ORIENTED_EDGE('',*,*,#18022,.F.);
#26627=ORIENTED_EDGE('',*,*,#19914,.F.);
#26628=ORIENTED_EDGE('',*,*,#19924,.F.);
#26629=ORIENTED_EDGE('',*,*,#19930,.F.);
#26630=ORIENTED_EDGE('',*,*,#18024,.F.);
#26631=ORIENTED_EDGE('',*,*,#19920,.F.);
#26632=ORIENTED_EDGE('',*,*,#19929,.F.);
#26633=ORIENTED_EDGE('',*,*,#19925,.F.);
#26634=ORIENTED_EDGE('',*,*,#19922,.F.);
#26635=ORIENTED_EDGE('',*,*,#19932,.F.);
#26636=ORIENTED_EDGE('',*,*,#19933,.F.);
#26637=ORIENTED_EDGE('',*,*,#19934,.F.);
#26638=ORIENTED_EDGE('',*,*,#19935,.F.);
#26639=ORIENTED_EDGE('',*,*,#19936,.F.);
#26640=ORIENTED_EDGE('',*,*,#19937,.F.);
#26641=ORIENTED_EDGE('',*,*,#19938,.F.);
#26642=ORIENTED_EDGE('',*,*,#19939,.F.);
#26643=ORIENTED_EDGE('',*,*,#19940,.F.);
#26644=ORIENTED_EDGE('',*,*,#18031,.T.);
#26645=ORIENTED_EDGE('',*,*,#19941,.T.);
#26646=ORIENTED_EDGE('',*,*,#19939,.T.);
#26647=ORIENTED_EDGE('',*,*,#19942,.T.);
#26648=ORIENTED_EDGE('',*,*,#19943,.F.);
#26649=ORIENTED_EDGE('',*,*,#19944,.F.);
#26650=ORIENTED_EDGE('',*,*,#19945,.F.);
#26651=ORIENTED_EDGE('',*,*,#18029,.T.);
#26652=ORIENTED_EDGE('',*,*,#19946,.T.);
#26653=ORIENTED_EDGE('',*,*,#19944,.T.);
#26654=ORIENTED_EDGE('',*,*,#19947,.T.);
#26655=ORIENTED_EDGE('',*,*,#19936,.T.);
#26656=ORIENTED_EDGE('',*,*,#19948,.T.);
#26657=ORIENTED_EDGE('',*,*,#19945,.T.);
#26658=ORIENTED_EDGE('',*,*,#19949,.T.);
#26659=ORIENTED_EDGE('',*,*,#19943,.T.);
#26660=ORIENTED_EDGE('',*,*,#19950,.T.);
#26661=ORIENTED_EDGE('',*,*,#19940,.T.);
#26662=ORIENTED_EDGE('',*,*,#19951,.T.);
#26663=ORIENTED_EDGE('',*,*,#19933,.T.);
#26664=ORIENTED_EDGE('',*,*,#19952,.T.);
#26665=ORIENTED_EDGE('',*,*,#19938,.T.);
#26666=ORIENTED_EDGE('',*,*,#19953,.T.);
#26667=ORIENTED_EDGE('',*,*,#18035,.T.);
#26668=ORIENTED_EDGE('',*,*,#19954,.T.);
#26669=ORIENTED_EDGE('',*,*,#19937,.T.);
#26670=ORIENTED_EDGE('',*,*,#19955,.T.);
#26671=ORIENTED_EDGE('',*,*,#19935,.T.);
#26672=ORIENTED_EDGE('',*,*,#19956,.T.);
#26673=ORIENTED_EDGE('',*,*,#19934,.T.);
#26674=ORIENTED_EDGE('',*,*,#19957,.T.);
#26675=ORIENTED_EDGE('',*,*,#18033,.T.);
#26676=ORIENTED_EDGE('',*,*,#19958,.T.);
#26677=ORIENTED_EDGE('',*,*,#19932,.T.);
#26678=ORIENTED_EDGE('',*,*,#19959,.T.);
#26679=ORIENTED_EDGE('',*,*,#19947,.F.);
#26680=ORIENTED_EDGE('',*,*,#19951,.F.);
#26681=ORIENTED_EDGE('',*,*,#19941,.F.);
#26682=ORIENTED_EDGE('',*,*,#18030,.F.);
#26683=ORIENTED_EDGE('',*,*,#19942,.F.);
#26684=ORIENTED_EDGE('',*,*,#19952,.F.);
#26685=ORIENTED_EDGE('',*,*,#19958,.F.);
#26686=ORIENTED_EDGE('',*,*,#18032,.F.);
#26687=ORIENTED_EDGE('',*,*,#19948,.F.);
#26688=ORIENTED_EDGE('',*,*,#19957,.F.);
#26689=ORIENTED_EDGE('',*,*,#19953,.F.);
#26690=ORIENTED_EDGE('',*,*,#19950,.F.);
#26691=ORIENTED_EDGE('',*,*,#19960,.T.);
#26692=ORIENTED_EDGE('',*,*,#19961,.T.);
#26693=ORIENTED_EDGE('',*,*,#18041,.T.);
#26694=ORIENTED_EDGE('',*,*,#19962,.T.);
#26695=ORIENTED_EDGE('',*,*,#19963,.T.);
#26696=ORIENTED_EDGE('',*,*,#19961,.F.);
#26697=ORIENTED_EDGE('',*,*,#19964,.F.);
#26698=ORIENTED_EDGE('',*,*,#19965,.F.);
#26699=ORIENTED_EDGE('',*,*,#18042,.F.);
#26700=ORIENTED_EDGE('',*,*,#19960,.F.);
#26701=ORIENTED_EDGE('',*,*,#19966,.F.);
#26702=ORIENTED_EDGE('',*,*,#19967,.T.);
#26703=ORIENTED_EDGE('',*,*,#19968,.T.);
#26704=ORIENTED_EDGE('',*,*,#19964,.T.);
#26705=ORIENTED_EDGE('',*,*,#19963,.F.);
#26706=ORIENTED_EDGE('',*,*,#19969,.T.);
#26707=ORIENTED_EDGE('',*,*,#19970,.T.);
#26708=ORIENTED_EDGE('',*,*,#19971,.T.);
#26709=ORIENTED_EDGE('',*,*,#19966,.T.);
#26710=ORIENTED_EDGE('',*,*,#19968,.F.);
#26711=ORIENTED_EDGE('',*,*,#19972,.F.);
#26712=ORIENTED_EDGE('',*,*,#19973,.F.);
#26713=ORIENTED_EDGE('',*,*,#19970,.F.);
#26714=ORIENTED_EDGE('',*,*,#19974,.F.);
#26715=ORIENTED_EDGE('',*,*,#19975,.F.);
#26716=ORIENTED_EDGE('',*,*,#18039,.T.);
#26717=ORIENTED_EDGE('',*,*,#19976,.T.);
#26718=ORIENTED_EDGE('',*,*,#19974,.T.);
#26719=ORIENTED_EDGE('',*,*,#19977,.T.);
#26720=ORIENTED_EDGE('',*,*,#19978,.F.);
#26721=ORIENTED_EDGE('',*,*,#19979,.F.);
#26722=ORIENTED_EDGE('',*,*,#19980,.F.);
#26723=ORIENTED_EDGE('',*,*,#18037,.T.);
#26724=ORIENTED_EDGE('',*,*,#19981,.T.);
#26725=ORIENTED_EDGE('',*,*,#19979,.T.);
#26726=ORIENTED_EDGE('',*,*,#19982,.T.);
#26727=ORIENTED_EDGE('',*,*,#19972,.T.);
#26728=ORIENTED_EDGE('',*,*,#19983,.T.);
#26729=ORIENTED_EDGE('',*,*,#19980,.T.);
#26730=ORIENTED_EDGE('',*,*,#19984,.T.);
#26731=ORIENTED_EDGE('',*,*,#19978,.T.);
#26732=ORIENTED_EDGE('',*,*,#19985,.T.);
#26733=ORIENTED_EDGE('',*,*,#19975,.T.);
#26734=ORIENTED_EDGE('',*,*,#19986,.T.);
#26735=ORIENTED_EDGE('',*,*,#18043,.T.);
#26736=ORIENTED_EDGE('',*,*,#19965,.T.);
#26737=ORIENTED_EDGE('',*,*,#19973,.T.);
#26738=ORIENTED_EDGE('',*,*,#19987,.T.);
#26739=ORIENTED_EDGE('',*,*,#19962,.F.);
#26740=ORIENTED_EDGE('',*,*,#18040,.F.);
#26741=ORIENTED_EDGE('',*,*,#19977,.F.);
#26742=ORIENTED_EDGE('',*,*,#19969,.F.);
#26743=ORIENTED_EDGE('',*,*,#19983,.F.);
#26744=ORIENTED_EDGE('',*,*,#19967,.F.);
#26745=ORIENTED_EDGE('',*,*,#19971,.F.);
#26746=ORIENTED_EDGE('',*,*,#19985,.F.);
#26747=ORIENTED_EDGE('',*,*,#19988,.F.);
#26748=ORIENTED_EDGE('',*,*,#19989,.F.);
#26749=ORIENTED_EDGE('',*,*,#19990,.F.);
#26750=ORIENTED_EDGE('',*,*,#19991,.F.);
#26751=ORIENTED_EDGE('',*,*,#19992,.F.);
#26752=ORIENTED_EDGE('',*,*,#19993,.F.);
#26753=ORIENTED_EDGE('',*,*,#19994,.F.);
#26754=ORIENTED_EDGE('',*,*,#19995,.F.);
#26755=ORIENTED_EDGE('',*,*,#19996,.F.);
#26756=ORIENTED_EDGE('',*,*,#18047,.T.);
#26757=ORIENTED_EDGE('',*,*,#19997,.T.);
#26758=ORIENTED_EDGE('',*,*,#19995,.T.);
#26759=ORIENTED_EDGE('',*,*,#19998,.T.);
#26760=ORIENTED_EDGE('',*,*,#19999,.F.);
#26761=ORIENTED_EDGE('',*,*,#20000,.F.);
#26762=ORIENTED_EDGE('',*,*,#20001,.F.);
#26763=ORIENTED_EDGE('',*,*,#18045,.T.);
#26764=ORIENTED_EDGE('',*,*,#20002,.T.);
#26765=ORIENTED_EDGE('',*,*,#20000,.T.);
#26766=ORIENTED_EDGE('',*,*,#20003,.T.);
#26767=ORIENTED_EDGE('',*,*,#19992,.T.);
#26768=ORIENTED_EDGE('',*,*,#20004,.T.);
#26769=ORIENTED_EDGE('',*,*,#20001,.T.);
#26770=ORIENTED_EDGE('',*,*,#20005,.T.);
#26771=ORIENTED_EDGE('',*,*,#19999,.T.);
#26772=ORIENTED_EDGE('',*,*,#20006,.T.);
#26773=ORIENTED_EDGE('',*,*,#19996,.T.);
#26774=ORIENTED_EDGE('',*,*,#20007,.T.);
#26775=ORIENTED_EDGE('',*,*,#19989,.T.);
#26776=ORIENTED_EDGE('',*,*,#20008,.T.);
#26777=ORIENTED_EDGE('',*,*,#19994,.T.);
#26778=ORIENTED_EDGE('',*,*,#20009,.T.);
#26779=ORIENTED_EDGE('',*,*,#18051,.T.);
#26780=ORIENTED_EDGE('',*,*,#20010,.T.);
#26781=ORIENTED_EDGE('',*,*,#19993,.T.);
#26782=ORIENTED_EDGE('',*,*,#20011,.T.);
#26783=ORIENTED_EDGE('',*,*,#19991,.T.);
#26784=ORIENTED_EDGE('',*,*,#20012,.T.);
#26785=ORIENTED_EDGE('',*,*,#19990,.T.);
#26786=ORIENTED_EDGE('',*,*,#20013,.T.);
#26787=ORIENTED_EDGE('',*,*,#18049,.T.);
#26788=ORIENTED_EDGE('',*,*,#20014,.T.);
#26789=ORIENTED_EDGE('',*,*,#19988,.T.);
#26790=ORIENTED_EDGE('',*,*,#20015,.T.);
#26791=ORIENTED_EDGE('',*,*,#20003,.F.);
#26792=ORIENTED_EDGE('',*,*,#20007,.F.);
#26793=ORIENTED_EDGE('',*,*,#19997,.F.);
#26794=ORIENTED_EDGE('',*,*,#18046,.F.);
#26795=ORIENTED_EDGE('',*,*,#19998,.F.);
#26796=ORIENTED_EDGE('',*,*,#20008,.F.);
#26797=ORIENTED_EDGE('',*,*,#20014,.F.);
#26798=ORIENTED_EDGE('',*,*,#18048,.F.);
#26799=ORIENTED_EDGE('',*,*,#20004,.F.);
#26800=ORIENTED_EDGE('',*,*,#20013,.F.);
#26801=ORIENTED_EDGE('',*,*,#20009,.F.);
#26802=ORIENTED_EDGE('',*,*,#20006,.F.);
#26803=ORIENTED_EDGE('',*,*,#20016,.F.);
#26804=ORIENTED_EDGE('',*,*,#20017,.F.);
#26805=ORIENTED_EDGE('',*,*,#20018,.F.);
#26806=ORIENTED_EDGE('',*,*,#20019,.T.);
#26807=ORIENTED_EDGE('',*,*,#20020,.T.);
#26808=ORIENTED_EDGE('',*,*,#20017,.T.);
#26809=ORIENTED_EDGE('',*,*,#20021,.T.);
#26810=ORIENTED_EDGE('',*,*,#20022,.T.);
#26811=ORIENTED_EDGE('',*,*,#18059,.T.);
#26812=ORIENTED_EDGE('',*,*,#20023,.T.);
#26813=ORIENTED_EDGE('',*,*,#20018,.T.);
#26814=ORIENTED_EDGE('',*,*,#20024,.T.);
#26815=ORIENTED_EDGE('',*,*,#20025,.F.);
#26816=ORIENTED_EDGE('',*,*,#20026,.F.);
#26817=ORIENTED_EDGE('',*,*,#20027,.F.);
#26818=ORIENTED_EDGE('',*,*,#20028,.T.);
#26819=ORIENTED_EDGE('',*,*,#20029,.T.);
#26820=ORIENTED_EDGE('',*,*,#20026,.T.);
#26821=ORIENTED_EDGE('',*,*,#20030,.T.);
#26822=ORIENTED_EDGE('',*,*,#20031,.T.);
#26823=ORIENTED_EDGE('',*,*,#20016,.T.);
#26824=ORIENTED_EDGE('',*,*,#20032,.T.);
#26825=ORIENTED_EDGE('',*,*,#20027,.T.);
#26826=ORIENTED_EDGE('',*,*,#20033,.T.);
#26827=ORIENTED_EDGE('',*,*,#18057,.T.);
#26828=ORIENTED_EDGE('',*,*,#20034,.T.);
#26829=ORIENTED_EDGE('',*,*,#20025,.T.);
#26830=ORIENTED_EDGE('',*,*,#20035,.T.);
#26831=ORIENTED_EDGE('',*,*,#20019,.F.);
#26832=ORIENTED_EDGE('',*,*,#20036,.T.);
#26833=ORIENTED_EDGE('',*,*,#20037,.T.);
#26834=ORIENTED_EDGE('',*,*,#18053,.T.);
#26835=ORIENTED_EDGE('',*,*,#20038,.T.);
#26836=ORIENTED_EDGE('',*,*,#20021,.F.);
#26837=ORIENTED_EDGE('',*,*,#20033,.F.);
#26838=ORIENTED_EDGE('',*,*,#20029,.F.);
#26839=ORIENTED_EDGE('',*,*,#20039,.F.);
#26840=ORIENTED_EDGE('',*,*,#20022,.F.);
#26841=ORIENTED_EDGE('',*,*,#20039,.T.);
#26842=ORIENTED_EDGE('',*,*,#20028,.F.);
#26843=ORIENTED_EDGE('',*,*,#20040,.F.);
#26844=ORIENTED_EDGE('',*,*,#20041,.T.);
#26845=ORIENTED_EDGE('',*,*,#20036,.F.);
#26846=ORIENTED_EDGE('',*,*,#20031,.F.);
#26847=ORIENTED_EDGE('',*,*,#20042,.T.);
#26848=ORIENTED_EDGE('',*,*,#18055,.T.);
#26849=ORIENTED_EDGE('',*,*,#20043,.T.);
#26850=ORIENTED_EDGE('',*,*,#20040,.T.);
#26851=ORIENTED_EDGE('',*,*,#20030,.F.);
#26852=ORIENTED_EDGE('',*,*,#20034,.F.);
#26853=ORIENTED_EDGE('',*,*,#18056,.F.);
#26854=ORIENTED_EDGE('',*,*,#20042,.F.);
#26855=ORIENTED_EDGE('',*,*,#20020,.F.);
#26856=ORIENTED_EDGE('',*,*,#20038,.F.);
#26857=ORIENTED_EDGE('',*,*,#18052,.F.);
#26858=ORIENTED_EDGE('',*,*,#20024,.F.);
#26859=ORIENTED_EDGE('',*,*,#20044,.F.);
#26860=ORIENTED_EDGE('',*,*,#20045,.F.);
#26861=ORIENTED_EDGE('',*,*,#20046,.F.);
#26862=ORIENTED_EDGE('',*,*,#20047,.F.);
#26863=ORIENTED_EDGE('',*,*,#20048,.F.);
#26864=ORIENTED_EDGE('',*,*,#20049,.F.);
#26865=ORIENTED_EDGE('',*,*,#20050,.F.);
#26866=ORIENTED_EDGE('',*,*,#20051,.F.);
#26867=ORIENTED_EDGE('',*,*,#20052,.F.);
#26868=ORIENTED_EDGE('',*,*,#18063,.T.);
#26869=ORIENTED_EDGE('',*,*,#20053,.T.);
#26870=ORIENTED_EDGE('',*,*,#20051,.T.);
#26871=ORIENTED_EDGE('',*,*,#20054,.T.);
#26872=ORIENTED_EDGE('',*,*,#20055,.F.);
#26873=ORIENTED_EDGE('',*,*,#20056,.F.);
#26874=ORIENTED_EDGE('',*,*,#20057,.F.);
#26875=ORIENTED_EDGE('',*,*,#18061,.T.);
#26876=ORIENTED_EDGE('',*,*,#20058,.T.);
#26877=ORIENTED_EDGE('',*,*,#20056,.T.);
#26878=ORIENTED_EDGE('',*,*,#20059,.T.);
#26879=ORIENTED_EDGE('',*,*,#20048,.T.);
#26880=ORIENTED_EDGE('',*,*,#20060,.T.);
#26881=ORIENTED_EDGE('',*,*,#20057,.T.);
#26882=ORIENTED_EDGE('',*,*,#20061,.T.);
#26883=ORIENTED_EDGE('',*,*,#20055,.T.);
#26884=ORIENTED_EDGE('',*,*,#20062,.T.);
#26885=ORIENTED_EDGE('',*,*,#20052,.T.);
#26886=ORIENTED_EDGE('',*,*,#20063,.T.);
#26887=ORIENTED_EDGE('',*,*,#20045,.T.);
#26888=ORIENTED_EDGE('',*,*,#20064,.T.);
#26889=ORIENTED_EDGE('',*,*,#20050,.T.);
#26890=ORIENTED_EDGE('',*,*,#20065,.T.);
#26891=ORIENTED_EDGE('',*,*,#18067,.T.);
#26892=ORIENTED_EDGE('',*,*,#20066,.T.);
#26893=ORIENTED_EDGE('',*,*,#20049,.T.);
#26894=ORIENTED_EDGE('',*,*,#20067,.T.);
#26895=ORIENTED_EDGE('',*,*,#20047,.T.);
#26896=ORIENTED_EDGE('',*,*,#20068,.T.);
#26897=ORIENTED_EDGE('',*,*,#20046,.T.);
#26898=ORIENTED_EDGE('',*,*,#20069,.T.);
#26899=ORIENTED_EDGE('',*,*,#18065,.T.);
#26900=ORIENTED_EDGE('',*,*,#20070,.T.);
#26901=ORIENTED_EDGE('',*,*,#20044,.T.);
#26902=ORIENTED_EDGE('',*,*,#20071,.T.);
#26903=ORIENTED_EDGE('',*,*,#20059,.F.);
#26904=ORIENTED_EDGE('',*,*,#20063,.F.);
#26905=ORIENTED_EDGE('',*,*,#20053,.F.);
#26906=ORIENTED_EDGE('',*,*,#18062,.F.);
#26907=ORIENTED_EDGE('',*,*,#20054,.F.);
#26908=ORIENTED_EDGE('',*,*,#20064,.F.);
#26909=ORIENTED_EDGE('',*,*,#20070,.F.);
#26910=ORIENTED_EDGE('',*,*,#18064,.F.);
#26911=ORIENTED_EDGE('',*,*,#20060,.F.);
#26912=ORIENTED_EDGE('',*,*,#20069,.F.);
#26913=ORIENTED_EDGE('',*,*,#20065,.F.);
#26914=ORIENTED_EDGE('',*,*,#20062,.F.);
#26915=ORIENTED_EDGE('',*,*,#20072,.F.);
#26916=ORIENTED_EDGE('',*,*,#20073,.F.);
#26917=ORIENTED_EDGE('',*,*,#20074,.F.);
#26918=ORIENTED_EDGE('',*,*,#20075,.F.);
#26919=ORIENTED_EDGE('',*,*,#20076,.F.);
#26920=ORIENTED_EDGE('',*,*,#20077,.F.);
#26921=ORIENTED_EDGE('',*,*,#20078,.F.);
#26922=ORIENTED_EDGE('',*,*,#20079,.F.);
#26923=ORIENTED_EDGE('',*,*,#20080,.F.);
#26924=ORIENTED_EDGE('',*,*,#18071,.T.);
#26925=ORIENTED_EDGE('',*,*,#20081,.T.);
#26926=ORIENTED_EDGE('',*,*,#20079,.T.);
#26927=ORIENTED_EDGE('',*,*,#20082,.T.);
#26928=ORIENTED_EDGE('',*,*,#20083,.F.);
#26929=ORIENTED_EDGE('',*,*,#20084,.F.);
#26930=ORIENTED_EDGE('',*,*,#20085,.F.);
#26931=ORIENTED_EDGE('',*,*,#18069,.T.);
#26932=ORIENTED_EDGE('',*,*,#20086,.T.);
#26933=ORIENTED_EDGE('',*,*,#20084,.T.);
#26934=ORIENTED_EDGE('',*,*,#20087,.T.);
#26935=ORIENTED_EDGE('',*,*,#20076,.T.);
#26936=ORIENTED_EDGE('',*,*,#20088,.T.);
#26937=ORIENTED_EDGE('',*,*,#20085,.T.);
#26938=ORIENTED_EDGE('',*,*,#20089,.T.);
#26939=ORIENTED_EDGE('',*,*,#20083,.T.);
#26940=ORIENTED_EDGE('',*,*,#20090,.T.);
#26941=ORIENTED_EDGE('',*,*,#20080,.T.);
#26942=ORIENTED_EDGE('',*,*,#20091,.T.);
#26943=ORIENTED_EDGE('',*,*,#20073,.T.);
#26944=ORIENTED_EDGE('',*,*,#20092,.T.);
#26945=ORIENTED_EDGE('',*,*,#20078,.T.);
#26946=ORIENTED_EDGE('',*,*,#20093,.T.);
#26947=ORIENTED_EDGE('',*,*,#18075,.T.);
#26948=ORIENTED_EDGE('',*,*,#20094,.T.);
#26949=ORIENTED_EDGE('',*,*,#20077,.T.);
#26950=ORIENTED_EDGE('',*,*,#20095,.T.);
#26951=ORIENTED_EDGE('',*,*,#20075,.T.);
#26952=ORIENTED_EDGE('',*,*,#20096,.T.);
#26953=ORIENTED_EDGE('',*,*,#20074,.T.);
#26954=ORIENTED_EDGE('',*,*,#20097,.T.);
#26955=ORIENTED_EDGE('',*,*,#18073,.T.);
#26956=ORIENTED_EDGE('',*,*,#20098,.T.);
#26957=ORIENTED_EDGE('',*,*,#20072,.T.);
#26958=ORIENTED_EDGE('',*,*,#20099,.T.);
#26959=ORIENTED_EDGE('',*,*,#20087,.F.);
#26960=ORIENTED_EDGE('',*,*,#20091,.F.);
#26961=ORIENTED_EDGE('',*,*,#20081,.F.);
#26962=ORIENTED_EDGE('',*,*,#18070,.F.);
#26963=ORIENTED_EDGE('',*,*,#20082,.F.);
#26964=ORIENTED_EDGE('',*,*,#20092,.F.);
#26965=ORIENTED_EDGE('',*,*,#20098,.F.);
#26966=ORIENTED_EDGE('',*,*,#18072,.F.);
#26967=ORIENTED_EDGE('',*,*,#20088,.F.);
#26968=ORIENTED_EDGE('',*,*,#20097,.F.);
#26969=ORIENTED_EDGE('',*,*,#20093,.F.);
#26970=ORIENTED_EDGE('',*,*,#20090,.F.);
#26971=ORIENTED_EDGE('',*,*,#20100,.T.);
#26972=ORIENTED_EDGE('',*,*,#20101,.T.);
#26973=ORIENTED_EDGE('',*,*,#20102,.T.);
#26974=ORIENTED_EDGE('',*,*,#20103,.T.);
#26975=ORIENTED_EDGE('',*,*,#20104,.T.);
#26976=ORIENTED_EDGE('',*,*,#20102,.F.);
#26977=ORIENTED_EDGE('',*,*,#20100,.F.);
#26978=ORIENTED_EDGE('',*,*,#20101,.F.);
#26979=ORIENTED_EDGE('',*,*,#20105,.T.);
#26980=ORIENTED_EDGE('',*,*,#20106,.F.);
#26981=ORIENTED_EDGE('',*,*,#20107,.F.);
#26982=ORIENTED_EDGE('',*,*,#20105,.F.);
#26983=ORIENTED_EDGE('',*,*,#20108,.T.);
#26984=ORIENTED_EDGE('',*,*,#20109,.T.);
#26985=ORIENTED_EDGE('',*,*,#20103,.F.);
#26986=ORIENTED_EDGE('',*,*,#20104,.F.);
#26987=ORIENTED_EDGE('',*,*,#20109,.F.);
#26988=ORIENTED_EDGE('',*,*,#20110,.F.);
#26989=ORIENTED_EDGE('',*,*,#20111,.F.);
#26990=ORIENTED_EDGE('',*,*,#20112,.F.);
#26991=ORIENTED_EDGE('',*,*,#20113,.F.);
#26992=ORIENTED_EDGE('',*,*,#20114,.F.);
#26993=ORIENTED_EDGE('',*,*,#20115,.F.);
#26994=ORIENTED_EDGE('',*,*,#20116,.F.);
#26995=ORIENTED_EDGE('',*,*,#20117,.F.);
#26996=ORIENTED_EDGE('',*,*,#20118,.F.);
#26997=ORIENTED_EDGE('',*,*,#18079,.T.);
#26998=ORIENTED_EDGE('',*,*,#20119,.T.);
#26999=ORIENTED_EDGE('',*,*,#20117,.T.);
#27000=ORIENTED_EDGE('',*,*,#20120,.T.);
#27001=ORIENTED_EDGE('',*,*,#20121,.F.);
#27002=ORIENTED_EDGE('',*,*,#20122,.F.);
#27003=ORIENTED_EDGE('',*,*,#20123,.F.);
#27004=ORIENTED_EDGE('',*,*,#18077,.T.);
#27005=ORIENTED_EDGE('',*,*,#20124,.T.);
#27006=ORIENTED_EDGE('',*,*,#20122,.T.);
#27007=ORIENTED_EDGE('',*,*,#20125,.T.);
#27008=ORIENTED_EDGE('',*,*,#20114,.T.);
#27009=ORIENTED_EDGE('',*,*,#20126,.T.);
#27010=ORIENTED_EDGE('',*,*,#20123,.T.);
#27011=ORIENTED_EDGE('',*,*,#20127,.T.);
#27012=ORIENTED_EDGE('',*,*,#20121,.T.);
#27013=ORIENTED_EDGE('',*,*,#20128,.T.);
#27014=ORIENTED_EDGE('',*,*,#20118,.T.);
#27015=ORIENTED_EDGE('',*,*,#20129,.T.);
#27016=ORIENTED_EDGE('',*,*,#20111,.T.);
#27017=ORIENTED_EDGE('',*,*,#20130,.T.);
#27018=ORIENTED_EDGE('',*,*,#20116,.T.);
#27019=ORIENTED_EDGE('',*,*,#20131,.T.);
#27020=ORIENTED_EDGE('',*,*,#18083,.T.);
#27021=ORIENTED_EDGE('',*,*,#20132,.T.);
#27022=ORIENTED_EDGE('',*,*,#20115,.T.);
#27023=ORIENTED_EDGE('',*,*,#20133,.T.);
#27024=ORIENTED_EDGE('',*,*,#20113,.T.);
#27025=ORIENTED_EDGE('',*,*,#20134,.T.);
#27026=ORIENTED_EDGE('',*,*,#20112,.T.);
#27027=ORIENTED_EDGE('',*,*,#20135,.T.);
#27028=ORIENTED_EDGE('',*,*,#18081,.T.);
#27029=ORIENTED_EDGE('',*,*,#20136,.T.);
#27030=ORIENTED_EDGE('',*,*,#20110,.T.);
#27031=ORIENTED_EDGE('',*,*,#20137,.T.);
#27032=ORIENTED_EDGE('',*,*,#20125,.F.);
#27033=ORIENTED_EDGE('',*,*,#20129,.F.);
#27034=ORIENTED_EDGE('',*,*,#20119,.F.);
#27035=ORIENTED_EDGE('',*,*,#18078,.F.);
#27036=ORIENTED_EDGE('',*,*,#20120,.F.);
#27037=ORIENTED_EDGE('',*,*,#20130,.F.);
#27038=ORIENTED_EDGE('',*,*,#20136,.F.);
#27039=ORIENTED_EDGE('',*,*,#18080,.F.);
#27040=ORIENTED_EDGE('',*,*,#20126,.F.);
#27041=ORIENTED_EDGE('',*,*,#20135,.F.);
#27042=ORIENTED_EDGE('',*,*,#20131,.F.);
#27043=ORIENTED_EDGE('',*,*,#20128,.F.);
#27044=ORIENTED_EDGE('',*,*,#20138,.F.);
#27045=ORIENTED_EDGE('',*,*,#20139,.F.);
#27046=ORIENTED_EDGE('',*,*,#20140,.F.);
#27047=ORIENTED_EDGE('',*,*,#20141,.F.);
#27048=ORIENTED_EDGE('',*,*,#20142,.F.);
#27049=ORIENTED_EDGE('',*,*,#20143,.F.);
#27050=ORIENTED_EDGE('',*,*,#20144,.F.);
#27051=ORIENTED_EDGE('',*,*,#20145,.F.);
#27052=ORIENTED_EDGE('',*,*,#20146,.F.);
#27053=ORIENTED_EDGE('',*,*,#18087,.T.);
#27054=ORIENTED_EDGE('',*,*,#20147,.T.);
#27055=ORIENTED_EDGE('',*,*,#20145,.T.);
#27056=ORIENTED_EDGE('',*,*,#20148,.T.);
#27057=ORIENTED_EDGE('',*,*,#20149,.F.);
#27058=ORIENTED_EDGE('',*,*,#20150,.F.);
#27059=ORIENTED_EDGE('',*,*,#20151,.F.);
#27060=ORIENTED_EDGE('',*,*,#18085,.T.);
#27061=ORIENTED_EDGE('',*,*,#20152,.T.);
#27062=ORIENTED_EDGE('',*,*,#20150,.T.);
#27063=ORIENTED_EDGE('',*,*,#20153,.T.);
#27064=ORIENTED_EDGE('',*,*,#20142,.T.);
#27065=ORIENTED_EDGE('',*,*,#20154,.T.);
#27066=ORIENTED_EDGE('',*,*,#20151,.T.);
#27067=ORIENTED_EDGE('',*,*,#20155,.T.);
#27068=ORIENTED_EDGE('',*,*,#20149,.T.);
#27069=ORIENTED_EDGE('',*,*,#20156,.T.);
#27070=ORIENTED_EDGE('',*,*,#20146,.T.);
#27071=ORIENTED_EDGE('',*,*,#20157,.T.);
#27072=ORIENTED_EDGE('',*,*,#20139,.T.);
#27073=ORIENTED_EDGE('',*,*,#20158,.T.);
#27074=ORIENTED_EDGE('',*,*,#20144,.T.);
#27075=ORIENTED_EDGE('',*,*,#20159,.T.);
#27076=ORIENTED_EDGE('',*,*,#18091,.T.);
#27077=ORIENTED_EDGE('',*,*,#20160,.T.);
#27078=ORIENTED_EDGE('',*,*,#20143,.T.);
#27079=ORIENTED_EDGE('',*,*,#20161,.T.);
#27080=ORIENTED_EDGE('',*,*,#20141,.T.);
#27081=ORIENTED_EDGE('',*,*,#20162,.T.);
#27082=ORIENTED_EDGE('',*,*,#20140,.T.);
#27083=ORIENTED_EDGE('',*,*,#20163,.T.);
#27084=ORIENTED_EDGE('',*,*,#18089,.T.);
#27085=ORIENTED_EDGE('',*,*,#20164,.T.);
#27086=ORIENTED_EDGE('',*,*,#20138,.T.);
#27087=ORIENTED_EDGE('',*,*,#20165,.T.);
#27088=ORIENTED_EDGE('',*,*,#20153,.F.);
#27089=ORIENTED_EDGE('',*,*,#20157,.F.);
#27090=ORIENTED_EDGE('',*,*,#20147,.F.);
#27091=ORIENTED_EDGE('',*,*,#18086,.F.);
#27092=ORIENTED_EDGE('',*,*,#20148,.F.);
#27093=ORIENTED_EDGE('',*,*,#20158,.F.);
#27094=ORIENTED_EDGE('',*,*,#20164,.F.);
#27095=ORIENTED_EDGE('',*,*,#18088,.F.);
#27096=ORIENTED_EDGE('',*,*,#20154,.F.);
#27097=ORIENTED_EDGE('',*,*,#20163,.F.);
#27098=ORIENTED_EDGE('',*,*,#20159,.F.);
#27099=ORIENTED_EDGE('',*,*,#20156,.F.);
#27100=ORIENTED_EDGE('',*,*,#20166,.T.);
#27101=ORIENTED_EDGE('',*,*,#20167,.T.);
#27102=ORIENTED_EDGE('',*,*,#20168,.T.);
#27103=ORIENTED_EDGE('',*,*,#20169,.T.);
#27104=ORIENTED_EDGE('',*,*,#20170,.T.);
#27105=ORIENTED_EDGE('',*,*,#20168,.F.);
#27106=ORIENTED_EDGE('',*,*,#20169,.F.);
#27107=ORIENTED_EDGE('',*,*,#20170,.F.);
#27108=ORIENTED_EDGE('',*,*,#20171,.T.);
#27109=ORIENTED_EDGE('',*,*,#20172,.F.);
#27110=ORIENTED_EDGE('',*,*,#20173,.F.);
#27111=ORIENTED_EDGE('',*,*,#20171,.F.);
#27112=ORIENTED_EDGE('',*,*,#17518,.F.);
#27113=ORIENTED_EDGE('',*,*,#20174,.T.);
#27114=ORIENTED_EDGE('',*,*,#20166,.F.);
#27115=ORIENTED_EDGE('',*,*,#20167,.F.);
#27116=ORIENTED_EDGE('',*,*,#20174,.F.);
#27117=ORIENTED_EDGE('',*,*,#20175,.T.);
#27118=ORIENTED_EDGE('',*,*,#20176,.T.);
#27119=ORIENTED_EDGE('',*,*,#20106,.T.);
#27120=ORIENTED_EDGE('',*,*,#20107,.T.);
#27121=ORIENTED_EDGE('',*,*,#20176,.F.);
#27122=ORIENTED_EDGE('',*,*,#20177,.F.);
#27123=ORIENTED_EDGE('',*,*,#20175,.F.);
#27124=ORIENTED_EDGE('',*,*,#20178,.T.);
#27125=ORIENTED_EDGE('',*,*,#20179,.T.);
#27126=ORIENTED_EDGE('',*,*,#20172,.T.);
#27127=ORIENTED_EDGE('',*,*,#20173,.T.);
#27128=ORIENTED_EDGE('',*,*,#20179,.F.);
#27129=ORIENTED_EDGE('',*,*,#20178,.F.);
#27130=ORIENTED_EDGE('',*,*,#20180,.T.);
#27131=ORIENTED_EDGE('',*,*,#20181,.F.);
#27132=ORIENTED_EDGE('',*,*,#20180,.F.);
#27133=ORIENTED_EDGE('',*,*,#20181,.T.);
#27134=ORIENTED_EDGE('',*,*,#20182,.T.);
#27135=ORIENTED_EDGE('',*,*,#20177,.T.);
#27136=ORIENTED_EDGE('',*,*,#20182,.F.);
#27137=ORIENTED_EDGE('',*,*,#20152,.F.);
#27138=ORIENTED_EDGE('',*,*,#18084,.F.);
#27139=ORIENTED_EDGE('',*,*,#20161,.F.);
#27140=ORIENTED_EDGE('',*,*,#20155,.F.);
#27141=ORIENTED_EDGE('',*,*,#20160,.F.);
#27142=ORIENTED_EDGE('',*,*,#18090,.F.);
#27143=ORIENTED_EDGE('',*,*,#20165,.F.);
#27144=ORIENTED_EDGE('',*,*,#20162,.F.);
#27145=ORIENTED_EDGE('',*,*,#20124,.F.);
#27146=ORIENTED_EDGE('',*,*,#18076,.F.);
#27147=ORIENTED_EDGE('',*,*,#20133,.F.);
#27148=ORIENTED_EDGE('',*,*,#20127,.F.);
#27149=ORIENTED_EDGE('',*,*,#20132,.F.);
#27150=ORIENTED_EDGE('',*,*,#18082,.F.);
#27151=ORIENTED_EDGE('',*,*,#20137,.F.);
#27152=ORIENTED_EDGE('',*,*,#20134,.F.);
#27153=ORIENTED_EDGE('',*,*,#20086,.F.);
#27154=ORIENTED_EDGE('',*,*,#18068,.F.);
#27155=ORIENTED_EDGE('',*,*,#20095,.F.);
#27156=ORIENTED_EDGE('',*,*,#20089,.F.);
#27157=ORIENTED_EDGE('',*,*,#20094,.F.);
#27158=ORIENTED_EDGE('',*,*,#18074,.F.);
#27159=ORIENTED_EDGE('',*,*,#20099,.F.);
#27160=ORIENTED_EDGE('',*,*,#20096,.F.);
#27161=ORIENTED_EDGE('',*,*,#20058,.F.);
#27162=ORIENTED_EDGE('',*,*,#18060,.F.);
#27163=ORIENTED_EDGE('',*,*,#20067,.F.);
#27164=ORIENTED_EDGE('',*,*,#20061,.F.);
#27165=ORIENTED_EDGE('',*,*,#20066,.F.);
#27166=ORIENTED_EDGE('',*,*,#18066,.F.);
#27167=ORIENTED_EDGE('',*,*,#20071,.F.);
#27168=ORIENTED_EDGE('',*,*,#20068,.F.);
#27169=ORIENTED_EDGE('',*,*,#20043,.F.);
#27170=ORIENTED_EDGE('',*,*,#18054,.F.);
#27171=ORIENTED_EDGE('',*,*,#20037,.F.);
#27172=ORIENTED_EDGE('',*,*,#20041,.F.);
#27173=ORIENTED_EDGE('',*,*,#20023,.F.);
#27174=ORIENTED_EDGE('',*,*,#18058,.F.);
#27175=ORIENTED_EDGE('',*,*,#20035,.F.);
#27176=ORIENTED_EDGE('',*,*,#20032,.F.);
#27177=ORIENTED_EDGE('',*,*,#20002,.F.);
#27178=ORIENTED_EDGE('',*,*,#18044,.F.);
#27179=ORIENTED_EDGE('',*,*,#20011,.F.);
#27180=ORIENTED_EDGE('',*,*,#20005,.F.);
#27181=ORIENTED_EDGE('',*,*,#20010,.F.);
#27182=ORIENTED_EDGE('',*,*,#18050,.F.);
#27183=ORIENTED_EDGE('',*,*,#20015,.F.);
#27184=ORIENTED_EDGE('',*,*,#20012,.F.);
#27185=ORIENTED_EDGE('',*,*,#19976,.F.);
#27186=ORIENTED_EDGE('',*,*,#18038,.F.);
#27187=ORIENTED_EDGE('',*,*,#19982,.F.);
#27188=ORIENTED_EDGE('',*,*,#19986,.F.);
#27189=ORIENTED_EDGE('',*,*,#19981,.F.);
#27190=ORIENTED_EDGE('',*,*,#18036,.F.);
#27191=ORIENTED_EDGE('',*,*,#19987,.F.);
#27192=ORIENTED_EDGE('',*,*,#19984,.F.);
#27193=ORIENTED_EDGE('',*,*,#19946,.F.);
#27194=ORIENTED_EDGE('',*,*,#18028,.F.);
#27195=ORIENTED_EDGE('',*,*,#19955,.F.);
#27196=ORIENTED_EDGE('',*,*,#19949,.F.);
#27197=ORIENTED_EDGE('',*,*,#19954,.F.);
#27198=ORIENTED_EDGE('',*,*,#18034,.F.);
#27199=ORIENTED_EDGE('',*,*,#19959,.F.);
#27200=ORIENTED_EDGE('',*,*,#19956,.F.);
#27201=ORIENTED_EDGE('',*,*,#19918,.F.);
#27202=ORIENTED_EDGE('',*,*,#18020,.F.);
#27203=ORIENTED_EDGE('',*,*,#19927,.F.);
#27204=ORIENTED_EDGE('',*,*,#19921,.F.);
#27205=ORIENTED_EDGE('',*,*,#19926,.F.);
#27206=ORIENTED_EDGE('',*,*,#18026,.F.);
#27207=ORIENTED_EDGE('',*,*,#19931,.F.);
#27208=ORIENTED_EDGE('',*,*,#19928,.F.);
#27209=ORIENTED_EDGE('',*,*,#19903,.F.);
#27210=ORIENTED_EDGE('',*,*,#18014,.F.);
#27211=ORIENTED_EDGE('',*,*,#19897,.F.);
#27212=ORIENTED_EDGE('',*,*,#19901,.F.);
#27213=ORIENTED_EDGE('',*,*,#19883,.F.);
#27214=ORIENTED_EDGE('',*,*,#18018,.F.);
#27215=ORIENTED_EDGE('',*,*,#19895,.F.);
#27216=ORIENTED_EDGE('',*,*,#19892,.F.);
#27217=ORIENTED_EDGE('',*,*,#19862,.F.);
#27218=ORIENTED_EDGE('',*,*,#18004,.F.);
#27219=ORIENTED_EDGE('',*,*,#19871,.F.);
#27220=ORIENTED_EDGE('',*,*,#19865,.F.);
#27221=ORIENTED_EDGE('',*,*,#19870,.F.);
#27222=ORIENTED_EDGE('',*,*,#18010,.F.);
#27223=ORIENTED_EDGE('',*,*,#19875,.F.);
#27224=ORIENTED_EDGE('',*,*,#19872,.F.);
#27225=ORIENTED_EDGE('',*,*,#19836,.F.);
#27226=ORIENTED_EDGE('',*,*,#17998,.F.);
#27227=ORIENTED_EDGE('',*,*,#19842,.F.);
#27228=ORIENTED_EDGE('',*,*,#19846,.F.);
#27229=ORIENTED_EDGE('',*,*,#19841,.F.);
#27230=ORIENTED_EDGE('',*,*,#17996,.F.);
#27231=ORIENTED_EDGE('',*,*,#19847,.F.);
#27232=ORIENTED_EDGE('',*,*,#19844,.F.);
#27233=ORIENTED_EDGE('',*,*,#19806,.F.);
#27234=ORIENTED_EDGE('',*,*,#17988,.F.);
#27235=ORIENTED_EDGE('',*,*,#19815,.F.);
#27236=ORIENTED_EDGE('',*,*,#19809,.F.);
#27237=ORIENTED_EDGE('',*,*,#19814,.F.);
#27238=ORIENTED_EDGE('',*,*,#17994,.F.);
#27239=ORIENTED_EDGE('',*,*,#19819,.F.);
#27240=ORIENTED_EDGE('',*,*,#19816,.F.);
#27241=ORIENTED_EDGE('',*,*,#19778,.F.);
#27242=ORIENTED_EDGE('',*,*,#17980,.F.);
#27243=ORIENTED_EDGE('',*,*,#19787,.F.);
#27244=ORIENTED_EDGE('',*,*,#19781,.F.);
#27245=ORIENTED_EDGE('',*,*,#19786,.F.);
#27246=ORIENTED_EDGE('',*,*,#17986,.F.);
#27247=ORIENTED_EDGE('',*,*,#19791,.F.);
#27248=ORIENTED_EDGE('',*,*,#19788,.F.);
#27249=ORIENTED_EDGE('',*,*,#19763,.F.);
#27250=ORIENTED_EDGE('',*,*,#17974,.F.);
#27251=ORIENTED_EDGE('',*,*,#19757,.F.);
#27252=ORIENTED_EDGE('',*,*,#19761,.F.);
#27253=ORIENTED_EDGE('',*,*,#19743,.F.);
#27254=ORIENTED_EDGE('',*,*,#17978,.F.);
#27255=ORIENTED_EDGE('',*,*,#19755,.F.);
#27256=ORIENTED_EDGE('',*,*,#19752,.F.);
#27257=ORIENTED_EDGE('',*,*,#19722,.F.);
#27258=ORIENTED_EDGE('',*,*,#17964,.F.);
#27259=ORIENTED_EDGE('',*,*,#19731,.F.);
#27260=ORIENTED_EDGE('',*,*,#19725,.F.);
#27261=ORIENTED_EDGE('',*,*,#19730,.F.);
#27262=ORIENTED_EDGE('',*,*,#17970,.F.);
#27263=ORIENTED_EDGE('',*,*,#19735,.F.);
#27264=ORIENTED_EDGE('',*,*,#19732,.F.);
#27265=ORIENTED_EDGE('',*,*,#19696,.F.);
#27266=ORIENTED_EDGE('',*,*,#17958,.F.);
#27267=ORIENTED_EDGE('',*,*,#19702,.F.);
#27268=ORIENTED_EDGE('',*,*,#19706,.F.);
#27269=ORIENTED_EDGE('',*,*,#19701,.F.);
#27270=ORIENTED_EDGE('',*,*,#17956,.F.);
#27271=ORIENTED_EDGE('',*,*,#19707,.F.);
#27272=ORIENTED_EDGE('',*,*,#19704,.F.);
#27273=ORIENTED_EDGE('',*,*,#19666,.F.);
#27274=ORIENTED_EDGE('',*,*,#17948,.F.);
#27275=ORIENTED_EDGE('',*,*,#19675,.F.);
#27276=ORIENTED_EDGE('',*,*,#19669,.F.);
#27277=ORIENTED_EDGE('',*,*,#19674,.F.);
#27278=ORIENTED_EDGE('',*,*,#17954,.F.);
#27279=ORIENTED_EDGE('',*,*,#19679,.F.);
#27280=ORIENTED_EDGE('',*,*,#19676,.F.);
#27281=ORIENTED_EDGE('',*,*,#19638,.F.);
#27282=ORIENTED_EDGE('',*,*,#17940,.F.);
#27283=ORIENTED_EDGE('',*,*,#19647,.F.);
#27284=ORIENTED_EDGE('',*,*,#19641,.F.);
#27285=ORIENTED_EDGE('',*,*,#19646,.F.);
#27286=ORIENTED_EDGE('',*,*,#17946,.F.);
#27287=ORIENTED_EDGE('',*,*,#19651,.F.);
#27288=ORIENTED_EDGE('',*,*,#19648,.F.);
#27289=ORIENTED_EDGE('',*,*,#19623,.F.);
#27290=ORIENTED_EDGE('',*,*,#17934,.F.);
#27291=ORIENTED_EDGE('',*,*,#19617,.F.);
#27292=ORIENTED_EDGE('',*,*,#19621,.F.);
#27293=ORIENTED_EDGE('',*,*,#19603,.F.);
#27294=ORIENTED_EDGE('',*,*,#17938,.F.);
#27295=ORIENTED_EDGE('',*,*,#19615,.F.);
#27296=ORIENTED_EDGE('',*,*,#19612,.F.);
#27297=ORIENTED_EDGE('',*,*,#19582,.F.);
#27298=ORIENTED_EDGE('',*,*,#17924,.F.);
#27299=ORIENTED_EDGE('',*,*,#19591,.F.);
#27300=ORIENTED_EDGE('',*,*,#19585,.F.);
#27301=ORIENTED_EDGE('',*,*,#19590,.F.);
#27302=ORIENTED_EDGE('',*,*,#17930,.F.);
#27303=ORIENTED_EDGE('',*,*,#19595,.F.);
#27304=ORIENTED_EDGE('',*,*,#19592,.F.);
#27305=ORIENTED_EDGE('',*,*,#19556,.F.);
#27306=ORIENTED_EDGE('',*,*,#17918,.F.);
#27307=ORIENTED_EDGE('',*,*,#19562,.F.);
#27308=ORIENTED_EDGE('',*,*,#19566,.F.);
#27309=ORIENTED_EDGE('',*,*,#19561,.F.);
#27310=ORIENTED_EDGE('',*,*,#17916,.F.);
#27311=ORIENTED_EDGE('',*,*,#19567,.F.);
#27312=ORIENTED_EDGE('',*,*,#19564,.F.);
#27313=ORIENTED_EDGE('',*,*,#19526,.F.);
#27314=ORIENTED_EDGE('',*,*,#17908,.F.);
#27315=ORIENTED_EDGE('',*,*,#19535,.F.);
#27316=ORIENTED_EDGE('',*,*,#19529,.F.);
#27317=ORIENTED_EDGE('',*,*,#19534,.F.);
#27318=ORIENTED_EDGE('',*,*,#17914,.F.);
#27319=ORIENTED_EDGE('',*,*,#19539,.F.);
#27320=ORIENTED_EDGE('',*,*,#19536,.F.);
#27321=ORIENTED_EDGE('',*,*,#19498,.F.);
#27322=ORIENTED_EDGE('',*,*,#17900,.F.);
#27323=ORIENTED_EDGE('',*,*,#19507,.F.);
#27324=ORIENTED_EDGE('',*,*,#19501,.F.);
#27325=ORIENTED_EDGE('',*,*,#19506,.F.);
#27326=ORIENTED_EDGE('',*,*,#17906,.F.);
#27327=ORIENTED_EDGE('',*,*,#19511,.F.);
#27328=ORIENTED_EDGE('',*,*,#19508,.F.);
#27329=ORIENTED_EDGE('',*,*,#19483,.F.);
#27330=ORIENTED_EDGE('',*,*,#17894,.F.);
#27331=ORIENTED_EDGE('',*,*,#19477,.F.);
#27332=ORIENTED_EDGE('',*,*,#19481,.F.);
#27333=ORIENTED_EDGE('',*,*,#19463,.F.);
#27334=ORIENTED_EDGE('',*,*,#17898,.F.);
#27335=ORIENTED_EDGE('',*,*,#19475,.F.);
#27336=ORIENTED_EDGE('',*,*,#19472,.F.);
#27337=ORIENTED_EDGE('',*,*,#19442,.F.);
#27338=ORIENTED_EDGE('',*,*,#17884,.F.);
#27339=ORIENTED_EDGE('',*,*,#19451,.F.);
#27340=ORIENTED_EDGE('',*,*,#19445,.F.);
#27341=ORIENTED_EDGE('',*,*,#19450,.F.);
#27342=ORIENTED_EDGE('',*,*,#17890,.F.);
#27343=ORIENTED_EDGE('',*,*,#19455,.F.);
#27344=ORIENTED_EDGE('',*,*,#19452,.F.);
#27345=ORIENTED_EDGE('',*,*,#19416,.F.);
#27346=ORIENTED_EDGE('',*,*,#17878,.F.);
#27347=ORIENTED_EDGE('',*,*,#19422,.F.);
#27348=ORIENTED_EDGE('',*,*,#19426,.F.);
#27349=ORIENTED_EDGE('',*,*,#19421,.F.);
#27350=ORIENTED_EDGE('',*,*,#17876,.F.);
#27351=ORIENTED_EDGE('',*,*,#19427,.F.);
#27352=ORIENTED_EDGE('',*,*,#19424,.F.);
#27353=ORIENTED_EDGE('',*,*,#19386,.F.);
#27354=ORIENTED_EDGE('',*,*,#17868,.F.);
#27355=ORIENTED_EDGE('',*,*,#19395,.F.);
#27356=ORIENTED_EDGE('',*,*,#19389,.F.);
#27357=ORIENTED_EDGE('',*,*,#19394,.F.);
#27358=ORIENTED_EDGE('',*,*,#17874,.F.);
#27359=ORIENTED_EDGE('',*,*,#19399,.F.);
#27360=ORIENTED_EDGE('',*,*,#19396,.F.);
#27361=ORIENTED_EDGE('',*,*,#19358,.F.);
#27362=ORIENTED_EDGE('',*,*,#17860,.F.);
#27363=ORIENTED_EDGE('',*,*,#19367,.F.);
#27364=ORIENTED_EDGE('',*,*,#19361,.F.);
#27365=ORIENTED_EDGE('',*,*,#19366,.F.);
#27366=ORIENTED_EDGE('',*,*,#17866,.F.);
#27367=ORIENTED_EDGE('',*,*,#19371,.F.);
#27368=ORIENTED_EDGE('',*,*,#19368,.F.);
#27369=ORIENTED_EDGE('',*,*,#19343,.F.);
#27370=ORIENTED_EDGE('',*,*,#17854,.F.);
#27371=ORIENTED_EDGE('',*,*,#19337,.F.);
#27372=ORIENTED_EDGE('',*,*,#19341,.F.);
#27373=ORIENTED_EDGE('',*,*,#19323,.F.);
#27374=ORIENTED_EDGE('',*,*,#17858,.F.);
#27375=ORIENTED_EDGE('',*,*,#19335,.F.);
#27376=ORIENTED_EDGE('',*,*,#19332,.F.);
#27377=ORIENTED_EDGE('',*,*,#19302,.F.);
#27378=ORIENTED_EDGE('',*,*,#17844,.F.);
#27379=ORIENTED_EDGE('',*,*,#19311,.F.);
#27380=ORIENTED_EDGE('',*,*,#19305,.F.);
#27381=ORIENTED_EDGE('',*,*,#19310,.F.);
#27382=ORIENTED_EDGE('',*,*,#17850,.F.);
#27383=ORIENTED_EDGE('',*,*,#19315,.F.);
#27384=ORIENTED_EDGE('',*,*,#19312,.F.);
#27385=ORIENTED_EDGE('',*,*,#19276,.F.);
#27386=ORIENTED_EDGE('',*,*,#17838,.F.);
#27387=ORIENTED_EDGE('',*,*,#19282,.F.);
#27388=ORIENTED_EDGE('',*,*,#19286,.F.);
#27389=ORIENTED_EDGE('',*,*,#19281,.F.);
#27390=ORIENTED_EDGE('',*,*,#17836,.F.);
#27391=ORIENTED_EDGE('',*,*,#19287,.F.);
#27392=ORIENTED_EDGE('',*,*,#19284,.F.);
#27393=ORIENTED_EDGE('',*,*,#19246,.F.);
#27394=ORIENTED_EDGE('',*,*,#17828,.F.);
#27395=ORIENTED_EDGE('',*,*,#19255,.F.);
#27396=ORIENTED_EDGE('',*,*,#19249,.F.);
#27397=ORIENTED_EDGE('',*,*,#19254,.F.);
#27398=ORIENTED_EDGE('',*,*,#17834,.F.);
#27399=ORIENTED_EDGE('',*,*,#19259,.F.);
#27400=ORIENTED_EDGE('',*,*,#19256,.F.);
#27401=ORIENTED_EDGE('',*,*,#19218,.F.);
#27402=ORIENTED_EDGE('',*,*,#17820,.F.);
#27403=ORIENTED_EDGE('',*,*,#19227,.F.);
#27404=ORIENTED_EDGE('',*,*,#19221,.F.);
#27405=ORIENTED_EDGE('',*,*,#19226,.F.);
#27406=ORIENTED_EDGE('',*,*,#17826,.F.);
#27407=ORIENTED_EDGE('',*,*,#19231,.F.);
#27408=ORIENTED_EDGE('',*,*,#19228,.F.);
#27409=ORIENTED_EDGE('',*,*,#19203,.F.);
#27410=ORIENTED_EDGE('',*,*,#17814,.F.);
#27411=ORIENTED_EDGE('',*,*,#19197,.F.);
#27412=ORIENTED_EDGE('',*,*,#19201,.F.);
#27413=ORIENTED_EDGE('',*,*,#19183,.F.);
#27414=ORIENTED_EDGE('',*,*,#17818,.F.);
#27415=ORIENTED_EDGE('',*,*,#19195,.F.);
#27416=ORIENTED_EDGE('',*,*,#19192,.F.);
#27417=ORIENTED_EDGE('',*,*,#19162,.F.);
#27418=ORIENTED_EDGE('',*,*,#17804,.F.);
#27419=ORIENTED_EDGE('',*,*,#19171,.F.);
#27420=ORIENTED_EDGE('',*,*,#19165,.F.);
#27421=ORIENTED_EDGE('',*,*,#19170,.F.);
#27422=ORIENTED_EDGE('',*,*,#17810,.F.);
#27423=ORIENTED_EDGE('',*,*,#19175,.F.);
#27424=ORIENTED_EDGE('',*,*,#19172,.F.);
#27425=ORIENTED_EDGE('',*,*,#19136,.F.);
#27426=ORIENTED_EDGE('',*,*,#17798,.F.);
#27427=ORIENTED_EDGE('',*,*,#19142,.F.);
#27428=ORIENTED_EDGE('',*,*,#19146,.F.);
#27429=ORIENTED_EDGE('',*,*,#19141,.F.);
#27430=ORIENTED_EDGE('',*,*,#17796,.F.);
#27431=ORIENTED_EDGE('',*,*,#19147,.F.);
#27432=ORIENTED_EDGE('',*,*,#19144,.F.);
#27433=ORIENTED_EDGE('',*,*,#19106,.F.);
#27434=ORIENTED_EDGE('',*,*,#17788,.F.);
#27435=ORIENTED_EDGE('',*,*,#19115,.F.);
#27436=ORIENTED_EDGE('',*,*,#19109,.F.);
#27437=ORIENTED_EDGE('',*,*,#19114,.F.);
#27438=ORIENTED_EDGE('',*,*,#17794,.F.);
#27439=ORIENTED_EDGE('',*,*,#19119,.F.);
#27440=ORIENTED_EDGE('',*,*,#19116,.F.);
#27441=ORIENTED_EDGE('',*,*,#19078,.F.);
#27442=ORIENTED_EDGE('',*,*,#17780,.F.);
#27443=ORIENTED_EDGE('',*,*,#19087,.F.);
#27444=ORIENTED_EDGE('',*,*,#19081,.F.);
#27445=ORIENTED_EDGE('',*,*,#19086,.F.);
#27446=ORIENTED_EDGE('',*,*,#17786,.F.);
#27447=ORIENTED_EDGE('',*,*,#19091,.F.);
#27448=ORIENTED_EDGE('',*,*,#19088,.F.);
#27449=ORIENTED_EDGE('',*,*,#19063,.F.);
#27450=ORIENTED_EDGE('',*,*,#17774,.F.);
#27451=ORIENTED_EDGE('',*,*,#19057,.F.);
#27452=ORIENTED_EDGE('',*,*,#19061,.F.);
#27453=ORIENTED_EDGE('',*,*,#19043,.F.);
#27454=ORIENTED_EDGE('',*,*,#17778,.F.);
#27455=ORIENTED_EDGE('',*,*,#19055,.F.);
#27456=ORIENTED_EDGE('',*,*,#19052,.F.);
#27457=ORIENTED_EDGE('',*,*,#19022,.F.);
#27458=ORIENTED_EDGE('',*,*,#17764,.F.);
#27459=ORIENTED_EDGE('',*,*,#19031,.F.);
#27460=ORIENTED_EDGE('',*,*,#19025,.F.);
#27461=ORIENTED_EDGE('',*,*,#19030,.F.);
#27462=ORIENTED_EDGE('',*,*,#17770,.F.);
#27463=ORIENTED_EDGE('',*,*,#19035,.F.);
#27464=ORIENTED_EDGE('',*,*,#19032,.F.);
#27465=ORIENTED_EDGE('',*,*,#18996,.F.);
#27466=ORIENTED_EDGE('',*,*,#17758,.F.);
#27467=ORIENTED_EDGE('',*,*,#19002,.F.);
#27468=ORIENTED_EDGE('',*,*,#19006,.F.);
#27469=ORIENTED_EDGE('',*,*,#19001,.F.);
#27470=ORIENTED_EDGE('',*,*,#17756,.F.);
#27471=ORIENTED_EDGE('',*,*,#19007,.F.);
#27472=ORIENTED_EDGE('',*,*,#19004,.F.);
#27473=ORIENTED_EDGE('',*,*,#18966,.F.);
#27474=ORIENTED_EDGE('',*,*,#17748,.F.);
#27475=ORIENTED_EDGE('',*,*,#18975,.F.);
#27476=ORIENTED_EDGE('',*,*,#18969,.F.);
#27477=ORIENTED_EDGE('',*,*,#18974,.F.);
#27478=ORIENTED_EDGE('',*,*,#17754,.F.);
#27479=ORIENTED_EDGE('',*,*,#18979,.F.);
#27480=ORIENTED_EDGE('',*,*,#18976,.F.);
#27481=ORIENTED_EDGE('',*,*,#18938,.F.);
#27482=ORIENTED_EDGE('',*,*,#17740,.F.);
#27483=ORIENTED_EDGE('',*,*,#18947,.F.);
#27484=ORIENTED_EDGE('',*,*,#18941,.F.);
#27485=ORIENTED_EDGE('',*,*,#18946,.F.);
#27486=ORIENTED_EDGE('',*,*,#17746,.F.);
#27487=ORIENTED_EDGE('',*,*,#18951,.F.);
#27488=ORIENTED_EDGE('',*,*,#18948,.F.);
#27489=ORIENTED_EDGE('',*,*,#18923,.F.);
#27490=ORIENTED_EDGE('',*,*,#17734,.F.);
#27491=ORIENTED_EDGE('',*,*,#18917,.F.);
#27492=ORIENTED_EDGE('',*,*,#18921,.F.);
#27493=ORIENTED_EDGE('',*,*,#18903,.F.);
#27494=ORIENTED_EDGE('',*,*,#17738,.F.);
#27495=ORIENTED_EDGE('',*,*,#18915,.F.);
#27496=ORIENTED_EDGE('',*,*,#18912,.F.);
#27497=ORIENTED_EDGE('',*,*,#18882,.F.);
#27498=ORIENTED_EDGE('',*,*,#17724,.F.);
#27499=ORIENTED_EDGE('',*,*,#18891,.F.);
#27500=ORIENTED_EDGE('',*,*,#18885,.F.);
#27501=ORIENTED_EDGE('',*,*,#18890,.F.);
#27502=ORIENTED_EDGE('',*,*,#17730,.F.);
#27503=ORIENTED_EDGE('',*,*,#18895,.F.);
#27504=ORIENTED_EDGE('',*,*,#18892,.F.);
#27505=ORIENTED_EDGE('',*,*,#18856,.F.);
#27506=ORIENTED_EDGE('',*,*,#17718,.F.);
#27507=ORIENTED_EDGE('',*,*,#18862,.F.);
#27508=ORIENTED_EDGE('',*,*,#18866,.F.);
#27509=ORIENTED_EDGE('',*,*,#18861,.F.);
#27510=ORIENTED_EDGE('',*,*,#17716,.F.);
#27511=ORIENTED_EDGE('',*,*,#18867,.F.);
#27512=ORIENTED_EDGE('',*,*,#18864,.F.);
#27513=ORIENTED_EDGE('',*,*,#18826,.F.);
#27514=ORIENTED_EDGE('',*,*,#17708,.F.);
#27515=ORIENTED_EDGE('',*,*,#18835,.F.);
#27516=ORIENTED_EDGE('',*,*,#18829,.F.);
#27517=ORIENTED_EDGE('',*,*,#18834,.F.);
#27518=ORIENTED_EDGE('',*,*,#17714,.F.);
#27519=ORIENTED_EDGE('',*,*,#18839,.F.);
#27520=ORIENTED_EDGE('',*,*,#18836,.F.);
#27521=ORIENTED_EDGE('',*,*,#18798,.F.);
#27522=ORIENTED_EDGE('',*,*,#17700,.F.);
#27523=ORIENTED_EDGE('',*,*,#18807,.F.);
#27524=ORIENTED_EDGE('',*,*,#18801,.F.);
#27525=ORIENTED_EDGE('',*,*,#18806,.F.);
#27526=ORIENTED_EDGE('',*,*,#17706,.F.);
#27527=ORIENTED_EDGE('',*,*,#18811,.F.);
#27528=ORIENTED_EDGE('',*,*,#18808,.F.);
#27529=ORIENTED_EDGE('',*,*,#18783,.F.);
#27530=ORIENTED_EDGE('',*,*,#17694,.F.);
#27531=ORIENTED_EDGE('',*,*,#18777,.F.);
#27532=ORIENTED_EDGE('',*,*,#18781,.F.);
#27533=ORIENTED_EDGE('',*,*,#18763,.F.);
#27534=ORIENTED_EDGE('',*,*,#17698,.F.);
#27535=ORIENTED_EDGE('',*,*,#18775,.F.);
#27536=ORIENTED_EDGE('',*,*,#18772,.F.);
#27537=ORIENTED_EDGE('',*,*,#18742,.F.);
#27538=ORIENTED_EDGE('',*,*,#17684,.F.);
#27539=ORIENTED_EDGE('',*,*,#18751,.F.);
#27540=ORIENTED_EDGE('',*,*,#18745,.F.);
#27541=ORIENTED_EDGE('',*,*,#18750,.F.);
#27542=ORIENTED_EDGE('',*,*,#17690,.F.);
#27543=ORIENTED_EDGE('',*,*,#18755,.F.);
#27544=ORIENTED_EDGE('',*,*,#18752,.F.);
#27545=ORIENTED_EDGE('',*,*,#18716,.F.);
#27546=ORIENTED_EDGE('',*,*,#17678,.F.);
#27547=ORIENTED_EDGE('',*,*,#18722,.F.);
#27548=ORIENTED_EDGE('',*,*,#18726,.F.);
#27549=ORIENTED_EDGE('',*,*,#18721,.F.);
#27550=ORIENTED_EDGE('',*,*,#17676,.F.);
#27551=ORIENTED_EDGE('',*,*,#18727,.F.);
#27552=ORIENTED_EDGE('',*,*,#18724,.F.);
#27553=ORIENTED_EDGE('',*,*,#18686,.F.);
#27554=ORIENTED_EDGE('',*,*,#17668,.F.);
#27555=ORIENTED_EDGE('',*,*,#18695,.F.);
#27556=ORIENTED_EDGE('',*,*,#18689,.F.);
#27557=ORIENTED_EDGE('',*,*,#18694,.F.);
#27558=ORIENTED_EDGE('',*,*,#17674,.F.);
#27559=ORIENTED_EDGE('',*,*,#18699,.F.);
#27560=ORIENTED_EDGE('',*,*,#18696,.F.);
#27561=ORIENTED_EDGE('',*,*,#18658,.F.);
#27562=ORIENTED_EDGE('',*,*,#17514,.F.);
#27563=ORIENTED_EDGE('',*,*,#18667,.F.);
#27564=ORIENTED_EDGE('',*,*,#18661,.F.);
#27565=ORIENTED_EDGE('',*,*,#18666,.F.);
#27566=ORIENTED_EDGE('',*,*,#17512,.F.);
#27567=ORIENTED_EDGE('',*,*,#17523,.F.);
#27568=ORIENTED_EDGE('',*,*,#18671,.F.);
#27569=ORIENTED_EDGE('',*,*,#18668,.F.);
#27570=ORIENTED_EDGE('',*,*,#18643,.F.);
#27571=ORIENTED_EDGE('',*,*,#17662,.F.);
#27572=ORIENTED_EDGE('',*,*,#18637,.F.);
#27573=ORIENTED_EDGE('',*,*,#18641,.F.);
#27574=ORIENTED_EDGE('',*,*,#18623,.F.);
#27575=ORIENTED_EDGE('',*,*,#17666,.F.);
#27576=ORIENTED_EDGE('',*,*,#18635,.F.);
#27577=ORIENTED_EDGE('',*,*,#18632,.F.);
#27578=ORIENTED_EDGE('',*,*,#18602,.F.);
#27579=ORIENTED_EDGE('',*,*,#17652,.F.);
#27580=ORIENTED_EDGE('',*,*,#18611,.F.);
#27581=ORIENTED_EDGE('',*,*,#18605,.F.);
#27582=ORIENTED_EDGE('',*,*,#18610,.F.);
#27583=ORIENTED_EDGE('',*,*,#17658,.F.);
#27584=ORIENTED_EDGE('',*,*,#18615,.F.);
#27585=ORIENTED_EDGE('',*,*,#18612,.F.);
#27586=ORIENTED_EDGE('',*,*,#18576,.F.);
#27587=ORIENTED_EDGE('',*,*,#17646,.F.);
#27588=ORIENTED_EDGE('',*,*,#18582,.F.);
#27589=ORIENTED_EDGE('',*,*,#18586,.F.);
#27590=ORIENTED_EDGE('',*,*,#18581,.F.);
#27591=ORIENTED_EDGE('',*,*,#17644,.F.);
#27592=ORIENTED_EDGE('',*,*,#18587,.F.);
#27593=ORIENTED_EDGE('',*,*,#18584,.F.);
#27594=ORIENTED_EDGE('',*,*,#18546,.F.);
#27595=ORIENTED_EDGE('',*,*,#17636,.F.);
#27596=ORIENTED_EDGE('',*,*,#18555,.F.);
#27597=ORIENTED_EDGE('',*,*,#18549,.F.);
#27598=ORIENTED_EDGE('',*,*,#18554,.F.);
#27599=ORIENTED_EDGE('',*,*,#17642,.F.);
#27600=ORIENTED_EDGE('',*,*,#18559,.F.);
#27601=ORIENTED_EDGE('',*,*,#18556,.F.);
#27602=ORIENTED_EDGE('',*,*,#18518,.F.);
#27603=ORIENTED_EDGE('',*,*,#17628,.F.);
#27604=ORIENTED_EDGE('',*,*,#18527,.F.);
#27605=ORIENTED_EDGE('',*,*,#18521,.F.);
#27606=ORIENTED_EDGE('',*,*,#18526,.F.);
#27607=ORIENTED_EDGE('',*,*,#17634,.F.);
#27608=ORIENTED_EDGE('',*,*,#18531,.F.);
#27609=ORIENTED_EDGE('',*,*,#18528,.F.);
#27610=ORIENTED_EDGE('',*,*,#18503,.F.);
#27611=ORIENTED_EDGE('',*,*,#17622,.F.);
#27612=ORIENTED_EDGE('',*,*,#18497,.F.);
#27613=ORIENTED_EDGE('',*,*,#18501,.F.);
#27614=ORIENTED_EDGE('',*,*,#18483,.F.);
#27615=ORIENTED_EDGE('',*,*,#17626,.F.);
#27616=ORIENTED_EDGE('',*,*,#18495,.F.);
#27617=ORIENTED_EDGE('',*,*,#18492,.F.);
#27618=ORIENTED_EDGE('',*,*,#18462,.F.);
#27619=ORIENTED_EDGE('',*,*,#17612,.F.);
#27620=ORIENTED_EDGE('',*,*,#18471,.F.);
#27621=ORIENTED_EDGE('',*,*,#18465,.F.);
#27622=ORIENTED_EDGE('',*,*,#18470,.F.);
#27623=ORIENTED_EDGE('',*,*,#17618,.F.);
#27624=ORIENTED_EDGE('',*,*,#18475,.F.);
#27625=ORIENTED_EDGE('',*,*,#18472,.F.);
#27626=ORIENTED_EDGE('',*,*,#18436,.F.);
#27627=ORIENTED_EDGE('',*,*,#17606,.F.);
#27628=ORIENTED_EDGE('',*,*,#18442,.F.);
#27629=ORIENTED_EDGE('',*,*,#18446,.F.);
#27630=ORIENTED_EDGE('',*,*,#18441,.F.);
#27631=ORIENTED_EDGE('',*,*,#17604,.F.);
#27632=ORIENTED_EDGE('',*,*,#18447,.F.);
#27633=ORIENTED_EDGE('',*,*,#18444,.F.);
#27634=ORIENTED_EDGE('',*,*,#18406,.F.);
#27635=ORIENTED_EDGE('',*,*,#17596,.F.);
#27636=ORIENTED_EDGE('',*,*,#18415,.F.);
#27637=ORIENTED_EDGE('',*,*,#18409,.F.);
#27638=ORIENTED_EDGE('',*,*,#18414,.F.);
#27639=ORIENTED_EDGE('',*,*,#17602,.F.);
#27640=ORIENTED_EDGE('',*,*,#18419,.F.);
#27641=ORIENTED_EDGE('',*,*,#18416,.F.);
#27642=ORIENTED_EDGE('',*,*,#18378,.F.);
#27643=ORIENTED_EDGE('',*,*,#17588,.F.);
#27644=ORIENTED_EDGE('',*,*,#18387,.F.);
#27645=ORIENTED_EDGE('',*,*,#18381,.F.);
#27646=ORIENTED_EDGE('',*,*,#18386,.F.);
#27647=ORIENTED_EDGE('',*,*,#17594,.F.);
#27648=ORIENTED_EDGE('',*,*,#18391,.F.);
#27649=ORIENTED_EDGE('',*,*,#18388,.F.);
#27650=ORIENTED_EDGE('',*,*,#18363,.F.);
#27651=ORIENTED_EDGE('',*,*,#17582,.F.);
#27652=ORIENTED_EDGE('',*,*,#18357,.F.);
#27653=ORIENTED_EDGE('',*,*,#18361,.F.);
#27654=ORIENTED_EDGE('',*,*,#18343,.F.);
#27655=ORIENTED_EDGE('',*,*,#17586,.F.);
#27656=ORIENTED_EDGE('',*,*,#18355,.F.);
#27657=ORIENTED_EDGE('',*,*,#18352,.F.);
#27658=ORIENTED_EDGE('',*,*,#18322,.F.);
#27659=ORIENTED_EDGE('',*,*,#17572,.F.);
#27660=ORIENTED_EDGE('',*,*,#18331,.F.);
#27661=ORIENTED_EDGE('',*,*,#18325,.F.);
#27662=ORIENTED_EDGE('',*,*,#18330,.F.);
#27663=ORIENTED_EDGE('',*,*,#17578,.F.);
#27664=ORIENTED_EDGE('',*,*,#18335,.F.);
#27665=ORIENTED_EDGE('',*,*,#18332,.F.);
#27666=ORIENTED_EDGE('',*,*,#18296,.F.);
#27667=ORIENTED_EDGE('',*,*,#17566,.F.);
#27668=ORIENTED_EDGE('',*,*,#18302,.F.);
#27669=ORIENTED_EDGE('',*,*,#18306,.F.);
#27670=ORIENTED_EDGE('',*,*,#18301,.F.);
#27671=ORIENTED_EDGE('',*,*,#17564,.F.);
#27672=ORIENTED_EDGE('',*,*,#18307,.F.);
#27673=ORIENTED_EDGE('',*,*,#18304,.F.);
#27674=ORIENTED_EDGE('',*,*,#18266,.F.);
#27675=ORIENTED_EDGE('',*,*,#17556,.F.);
#27676=ORIENTED_EDGE('',*,*,#18275,.F.);
#27677=ORIENTED_EDGE('',*,*,#18269,.F.);
#27678=ORIENTED_EDGE('',*,*,#18274,.F.);
#27679=ORIENTED_EDGE('',*,*,#17562,.F.);
#27680=ORIENTED_EDGE('',*,*,#18279,.F.);
#27681=ORIENTED_EDGE('',*,*,#18276,.F.);
#27682=ORIENTED_EDGE('',*,*,#18238,.F.);
#27683=ORIENTED_EDGE('',*,*,#17548,.F.);
#27684=ORIENTED_EDGE('',*,*,#18247,.F.);
#27685=ORIENTED_EDGE('',*,*,#18241,.F.);
#27686=ORIENTED_EDGE('',*,*,#18246,.F.);
#27687=ORIENTED_EDGE('',*,*,#17554,.F.);
#27688=ORIENTED_EDGE('',*,*,#18251,.F.);
#27689=ORIENTED_EDGE('',*,*,#18248,.F.);
#27690=ORIENTED_EDGE('',*,*,#18223,.F.);
#27691=ORIENTED_EDGE('',*,*,#17542,.F.);
#27692=ORIENTED_EDGE('',*,*,#18217,.F.);
#27693=ORIENTED_EDGE('',*,*,#18221,.F.);
#27694=ORIENTED_EDGE('',*,*,#18203,.F.);
#27695=ORIENTED_EDGE('',*,*,#17546,.F.);
#27696=ORIENTED_EDGE('',*,*,#18215,.F.);
#27697=ORIENTED_EDGE('',*,*,#18212,.F.);
#27698=ORIENTED_EDGE('',*,*,#18182,.F.);
#27699=ORIENTED_EDGE('',*,*,#17532,.F.);
#27700=ORIENTED_EDGE('',*,*,#18191,.F.);
#27701=ORIENTED_EDGE('',*,*,#18185,.F.);
#27702=ORIENTED_EDGE('',*,*,#18190,.F.);
#27703=ORIENTED_EDGE('',*,*,#17538,.F.);
#27704=ORIENTED_EDGE('',*,*,#18195,.F.);
#27705=ORIENTED_EDGE('',*,*,#18192,.F.);
#27706=ORIENTED_EDGE('',*,*,#18156,.F.);
#27707=ORIENTED_EDGE('',*,*,#17526,.F.);
#27708=ORIENTED_EDGE('',*,*,#18162,.F.);
#27709=ORIENTED_EDGE('',*,*,#18166,.F.);
#27710=ORIENTED_EDGE('',*,*,#18161,.F.);
#27711=ORIENTED_EDGE('',*,*,#17524,.F.);
#27712=ORIENTED_EDGE('',*,*,#18167,.F.);
#27713=ORIENTED_EDGE('',*,*,#18164,.F.);
#27714=ORIENTED_EDGE('',*,*,#18135,.F.);
#27715=ORIENTED_EDGE('',*,*,#20183,.T.);
#27716=ORIENTED_EDGE('',*,*,#20184,.F.);
#27717=ORIENTED_EDGE('',*,*,#20183,.F.);
#27718=ORIENTED_EDGE('',*,*,#18136,.F.);
#27719=ORIENTED_EDGE('',*,*,#20185,.T.);
#27720=ORIENTED_EDGE('',*,*,#20186,.F.);
#27721=ORIENTED_EDGE('',*,*,#20185,.F.);
#27722=ORIENTED_EDGE('',*,*,#18137,.F.);
#27723=ORIENTED_EDGE('',*,*,#20187,.T.);
#27724=ORIENTED_EDGE('',*,*,#20188,.F.);
#27725=ORIENTED_EDGE('',*,*,#20187,.F.);
#27726=ORIENTED_EDGE('',*,*,#18138,.F.);
#27727=ORIENTED_EDGE('',*,*,#20189,.T.);
#27728=ORIENTED_EDGE('',*,*,#20190,.F.);
#27729=ORIENTED_EDGE('',*,*,#20189,.F.);
#27730=ORIENTED_EDGE('',*,*,#18139,.F.);
#27731=ORIENTED_EDGE('',*,*,#20191,.T.);
#27732=ORIENTED_EDGE('',*,*,#20192,.F.);
#27733=ORIENTED_EDGE('',*,*,#20191,.F.);
#27734=ORIENTED_EDGE('',*,*,#20193,.F.);
#27735=ORIENTED_EDGE('',*,*,#20194,.T.);
#27736=ORIENTED_EDGE('',*,*,#20195,.T.);
#27737=ORIENTED_EDGE('',*,*,#20194,.F.);
#27738=ORIENTED_EDGE('',*,*,#20195,.F.);
#27739=ORIENTED_EDGE('',*,*,#20196,.T.);
#27740=ORIENTED_EDGE('',*,*,#20197,.F.);
#27741=ORIENTED_EDGE('',*,*,#20196,.F.);
#27742=ORIENTED_EDGE('',*,*,#18098,.F.);
#27743=ORIENTED_EDGE('',*,*,#20198,.F.);
#27744=ORIENTED_EDGE('',*,*,#20199,.F.);
#27745=ORIENTED_EDGE('',*,*,#18133,.T.);
#27746=ORIENTED_EDGE('',*,*,#18101,.F.);
#27747=ORIENTED_EDGE('',*,*,#20200,.F.);
#27748=ORIENTED_EDGE('',*,*,#20201,.F.);
#27749=ORIENTED_EDGE('',*,*,#20198,.T.);
#27750=ORIENTED_EDGE('',*,*,#18104,.F.);
#27751=ORIENTED_EDGE('',*,*,#20202,.F.);
#27752=ORIENTED_EDGE('',*,*,#20203,.F.);
#27753=ORIENTED_EDGE('',*,*,#20200,.T.);
#27754=ORIENTED_EDGE('',*,*,#18107,.F.);
#27755=ORIENTED_EDGE('',*,*,#18124,.F.);
#27756=ORIENTED_EDGE('',*,*,#20204,.F.);
#27757=ORIENTED_EDGE('',*,*,#20202,.T.);
#27758=ORIENTED_EDGE('',*,*,#17494,.T.);
#27759=ORIENTED_EDGE('',*,*,#18126,.T.);
#27760=ORIENTED_EDGE('',*,*,#18128,.T.);
#27761=ORIENTED_EDGE('',*,*,#18130,.T.);
#27762=ORIENTED_EDGE('',*,*,#18132,.T.);
#27763=ORIENTED_EDGE('',*,*,#18134,.T.);
#27764=ORIENTED_EDGE('',*,*,#20199,.T.);
#27765=ORIENTED_EDGE('',*,*,#20201,.T.);
#27766=ORIENTED_EDGE('',*,*,#20203,.T.);
#27767=ORIENTED_EDGE('',*,*,#20204,.T.);
#27768=ORIENTED_EDGE('',*,*,#18123,.T.);
#27769=ORIENTED_EDGE('',*,*,#17480,.T.);
#27770=ORIENTED_EDGE('',*,*,#20205,.T.);
#27771=ORIENTED_EDGE('',*,*,#20206,.F.);
#27772=ORIENTED_EDGE('',*,*,#20205,.F.);
#27773=ORIENTED_EDGE('',*,*,#20206,.T.);
#27774=ORIENTED_EDGE('',*,*,#20197,.T.);
#27775=ORIENTED_EDGE('',*,*,#20193,.T.);
#27776=ORIENTED_EDGE('',*,*,#20207,.T.);
#27777=ORIENTED_EDGE('',*,*,#20208,.F.);
#27778=ORIENTED_EDGE('',*,*,#20207,.F.);
#27779=ORIENTED_EDGE('',*,*,#20208,.T.);
#27780=ORIENTED_EDGE('',*,*,#17470,.F.);
#27781=ORIENTED_EDGE('',*,*,#17472,.T.);
#27782=ORIENTED_EDGE('',*,*,#20209,.T.);
#27783=ORIENTED_EDGE('',*,*,#20210,.F.);
#27784=ORIENTED_EDGE('',*,*,#20209,.F.);
#27785=ORIENTED_EDGE('',*,*,#20211,.F.);
#27786=ORIENTED_EDGE('',*,*,#20210,.T.);
#27787=ORIENTED_EDGE('',*,*,#20211,.T.);
#27788=ORIENTED_EDGE('',*,*,#20212,.T.);
#27789=ORIENTED_EDGE('',*,*,#20213,.F.);
#27790=ORIENTED_EDGE('',*,*,#20212,.F.);
#27791=ORIENTED_EDGE('',*,*,#20213,.T.);
#27792=ORIENTED_EDGE('',*,*,#20214,.T.);
#27793=ORIENTED_EDGE('',*,*,#17465,.F.);
#27794=ORIENTED_EDGE('',*,*,#20214,.F.);
#27795=ORIENTED_EDGE('',*,*,#20215,.F.);
#27796=ORIENTED_EDGE('',*,*,#20216,.T.);
#27797=ORIENTED_EDGE('',*,*,#17461,.T.);
#27798=ORIENTED_EDGE('',*,*,#20216,.F.);
#27799=ORIENTED_EDGE('',*,*,#20217,.F.);
#27800=ORIENTED_EDGE('',*,*,#20215,.T.);
#27801=ORIENTED_EDGE('',*,*,#20192,.T.);
#27802=ORIENTED_EDGE('',*,*,#20190,.T.);
#27803=ORIENTED_EDGE('',*,*,#20188,.T.);
#27804=ORIENTED_EDGE('',*,*,#20186,.T.);
#27805=ORIENTED_EDGE('',*,*,#20184,.T.);
#27806=ORIENTED_EDGE('',*,*,#20217,.T.);
#27807=ORIENTED_EDGE('',*,*,#20218,.T.);
#27808=ORIENTED_EDGE('',*,*,#20219,.F.);
#27809=ORIENTED_EDGE('',*,*,#20218,.F.);
#27810=ORIENTED_EDGE('',*,*,#20219,.T.);
#27811=ORIENTED_EDGE('',*,*,#20220,.T.);
#27812=ORIENTED_EDGE('',*,*,#20108,.F.);
#27813=ORIENTED_EDGE('',*,*,#20220,.F.);
#31928=CONICAL_SURFACE('',#34367,39.77639320225,0.553574358897046);
#31929=CONICAL_SURFACE('',#34372,38.5,1.10714871779409);
#31930=CONICAL_SURFACE('',#34377,36.97360679775,1.33897252229449);
#31931=CONICAL_SURFACE('',#34381,26.25,0.785398163397448);
#31932=CONICAL_SURFACE('',#34389,31.9267766952966,1.17809724509617);
#31933=CONICAL_SURFACE('',#34393,33.,0.78539816339745);
#31934=CONICAL_SURFACE('',#34398,33.8502380998955,0.44683437712894);
#31935=CONICAL_SURFACE('',#34401,35.25,0.108270590860456);
#31936=CONICAL_SURFACE('',#34403,126.961414092626,1.19422068631379);
#31937=CONICAL_SURFACE('',#34408,129.25,0.98279372324733);
#31938=CONICAL_SURFACE('',#34411,124.,1.40564764938027);
#31939=CONICAL_SURFACE('',#34413,131.441987426416,0.813147416020307);
#31940=CONICAL_SURFACE('',#34416,133.,0.643501108793283);
#31941=CONICAL_SURFACE('',#34419,134.437780860397,0.501135889531925);
#31942=CONICAL_SURFACE('',#34422,135.25,0.358770670270573);
#31943=CONICAL_SURFACE('',#34425,135.912219139603,0.17938533513529);
#31944=CONICAL_SURFACE('',#34864,51.75,0.785398163397448);
#31945=CONICAL_SURFACE('',#34867,14.75,0.785398163397448);
#31946=CONICAL_SURFACE('',#34870,51.75,0.785398163397457);
#31947=CONICAL_SURFACE('',#34873,14.75,0.785398163397448);
#31948=CONICAL_SURFACE('',#34876,51.75,0.785398163397457);
#31949=CONICAL_SURFACE('',#34879,14.75,0.785398163397448);
#31950=CONICAL_SURFACE('',#34882,51.75,0.785398163397448);
#31951=CONICAL_SURFACE('',#34885,14.75,0.785398163397453);
#31952=CONICAL_SURFACE('',#34888,51.75,0.785398163397448);
#31953=CONICAL_SURFACE('',#34891,14.75,0.785398163397453);
#31954=CONICAL_SURFACE('',#35920,127.185823536562,0.418990612504199);
#31955=CONICAL_SURFACE('',#35925,128.,0.837981225008393);
#31956=CONICAL_SURFACE('',#35960,138.753401519042,0.70282382469014);
#31957=CONICAL_SURFACE('',#35968,137.5,1.40564764938027);
#31958=CONICAL_SURFACE('',#35969,129.064176463438,1.20438877590164);
#31959=CONICAL_SURFACE('',#35973,138.823223304703,0.392699081698721);
#31960=CONICAL_SURFACE('',#35975,138.5,0.785398163397447);
#31961=CONICAL_SURFACE('',#35977,137.926776695297,1.17809724509618);
#31962=CONICAL_SURFACE('',#36132,25.,1.10714871779409);
#31963=CONICAL_SURFACE('',#36158,32.9,0.785398163397449);
#31964=CONICAL_SURFACE('',#36159,43.,0.785398163397448);
#31965=CONICAL_SURFACE('',#36163,124.75,1.05165021254837);
#31966=CONICAL_SURFACE('',#36165,126.75,1.10714871779408);
#32113=ADVANCED_FACE('',(#3139),#31928,.T.);
#32114=ADVANCED_FACE('',(#3140),#31929,.T.);
#32115=ADVANCED_FACE('',(#3141),#2992,.T.);
#32116=ADVANCED_FACE('',(#3142),#31930,.T.);
#32117=ADVANCED_FACE('',(#3143,#1130),#1335,.T.);
#32118=ADVANCED_FACE('',(#3144),#31931,.F.);
#32119=ADVANCED_FACE('',(#3145),#2993,.F.);
#32120=ADVANCED_FACE('',(#3146,#1131),#1336,.T.);
#32121=ADVANCED_FACE('',(#3147),#31932,.T.);
#32122=ADVANCED_FACE('',(#3148),#31933,.T.);
#32123=ADVANCED_FACE('',(#3149,#1132),#1337,.T.);
#32124=ADVANCED_FACE('',(#3150),#31934,.T.);
#32125=ADVANCED_FACE('',(#3151),#31935,.T.);
#32126=ADVANCED_FACE('',(#3152),#31936,.T.);
#32127=ADVANCED_FACE('',(#3153),#31937,.T.);
#32128=ADVANCED_FACE('',(#3154),#31938,.T.);
#32129=ADVANCED_FACE('',(#3155),#31939,.T.);
#32130=ADVANCED_FACE('',(#3156),#31940,.T.);
#32131=ADVANCED_FACE('',(#3157),#31941,.T.);
#32132=ADVANCED_FACE('',(#3158),#31942,.T.);
#32133=ADVANCED_FACE('',(#3159),#31943,.T.);
#32134=ADVANCED_FACE('',(#3160,#1133,#1134,#1135,#1136,#1137,#1138,#1139,
#1140,#1141,#1142,#1143,#1144,#1145,#1146,#1147,#1148,#1149,#1150,#1151,
#1152,#1153,#1154,#1155,#1156,#1157,#1158,#1159,#1160,#1161,#1162,#1163,
#1164,#1165,#1166,#1167,#1168,#1169,#1170,#1171,#1172,#1173,#1174,#1175,
#1176,#1177,#1178,#1179,#1180,#1181,#1182,#1183,#1184,#1185,#1186,#1187,
#1188,#1189,#1190,#1191,#1192,#1193,#1194,#1195,#1196,#1197,#1198,#1199,
#1200,#1201,#1202,#1203),#2994,.T.);
#32135=ADVANCED_FACE('',(#3161),#31944,.T.);
#32136=ADVANCED_FACE('',(#3162),#31945,.T.);
#32137=ADVANCED_FACE('',(#3163),#31946,.T.);
#32138=ADVANCED_FACE('',(#3164),#31947,.T.);
#32139=ADVANCED_FACE('',(#3165),#31948,.T.);
#32140=ADVANCED_FACE('',(#3166),#31949,.T.);
#32141=ADVANCED_FACE('',(#3167),#31950,.T.);
#32142=ADVANCED_FACE('',(#3168),#31951,.T.);
#32143=ADVANCED_FACE('',(#3169),#31952,.T.);
#32144=ADVANCED_FACE('',(#3170),#31953,.T.);
#32145=ADVANCED_FACE('',(#3171),#2995,.T.);
#32146=ADVANCED_FACE('',(#3172),#2996,.T.);
#32147=ADVANCED_FACE('',(#3173),#2997,.T.);
#32148=ADVANCED_FACE('',(#3174),#2998,.T.);
#32149=ADVANCED_FACE('',(#3175),#2999,.T.);
#32150=ADVANCED_FACE('',(#3176),#3000,.T.);
#32151=ADVANCED_FACE('',(#3177,#1204,#1205,#1206,#1207,#1208,#1209),#1338,
 .T.);
#32152=ADVANCED_FACE('',(#3178),#1339,.T.);
#32153=ADVANCED_FACE('',(#3179),#1340,.T.);
#32154=ADVANCED_FACE('',(#3180),#1341,.T.);
#32155=ADVANCED_FACE('',(#3181),#1342,.T.);
#32156=ADVANCED_FACE('',(#3182),#1343,.T.);
#32157=ADVANCED_FACE('',(#3183),#1344,.T.);
#32158=ADVANCED_FACE('',(#3184),#1345,.T.);
#32159=ADVANCED_FACE('',(#3185),#1346,.T.);
#32160=ADVANCED_FACE('',(#3186),#1347,.T.);
#32161=ADVANCED_FACE('',(#3187),#1348,.T.);
#32162=ADVANCED_FACE('',(#3188),#1349,.T.);
#32163=ADVANCED_FACE('',(#3189),#1350,.T.);
#32164=ADVANCED_FACE('',(#3190),#1351,.T.);
#32165=ADVANCED_FACE('',(#3191),#1352,.T.);
#32166=ADVANCED_FACE('',(#3192),#1353,.T.);
#32167=ADVANCED_FACE('',(#3193),#1354,.T.);
#32168=ADVANCED_FACE('',(#3194),#1355,.T.);
#32169=ADVANCED_FACE('',(#3195),#1356,.T.);
#32170=ADVANCED_FACE('',(#3196),#1357,.T.);
#32171=ADVANCED_FACE('',(#3197),#1358,.T.);
#32172=ADVANCED_FACE('',(#3198),#1359,.T.);
#32173=ADVANCED_FACE('',(#3199),#1360,.T.);
#32174=ADVANCED_FACE('',(#3200),#1361,.T.);
#32175=ADVANCED_FACE('',(#3201),#1362,.T.);
#32176=ADVANCED_FACE('',(#3202),#1363,.T.);
#32177=ADVANCED_FACE('',(#3203),#1364,.T.);
#32178=ADVANCED_FACE('',(#3204),#1365,.F.);
#32179=ADVANCED_FACE('',(#3205),#1366,.T.);
#32180=ADVANCED_FACE('',(#3206),#1367,.T.);
#32181=ADVANCED_FACE('',(#3207),#1368,.T.);
#32182=ADVANCED_FACE('',(#3208),#1369,.T.);
#32183=ADVANCED_FACE('',(#3209),#1370,.T.);
#32184=ADVANCED_FACE('',(#3210),#1371,.T.);
#32185=ADVANCED_FACE('',(#3211),#1372,.T.);
#32186=ADVANCED_FACE('',(#3212),#1373,.T.);
#32187=ADVANCED_FACE('',(#3213),#1374,.T.);
#32188=ADVANCED_FACE('',(#3214),#1375,.T.);
#32189=ADVANCED_FACE('',(#3215),#1376,.T.);
#32190=ADVANCED_FACE('',(#3216),#1377,.T.);
#32191=ADVANCED_FACE('',(#3217),#1378,.T.);
#32192=ADVANCED_FACE('',(#3218),#1379,.T.);
#32193=ADVANCED_FACE('',(#3219),#1380,.T.);
#32194=ADVANCED_FACE('',(#3220),#1381,.T.);
#32195=ADVANCED_FACE('',(#3221),#1382,.T.);
#32196=ADVANCED_FACE('',(#3222),#1383,.T.);
#32197=ADVANCED_FACE('',(#3223),#1384,.T.);
#32198=ADVANCED_FACE('',(#3224),#1385,.T.);
#32199=ADVANCED_FACE('',(#3225),#1386,.T.);
#32200=ADVANCED_FACE('',(#3226),#1387,.T.);
#32201=ADVANCED_FACE('',(#3227),#1388,.T.);
#32202=ADVANCED_FACE('',(#3228),#1389,.T.);
#32203=ADVANCED_FACE('',(#3229),#1390,.T.);
#32204=ADVANCED_FACE('',(#3230),#1391,.T.);
#32205=ADVANCED_FACE('',(#3231),#1392,.T.);
#32206=ADVANCED_FACE('',(#3232),#1393,.F.);
#32207=ADVANCED_FACE('',(#3233),#1394,.T.);
#32208=ADVANCED_FACE('',(#3234),#1395,.T.);
#32209=ADVANCED_FACE('',(#3235),#1396,.T.);
#32210=ADVANCED_FACE('',(#3236),#1397,.T.);
#32211=ADVANCED_FACE('',(#3237),#1398,.T.);
#32212=ADVANCED_FACE('',(#3238),#1399,.T.);
#32213=ADVANCED_FACE('',(#3239),#1400,.T.);
#32214=ADVANCED_FACE('',(#3240),#1401,.T.);
#32215=ADVANCED_FACE('',(#3241),#1402,.T.);
#32216=ADVANCED_FACE('',(#3242),#1403,.T.);
#32217=ADVANCED_FACE('',(#3243),#1404,.T.);
#32218=ADVANCED_FACE('',(#3244),#1405,.T.);
#32219=ADVANCED_FACE('',(#3245),#1406,.T.);
#32220=ADVANCED_FACE('',(#3246),#1407,.T.);
#32221=ADVANCED_FACE('',(#3247),#1408,.F.);
#32222=ADVANCED_FACE('',(#3248),#1409,.T.);
#32223=ADVANCED_FACE('',(#3249),#1410,.T.);
#32224=ADVANCED_FACE('',(#3250),#1411,.T.);
#32225=ADVANCED_FACE('',(#3251),#1412,.T.);
#32226=ADVANCED_FACE('',(#3252),#1413,.T.);
#32227=ADVANCED_FACE('',(#3253),#1414,.T.);
#32228=ADVANCED_FACE('',(#3254),#1415,.T.);
#32229=ADVANCED_FACE('',(#3255),#1416,.T.);
#32230=ADVANCED_FACE('',(#3256),#1417,.T.);
#32231=ADVANCED_FACE('',(#3257),#1418,.T.);
#32232=ADVANCED_FACE('',(#3258),#1419,.T.);
#32233=ADVANCED_FACE('',(#3259),#1420,.T.);
#32234=ADVANCED_FACE('',(#3260),#1421,.T.);
#32235=ADVANCED_FACE('',(#3261),#1422,.T.);
#32236=ADVANCED_FACE('',(#3262),#1423,.T.);
#32237=ADVANCED_FACE('',(#3263),#1424,.T.);
#32238=ADVANCED_FACE('',(#3264),#1425,.T.);
#32239=ADVANCED_FACE('',(#3265),#1426,.T.);
#32240=ADVANCED_FACE('',(#3266),#1427,.T.);
#32241=ADVANCED_FACE('',(#3267),#1428,.T.);
#32242=ADVANCED_FACE('',(#3268),#1429,.T.);
#32243=ADVANCED_FACE('',(#3269),#1430,.T.);
#32244=ADVANCED_FACE('',(#3270),#1431,.T.);
#32245=ADVANCED_FACE('',(#3271),#1432,.T.);
#32246=ADVANCED_FACE('',(#3272),#1433,.T.);
#32247=ADVANCED_FACE('',(#3273),#1434,.T.);
#32248=ADVANCED_FACE('',(#3274),#1435,.T.);
#32249=ADVANCED_FACE('',(#3275),#1436,.T.);
#32250=ADVANCED_FACE('',(#3276),#1437,.F.);
#32251=ADVANCED_FACE('',(#3277),#1438,.T.);
#32252=ADVANCED_FACE('',(#3278),#1439,.T.);
#32253=ADVANCED_FACE('',(#3279),#1440,.T.);
#32254=ADVANCED_FACE('',(#3280),#1441,.T.);
#32255=ADVANCED_FACE('',(#3281),#1442,.T.);
#32256=ADVANCED_FACE('',(#3282),#1443,.T.);
#32257=ADVANCED_FACE('',(#3283),#1444,.T.);
#32258=ADVANCED_FACE('',(#3284),#1445,.T.);
#32259=ADVANCED_FACE('',(#3285),#1446,.T.);
#32260=ADVANCED_FACE('',(#3286),#1447,.T.);
#32261=ADVANCED_FACE('',(#3287),#1448,.T.);
#32262=ADVANCED_FACE('',(#3288),#1449,.T.);
#32263=ADVANCED_FACE('',(#3289),#1450,.T.);
#32264=ADVANCED_FACE('',(#3290),#1451,.T.);
#32265=ADVANCED_FACE('',(#3291),#1452,.T.);
#32266=ADVANCED_FACE('',(#3292),#1453,.T.);
#32267=ADVANCED_FACE('',(#3293),#1454,.T.);
#32268=ADVANCED_FACE('',(#3294),#1455,.T.);
#32269=ADVANCED_FACE('',(#3295),#1456,.T.);
#32270=ADVANCED_FACE('',(#3296),#1457,.T.);
#32271=ADVANCED_FACE('',(#3297),#1458,.T.);
#32272=ADVANCED_FACE('',(#3298),#1459,.T.);
#32273=ADVANCED_FACE('',(#3299),#1460,.T.);
#32274=ADVANCED_FACE('',(#3300),#1461,.T.);
#32275=ADVANCED_FACE('',(#3301),#1462,.T.);
#32276=ADVANCED_FACE('',(#3302),#1463,.T.);
#32277=ADVANCED_FACE('',(#3303),#1464,.T.);
#32278=ADVANCED_FACE('',(#3304),#1465,.F.);
#32279=ADVANCED_FACE('',(#3305),#1466,.T.);
#32280=ADVANCED_FACE('',(#3306),#1467,.T.);
#32281=ADVANCED_FACE('',(#3307),#1468,.T.);
#32282=ADVANCED_FACE('',(#3308),#1469,.T.);
#32283=ADVANCED_FACE('',(#3309),#1470,.T.);
#32284=ADVANCED_FACE('',(#3310),#1471,.T.);
#32285=ADVANCED_FACE('',(#3311),#1472,.T.);
#32286=ADVANCED_FACE('',(#3312),#1473,.T.);
#32287=ADVANCED_FACE('',(#3313),#1474,.T.);
#32288=ADVANCED_FACE('',(#3314),#1475,.T.);
#32289=ADVANCED_FACE('',(#3315),#1476,.T.);
#32290=ADVANCED_FACE('',(#3316),#1477,.T.);
#32291=ADVANCED_FACE('',(#3317),#1478,.T.);
#32292=ADVANCED_FACE('',(#3318),#1479,.T.);
#32293=ADVANCED_FACE('',(#3319),#1480,.F.);
#32294=ADVANCED_FACE('',(#3320),#1481,.T.);
#32295=ADVANCED_FACE('',(#3321),#1482,.T.);
#32296=ADVANCED_FACE('',(#3322),#1483,.T.);
#32297=ADVANCED_FACE('',(#3323),#1484,.T.);
#32298=ADVANCED_FACE('',(#3324),#1485,.T.);
#32299=ADVANCED_FACE('',(#3325),#1486,.T.);
#32300=ADVANCED_FACE('',(#3326),#1487,.T.);
#32301=ADVANCED_FACE('',(#3327),#1488,.T.);
#32302=ADVANCED_FACE('',(#3328),#1489,.T.);
#32303=ADVANCED_FACE('',(#3329),#1490,.T.);
#32304=ADVANCED_FACE('',(#3330),#1491,.T.);
#32305=ADVANCED_FACE('',(#3331),#1492,.T.);
#32306=ADVANCED_FACE('',(#3332),#1493,.T.);
#32307=ADVANCED_FACE('',(#3333),#1494,.T.);
#32308=ADVANCED_FACE('',(#3334),#1495,.T.);
#32309=ADVANCED_FACE('',(#3335),#1496,.T.);
#32310=ADVANCED_FACE('',(#3336),#1497,.T.);
#32311=ADVANCED_FACE('',(#3337),#1498,.T.);
#32312=ADVANCED_FACE('',(#3338),#1499,.T.);
#32313=ADVANCED_FACE('',(#3339),#1500,.T.);
#32314=ADVANCED_FACE('',(#3340),#1501,.T.);
#32315=ADVANCED_FACE('',(#3341),#1502,.T.);
#32316=ADVANCED_FACE('',(#3342),#1503,.T.);
#32317=ADVANCED_FACE('',(#3343),#1504,.T.);
#32318=ADVANCED_FACE('',(#3344),#1505,.T.);
#32319=ADVANCED_FACE('',(#3345),#1506,.T.);
#32320=ADVANCED_FACE('',(#3346),#1507,.T.);
#32321=ADVANCED_FACE('',(#3347),#1508,.T.);
#32322=ADVANCED_FACE('',(#3348),#1509,.F.);
#32323=ADVANCED_FACE('',(#3349),#1510,.T.);
#32324=ADVANCED_FACE('',(#3350),#1511,.T.);
#32325=ADVANCED_FACE('',(#3351),#1512,.T.);
#32326=ADVANCED_FACE('',(#3352),#1513,.T.);
#32327=ADVANCED_FACE('',(#3353),#1514,.T.);
#32328=ADVANCED_FACE('',(#3354),#1515,.T.);
#32329=ADVANCED_FACE('',(#3355),#1516,.T.);
#32330=ADVANCED_FACE('',(#3356),#1517,.T.);
#32331=ADVANCED_FACE('',(#3357),#1518,.T.);
#32332=ADVANCED_FACE('',(#3358),#1519,.T.);
#32333=ADVANCED_FACE('',(#3359),#1520,.T.);
#32334=ADVANCED_FACE('',(#3360),#1521,.T.);
#32335=ADVANCED_FACE('',(#3361),#1522,.T.);
#32336=ADVANCED_FACE('',(#3362),#1523,.T.);
#32337=ADVANCED_FACE('',(#3363),#1524,.T.);
#32338=ADVANCED_FACE('',(#3364),#1525,.T.);
#32339=ADVANCED_FACE('',(#3365),#1526,.T.);
#32340=ADVANCED_FACE('',(#3366),#1527,.T.);
#32341=ADVANCED_FACE('',(#3367),#1528,.T.);
#32342=ADVANCED_FACE('',(#3368),#1529,.T.);
#32343=ADVANCED_FACE('',(#3369),#1530,.T.);
#32344=ADVANCED_FACE('',(#3370),#1531,.T.);
#32345=ADVANCED_FACE('',(#3371),#1532,.T.);
#32346=ADVANCED_FACE('',(#3372),#1533,.T.);
#32347=ADVANCED_FACE('',(#3373),#1534,.T.);
#32348=ADVANCED_FACE('',(#3374),#1535,.T.);
#32349=ADVANCED_FACE('',(#3375),#1536,.T.);
#32350=ADVANCED_FACE('',(#3376),#1537,.F.);
#32351=ADVANCED_FACE('',(#3377),#1538,.T.);
#32352=ADVANCED_FACE('',(#3378),#1539,.T.);
#32353=ADVANCED_FACE('',(#3379),#1540,.T.);
#32354=ADVANCED_FACE('',(#3380),#1541,.T.);
#32355=ADVANCED_FACE('',(#3381),#1542,.T.);
#32356=ADVANCED_FACE('',(#3382),#1543,.T.);
#32357=ADVANCED_FACE('',(#3383),#1544,.T.);
#32358=ADVANCED_FACE('',(#3384),#1545,.T.);
#32359=ADVANCED_FACE('',(#3385),#1546,.T.);
#32360=ADVANCED_FACE('',(#3386),#1547,.T.);
#32361=ADVANCED_FACE('',(#3387),#1548,.T.);
#32362=ADVANCED_FACE('',(#3388),#1549,.T.);
#32363=ADVANCED_FACE('',(#3389),#1550,.T.);
#32364=ADVANCED_FACE('',(#3390),#1551,.T.);
#32365=ADVANCED_FACE('',(#3391),#1552,.F.);
#32366=ADVANCED_FACE('',(#3392),#1553,.T.);
#32367=ADVANCED_FACE('',(#3393),#1554,.T.);
#32368=ADVANCED_FACE('',(#3394),#1555,.T.);
#32369=ADVANCED_FACE('',(#3395),#1556,.T.);
#32370=ADVANCED_FACE('',(#3396),#1557,.T.);
#32371=ADVANCED_FACE('',(#3397),#1558,.T.);
#32372=ADVANCED_FACE('',(#3398),#1559,.T.);
#32373=ADVANCED_FACE('',(#3399),#1560,.T.);
#32374=ADVANCED_FACE('',(#3400),#1561,.T.);
#32375=ADVANCED_FACE('',(#3401),#1562,.T.);
#32376=ADVANCED_FACE('',(#3402),#1563,.T.);
#32377=ADVANCED_FACE('',(#3403),#1564,.T.);
#32378=ADVANCED_FACE('',(#3404),#1565,.T.);
#32379=ADVANCED_FACE('',(#3405),#1566,.T.);
#32380=ADVANCED_FACE('',(#3406),#1567,.T.);
#32381=ADVANCED_FACE('',(#3407),#1568,.T.);
#32382=ADVANCED_FACE('',(#3408),#1569,.T.);
#32383=ADVANCED_FACE('',(#3409),#1570,.T.);
#32384=ADVANCED_FACE('',(#3410),#1571,.T.);
#32385=ADVANCED_FACE('',(#3411),#1572,.T.);
#32386=ADVANCED_FACE('',(#3412),#1573,.T.);
#32387=ADVANCED_FACE('',(#3413),#1574,.T.);
#32388=ADVANCED_FACE('',(#3414),#1575,.T.);
#32389=ADVANCED_FACE('',(#3415),#1576,.T.);
#32390=ADVANCED_FACE('',(#3416),#1577,.T.);
#32391=ADVANCED_FACE('',(#3417),#1578,.T.);
#32392=ADVANCED_FACE('',(#3418),#1579,.T.);
#32393=ADVANCED_FACE('',(#3419),#1580,.T.);
#32394=ADVANCED_FACE('',(#3420),#1581,.F.);
#32395=ADVANCED_FACE('',(#3421),#1582,.T.);
#32396=ADVANCED_FACE('',(#3422),#1583,.T.);
#32397=ADVANCED_FACE('',(#3423),#1584,.T.);
#32398=ADVANCED_FACE('',(#3424),#1585,.T.);
#32399=ADVANCED_FACE('',(#3425),#1586,.T.);
#32400=ADVANCED_FACE('',(#3426),#1587,.T.);
#32401=ADVANCED_FACE('',(#3427),#1588,.T.);
#32402=ADVANCED_FACE('',(#3428),#1589,.T.);
#32403=ADVANCED_FACE('',(#3429),#1590,.T.);
#32404=ADVANCED_FACE('',(#3430),#1591,.T.);
#32405=ADVANCED_FACE('',(#3431),#1592,.T.);
#32406=ADVANCED_FACE('',(#3432),#1593,.T.);
#32407=ADVANCED_FACE('',(#3433),#1594,.T.);
#32408=ADVANCED_FACE('',(#3434),#1595,.T.);
#32409=ADVANCED_FACE('',(#3435),#1596,.T.);
#32410=ADVANCED_FACE('',(#3436),#1597,.T.);
#32411=ADVANCED_FACE('',(#3437),#1598,.T.);
#32412=ADVANCED_FACE('',(#3438),#1599,.T.);
#32413=ADVANCED_FACE('',(#3439),#1600,.T.);
#32414=ADVANCED_FACE('',(#3440),#1601,.T.);
#32415=ADVANCED_FACE('',(#3441),#1602,.T.);
#32416=ADVANCED_FACE('',(#3442),#1603,.T.);
#32417=ADVANCED_FACE('',(#3443),#1604,.T.);
#32418=ADVANCED_FACE('',(#3444),#1605,.T.);
#32419=ADVANCED_FACE('',(#3445),#1606,.T.);
#32420=ADVANCED_FACE('',(#3446),#1607,.T.);
#32421=ADVANCED_FACE('',(#3447),#1608,.T.);
#32422=ADVANCED_FACE('',(#3448),#1609,.F.);
#32423=ADVANCED_FACE('',(#3449),#1610,.T.);
#32424=ADVANCED_FACE('',(#3450),#1611,.T.);
#32425=ADVANCED_FACE('',(#3451),#1612,.T.);
#32426=ADVANCED_FACE('',(#3452),#1613,.T.);
#32427=ADVANCED_FACE('',(#3453),#1614,.T.);
#32428=ADVANCED_FACE('',(#3454),#1615,.T.);
#32429=ADVANCED_FACE('',(#3455),#1616,.T.);
#32430=ADVANCED_FACE('',(#3456),#1617,.T.);
#32431=ADVANCED_FACE('',(#3457),#1618,.T.);
#32432=ADVANCED_FACE('',(#3458),#1619,.T.);
#32433=ADVANCED_FACE('',(#3459),#1620,.T.);
#32434=ADVANCED_FACE('',(#3460),#1621,.T.);
#32435=ADVANCED_FACE('',(#3461),#1622,.T.);
#32436=ADVANCED_FACE('',(#3462),#1623,.T.);
#32437=ADVANCED_FACE('',(#3463),#1624,.F.);
#32438=ADVANCED_FACE('',(#3464),#1625,.T.);
#32439=ADVANCED_FACE('',(#3465),#1626,.T.);
#32440=ADVANCED_FACE('',(#3466),#1627,.T.);
#32441=ADVANCED_FACE('',(#3467),#1628,.T.);
#32442=ADVANCED_FACE('',(#3468),#1629,.T.);
#32443=ADVANCED_FACE('',(#3469),#1630,.T.);
#32444=ADVANCED_FACE('',(#3470),#1631,.T.);
#32445=ADVANCED_FACE('',(#3471),#1632,.T.);
#32446=ADVANCED_FACE('',(#3472),#1633,.T.);
#32447=ADVANCED_FACE('',(#3473),#1634,.T.);
#32448=ADVANCED_FACE('',(#3474),#1635,.T.);
#32449=ADVANCED_FACE('',(#3475),#1636,.T.);
#32450=ADVANCED_FACE('',(#3476),#1637,.T.);
#32451=ADVANCED_FACE('',(#3477),#1638,.T.);
#32452=ADVANCED_FACE('',(#3478),#1639,.T.);
#32453=ADVANCED_FACE('',(#3479),#1640,.T.);
#32454=ADVANCED_FACE('',(#3480),#1641,.T.);
#32455=ADVANCED_FACE('',(#3481),#1642,.T.);
#32456=ADVANCED_FACE('',(#3482),#1643,.T.);
#32457=ADVANCED_FACE('',(#3483),#1644,.T.);
#32458=ADVANCED_FACE('',(#3484),#1645,.T.);
#32459=ADVANCED_FACE('',(#3485),#1646,.T.);
#32460=ADVANCED_FACE('',(#3486),#1647,.T.);
#32461=ADVANCED_FACE('',(#3487),#1648,.T.);
#32462=ADVANCED_FACE('',(#3488),#1649,.T.);
#32463=ADVANCED_FACE('',(#3489),#1650,.T.);
#32464=ADVANCED_FACE('',(#3490),#1651,.T.);
#32465=ADVANCED_FACE('',(#3491),#1652,.T.);
#32466=ADVANCED_FACE('',(#3492),#1653,.F.);
#32467=ADVANCED_FACE('',(#3493),#1654,.T.);
#32468=ADVANCED_FACE('',(#3494),#1655,.T.);
#32469=ADVANCED_FACE('',(#3495),#1656,.T.);
#32470=ADVANCED_FACE('',(#3496),#1657,.T.);
#32471=ADVANCED_FACE('',(#3497),#1658,.T.);
#32472=ADVANCED_FACE('',(#3498),#1659,.T.);
#32473=ADVANCED_FACE('',(#3499),#1660,.T.);
#32474=ADVANCED_FACE('',(#3500),#1661,.T.);
#32475=ADVANCED_FACE('',(#3501),#1662,.T.);
#32476=ADVANCED_FACE('',(#3502),#1663,.T.);
#32477=ADVANCED_FACE('',(#3503),#1664,.T.);
#32478=ADVANCED_FACE('',(#3504),#1665,.T.);
#32479=ADVANCED_FACE('',(#3505),#1666,.T.);
#32480=ADVANCED_FACE('',(#3506),#1667,.T.);
#32481=ADVANCED_FACE('',(#3507),#1668,.T.);
#32482=ADVANCED_FACE('',(#3508),#1669,.T.);
#32483=ADVANCED_FACE('',(#3509),#1670,.T.);
#32484=ADVANCED_FACE('',(#3510),#1671,.T.);
#32485=ADVANCED_FACE('',(#3511),#1672,.T.);
#32486=ADVANCED_FACE('',(#3512),#1673,.T.);
#32487=ADVANCED_FACE('',(#3513),#1674,.T.);
#32488=ADVANCED_FACE('',(#3514),#1675,.T.);
#32489=ADVANCED_FACE('',(#3515),#1676,.T.);
#32490=ADVANCED_FACE('',(#3516),#1677,.T.);
#32491=ADVANCED_FACE('',(#3517),#1678,.T.);
#32492=ADVANCED_FACE('',(#3518),#1679,.T.);
#32493=ADVANCED_FACE('',(#3519),#1680,.T.);
#32494=ADVANCED_FACE('',(#3520),#1681,.F.);
#32495=ADVANCED_FACE('',(#3521),#1682,.T.);
#32496=ADVANCED_FACE('',(#3522),#1683,.T.);
#32497=ADVANCED_FACE('',(#3523),#1684,.T.);
#32498=ADVANCED_FACE('',(#3524),#1685,.T.);
#32499=ADVANCED_FACE('',(#3525),#1686,.T.);
#32500=ADVANCED_FACE('',(#3526),#1687,.T.);
#32501=ADVANCED_FACE('',(#3527),#1688,.T.);
#32502=ADVANCED_FACE('',(#3528),#1689,.T.);
#32503=ADVANCED_FACE('',(#3529),#1690,.T.);
#32504=ADVANCED_FACE('',(#3530),#1691,.T.);
#32505=ADVANCED_FACE('',(#3531),#1692,.T.);
#32506=ADVANCED_FACE('',(#3532),#1693,.T.);
#32507=ADVANCED_FACE('',(#3533),#1694,.T.);
#32508=ADVANCED_FACE('',(#3534),#1695,.T.);
#32509=ADVANCED_FACE('',(#3535),#1696,.F.);
#32510=ADVANCED_FACE('',(#3536),#1697,.T.);
#32511=ADVANCED_FACE('',(#3537),#1698,.T.);
#32512=ADVANCED_FACE('',(#3538),#1699,.T.);
#32513=ADVANCED_FACE('',(#3539),#1700,.T.);
#32514=ADVANCED_FACE('',(#3540),#1701,.T.);
#32515=ADVANCED_FACE('',(#3541),#1702,.T.);
#32516=ADVANCED_FACE('',(#3542),#1703,.T.);
#32517=ADVANCED_FACE('',(#3543),#1704,.T.);
#32518=ADVANCED_FACE('',(#3544),#1705,.T.);
#32519=ADVANCED_FACE('',(#3545),#1706,.T.);
#32520=ADVANCED_FACE('',(#3546),#1707,.T.);
#32521=ADVANCED_FACE('',(#3547),#1708,.T.);
#32522=ADVANCED_FACE('',(#3548),#1709,.T.);
#32523=ADVANCED_FACE('',(#3549),#1710,.T.);
#32524=ADVANCED_FACE('',(#3550),#1711,.T.);
#32525=ADVANCED_FACE('',(#3551),#1712,.T.);
#32526=ADVANCED_FACE('',(#3552),#1713,.T.);
#32527=ADVANCED_FACE('',(#3553),#1714,.T.);
#32528=ADVANCED_FACE('',(#3554),#1715,.T.);
#32529=ADVANCED_FACE('',(#3555),#1716,.T.);
#32530=ADVANCED_FACE('',(#3556),#1717,.T.);
#32531=ADVANCED_FACE('',(#3557),#1718,.T.);
#32532=ADVANCED_FACE('',(#3558),#1719,.T.);
#32533=ADVANCED_FACE('',(#3559),#1720,.T.);
#32534=ADVANCED_FACE('',(#3560),#1721,.T.);
#32535=ADVANCED_FACE('',(#3561),#1722,.T.);
#32536=ADVANCED_FACE('',(#3562),#1723,.T.);
#32537=ADVANCED_FACE('',(#3563),#1724,.T.);
#32538=ADVANCED_FACE('',(#3564),#1725,.F.);
#32539=ADVANCED_FACE('',(#3565),#1726,.T.);
#32540=ADVANCED_FACE('',(#3566),#1727,.T.);
#32541=ADVANCED_FACE('',(#3567),#1728,.T.);
#32542=ADVANCED_FACE('',(#3568),#1729,.T.);
#32543=ADVANCED_FACE('',(#3569),#1730,.T.);
#32544=ADVANCED_FACE('',(#3570),#1731,.T.);
#32545=ADVANCED_FACE('',(#3571),#1732,.T.);
#32546=ADVANCED_FACE('',(#3572),#1733,.T.);
#32547=ADVANCED_FACE('',(#3573),#1734,.T.);
#32548=ADVANCED_FACE('',(#3574),#1735,.T.);
#32549=ADVANCED_FACE('',(#3575),#1736,.T.);
#32550=ADVANCED_FACE('',(#3576),#1737,.T.);
#32551=ADVANCED_FACE('',(#3577),#1738,.T.);
#32552=ADVANCED_FACE('',(#3578),#1739,.T.);
#32553=ADVANCED_FACE('',(#3579),#1740,.T.);
#32554=ADVANCED_FACE('',(#3580),#1741,.T.);
#32555=ADVANCED_FACE('',(#3581),#1742,.T.);
#32556=ADVANCED_FACE('',(#3582),#1743,.T.);
#32557=ADVANCED_FACE('',(#3583),#1744,.T.);
#32558=ADVANCED_FACE('',(#3584),#1745,.T.);
#32559=ADVANCED_FACE('',(#3585),#1746,.T.);
#32560=ADVANCED_FACE('',(#3586),#1747,.T.);
#32561=ADVANCED_FACE('',(#3587),#1748,.T.);
#32562=ADVANCED_FACE('',(#3588),#1749,.T.);
#32563=ADVANCED_FACE('',(#3589),#1750,.T.);
#32564=ADVANCED_FACE('',(#3590),#1751,.T.);
#32565=ADVANCED_FACE('',(#3591),#1752,.T.);
#32566=ADVANCED_FACE('',(#3592),#1753,.F.);
#32567=ADVANCED_FACE('',(#3593),#1754,.T.);
#32568=ADVANCED_FACE('',(#3594),#1755,.T.);
#32569=ADVANCED_FACE('',(#3595),#1756,.T.);
#32570=ADVANCED_FACE('',(#3596),#1757,.T.);
#32571=ADVANCED_FACE('',(#3597),#1758,.T.);
#32572=ADVANCED_FACE('',(#3598),#1759,.T.);
#32573=ADVANCED_FACE('',(#3599),#1760,.T.);
#32574=ADVANCED_FACE('',(#3600),#1761,.T.);
#32575=ADVANCED_FACE('',(#3601),#1762,.T.);
#32576=ADVANCED_FACE('',(#3602),#1763,.T.);
#32577=ADVANCED_FACE('',(#3603),#1764,.T.);
#32578=ADVANCED_FACE('',(#3604),#1765,.T.);
#32579=ADVANCED_FACE('',(#3605),#1766,.T.);
#32580=ADVANCED_FACE('',(#3606),#1767,.T.);
#32581=ADVANCED_FACE('',(#3607),#1768,.F.);
#32582=ADVANCED_FACE('',(#3608),#1769,.T.);
#32583=ADVANCED_FACE('',(#3609),#1770,.T.);
#32584=ADVANCED_FACE('',(#3610),#1771,.T.);
#32585=ADVANCED_FACE('',(#3611),#1772,.T.);
#32586=ADVANCED_FACE('',(#3612),#1773,.T.);
#32587=ADVANCED_FACE('',(#3613),#1774,.T.);
#32588=ADVANCED_FACE('',(#3614),#1775,.T.);
#32589=ADVANCED_FACE('',(#3615),#1776,.T.);
#32590=ADVANCED_FACE('',(#3616),#1777,.T.);
#32591=ADVANCED_FACE('',(#3617),#1778,.T.);
#32592=ADVANCED_FACE('',(#3618),#1779,.T.);
#32593=ADVANCED_FACE('',(#3619),#1780,.T.);
#32594=ADVANCED_FACE('',(#3620),#1781,.T.);
#32595=ADVANCED_FACE('',(#3621),#1782,.T.);
#32596=ADVANCED_FACE('',(#3622),#1783,.T.);
#32597=ADVANCED_FACE('',(#3623),#1784,.T.);
#32598=ADVANCED_FACE('',(#3624),#1785,.T.);
#32599=ADVANCED_FACE('',(#3625),#1786,.T.);
#32600=ADVANCED_FACE('',(#3626),#1787,.T.);
#32601=ADVANCED_FACE('',(#3627),#1788,.T.);
#32602=ADVANCED_FACE('',(#3628),#1789,.T.);
#32603=ADVANCED_FACE('',(#3629),#1790,.T.);
#32604=ADVANCED_FACE('',(#3630),#1791,.T.);
#32605=ADVANCED_FACE('',(#3631),#1792,.T.);
#32606=ADVANCED_FACE('',(#3632),#1793,.T.);
#32607=ADVANCED_FACE('',(#3633),#1794,.T.);
#32608=ADVANCED_FACE('',(#3634),#1795,.T.);
#32609=ADVANCED_FACE('',(#3635),#1796,.T.);
#32610=ADVANCED_FACE('',(#3636),#1797,.F.);
#32611=ADVANCED_FACE('',(#3637),#1798,.T.);
#32612=ADVANCED_FACE('',(#3638),#1799,.T.);
#32613=ADVANCED_FACE('',(#3639),#1800,.T.);
#32614=ADVANCED_FACE('',(#3640),#1801,.T.);
#32615=ADVANCED_FACE('',(#3641),#1802,.T.);
#32616=ADVANCED_FACE('',(#3642),#1803,.T.);
#32617=ADVANCED_FACE('',(#3643),#1804,.T.);
#32618=ADVANCED_FACE('',(#3644),#1805,.T.);
#32619=ADVANCED_FACE('',(#3645),#1806,.T.);
#32620=ADVANCED_FACE('',(#3646),#1807,.T.);
#32621=ADVANCED_FACE('',(#3647),#1808,.T.);
#32622=ADVANCED_FACE('',(#3648),#1809,.T.);
#32623=ADVANCED_FACE('',(#3649),#1810,.T.);
#32624=ADVANCED_FACE('',(#3650),#1811,.T.);
#32625=ADVANCED_FACE('',(#3651),#1812,.T.);
#32626=ADVANCED_FACE('',(#3652),#1813,.T.);
#32627=ADVANCED_FACE('',(#3653),#1814,.T.);
#32628=ADVANCED_FACE('',(#3654),#1815,.T.);
#32629=ADVANCED_FACE('',(#3655),#1816,.T.);
#32630=ADVANCED_FACE('',(#3656),#1817,.T.);
#32631=ADVANCED_FACE('',(#3657),#1818,.T.);
#32632=ADVANCED_FACE('',(#3658),#1819,.T.);
#32633=ADVANCED_FACE('',(#3659),#1820,.T.);
#32634=ADVANCED_FACE('',(#3660),#1821,.T.);
#32635=ADVANCED_FACE('',(#3661),#1822,.T.);
#32636=ADVANCED_FACE('',(#3662),#1823,.T.);
#32637=ADVANCED_FACE('',(#3663),#1824,.T.);
#32638=ADVANCED_FACE('',(#3664),#1825,.F.);
#32639=ADVANCED_FACE('',(#3665),#1826,.T.);
#32640=ADVANCED_FACE('',(#3666),#1827,.T.);
#32641=ADVANCED_FACE('',(#3667),#1828,.T.);
#32642=ADVANCED_FACE('',(#3668),#1829,.T.);
#32643=ADVANCED_FACE('',(#3669),#1830,.T.);
#32644=ADVANCED_FACE('',(#3670),#1831,.T.);
#32645=ADVANCED_FACE('',(#3671),#1832,.T.);
#32646=ADVANCED_FACE('',(#3672),#1833,.T.);
#32647=ADVANCED_FACE('',(#3673),#1834,.T.);
#32648=ADVANCED_FACE('',(#3674),#1835,.T.);
#32649=ADVANCED_FACE('',(#3675),#1836,.T.);
#32650=ADVANCED_FACE('',(#3676),#1837,.T.);
#32651=ADVANCED_FACE('',(#3677),#1838,.T.);
#32652=ADVANCED_FACE('',(#3678),#1839,.T.);
#32653=ADVANCED_FACE('',(#3679),#1840,.F.);
#32654=ADVANCED_FACE('',(#3680),#1841,.T.);
#32655=ADVANCED_FACE('',(#3681),#1842,.T.);
#32656=ADVANCED_FACE('',(#3682),#1843,.T.);
#32657=ADVANCED_FACE('',(#3683),#1844,.T.);
#32658=ADVANCED_FACE('',(#3684),#1845,.T.);
#32659=ADVANCED_FACE('',(#3685),#1846,.T.);
#32660=ADVANCED_FACE('',(#3686),#1847,.T.);
#32661=ADVANCED_FACE('',(#3687),#1848,.T.);
#32662=ADVANCED_FACE('',(#3688),#1849,.T.);
#32663=ADVANCED_FACE('',(#3689),#1850,.T.);
#32664=ADVANCED_FACE('',(#3690),#1851,.T.);
#32665=ADVANCED_FACE('',(#3691),#1852,.T.);
#32666=ADVANCED_FACE('',(#3692),#1853,.T.);
#32667=ADVANCED_FACE('',(#3693),#1854,.T.);
#32668=ADVANCED_FACE('',(#3694),#1855,.T.);
#32669=ADVANCED_FACE('',(#3695),#1856,.T.);
#32670=ADVANCED_FACE('',(#3696),#1857,.T.);
#32671=ADVANCED_FACE('',(#3697),#1858,.T.);
#32672=ADVANCED_FACE('',(#3698),#1859,.T.);
#32673=ADVANCED_FACE('',(#3699),#1860,.T.);
#32674=ADVANCED_FACE('',(#3700),#1861,.T.);
#32675=ADVANCED_FACE('',(#3701),#1862,.T.);
#32676=ADVANCED_FACE('',(#3702),#1863,.T.);
#32677=ADVANCED_FACE('',(#3703),#1864,.T.);
#32678=ADVANCED_FACE('',(#3704),#1865,.T.);
#32679=ADVANCED_FACE('',(#3705),#1866,.T.);
#32680=ADVANCED_FACE('',(#3706),#1867,.T.);
#32681=ADVANCED_FACE('',(#3707),#1868,.T.);
#32682=ADVANCED_FACE('',(#3708),#1869,.F.);
#32683=ADVANCED_FACE('',(#3709),#1870,.T.);
#32684=ADVANCED_FACE('',(#3710),#1871,.T.);
#32685=ADVANCED_FACE('',(#3711),#1872,.T.);
#32686=ADVANCED_FACE('',(#3712),#1873,.T.);
#32687=ADVANCED_FACE('',(#3713),#1874,.T.);
#32688=ADVANCED_FACE('',(#3714),#1875,.T.);
#32689=ADVANCED_FACE('',(#3715),#1876,.T.);
#32690=ADVANCED_FACE('',(#3716),#1877,.T.);
#32691=ADVANCED_FACE('',(#3717),#1878,.T.);
#32692=ADVANCED_FACE('',(#3718),#1879,.T.);
#32693=ADVANCED_FACE('',(#3719),#1880,.T.);
#32694=ADVANCED_FACE('',(#3720),#1881,.T.);
#32695=ADVANCED_FACE('',(#3721),#1882,.T.);
#32696=ADVANCED_FACE('',(#3722),#1883,.T.);
#32697=ADVANCED_FACE('',(#3723),#1884,.T.);
#32698=ADVANCED_FACE('',(#3724),#1885,.T.);
#32699=ADVANCED_FACE('',(#3725),#1886,.T.);
#32700=ADVANCED_FACE('',(#3726),#1887,.T.);
#32701=ADVANCED_FACE('',(#3727),#1888,.T.);
#32702=ADVANCED_FACE('',(#3728),#1889,.T.);
#32703=ADVANCED_FACE('',(#3729),#1890,.T.);
#32704=ADVANCED_FACE('',(#3730),#1891,.T.);
#32705=ADVANCED_FACE('',(#3731),#1892,.T.);
#32706=ADVANCED_FACE('',(#3732),#1893,.T.);
#32707=ADVANCED_FACE('',(#3733),#1894,.T.);
#32708=ADVANCED_FACE('',(#3734),#1895,.T.);
#32709=ADVANCED_FACE('',(#3735),#1896,.T.);
#32710=ADVANCED_FACE('',(#3736),#1897,.F.);
#32711=ADVANCED_FACE('',(#3737),#1898,.T.);
#32712=ADVANCED_FACE('',(#3738),#1899,.T.);
#32713=ADVANCED_FACE('',(#3739),#1900,.T.);
#32714=ADVANCED_FACE('',(#3740),#1901,.T.);
#32715=ADVANCED_FACE('',(#3741),#1902,.T.);
#32716=ADVANCED_FACE('',(#3742),#1903,.T.);
#32717=ADVANCED_FACE('',(#3743),#1904,.T.);
#32718=ADVANCED_FACE('',(#3744),#1905,.T.);
#32719=ADVANCED_FACE('',(#3745),#1906,.T.);
#32720=ADVANCED_FACE('',(#3746),#1907,.T.);
#32721=ADVANCED_FACE('',(#3747),#1908,.T.);
#32722=ADVANCED_FACE('',(#3748),#1909,.T.);
#32723=ADVANCED_FACE('',(#3749),#1910,.T.);
#32724=ADVANCED_FACE('',(#3750),#1911,.T.);
#32725=ADVANCED_FACE('',(#3751),#1912,.F.);
#32726=ADVANCED_FACE('',(#3752),#1913,.T.);
#32727=ADVANCED_FACE('',(#3753),#1914,.T.);
#32728=ADVANCED_FACE('',(#3754),#1915,.T.);
#32729=ADVANCED_FACE('',(#3755),#1916,.T.);
#32730=ADVANCED_FACE('',(#3756),#1917,.T.);
#32731=ADVANCED_FACE('',(#3757),#1918,.T.);
#32732=ADVANCED_FACE('',(#3758),#1919,.T.);
#32733=ADVANCED_FACE('',(#3759),#1920,.T.);
#32734=ADVANCED_FACE('',(#3760),#1921,.T.);
#32735=ADVANCED_FACE('',(#3761),#1922,.T.);
#32736=ADVANCED_FACE('',(#3762),#1923,.T.);
#32737=ADVANCED_FACE('',(#3763),#1924,.T.);
#32738=ADVANCED_FACE('',(#3764),#1925,.T.);
#32739=ADVANCED_FACE('',(#3765),#1926,.T.);
#32740=ADVANCED_FACE('',(#3766),#1927,.T.);
#32741=ADVANCED_FACE('',(#3767),#1928,.T.);
#32742=ADVANCED_FACE('',(#3768),#1929,.T.);
#32743=ADVANCED_FACE('',(#3769),#1930,.T.);
#32744=ADVANCED_FACE('',(#3770),#1931,.T.);
#32745=ADVANCED_FACE('',(#3771),#1932,.T.);
#32746=ADVANCED_FACE('',(#3772),#1933,.T.);
#32747=ADVANCED_FACE('',(#3773),#1934,.T.);
#32748=ADVANCED_FACE('',(#3774),#1935,.T.);
#32749=ADVANCED_FACE('',(#3775),#1936,.T.);
#32750=ADVANCED_FACE('',(#3776),#1937,.T.);
#32751=ADVANCED_FACE('',(#3777),#1938,.T.);
#32752=ADVANCED_FACE('',(#3778),#1939,.T.);
#32753=ADVANCED_FACE('',(#3779),#1940,.T.);
#32754=ADVANCED_FACE('',(#3780),#1941,.F.);
#32755=ADVANCED_FACE('',(#3781),#1942,.T.);
#32756=ADVANCED_FACE('',(#3782),#1943,.T.);
#32757=ADVANCED_FACE('',(#3783),#1944,.T.);
#32758=ADVANCED_FACE('',(#3784),#1945,.T.);
#32759=ADVANCED_FACE('',(#3785),#1946,.T.);
#32760=ADVANCED_FACE('',(#3786),#1947,.T.);
#32761=ADVANCED_FACE('',(#3787),#1948,.T.);
#32762=ADVANCED_FACE('',(#3788),#1949,.T.);
#32763=ADVANCED_FACE('',(#3789),#1950,.T.);
#32764=ADVANCED_FACE('',(#3790),#1951,.T.);
#32765=ADVANCED_FACE('',(#3791),#1952,.T.);
#32766=ADVANCED_FACE('',(#3792),#1953,.T.);
#32767=ADVANCED_FACE('',(#3793),#1954,.T.);
#32768=ADVANCED_FACE('',(#3794),#1955,.T.);
#32769=ADVANCED_FACE('',(#3795),#1956,.T.);
#32770=ADVANCED_FACE('',(#3796),#1957,.T.);
#32771=ADVANCED_FACE('',(#3797),#1958,.T.);
#32772=ADVANCED_FACE('',(#3798),#1959,.T.);
#32773=ADVANCED_FACE('',(#3799),#1960,.T.);
#32774=ADVANCED_FACE('',(#3800),#1961,.T.);
#32775=ADVANCED_FACE('',(#3801),#1962,.T.);
#32776=ADVANCED_FACE('',(#3802),#1963,.T.);
#32777=ADVANCED_FACE('',(#3803),#1964,.T.);
#32778=ADVANCED_FACE('',(#3804),#1965,.T.);
#32779=ADVANCED_FACE('',(#3805),#1966,.T.);
#32780=ADVANCED_FACE('',(#3806),#1967,.T.);
#32781=ADVANCED_FACE('',(#3807),#1968,.T.);
#32782=ADVANCED_FACE('',(#3808),#1969,.F.);
#32783=ADVANCED_FACE('',(#3809),#1970,.T.);
#32784=ADVANCED_FACE('',(#3810),#1971,.T.);
#32785=ADVANCED_FACE('',(#3811),#1972,.T.);
#32786=ADVANCED_FACE('',(#3812),#1973,.T.);
#32787=ADVANCED_FACE('',(#3813),#1974,.T.);
#32788=ADVANCED_FACE('',(#3814),#1975,.T.);
#32789=ADVANCED_FACE('',(#3815),#1976,.T.);
#32790=ADVANCED_FACE('',(#3816),#1977,.T.);
#32791=ADVANCED_FACE('',(#3817),#1978,.T.);
#32792=ADVANCED_FACE('',(#3818),#1979,.T.);
#32793=ADVANCED_FACE('',(#3819),#1980,.T.);
#32794=ADVANCED_FACE('',(#3820),#1981,.T.);
#32795=ADVANCED_FACE('',(#3821),#1982,.T.);
#32796=ADVANCED_FACE('',(#3822),#1983,.T.);
#32797=ADVANCED_FACE('',(#3823),#1984,.F.);
#32798=ADVANCED_FACE('',(#3824),#1985,.T.);
#32799=ADVANCED_FACE('',(#3825),#1986,.T.);
#32800=ADVANCED_FACE('',(#3826),#1987,.T.);
#32801=ADVANCED_FACE('',(#3827),#1988,.T.);
#32802=ADVANCED_FACE('',(#3828),#1989,.T.);
#32803=ADVANCED_FACE('',(#3829),#1990,.T.);
#32804=ADVANCED_FACE('',(#3830),#1991,.T.);
#32805=ADVANCED_FACE('',(#3831),#1992,.T.);
#32806=ADVANCED_FACE('',(#3832),#1993,.T.);
#32807=ADVANCED_FACE('',(#3833),#1994,.T.);
#32808=ADVANCED_FACE('',(#3834),#1995,.T.);
#32809=ADVANCED_FACE('',(#3835),#1996,.T.);
#32810=ADVANCED_FACE('',(#3836),#1997,.T.);
#32811=ADVANCED_FACE('',(#3837),#1998,.T.);
#32812=ADVANCED_FACE('',(#3838),#1999,.T.);
#32813=ADVANCED_FACE('',(#3839),#2000,.T.);
#32814=ADVANCED_FACE('',(#3840),#2001,.T.);
#32815=ADVANCED_FACE('',(#3841),#2002,.T.);
#32816=ADVANCED_FACE('',(#3842),#2003,.T.);
#32817=ADVANCED_FACE('',(#3843),#2004,.T.);
#32818=ADVANCED_FACE('',(#3844),#2005,.T.);
#32819=ADVANCED_FACE('',(#3845),#2006,.T.);
#32820=ADVANCED_FACE('',(#3846),#2007,.T.);
#32821=ADVANCED_FACE('',(#3847),#2008,.T.);
#32822=ADVANCED_FACE('',(#3848),#2009,.T.);
#32823=ADVANCED_FACE('',(#3849),#2010,.T.);
#32824=ADVANCED_FACE('',(#3850),#2011,.T.);
#32825=ADVANCED_FACE('',(#3851),#2012,.T.);
#32826=ADVANCED_FACE('',(#3852),#2013,.F.);
#32827=ADVANCED_FACE('',(#3853),#2014,.T.);
#32828=ADVANCED_FACE('',(#3854),#2015,.T.);
#32829=ADVANCED_FACE('',(#3855),#2016,.T.);
#32830=ADVANCED_FACE('',(#3856),#2017,.T.);
#32831=ADVANCED_FACE('',(#3857),#2018,.T.);
#32832=ADVANCED_FACE('',(#3858),#2019,.T.);
#32833=ADVANCED_FACE('',(#3859),#2020,.T.);
#32834=ADVANCED_FACE('',(#3860),#2021,.T.);
#32835=ADVANCED_FACE('',(#3861),#2022,.T.);
#32836=ADVANCED_FACE('',(#3862),#2023,.T.);
#32837=ADVANCED_FACE('',(#3863),#2024,.T.);
#32838=ADVANCED_FACE('',(#3864),#2025,.T.);
#32839=ADVANCED_FACE('',(#3865),#2026,.T.);
#32840=ADVANCED_FACE('',(#3866),#2027,.T.);
#32841=ADVANCED_FACE('',(#3867),#2028,.T.);
#32842=ADVANCED_FACE('',(#3868),#2029,.T.);
#32843=ADVANCED_FACE('',(#3869),#2030,.T.);
#32844=ADVANCED_FACE('',(#3870),#2031,.T.);
#32845=ADVANCED_FACE('',(#3871),#2032,.T.);
#32846=ADVANCED_FACE('',(#3872),#2033,.T.);
#32847=ADVANCED_FACE('',(#3873),#2034,.T.);
#32848=ADVANCED_FACE('',(#3874),#2035,.T.);
#32849=ADVANCED_FACE('',(#3875),#2036,.T.);
#32850=ADVANCED_FACE('',(#3876),#2037,.T.);
#32851=ADVANCED_FACE('',(#3877),#2038,.T.);
#32852=ADVANCED_FACE('',(#3878),#2039,.T.);
#32853=ADVANCED_FACE('',(#3879),#2040,.T.);
#32854=ADVANCED_FACE('',(#3880),#2041,.F.);
#32855=ADVANCED_FACE('',(#3881),#2042,.T.);
#32856=ADVANCED_FACE('',(#3882),#2043,.T.);
#32857=ADVANCED_FACE('',(#3883),#2044,.T.);
#32858=ADVANCED_FACE('',(#3884),#2045,.T.);
#32859=ADVANCED_FACE('',(#3885),#2046,.T.);
#32860=ADVANCED_FACE('',(#3886),#2047,.T.);
#32861=ADVANCED_FACE('',(#3887),#2048,.T.);
#32862=ADVANCED_FACE('',(#3888),#2049,.T.);
#32863=ADVANCED_FACE('',(#3889),#2050,.T.);
#32864=ADVANCED_FACE('',(#3890),#2051,.T.);
#32865=ADVANCED_FACE('',(#3891),#2052,.T.);
#32866=ADVANCED_FACE('',(#3892),#2053,.T.);
#32867=ADVANCED_FACE('',(#3893),#2054,.T.);
#32868=ADVANCED_FACE('',(#3894),#2055,.T.);
#32869=ADVANCED_FACE('',(#3895),#2056,.F.);
#32870=ADVANCED_FACE('',(#3896),#2057,.T.);
#32871=ADVANCED_FACE('',(#3897),#2058,.T.);
#32872=ADVANCED_FACE('',(#3898),#2059,.T.);
#32873=ADVANCED_FACE('',(#3899),#2060,.T.);
#32874=ADVANCED_FACE('',(#3900),#2061,.T.);
#32875=ADVANCED_FACE('',(#3901),#2062,.T.);
#32876=ADVANCED_FACE('',(#3902),#2063,.T.);
#32877=ADVANCED_FACE('',(#3903),#2064,.T.);
#32878=ADVANCED_FACE('',(#3904),#2065,.T.);
#32879=ADVANCED_FACE('',(#3905),#2066,.T.);
#32880=ADVANCED_FACE('',(#3906),#2067,.T.);
#32881=ADVANCED_FACE('',(#3907),#2068,.T.);
#32882=ADVANCED_FACE('',(#3908),#2069,.T.);
#32883=ADVANCED_FACE('',(#3909),#2070,.T.);
#32884=ADVANCED_FACE('',(#3910),#2071,.T.);
#32885=ADVANCED_FACE('',(#3911),#2072,.T.);
#32886=ADVANCED_FACE('',(#3912),#2073,.T.);
#32887=ADVANCED_FACE('',(#3913),#2074,.T.);
#32888=ADVANCED_FACE('',(#3914),#2075,.T.);
#32889=ADVANCED_FACE('',(#3915),#2076,.T.);
#32890=ADVANCED_FACE('',(#3916),#2077,.T.);
#32891=ADVANCED_FACE('',(#3917),#2078,.T.);
#32892=ADVANCED_FACE('',(#3918),#2079,.T.);
#32893=ADVANCED_FACE('',(#3919),#2080,.T.);
#32894=ADVANCED_FACE('',(#3920),#2081,.T.);
#32895=ADVANCED_FACE('',(#3921),#2082,.T.);
#32896=ADVANCED_FACE('',(#3922),#2083,.T.);
#32897=ADVANCED_FACE('',(#3923),#2084,.T.);
#32898=ADVANCED_FACE('',(#3924),#2085,.F.);
#32899=ADVANCED_FACE('',(#3925),#2086,.T.);
#32900=ADVANCED_FACE('',(#3926),#2087,.T.);
#32901=ADVANCED_FACE('',(#3927),#2088,.T.);
#32902=ADVANCED_FACE('',(#3928),#2089,.T.);
#32903=ADVANCED_FACE('',(#3929),#2090,.T.);
#32904=ADVANCED_FACE('',(#3930),#2091,.T.);
#32905=ADVANCED_FACE('',(#3931),#2092,.T.);
#32906=ADVANCED_FACE('',(#3932),#2093,.T.);
#32907=ADVANCED_FACE('',(#3933),#2094,.T.);
#32908=ADVANCED_FACE('',(#3934),#2095,.T.);
#32909=ADVANCED_FACE('',(#3935),#2096,.T.);
#32910=ADVANCED_FACE('',(#3936),#2097,.T.);
#32911=ADVANCED_FACE('',(#3937),#2098,.T.);
#32912=ADVANCED_FACE('',(#3938),#2099,.T.);
#32913=ADVANCED_FACE('',(#3939),#2100,.T.);
#32914=ADVANCED_FACE('',(#3940),#2101,.T.);
#32915=ADVANCED_FACE('',(#3941),#2102,.T.);
#32916=ADVANCED_FACE('',(#3942),#2103,.T.);
#32917=ADVANCED_FACE('',(#3943),#2104,.T.);
#32918=ADVANCED_FACE('',(#3944),#2105,.T.);
#32919=ADVANCED_FACE('',(#3945),#2106,.T.);
#32920=ADVANCED_FACE('',(#3946),#2107,.T.);
#32921=ADVANCED_FACE('',(#3947),#2108,.T.);
#32922=ADVANCED_FACE('',(#3948),#2109,.T.);
#32923=ADVANCED_FACE('',(#3949),#2110,.T.);
#32924=ADVANCED_FACE('',(#3950),#2111,.T.);
#32925=ADVANCED_FACE('',(#3951),#2112,.T.);
#32926=ADVANCED_FACE('',(#3952),#2113,.F.);
#32927=ADVANCED_FACE('',(#3953),#2114,.T.);
#32928=ADVANCED_FACE('',(#3954),#2115,.T.);
#32929=ADVANCED_FACE('',(#3955),#2116,.T.);
#32930=ADVANCED_FACE('',(#3956),#2117,.T.);
#32931=ADVANCED_FACE('',(#3957),#2118,.T.);
#32932=ADVANCED_FACE('',(#3958),#2119,.T.);
#32933=ADVANCED_FACE('',(#3959),#2120,.T.);
#32934=ADVANCED_FACE('',(#3960),#2121,.T.);
#32935=ADVANCED_FACE('',(#3961),#2122,.T.);
#32936=ADVANCED_FACE('',(#3962),#2123,.T.);
#32937=ADVANCED_FACE('',(#3963),#2124,.T.);
#32938=ADVANCED_FACE('',(#3964),#2125,.T.);
#32939=ADVANCED_FACE('',(#3965),#2126,.T.);
#32940=ADVANCED_FACE('',(#3966),#2127,.T.);
#32941=ADVANCED_FACE('',(#3967),#2128,.F.);
#32942=ADVANCED_FACE('',(#3968),#2129,.T.);
#32943=ADVANCED_FACE('',(#3969),#2130,.T.);
#32944=ADVANCED_FACE('',(#3970),#2131,.T.);
#32945=ADVANCED_FACE('',(#3971),#2132,.T.);
#32946=ADVANCED_FACE('',(#3972),#2133,.T.);
#32947=ADVANCED_FACE('',(#3973),#2134,.T.);
#32948=ADVANCED_FACE('',(#3974),#2135,.T.);
#32949=ADVANCED_FACE('',(#3975),#2136,.T.);
#32950=ADVANCED_FACE('',(#3976),#2137,.T.);
#32951=ADVANCED_FACE('',(#3977),#2138,.T.);
#32952=ADVANCED_FACE('',(#3978),#2139,.T.);
#32953=ADVANCED_FACE('',(#3979),#2140,.T.);
#32954=ADVANCED_FACE('',(#3980),#2141,.T.);
#32955=ADVANCED_FACE('',(#3981),#2142,.T.);
#32956=ADVANCED_FACE('',(#3982),#2143,.T.);
#32957=ADVANCED_FACE('',(#3983),#2144,.T.);
#32958=ADVANCED_FACE('',(#3984),#2145,.T.);
#32959=ADVANCED_FACE('',(#3985),#2146,.T.);
#32960=ADVANCED_FACE('',(#3986),#2147,.T.);
#32961=ADVANCED_FACE('',(#3987),#2148,.T.);
#32962=ADVANCED_FACE('',(#3988),#2149,.T.);
#32963=ADVANCED_FACE('',(#3989),#2150,.T.);
#32964=ADVANCED_FACE('',(#3990),#2151,.T.);
#32965=ADVANCED_FACE('',(#3991),#2152,.T.);
#32966=ADVANCED_FACE('',(#3992),#2153,.T.);
#32967=ADVANCED_FACE('',(#3993),#2154,.T.);
#32968=ADVANCED_FACE('',(#3994),#2155,.T.);
#32969=ADVANCED_FACE('',(#3995),#2156,.T.);
#32970=ADVANCED_FACE('',(#3996),#2157,.F.);
#32971=ADVANCED_FACE('',(#3997),#2158,.T.);
#32972=ADVANCED_FACE('',(#3998),#2159,.T.);
#32973=ADVANCED_FACE('',(#3999),#2160,.T.);
#32974=ADVANCED_FACE('',(#4000),#2161,.T.);
#32975=ADVANCED_FACE('',(#4001),#2162,.T.);
#32976=ADVANCED_FACE('',(#4002),#2163,.T.);
#32977=ADVANCED_FACE('',(#4003),#2164,.T.);
#32978=ADVANCED_FACE('',(#4004),#2165,.T.);
#32979=ADVANCED_FACE('',(#4005),#2166,.T.);
#32980=ADVANCED_FACE('',(#4006),#2167,.T.);
#32981=ADVANCED_FACE('',(#4007),#2168,.T.);
#32982=ADVANCED_FACE('',(#4008),#2169,.T.);
#32983=ADVANCED_FACE('',(#4009),#2170,.T.);
#32984=ADVANCED_FACE('',(#4010),#2171,.T.);
#32985=ADVANCED_FACE('',(#4011),#2172,.T.);
#32986=ADVANCED_FACE('',(#4012),#2173,.T.);
#32987=ADVANCED_FACE('',(#4013),#2174,.T.);
#32988=ADVANCED_FACE('',(#4014),#2175,.T.);
#32989=ADVANCED_FACE('',(#4015),#2176,.T.);
#32990=ADVANCED_FACE('',(#4016),#2177,.T.);
#32991=ADVANCED_FACE('',(#4017),#2178,.T.);
#32992=ADVANCED_FACE('',(#4018),#2179,.T.);
#32993=ADVANCED_FACE('',(#4019),#2180,.T.);
#32994=ADVANCED_FACE('',(#4020),#2181,.T.);
#32995=ADVANCED_FACE('',(#4021),#2182,.T.);
#32996=ADVANCED_FACE('',(#4022),#2183,.T.);
#32997=ADVANCED_FACE('',(#4023),#2184,.T.);
#32998=ADVANCED_FACE('',(#4024),#2185,.F.);
#32999=ADVANCED_FACE('',(#4025),#2186,.T.);
#33000=ADVANCED_FACE('',(#4026),#2187,.T.);
#33001=ADVANCED_FACE('',(#4027),#2188,.T.);
#33002=ADVANCED_FACE('',(#4028),#2189,.T.);
#33003=ADVANCED_FACE('',(#4029),#2190,.T.);
#33004=ADVANCED_FACE('',(#4030),#2191,.T.);
#33005=ADVANCED_FACE('',(#4031),#2192,.T.);
#33006=ADVANCED_FACE('',(#4032),#2193,.T.);
#33007=ADVANCED_FACE('',(#4033),#2194,.T.);
#33008=ADVANCED_FACE('',(#4034),#2195,.T.);
#33009=ADVANCED_FACE('',(#4035),#2196,.T.);
#33010=ADVANCED_FACE('',(#4036),#2197,.T.);
#33011=ADVANCED_FACE('',(#4037),#2198,.T.);
#33012=ADVANCED_FACE('',(#4038),#2199,.T.);
#33013=ADVANCED_FACE('',(#4039),#2200,.F.);
#33014=ADVANCED_FACE('',(#4040),#2201,.T.);
#33015=ADVANCED_FACE('',(#4041),#2202,.T.);
#33016=ADVANCED_FACE('',(#4042),#2203,.T.);
#33017=ADVANCED_FACE('',(#4043),#2204,.T.);
#33018=ADVANCED_FACE('',(#4044),#2205,.T.);
#33019=ADVANCED_FACE('',(#4045),#2206,.T.);
#33020=ADVANCED_FACE('',(#4046),#2207,.T.);
#33021=ADVANCED_FACE('',(#4047),#2208,.T.);
#33022=ADVANCED_FACE('',(#4048),#2209,.T.);
#33023=ADVANCED_FACE('',(#4049),#2210,.T.);
#33024=ADVANCED_FACE('',(#4050),#2211,.T.);
#33025=ADVANCED_FACE('',(#4051),#2212,.T.);
#33026=ADVANCED_FACE('',(#4052),#2213,.T.);
#33027=ADVANCED_FACE('',(#4053),#2214,.T.);
#33028=ADVANCED_FACE('',(#4054),#2215,.T.);
#33029=ADVANCED_FACE('',(#4055),#2216,.T.);
#33030=ADVANCED_FACE('',(#4056),#2217,.T.);
#33031=ADVANCED_FACE('',(#4057),#2218,.T.);
#33032=ADVANCED_FACE('',(#4058),#2219,.T.);
#33033=ADVANCED_FACE('',(#4059),#2220,.T.);
#33034=ADVANCED_FACE('',(#4060),#2221,.T.);
#33035=ADVANCED_FACE('',(#4061),#2222,.T.);
#33036=ADVANCED_FACE('',(#4062),#2223,.T.);
#33037=ADVANCED_FACE('',(#4063),#2224,.T.);
#33038=ADVANCED_FACE('',(#4064),#2225,.T.);
#33039=ADVANCED_FACE('',(#4065),#2226,.T.);
#33040=ADVANCED_FACE('',(#4066),#2227,.T.);
#33041=ADVANCED_FACE('',(#4067),#2228,.T.);
#33042=ADVANCED_FACE('',(#4068),#2229,.F.);
#33043=ADVANCED_FACE('',(#4069),#2230,.T.);
#33044=ADVANCED_FACE('',(#4070),#2231,.T.);
#33045=ADVANCED_FACE('',(#4071),#2232,.T.);
#33046=ADVANCED_FACE('',(#4072),#2233,.T.);
#33047=ADVANCED_FACE('',(#4073),#2234,.T.);
#33048=ADVANCED_FACE('',(#4074),#2235,.T.);
#33049=ADVANCED_FACE('',(#4075),#2236,.T.);
#33050=ADVANCED_FACE('',(#4076),#2237,.T.);
#33051=ADVANCED_FACE('',(#4077),#2238,.T.);
#33052=ADVANCED_FACE('',(#4078),#2239,.T.);
#33053=ADVANCED_FACE('',(#4079),#2240,.T.);
#33054=ADVANCED_FACE('',(#4080),#2241,.T.);
#33055=ADVANCED_FACE('',(#4081),#2242,.T.);
#33056=ADVANCED_FACE('',(#4082),#2243,.T.);
#33057=ADVANCED_FACE('',(#4083),#2244,.T.);
#33058=ADVANCED_FACE('',(#4084),#2245,.T.);
#33059=ADVANCED_FACE('',(#4085),#2246,.T.);
#33060=ADVANCED_FACE('',(#4086),#2247,.T.);
#33061=ADVANCED_FACE('',(#4087),#2248,.T.);
#33062=ADVANCED_FACE('',(#4088),#2249,.T.);
#33063=ADVANCED_FACE('',(#4089),#2250,.T.);
#33064=ADVANCED_FACE('',(#4090),#2251,.T.);
#33065=ADVANCED_FACE('',(#4091),#2252,.T.);
#33066=ADVANCED_FACE('',(#4092),#2253,.T.);
#33067=ADVANCED_FACE('',(#4093),#2254,.T.);
#33068=ADVANCED_FACE('',(#4094),#2255,.T.);
#33069=ADVANCED_FACE('',(#4095),#2256,.T.);
#33070=ADVANCED_FACE('',(#4096),#2257,.F.);
#33071=ADVANCED_FACE('',(#4097),#2258,.T.);
#33072=ADVANCED_FACE('',(#4098),#2259,.T.);
#33073=ADVANCED_FACE('',(#4099),#2260,.T.);
#33074=ADVANCED_FACE('',(#4100),#2261,.T.);
#33075=ADVANCED_FACE('',(#4101),#2262,.T.);
#33076=ADVANCED_FACE('',(#4102),#2263,.T.);
#33077=ADVANCED_FACE('',(#4103),#2264,.T.);
#33078=ADVANCED_FACE('',(#4104),#2265,.T.);
#33079=ADVANCED_FACE('',(#4105),#2266,.T.);
#33080=ADVANCED_FACE('',(#4106),#2267,.T.);
#33081=ADVANCED_FACE('',(#4107),#2268,.T.);
#33082=ADVANCED_FACE('',(#4108),#2269,.T.);
#33083=ADVANCED_FACE('',(#4109),#2270,.T.);
#33084=ADVANCED_FACE('',(#4110),#2271,.T.);
#33085=ADVANCED_FACE('',(#4111),#2272,.F.);
#33086=ADVANCED_FACE('',(#4112),#2273,.T.);
#33087=ADVANCED_FACE('',(#4113),#2274,.T.);
#33088=ADVANCED_FACE('',(#4114),#2275,.T.);
#33089=ADVANCED_FACE('',(#4115),#2276,.T.);
#33090=ADVANCED_FACE('',(#4116),#2277,.T.);
#33091=ADVANCED_FACE('',(#4117),#2278,.T.);
#33092=ADVANCED_FACE('',(#4118),#2279,.T.);
#33093=ADVANCED_FACE('',(#4119),#2280,.T.);
#33094=ADVANCED_FACE('',(#4120),#2281,.T.);
#33095=ADVANCED_FACE('',(#4121),#2282,.T.);
#33096=ADVANCED_FACE('',(#4122),#2283,.T.);
#33097=ADVANCED_FACE('',(#4123),#2284,.T.);
#33098=ADVANCED_FACE('',(#4124),#2285,.T.);
#33099=ADVANCED_FACE('',(#4125),#2286,.T.);
#33100=ADVANCED_FACE('',(#4126),#2287,.T.);
#33101=ADVANCED_FACE('',(#4127),#2288,.T.);
#33102=ADVANCED_FACE('',(#4128),#2289,.T.);
#33103=ADVANCED_FACE('',(#4129),#2290,.T.);
#33104=ADVANCED_FACE('',(#4130),#2291,.T.);
#33105=ADVANCED_FACE('',(#4131),#2292,.T.);
#33106=ADVANCED_FACE('',(#4132),#2293,.T.);
#33107=ADVANCED_FACE('',(#4133),#2294,.T.);
#33108=ADVANCED_FACE('',(#4134),#2295,.T.);
#33109=ADVANCED_FACE('',(#4135),#2296,.T.);
#33110=ADVANCED_FACE('',(#4136),#2297,.T.);
#33111=ADVANCED_FACE('',(#4137),#2298,.T.);
#33112=ADVANCED_FACE('',(#4138),#2299,.T.);
#33113=ADVANCED_FACE('',(#4139),#2300,.T.);
#33114=ADVANCED_FACE('',(#4140),#2301,.F.);
#33115=ADVANCED_FACE('',(#4141),#2302,.T.);
#33116=ADVANCED_FACE('',(#4142),#2303,.T.);
#33117=ADVANCED_FACE('',(#4143),#2304,.T.);
#33118=ADVANCED_FACE('',(#4144),#2305,.T.);
#33119=ADVANCED_FACE('',(#4145),#2306,.T.);
#33120=ADVANCED_FACE('',(#4146),#2307,.T.);
#33121=ADVANCED_FACE('',(#4147),#2308,.T.);
#33122=ADVANCED_FACE('',(#4148),#2309,.T.);
#33123=ADVANCED_FACE('',(#4149),#2310,.T.);
#33124=ADVANCED_FACE('',(#4150),#2311,.T.);
#33125=ADVANCED_FACE('',(#4151),#2312,.T.);
#33126=ADVANCED_FACE('',(#4152),#2313,.T.);
#33127=ADVANCED_FACE('',(#4153),#2314,.T.);
#33128=ADVANCED_FACE('',(#4154),#2315,.T.);
#33129=ADVANCED_FACE('',(#4155),#2316,.T.);
#33130=ADVANCED_FACE('',(#4156),#2317,.T.);
#33131=ADVANCED_FACE('',(#4157),#2318,.T.);
#33132=ADVANCED_FACE('',(#4158),#2319,.T.);
#33133=ADVANCED_FACE('',(#4159),#2320,.T.);
#33134=ADVANCED_FACE('',(#4160),#2321,.T.);
#33135=ADVANCED_FACE('',(#4161),#2322,.T.);
#33136=ADVANCED_FACE('',(#4162),#2323,.T.);
#33137=ADVANCED_FACE('',(#4163),#2324,.T.);
#33138=ADVANCED_FACE('',(#4164),#2325,.T.);
#33139=ADVANCED_FACE('',(#4165),#2326,.T.);
#33140=ADVANCED_FACE('',(#4166),#2327,.T.);
#33141=ADVANCED_FACE('',(#4167),#2328,.T.);
#33142=ADVANCED_FACE('',(#4168),#2329,.F.);
#33143=ADVANCED_FACE('',(#4169),#2330,.T.);
#33144=ADVANCED_FACE('',(#4170),#2331,.T.);
#33145=ADVANCED_FACE('',(#4171),#2332,.T.);
#33146=ADVANCED_FACE('',(#4172),#2333,.T.);
#33147=ADVANCED_FACE('',(#4173),#2334,.T.);
#33148=ADVANCED_FACE('',(#4174),#2335,.T.);
#33149=ADVANCED_FACE('',(#4175),#2336,.T.);
#33150=ADVANCED_FACE('',(#4176),#2337,.T.);
#33151=ADVANCED_FACE('',(#4177),#2338,.T.);
#33152=ADVANCED_FACE('',(#4178),#2339,.T.);
#33153=ADVANCED_FACE('',(#4179),#2340,.T.);
#33154=ADVANCED_FACE('',(#4180),#2341,.T.);
#33155=ADVANCED_FACE('',(#4181),#2342,.T.);
#33156=ADVANCED_FACE('',(#4182),#2343,.T.);
#33157=ADVANCED_FACE('',(#4183),#2344,.F.);
#33158=ADVANCED_FACE('',(#4184),#2345,.T.);
#33159=ADVANCED_FACE('',(#4185),#2346,.T.);
#33160=ADVANCED_FACE('',(#4186),#31954,.F.);
#33161=ADVANCED_FACE('',(#4187),#31955,.F.);
#33162=ADVANCED_FACE('',(#4188),#3001,.F.);
#33163=ADVANCED_FACE('',(#4189),#2347,.T.);
#33164=ADVANCED_FACE('',(#4190),#2348,.T.);
#33165=ADVANCED_FACE('',(#4191),#2349,.T.);
#33166=ADVANCED_FACE('',(#4192),#2350,.T.);
#33167=ADVANCED_FACE('',(#4193),#2351,.T.);
#33168=ADVANCED_FACE('',(#4194),#2352,.T.);
#33169=ADVANCED_FACE('',(#4195),#2353,.T.);
#33170=ADVANCED_FACE('',(#4196),#2354,.T.);
#33171=ADVANCED_FACE('',(#4197),#2355,.T.);
#33172=ADVANCED_FACE('',(#4198),#2356,.T.);
#33173=ADVANCED_FACE('',(#4199),#2357,.T.);
#33174=ADVANCED_FACE('',(#4200),#2358,.T.);
#33175=ADVANCED_FACE('',(#4201),#2359,.F.);
#33176=ADVANCED_FACE('',(#4202),#2360,.T.);
#33177=ADVANCED_FACE('',(#4203),#2361,.T.);
#33178=ADVANCED_FACE('',(#4204),#2362,.T.);
#33179=ADVANCED_FACE('',(#4205),#2363,.T.);
#33180=ADVANCED_FACE('',(#4206),#2364,.T.);
#33181=ADVANCED_FACE('',(#4207),#2365,.T.);
#33182=ADVANCED_FACE('',(#4208),#2366,.T.);
#33183=ADVANCED_FACE('',(#4209),#2367,.T.);
#33184=ADVANCED_FACE('',(#4210),#2368,.T.);
#33185=ADVANCED_FACE('',(#4211),#2369,.T.);
#33186=ADVANCED_FACE('',(#4212),#2370,.T.);
#33187=ADVANCED_FACE('',(#4213),#2371,.T.);
#33188=ADVANCED_FACE('',(#4214),#2372,.T.);
#33189=ADVANCED_FACE('',(#4215),#2373,.T.);
#33190=ADVANCED_FACE('',(#4216),#2374,.F.);
#33191=ADVANCED_FACE('',(#4217),#2375,.T.);
#33192=ADVANCED_FACE('',(#4218),#2376,.T.);
#33193=ADVANCED_FACE('',(#4219),#31956,.T.);
#33194=ADVANCED_FACE('',(#4220),#3002,.T.);
#33195=ADVANCED_FACE('',(#4221),#31957,.T.);
#33196=ADVANCED_FACE('',(#4222),#31958,.F.);
#33197=ADVANCED_FACE('',(#4223,#1210),#2377,.T.);
#33198=ADVANCED_FACE('',(#4224),#31959,.T.);
#33199=ADVANCED_FACE('',(#4225),#31960,.T.);
#33200=ADVANCED_FACE('',(#4226),#31961,.T.);
#33201=ADVANCED_FACE('',(#4227),#2378,.T.);
#33202=ADVANCED_FACE('',(#4228),#2379,.T.);
#33203=ADVANCED_FACE('',(#4229),#2380,.T.);
#33204=ADVANCED_FACE('',(#4230),#2381,.T.);
#33205=ADVANCED_FACE('',(#4231),#2382,.T.);
#33206=ADVANCED_FACE('',(#4232),#2383,.T.);
#33207=ADVANCED_FACE('',(#4233),#2384,.T.);
#33208=ADVANCED_FACE('',(#4234),#2385,.T.);
#33209=ADVANCED_FACE('',(#4235),#2386,.F.);
#33210=ADVANCED_FACE('',(#4236),#2387,.T.);
#33211=ADVANCED_FACE('',(#4237),#2388,.T.);
#33212=ADVANCED_FACE('',(#4238),#2389,.T.);
#33213=ADVANCED_FACE('',(#4239),#2390,.F.);
#33214=ADVANCED_FACE('',(#4240),#2391,.T.);
#33215=ADVANCED_FACE('',(#4241),#2392,.T.);
#33216=ADVANCED_FACE('',(#4242),#2393,.T.);
#33217=ADVANCED_FACE('',(#4243),#2394,.T.);
#33218=ADVANCED_FACE('',(#4244),#2395,.T.);
#33219=ADVANCED_FACE('',(#4245),#2396,.F.);
#33220=ADVANCED_FACE('',(#4246),#2397,.T.);
#33221=ADVANCED_FACE('',(#4247),#2398,.T.);
#33222=ADVANCED_FACE('',(#4248),#2399,.T.);
#33223=ADVANCED_FACE('',(#4249),#2400,.F.);
#33224=ADVANCED_FACE('',(#4250),#2401,.T.);
#33225=ADVANCED_FACE('',(#4251),#2402,.T.);
#33226=ADVANCED_FACE('',(#4252),#2403,.T.);
#33227=ADVANCED_FACE('',(#4253),#2404,.T.);
#33228=ADVANCED_FACE('',(#4254),#2405,.T.);
#33229=ADVANCED_FACE('',(#4255),#2406,.F.);
#33230=ADVANCED_FACE('',(#4256),#2407,.T.);
#33231=ADVANCED_FACE('',(#4257),#2408,.T.);
#33232=ADVANCED_FACE('',(#4258),#2409,.T.);
#33233=ADVANCED_FACE('',(#4259),#2410,.F.);
#33234=ADVANCED_FACE('',(#4260),#2411,.T.);
#33235=ADVANCED_FACE('',(#4261),#2412,.T.);
#33236=ADVANCED_FACE('',(#4262),#2413,.T.);
#33237=ADVANCED_FACE('',(#4263),#2414,.T.);
#33238=ADVANCED_FACE('',(#4264),#2415,.T.);
#33239=ADVANCED_FACE('',(#4265),#2416,.F.);
#33240=ADVANCED_FACE('',(#4266),#2417,.T.);
#33241=ADVANCED_FACE('',(#4267),#2418,.T.);
#33242=ADVANCED_FACE('',(#4268),#2419,.T.);
#33243=ADVANCED_FACE('',(#4269),#2420,.F.);
#33244=ADVANCED_FACE('',(#4270),#2421,.T.);
#33245=ADVANCED_FACE('',(#4271),#2422,.T.);
#33246=ADVANCED_FACE('',(#4272),#2423,.T.);
#33247=ADVANCED_FACE('',(#4273),#2424,.T.);
#33248=ADVANCED_FACE('',(#4274),#2425,.T.);
#33249=ADVANCED_FACE('',(#4275),#2426,.F.);
#33250=ADVANCED_FACE('',(#4276),#2427,.T.);
#33251=ADVANCED_FACE('',(#4277),#2428,.T.);
#33252=ADVANCED_FACE('',(#4278),#2429,.T.);
#33253=ADVANCED_FACE('',(#4279),#2430,.F.);
#33254=ADVANCED_FACE('',(#4280),#2431,.T.);
#33255=ADVANCED_FACE('',(#4281),#2432,.T.);
#33256=ADVANCED_FACE('',(#4282),#2433,.T.);
#33257=ADVANCED_FACE('',(#4283),#2434,.T.);
#33258=ADVANCED_FACE('',(#4284),#2435,.T.);
#33259=ADVANCED_FACE('',(#4285),#2436,.F.);
#33260=ADVANCED_FACE('',(#4286),#2437,.T.);
#33261=ADVANCED_FACE('',(#4287),#2438,.T.);
#33262=ADVANCED_FACE('',(#4288),#2439,.T.);
#33263=ADVANCED_FACE('',(#4289),#2440,.F.);
#33264=ADVANCED_FACE('',(#4290),#2441,.T.);
#33265=ADVANCED_FACE('',(#4291),#2442,.T.);
#33266=ADVANCED_FACE('',(#4292),#2443,.T.);
#33267=ADVANCED_FACE('',(#4293),#2444,.T.);
#33268=ADVANCED_FACE('',(#4294),#2445,.T.);
#33269=ADVANCED_FACE('',(#4295),#2446,.F.);
#33270=ADVANCED_FACE('',(#4296),#2447,.T.);
#33271=ADVANCED_FACE('',(#4297),#2448,.T.);
#33272=ADVANCED_FACE('',(#4298),#2449,.T.);
#33273=ADVANCED_FACE('',(#4299),#2450,.F.);
#33274=ADVANCED_FACE('',(#4300),#2451,.T.);
#33275=ADVANCED_FACE('',(#4301),#2452,.T.);
#33276=ADVANCED_FACE('',(#4302),#2453,.T.);
#33277=ADVANCED_FACE('',(#4303),#2454,.T.);
#33278=ADVANCED_FACE('',(#4304),#2455,.T.);
#33279=ADVANCED_FACE('',(#4305),#2456,.F.);
#33280=ADVANCED_FACE('',(#4306),#2457,.T.);
#33281=ADVANCED_FACE('',(#4307),#2458,.T.);
#33282=ADVANCED_FACE('',(#4308),#2459,.T.);
#33283=ADVANCED_FACE('',(#4309),#2460,.F.);
#33284=ADVANCED_FACE('',(#4310),#2461,.T.);
#33285=ADVANCED_FACE('',(#4311),#2462,.T.);
#33286=ADVANCED_FACE('',(#4312),#2463,.T.);
#33287=ADVANCED_FACE('',(#4313),#2464,.T.);
#33288=ADVANCED_FACE('',(#4314),#2465,.T.);
#33289=ADVANCED_FACE('',(#4315),#2466,.F.);
#33290=ADVANCED_FACE('',(#4316),#2467,.T.);
#33291=ADVANCED_FACE('',(#4317),#2468,.T.);
#33292=ADVANCED_FACE('',(#4318),#2469,.T.);
#33293=ADVANCED_FACE('',(#4319),#2470,.F.);
#33294=ADVANCED_FACE('',(#4320),#2471,.T.);
#33295=ADVANCED_FACE('',(#4321),#2472,.T.);
#33296=ADVANCED_FACE('',(#4322),#2473,.T.);
#33297=ADVANCED_FACE('',(#4323),#2474,.T.);
#33298=ADVANCED_FACE('',(#4324),#2475,.T.);
#33299=ADVANCED_FACE('',(#4325),#2476,.F.);
#33300=ADVANCED_FACE('',(#4326),#2477,.T.);
#33301=ADVANCED_FACE('',(#4327),#2478,.T.);
#33302=ADVANCED_FACE('',(#4328),#2479,.T.);
#33303=ADVANCED_FACE('',(#4329),#2480,.F.);
#33304=ADVANCED_FACE('',(#4330),#2481,.T.);
#33305=ADVANCED_FACE('',(#4331),#2482,.T.);
#33306=ADVANCED_FACE('',(#4332),#2483,.T.);
#33307=ADVANCED_FACE('',(#4333),#2484,.T.);
#33308=ADVANCED_FACE('',(#4334),#2485,.T.);
#33309=ADVANCED_FACE('',(#4335),#2486,.F.);
#33310=ADVANCED_FACE('',(#4336),#2487,.T.);
#33311=ADVANCED_FACE('',(#4337),#2488,.T.);
#33312=ADVANCED_FACE('',(#4338),#2489,.T.);
#33313=ADVANCED_FACE('',(#4339),#2490,.F.);
#33314=ADVANCED_FACE('',(#4340),#2491,.T.);
#33315=ADVANCED_FACE('',(#4341),#2492,.T.);
#33316=ADVANCED_FACE('',(#4342),#2493,.T.);
#33317=ADVANCED_FACE('',(#4343),#2494,.T.);
#33318=ADVANCED_FACE('',(#4344),#2495,.T.);
#33319=ADVANCED_FACE('',(#4345),#2496,.F.);
#33320=ADVANCED_FACE('',(#4346),#2497,.T.);
#33321=ADVANCED_FACE('',(#4347),#2498,.T.);
#33322=ADVANCED_FACE('',(#4348),#2499,.T.);
#33323=ADVANCED_FACE('',(#4349),#2500,.F.);
#33324=ADVANCED_FACE('',(#4350),#2501,.T.);
#33325=ADVANCED_FACE('',(#4351),#2502,.T.);
#33326=ADVANCED_FACE('',(#4352),#2503,.T.);
#33327=ADVANCED_FACE('',(#4353),#2504,.T.);
#33328=ADVANCED_FACE('',(#4354),#2505,.T.);
#33329=ADVANCED_FACE('',(#4355),#2506,.F.);
#33330=ADVANCED_FACE('',(#4356),#2507,.T.);
#33331=ADVANCED_FACE('',(#4357),#2508,.T.);
#33332=ADVANCED_FACE('',(#4358),#2509,.T.);
#33333=ADVANCED_FACE('',(#4359),#2510,.F.);
#33334=ADVANCED_FACE('',(#4360),#2511,.T.);
#33335=ADVANCED_FACE('',(#4361),#2512,.T.);
#33336=ADVANCED_FACE('',(#4362),#2513,.T.);
#33337=ADVANCED_FACE('',(#4363),#2514,.T.);
#33338=ADVANCED_FACE('',(#4364),#2515,.T.);
#33339=ADVANCED_FACE('',(#4365),#2516,.F.);
#33340=ADVANCED_FACE('',(#4366),#2517,.T.);
#33341=ADVANCED_FACE('',(#4367),#2518,.T.);
#33342=ADVANCED_FACE('',(#4368),#2519,.T.);
#33343=ADVANCED_FACE('',(#4369),#2520,.F.);
#33344=ADVANCED_FACE('',(#4370),#2521,.T.);
#33345=ADVANCED_FACE('',(#4371),#3003,.F.);
#33346=ADVANCED_FACE('',(#4372),#3004,.F.);
#33347=ADVANCED_FACE('',(#4373),#3005,.F.);
#33348=ADVANCED_FACE('',(#4374),#3006,.F.);
#33349=ADVANCED_FACE('',(#4375),#3007,.F.);
#33350=ADVANCED_FACE('',(#4376),#31962,.F.);
#33351=ADVANCED_FACE('',(#4377),#3008,.F.);
#33352=ADVANCED_FACE('',(#4378),#3009,.T.);
#33353=ADVANCED_FACE('',(#4379),#3010,.T.);
#33354=ADVANCED_FACE('',(#4380),#3011,.T.);
#33355=ADVANCED_FACE('',(#4381),#3012,.T.);
#33356=ADVANCED_FACE('',(#4382,#1211),#2522,.T.);
#33357=ADVANCED_FACE('',(#4383),#3013,.F.);
#33358=ADVANCED_FACE('',(#4384,#1212),#2523,.T.);
#33359=ADVANCED_FACE('',(#4385),#3014,.F.);
#33360=ADVANCED_FACE('',(#4386,#1213),#2524,.T.);
#33361=ADVANCED_FACE('',(#4387),#3015,.F.);
#33362=ADVANCED_FACE('',(#4388,#1214),#2525,.T.);
#33363=ADVANCED_FACE('',(#4389),#3016,.F.);
#33364=ADVANCED_FACE('',(#4390),#31963,.F.);
#33365=ADVANCED_FACE('',(#4391),#31964,.T.);
#33366=ADVANCED_FACE('',(#4392,#1215,#1216,#1217,#1218,#1219,#1220),#2526,
 .T.);
#33367=ADVANCED_FACE('',(#4393),#31965,.F.);
#33368=ADVANCED_FACE('',(#4394),#31966,.F.);
#34208=CLOSED_SHELL('',(#32113,#32114,#32115,#32116,#32117,#32118,#32119,
#32120,#32121,#32122,#32123,#32124,#32125,#32126,#32127,#32128,#32129,#32130,
#32131,#32132,#32133,#32134,#32135,#32136,#32137,#32138,#32139,#32140,#32141,
#32142,#32143,#32144,#32145,#32146,#32147,#32148,#32149,#32150,#32151,#32152,
#32153,#32154,#32155,#32156,#32157,#32158,#32159,#32160,#32161,#32162,#32163,
#32164,#32165,#32166,#32167,#32168,#32169,#32170,#32171,#32172,#32173,#32174,
#32175,#32176,#32177,#32178,#32179,#32180,#32181,#32182,#32183,#32184,#32185,
#32186,#32187,#32188,#32189,#32190,#32191,#32192,#32193,#32194,#32195,#32196,
#32197,#32198,#32199,#32200,#32201,#32202,#32203,#32204,#32205,#32206,#32207,
#32208,#32209,#32210,#32211,#32212,#32213,#32214,#32215,#32216,#32217,#32218,
#32219,#32220,#32221,#32222,#32223,#32224,#32225,#32226,#32227,#32228,#32229,
#32230,#32231,#32232,#32233,#32234,#32235,#32236,#32237,#32238,#32239,#32240,
#32241,#32242,#32243,#32244,#32245,#32246,#32247,#32248,#32249,#32250,#32251,
#32252,#32253,#32254,#32255,#32256,#32257,#32258,#32259,#32260,#32261,#32262,
#32263,#32264,#32265,#32266,#32267,#32268,#32269,#32270,#32271,#32272,#32273,
#32274,#32275,#32276,#32277,#32278,#32279,#32280,#32281,#32282,#32283,#32284,
#32285,#32286,#32287,#32288,#32289,#32290,#32291,#32292,#32293,#32294,#32295,
#32296,#32297,#32298,#32299,#32300,#32301,#32302,#32303,#32304,#32305,#32306,
#32307,#32308,#32309,#32310,#32311,#32312,#32313,#32314,#32315,#32316,#32317,
#32318,#32319,#32320,#32321,#32322,#32323,#32324,#32325,#32326,#32327,#32328,
#32329,#32330,#32331,#32332,#32333,#32334,#32335,#32336,#32337,#32338,#32339,
#32340,#32341,#32342,#32343,#32344,#32345,#32346,#32347,#32348,#32349,#32350,
#32351,#32352,#32353,#32354,#32355,#32356,#32357,#32358,#32359,#32360,#32361,
#32362,#32363,#32364,#32365,#32366,#32367,#32368,#32369,#32370,#32371,#32372,
#32373,#32374,#32375,#32376,#32377,#32378,#32379,#32380,#32381,#32382,#32383,
#32384,#32385,#32386,#32387,#32388,#32389,#32390,#32391,#32392,#32393,#32394,
#32395,#32396,#32397,#32398,#32399,#32400,#32401,#32402,#32403,#32404,#32405,
#32406,#32407,#32408,#32409,#32410,#32411,#32412,#32413,#32414,#32415,#32416,
#32417,#32418,#32419,#32420,#32421,#32422,#32423,#32424,#32425,#32426,#32427,
#32428,#32429,#32430,#32431,#32432,#32433,#32434,#32435,#32436,#32437,#32438,
#32439,#32440,#32441,#32442,#32443,#32444,#32445,#32446,#32447,#32448,#32449,
#32450,#32451,#32452,#32453,#32454,#32455,#32456,#32457,#32458,#32459,#32460,
#32461,#32462,#32463,#32464,#32465,#32466,#32467,#32468,#32469,#32470,#32471,
#32472,#32473,#32474,#32475,#32476,#32477,#32478,#32479,#32480,#32481,#32482,
#32483,#32484,#32485,#32486,#32487,#32488,#32489,#32490,#32491,#32492,#32493,
#32494,#32495,#32496,#32497,#32498,#32499,#32500,#32501,#32502,#32503,#32504,
#32505,#32506,#32507,#32508,#32509,#32510,#32511,#32512,#32513,#32514,#32515,
#32516,#32517,#32518,#32519,#32520,#32521,#32522,#32523,#32524,#32525,#32526,
#32527,#32528,#32529,#32530,#32531,#32532,#32533,#32534,#32535,#32536,#32537,
#32538,#32539,#32540,#32541,#32542,#32543,#32544,#32545,#32546,#32547,#32548,
#32549,#32550,#32551,#32552,#32553,#32554,#32555,#32556,#32557,#32558,#32559,
#32560,#32561,#32562,#32563,#32564,#32565,#32566,#32567,#32568,#32569,#32570,
#32571,#32572,#32573,#32574,#32575,#32576,#32577,#32578,#32579,#32580,#32581,
#32582,#32583,#32584,#32585,#32586,#32587,#32588,#32589,#32590,#32591,#32592,
#32593,#32594,#32595,#32596,#32597,#32598,#32599,#32600,#32601,#32602,#32603,
#32604,#32605,#32606,#32607,#32608,#32609,#32610,#32611,#32612,#32613,#32614,
#32615,#32616,#32617,#32618,#32619,#32620,#32621,#32622,#32623,#32624,#32625,
#32626,#32627,#32628,#32629,#32630,#32631,#32632,#32633,#32634,#32635,#32636,
#32637,#32638,#32639,#32640,#32641,#32642,#32643,#32644,#32645,#32646,#32647,
#32648,#32649,#32650,#32651,#32652,#32653,#32654,#32655,#32656,#32657,#32658,
#32659,#32660,#32661,#32662,#32663,#32664,#32665,#32666,#32667,#32668,#32669,
#32670,#32671,#32672,#32673,#32674,#32675,#32676,#32677,#32678,#32679,#32680,
#32681,#32682,#32683,#32684,#32685,#32686,#32687,#32688,#32689,#32690,#32691,
#32692,#32693,#32694,#32695,#32696,#32697,#32698,#32699,#32700,#32701,#32702,
#32703,#32704,#32705,#32706,#32707,#32708,#32709,#32710,#32711,#32712,#32713,
#32714,#32715,#32716,#32717,#32718,#32719,#32720,#32721,#32722,#32723,#32724,
#32725,#32726,#32727,#32728,#32729,#32730,#32731,#32732,#32733,#32734,#32735,
#32736,#32737,#32738,#32739,#32740,#32741,#32742,#32743,#32744,#32745,#32746,
#32747,#32748,#32749,#32750,#32751,#32752,#32753,#32754,#32755,#32756,#32757,
#32758,#32759,#32760,#32761,#32762,#32763,#32764,#32765,#32766,#32767,#32768,
#32769,#32770,#32771,#32772,#32773,#32774,#32775,#32776,#32777,#32778,#32779,
#32780,#32781,#32782,#32783,#32784,#32785,#32786,#32787,#32788,#32789,#32790,
#32791,#32792,#32793,#32794,#32795,#32796,#32797,#32798,#32799,#32800,#32801,
#32802,#32803,#32804,#32805,#32806,#32807,#32808,#32809,#32810,#32811,#32812,
#32813,#32814,#32815,#32816,#32817,#32818,#32819,#32820,#32821,#32822,#32823,
#32824,#32825,#32826,#32827,#32828,#32829,#32830,#32831,#32832,#32833,#32834,
#32835,#32836,#32837,#32838,#32839,#32840,#32841,#32842,#32843,#32844,#32845,
#32846,#32847,#32848,#32849,#32850,#32851,#32852,#32853,#32854,#32855,#32856,
#32857,#32858,#32859,#32860,#32861,#32862,#32863,#32864,#32865,#32866,#32867,
#32868,#32869,#32870,#32871,#32872,#32873,#32874,#32875,#32876,#32877,#32878,
#32879,#32880,#32881,#32882,#32883,#32884,#32885,#32886,#32887,#32888,#32889,
#32890,#32891,#32892,#32893,#32894,#32895,#32896,#32897,#32898,#32899,#32900,
#32901,#32902,#32903,#32904,#32905,#32906,#32907,#32908,#32909,#32910,#32911,
#32912,#32913,#32914,#32915,#32916,#32917,#32918,#32919,#32920,#32921,#32922,
#32923,#32924,#32925,#32926,#32927,#32928,#32929,#32930,#32931,#32932,#32933,
#32934,#32935,#32936,#32937,#32938,#32939,#32940,#32941,#32942,#32943,#32944,
#32945,#32946,#32947,#32948,#32949,#32950,#32951,#32952,#32953,#32954,#32955,
#32956,#32957,#32958,#32959,#32960,#32961,#32962,#32963,#32964,#32965,#32966,
#32967,#32968,#32969,#32970,#32971,#32972,#32973,#32974,#32975,#32976,#32977,
#32978,#32979,#32980,#32981,#32982,#32983,#32984,#32985,#32986,#32987,#32988,
#32989,#32990,#32991,#32992,#32993,#32994,#32995,#32996,#32997,#32998,#32999,
#33000,#33001,#33002,#33003,#33004,#33005,#33006,#33007,#33008,#33009,#33010,
#33011,#33012,#33013,#33014,#33015,#33016,#33017,#33018,#33019,#33020,#33021,
#33022,#33023,#33024,#33025,#33026,#33027,#33028,#33029,#33030,#33031,#33032,
#33033,#33034,#33035,#33036,#33037,#33038,#33039,#33040,#33041,#33042,#33043,
#33044,#33045,#33046,#33047,#33048,#33049,#33050,#33051,#33052,#33053,#33054,
#33055,#33056,#33057,#33058,#33059,#33060,#33061,#33062,#33063,#33064,#33065,
#33066,#33067,#33068,#33069,#33070,#33071,#33072,#33073,#33074,#33075,#33076,
#33077,#33078,#33079,#33080,#33081,#33082,#33083,#33084,#33085,#33086,#33087,
#33088,#33089,#33090,#33091,#33092,#33093,#33094,#33095,#33096,#33097,#33098,
#33099,#33100,#33101,#33102,#33103,#33104,#33105,#33106,#33107,#33108,#33109,
#33110,#33111,#33112,#33113,#33114,#33115,#33116,#33117,#33118,#33119,#33120,
#33121,#33122,#33123,#33124,#33125,#33126,#33127,#33128,#33129,#33130,#33131,
#33132,#33133,#33134,#33135,#33136,#33137,#33138,#33139,#33140,#33141,#33142,
#33143,#33144,#33145,#33146,#33147,#33148,#33149,#33150,#33151,#33152,#33153,
#33154,#33155,#33156,#33157,#33158,#33159,#33160,#33161,#33162,#33163,#33164,
#33165,#33166,#33167,#33168,#33169,#33170,#33171,#33172,#33173,#33174,#33175,
#33176,#33177,#33178,#33179,#33180,#33181,#33182,#33183,#33184,#33185,#33186,
#33187,#33188,#33189,#33190,#33191,#33192,#33193,#33194,#33195,#33196,#33197,
#33198,#33199,#33200,#33201,#33202,#33203,#33204,#33205,#33206,#33207,#33208,
#33209,#33210,#33211,#33212,#33213,#33214,#33215,#33216,#33217,#33218,#33219,
#33220,#33221,#33222,#33223,#33224,#33225,#33226,#33227,#33228,#33229,#33230,
#33231,#33232,#33233,#33234,#33235,#33236,#33237,#33238,#33239,#33240,#33241,
#33242,#33243,#33244,#33245,#33246,#33247,#33248,#33249,#33250,#33251,#33252,
#33253,#33254,#33255,#33256,#33257,#33258,#33259,#33260,#33261,#33262,#33263,
#33264,#33265,#33266,#33267,#33268,#33269,#33270,#33271,#33272,#33273,#33274,
#33275,#33276,#33277,#33278,#33279,#33280,#33281,#33282,#33283,#33284,#33285,
#33286,#33287,#33288,#33289,#33290,#33291,#33292,#33293,#33294,#33295,#33296,
#33297,#33298,#33299,#33300,#33301,#33302,#33303,#33304,#33305,#33306,#33307,
#33308,#33309,#33310,#33311,#33312,#33313,#33314,#33315,#33316,#33317,#33318,
#33319,#33320,#33321,#33322,#33323,#33324,#33325,#33326,#33327,#33328,#33329,
#33330,#33331,#33332,#33333,#33334,#33335,#33336,#33337,#33338,#33339,#33340,
#33341,#33342,#33343,#33344,#33345,#33346,#33347,#33348,#33349,#33350,#33351,
#33352,#33353,#33354,#33355,#33356,#33357,#33358,#33359,#33360,#33361,#33362,
#33363,#33364,#33365,#33366,#33367,#33368));
#34366=AXIS2_PLACEMENT_3D('',#47304,#37663,#37664);
#34367=AXIS2_PLACEMENT_3D('',#47305,#37665,#37666);
#34368=AXIS2_PLACEMENT_3D('',#47308,#37667,#37668);
#34369=AXIS2_PLACEMENT_3D('',#47309,#37669,#37670);
#34370=AXIS2_PLACEMENT_3D('',#47313,#37672,#37673);
#34371=AXIS2_PLACEMENT_3D('',#47314,#37674,#37675);
#34372=AXIS2_PLACEMENT_3D('',#47315,#37676,#37677);
#34373=AXIS2_PLACEMENT_3D('',#47319,#37679,#37680);
#34374=AXIS2_PLACEMENT_3D('',#47320,#37681,#37682);
#34375=AXIS2_PLACEMENT_3D('',#47321,#37683,#37684);
#34376=AXIS2_PLACEMENT_3D('',#47323,#37685,#37686);
#34377=AXIS2_PLACEMENT_3D('',#47325,#37688,#37689);
#34378=AXIS2_PLACEMENT_3D('',#47328,#37691,#37692);
#34379=AXIS2_PLACEMENT_3D('',#47329,#37693,#37694);
#34380=AXIS2_PLACEMENT_3D('',#47331,#37695,#37696);
#34381=AXIS2_PLACEMENT_3D('',#47332,#37697,#37698);
#34382=AXIS2_PLACEMENT_3D('',#47334,#37699,#37700);
#34383=AXIS2_PLACEMENT_3D('',#47338,#37702,#37703);
#34384=AXIS2_PLACEMENT_3D('',#47339,#37704,#37705);
#34385=AXIS2_PLACEMENT_3D('',#47340,#37706,#37707);
#34386=AXIS2_PLACEMENT_3D('',#47342,#37708,#37709);
#34387=AXIS2_PLACEMENT_3D('',#47344,#37711,#37712);
#34388=AXIS2_PLACEMENT_3D('',#47346,#37713,#37714);
#34389=AXIS2_PLACEMENT_3D('',#47347,#37715,#37716);
#34390=AXIS2_PLACEMENT_3D('',#47349,#37717,#37718);
#34391=AXIS2_PLACEMENT_3D('',#47353,#37720,#37721);
#34392=AXIS2_PLACEMENT_3D('',#47354,#37722,#37723);
#34393=AXIS2_PLACEMENT_3D('',#47355,#37724,#37725);
#34394=AXIS2_PLACEMENT_3D('',#47359,#37727,#37728);
#34395=AXIS2_PLACEMENT_3D('',#47360,#37729,#37730);
#34396=AXIS2_PLACEMENT_3D('',#47361,#37731,#37732);
#34397=AXIS2_PLACEMENT_3D('',#47363,#37733,#37734);
#34398=AXIS2_PLACEMENT_3D('',#47364,#37735,#37736);
#34399=AXIS2_PLACEMENT_3D('',#47368,#37738,#37739);
#34400=AXIS2_PLACEMENT_3D('',#47369,#37740,#37741);
#34401=AXIS2_PLACEMENT_3D('',#47370,#37742,#37743);
#34402=AXIS2_PLACEMENT_3D('',#47373,#37745,#37746);
#34403=AXIS2_PLACEMENT_3D('',#47374,#37747,#37748);
#34404=AXIS2_PLACEMENT_3D('',#47377,#37749,#37750);
#34405=AXIS2_PLACEMENT_3D('',#47378,#37751,#37752);
#34406=AXIS2_PLACEMENT_3D('',#47382,#37754,#37755);
#34407=AXIS2_PLACEMENT_3D('',#47383,#37756,#37757);
#34408=AXIS2_PLACEMENT_3D('',#47384,#37758,#37759);
#34409=AXIS2_PLACEMENT_3D('',#47388,#37761,#37762);
#34410=AXIS2_PLACEMENT_3D('',#47389,#37763,#37764);
#34411=AXIS2_PLACEMENT_3D('',#47390,#37765,#37766);
#34412=AXIS2_PLACEMENT_3D('',#47392,#37767,#37768);
#34413=AXIS2_PLACEMENT_3D('',#47394,#37770,#37771);
#34414=AXIS2_PLACEMENT_3D('',#47398,#37773,#37774);
#34415=AXIS2_PLACEMENT_3D('',#47399,#37775,#37776);
#34416=AXIS2_PLACEMENT_3D('',#47400,#37777,#37778);
#34417=AXIS2_PLACEMENT_3D('',#47404,#37780,#37781);
#34418=AXIS2_PLACEMENT_3D('',#47405,#37782,#37783);
#34419=AXIS2_PLACEMENT_3D('',#47406,#37784,#37785);
#34420=AXIS2_PLACEMENT_3D('',#47410,#37787,#37788);
#34421=AXIS2_PLACEMENT_3D('',#47411,#37789,#37790);
#34422=AXIS2_PLACEMENT_3D('',#47412,#37791,#37792);
#34423=AXIS2_PLACEMENT_3D('',#47416,#37794,#37795);
#34424=AXIS2_PLACEMENT_3D('',#47417,#37796,#37797);
#34425=AXIS2_PLACEMENT_3D('',#47418,#37798,#37799);
#34426=AXIS2_PLACEMENT_3D('',#47422,#37801,#37802);
#34427=AXIS2_PLACEMENT_3D('',#47423,#37803,#37804);
#34428=AXIS2_PLACEMENT_3D('',#47424,#37805,#37806);
#34429=AXIS2_PLACEMENT_3D('',#47428,#37808,#37809);
#34430=AXIS2_PLACEMENT_3D('',#47430,#37810,#37811);
#34431=AXIS2_PLACEMENT_3D('',#47434,#37813,#37814);
#34432=AXIS2_PLACEMENT_3D('',#47436,#37815,#37816);
#34433=AXIS2_PLACEMENT_3D('',#47439,#37818,#37819);
#34434=AXIS2_PLACEMENT_3D('',#47441,#37820,#37821);
#34435=AXIS2_PLACEMENT_3D('',#47443,#37822,#37823);
#34436=AXIS2_PLACEMENT_3D('',#47447,#37825,#37826);
#34437=AXIS2_PLACEMENT_3D('',#47448,#37827,#37828);
#34438=AXIS2_PLACEMENT_3D('',#47453,#37830,#37831);
#34439=AXIS2_PLACEMENT_3D('',#47455,#37832,#37833);
#34440=AXIS2_PLACEMENT_3D('',#47457,#37834,#37835);
#34441=AXIS2_PLACEMENT_3D('',#47461,#37837,#37838);
#34442=AXIS2_PLACEMENT_3D('',#47463,#37839,#37840);
#34443=AXIS2_PLACEMENT_3D('',#47464,#37841,#37842);
#34444=AXIS2_PLACEMENT_3D('',#47469,#37844,#37845);
#34445=AXIS2_PLACEMENT_3D('',#47471,#37846,#37847);
#34446=AXIS2_PLACEMENT_3D('',#47473,#37848,#37849);
#34447=AXIS2_PLACEMENT_3D('',#47477,#37851,#37852);
#34448=AXIS2_PLACEMENT_3D('',#47479,#37853,#37854);
#34449=AXIS2_PLACEMENT_3D('',#47480,#37855,#37856);
#34450=AXIS2_PLACEMENT_3D('',#47485,#37858,#37859);
#34451=AXIS2_PLACEMENT_3D('',#47487,#37860,#37861);
#34452=AXIS2_PLACEMENT_3D('',#47489,#37862,#37863);
#34453=AXIS2_PLACEMENT_3D('',#47493,#37865,#37866);
#34454=AXIS2_PLACEMENT_3D('',#47495,#37867,#37868);
#34455=AXIS2_PLACEMENT_3D('',#47496,#37869,#37870);
#34456=AXIS2_PLACEMENT_3D('',#47501,#37872,#37873);
#34457=AXIS2_PLACEMENT_3D('',#47503,#37874,#37875);
#34458=AXIS2_PLACEMENT_3D('',#47505,#37876,#37877);
#34459=AXIS2_PLACEMENT_3D('',#47509,#37879,#37880);
#34460=AXIS2_PLACEMENT_3D('',#47511,#37881,#37882);
#34461=AXIS2_PLACEMENT_3D('',#47512,#37883,#37884);
#34462=AXIS2_PLACEMENT_3D('',#47517,#37886,#37887);
#34463=AXIS2_PLACEMENT_3D('',#47519,#37888,#37889);
#34464=AXIS2_PLACEMENT_3D('',#47521,#37890,#37891);
#34465=AXIS2_PLACEMENT_3D('',#47525,#37893,#37894);
#34466=AXIS2_PLACEMENT_3D('',#47527,#37895,#37896);
#34467=AXIS2_PLACEMENT_3D('',#47528,#37897,#37898);
#34468=AXIS2_PLACEMENT_3D('',#47533,#37900,#37901);
#34469=AXIS2_PLACEMENT_3D('',#47535,#37902,#37903);
#34470=AXIS2_PLACEMENT_3D('',#47537,#37904,#37905);
#34471=AXIS2_PLACEMENT_3D('',#47541,#37907,#37908);
#34472=AXIS2_PLACEMENT_3D('',#47543,#37909,#37910);
#34473=AXIS2_PLACEMENT_3D('',#47544,#37911,#37912);
#34474=AXIS2_PLACEMENT_3D('',#47549,#37914,#37915);
#34475=AXIS2_PLACEMENT_3D('',#47551,#37916,#37917);
#34476=AXIS2_PLACEMENT_3D('',#47553,#37918,#37919);
#34477=AXIS2_PLACEMENT_3D('',#47557,#37921,#37922);
#34478=AXIS2_PLACEMENT_3D('',#47559,#37923,#37924);
#34479=AXIS2_PLACEMENT_3D('',#47560,#37925,#37926);
#34480=AXIS2_PLACEMENT_3D('',#47565,#37928,#37929);
#34481=AXIS2_PLACEMENT_3D('',#47567,#37930,#37931);
#34482=AXIS2_PLACEMENT_3D('',#47569,#37932,#37933);
#34483=AXIS2_PLACEMENT_3D('',#47573,#37935,#37936);
#34484=AXIS2_PLACEMENT_3D('',#47575,#37937,#37938);
#34485=AXIS2_PLACEMENT_3D('',#47576,#37939,#37940);
#34486=AXIS2_PLACEMENT_3D('',#47581,#37942,#37943);
#34487=AXIS2_PLACEMENT_3D('',#47583,#37944,#37945);
#34488=AXIS2_PLACEMENT_3D('',#47585,#37946,#37947);
#34489=AXIS2_PLACEMENT_3D('',#47589,#37949,#37950);
#34490=AXIS2_PLACEMENT_3D('',#47591,#37951,#37952);
#34491=AXIS2_PLACEMENT_3D('',#47592,#37953,#37954);
#34492=AXIS2_PLACEMENT_3D('',#47597,#37956,#37957);
#34493=AXIS2_PLACEMENT_3D('',#47599,#37958,#37959);
#34494=AXIS2_PLACEMENT_3D('',#47601,#37960,#37961);
#34495=AXIS2_PLACEMENT_3D('',#47605,#37963,#37964);
#34496=AXIS2_PLACEMENT_3D('',#47607,#37965,#37966);
#34497=AXIS2_PLACEMENT_3D('',#47608,#37967,#37968);
#34498=AXIS2_PLACEMENT_3D('',#47613,#37970,#37971);
#34499=AXIS2_PLACEMENT_3D('',#47615,#37972,#37973);
#34500=AXIS2_PLACEMENT_3D('',#47617,#37974,#37975);
#34501=AXIS2_PLACEMENT_3D('',#47621,#37977,#37978);
#34502=AXIS2_PLACEMENT_3D('',#47623,#37979,#37980);
#34503=AXIS2_PLACEMENT_3D('',#47624,#37981,#37982);
#34504=AXIS2_PLACEMENT_3D('',#47629,#37984,#37985);
#34505=AXIS2_PLACEMENT_3D('',#47631,#37986,#37987);
#34506=AXIS2_PLACEMENT_3D('',#47633,#37988,#37989);
#34507=AXIS2_PLACEMENT_3D('',#47637,#37991,#37992);
#34508=AXIS2_PLACEMENT_3D('',#47639,#37993,#37994);
#34509=AXIS2_PLACEMENT_3D('',#47640,#37995,#37996);
#34510=AXIS2_PLACEMENT_3D('',#47645,#37998,#37999);
#34511=AXIS2_PLACEMENT_3D('',#47647,#38000,#38001);
#34512=AXIS2_PLACEMENT_3D('',#47649,#38002,#38003);
#34513=AXIS2_PLACEMENT_3D('',#47653,#38005,#38006);
#34514=AXIS2_PLACEMENT_3D('',#47655,#38007,#38008);
#34515=AXIS2_PLACEMENT_3D('',#47656,#38009,#38010);
#34516=AXIS2_PLACEMENT_3D('',#47661,#38012,#38013);
#34517=AXIS2_PLACEMENT_3D('',#47663,#38014,#38015);
#34518=AXIS2_PLACEMENT_3D('',#47665,#38016,#38017);
#34519=AXIS2_PLACEMENT_3D('',#47669,#38019,#38020);
#34520=AXIS2_PLACEMENT_3D('',#47671,#38021,#38022);
#34521=AXIS2_PLACEMENT_3D('',#47672,#38023,#38024);
#34522=AXIS2_PLACEMENT_3D('',#47677,#38026,#38027);
#34523=AXIS2_PLACEMENT_3D('',#47679,#38028,#38029);
#34524=AXIS2_PLACEMENT_3D('',#47681,#38030,#38031);
#34525=AXIS2_PLACEMENT_3D('',#47685,#38033,#38034);
#34526=AXIS2_PLACEMENT_3D('',#47687,#38035,#38036);
#34527=AXIS2_PLACEMENT_3D('',#47688,#38037,#38038);
#34528=AXIS2_PLACEMENT_3D('',#47693,#38040,#38041);
#34529=AXIS2_PLACEMENT_3D('',#47695,#38042,#38043);
#34530=AXIS2_PLACEMENT_3D('',#47697,#38044,#38045);
#34531=AXIS2_PLACEMENT_3D('',#47701,#38047,#38048);
#34532=AXIS2_PLACEMENT_3D('',#47703,#38049,#38050);
#34533=AXIS2_PLACEMENT_3D('',#47704,#38051,#38052);
#34534=AXIS2_PLACEMENT_3D('',#47709,#38054,#38055);
#34535=AXIS2_PLACEMENT_3D('',#47711,#38056,#38057);
#34536=AXIS2_PLACEMENT_3D('',#47713,#38058,#38059);
#34537=AXIS2_PLACEMENT_3D('',#47717,#38061,#38062);
#34538=AXIS2_PLACEMENT_3D('',#47719,#38063,#38064);
#34539=AXIS2_PLACEMENT_3D('',#47720,#38065,#38066);
#34540=AXIS2_PLACEMENT_3D('',#47725,#38068,#38069);
#34541=AXIS2_PLACEMENT_3D('',#47727,#38070,#38071);
#34542=AXIS2_PLACEMENT_3D('',#47729,#38072,#38073);
#34543=AXIS2_PLACEMENT_3D('',#47733,#38075,#38076);
#34544=AXIS2_PLACEMENT_3D('',#47735,#38077,#38078);
#34545=AXIS2_PLACEMENT_3D('',#47736,#38079,#38080);
#34546=AXIS2_PLACEMENT_3D('',#47741,#38082,#38083);
#34547=AXIS2_PLACEMENT_3D('',#47743,#38084,#38085);
#34548=AXIS2_PLACEMENT_3D('',#47745,#38086,#38087);
#34549=AXIS2_PLACEMENT_3D('',#47749,#38089,#38090);
#34550=AXIS2_PLACEMENT_3D('',#47751,#38091,#38092);
#34551=AXIS2_PLACEMENT_3D('',#47752,#38093,#38094);
#34552=AXIS2_PLACEMENT_3D('',#47757,#38096,#38097);
#34553=AXIS2_PLACEMENT_3D('',#47759,#38098,#38099);
#34554=AXIS2_PLACEMENT_3D('',#47761,#38100,#38101);
#34555=AXIS2_PLACEMENT_3D('',#47765,#38103,#38104);
#34556=AXIS2_PLACEMENT_3D('',#47767,#38105,#38106);
#34557=AXIS2_PLACEMENT_3D('',#47768,#38107,#38108);
#34558=AXIS2_PLACEMENT_3D('',#47773,#38110,#38111);
#34559=AXIS2_PLACEMENT_3D('',#47775,#38112,#38113);
#34560=AXIS2_PLACEMENT_3D('',#47777,#38114,#38115);
#34561=AXIS2_PLACEMENT_3D('',#47781,#38117,#38118);
#34562=AXIS2_PLACEMENT_3D('',#47783,#38119,#38120);
#34563=AXIS2_PLACEMENT_3D('',#47784,#38121,#38122);
#34564=AXIS2_PLACEMENT_3D('',#47789,#38124,#38125);
#34565=AXIS2_PLACEMENT_3D('',#47791,#38126,#38127);
#34566=AXIS2_PLACEMENT_3D('',#47793,#38128,#38129);
#34567=AXIS2_PLACEMENT_3D('',#47797,#38131,#38132);
#34568=AXIS2_PLACEMENT_3D('',#47799,#38133,#38134);
#34569=AXIS2_PLACEMENT_3D('',#47800,#38135,#38136);
#34570=AXIS2_PLACEMENT_3D('',#47805,#38138,#38139);
#34571=AXIS2_PLACEMENT_3D('',#47807,#38140,#38141);
#34572=AXIS2_PLACEMENT_3D('',#47809,#38142,#38143);
#34573=AXIS2_PLACEMENT_3D('',#47813,#38145,#38146);
#34574=AXIS2_PLACEMENT_3D('',#47815,#38147,#38148);
#34575=AXIS2_PLACEMENT_3D('',#47816,#38149,#38150);
#34576=AXIS2_PLACEMENT_3D('',#47821,#38152,#38153);
#34577=AXIS2_PLACEMENT_3D('',#47823,#38154,#38155);
#34578=AXIS2_PLACEMENT_3D('',#47825,#38156,#38157);
#34579=AXIS2_PLACEMENT_3D('',#47829,#38159,#38160);
#34580=AXIS2_PLACEMENT_3D('',#47831,#38161,#38162);
#34581=AXIS2_PLACEMENT_3D('',#47832,#38163,#38164);
#34582=AXIS2_PLACEMENT_3D('',#47837,#38166,#38167);
#34583=AXIS2_PLACEMENT_3D('',#47839,#38168,#38169);
#34584=AXIS2_PLACEMENT_3D('',#47841,#38170,#38171);
#34585=AXIS2_PLACEMENT_3D('',#47845,#38173,#38174);
#34586=AXIS2_PLACEMENT_3D('',#47847,#38175,#38176);
#34587=AXIS2_PLACEMENT_3D('',#47848,#38177,#38178);
#34588=AXIS2_PLACEMENT_3D('',#47853,#38180,#38181);
#34589=AXIS2_PLACEMENT_3D('',#47855,#38182,#38183);
#34590=AXIS2_PLACEMENT_3D('',#47857,#38184,#38185);
#34591=AXIS2_PLACEMENT_3D('',#47861,#38187,#38188);
#34592=AXIS2_PLACEMENT_3D('',#47863,#38189,#38190);
#34593=AXIS2_PLACEMENT_3D('',#47864,#38191,#38192);
#34594=AXIS2_PLACEMENT_3D('',#47869,#38194,#38195);
#34595=AXIS2_PLACEMENT_3D('',#47871,#38196,#38197);
#34596=AXIS2_PLACEMENT_3D('',#47873,#38198,#38199);
#34597=AXIS2_PLACEMENT_3D('',#47877,#38201,#38202);
#34598=AXIS2_PLACEMENT_3D('',#47879,#38203,#38204);
#34599=AXIS2_PLACEMENT_3D('',#47880,#38205,#38206);
#34600=AXIS2_PLACEMENT_3D('',#47885,#38208,#38209);
#34601=AXIS2_PLACEMENT_3D('',#47887,#38210,#38211);
#34602=AXIS2_PLACEMENT_3D('',#47889,#38212,#38213);
#34603=AXIS2_PLACEMENT_3D('',#47893,#38215,#38216);
#34604=AXIS2_PLACEMENT_3D('',#47895,#38217,#38218);
#34605=AXIS2_PLACEMENT_3D('',#47896,#38219,#38220);
#34606=AXIS2_PLACEMENT_3D('',#47901,#38222,#38223);
#34607=AXIS2_PLACEMENT_3D('',#47903,#38224,#38225);
#34608=AXIS2_PLACEMENT_3D('',#47905,#38226,#38227);
#34609=AXIS2_PLACEMENT_3D('',#47909,#38229,#38230);
#34610=AXIS2_PLACEMENT_3D('',#47911,#38231,#38232);
#34611=AXIS2_PLACEMENT_3D('',#47912,#38233,#38234);
#34612=AXIS2_PLACEMENT_3D('',#47917,#38236,#38237);
#34613=AXIS2_PLACEMENT_3D('',#47919,#38238,#38239);
#34614=AXIS2_PLACEMENT_3D('',#47921,#38240,#38241);
#34615=AXIS2_PLACEMENT_3D('',#47925,#38243,#38244);
#34616=AXIS2_PLACEMENT_3D('',#47927,#38245,#38246);
#34617=AXIS2_PLACEMENT_3D('',#47928,#38247,#38248);
#34618=AXIS2_PLACEMENT_3D('',#47933,#38250,#38251);
#34619=AXIS2_PLACEMENT_3D('',#47935,#38252,#38253);
#34620=AXIS2_PLACEMENT_3D('',#47937,#38254,#38255);
#34621=AXIS2_PLACEMENT_3D('',#47941,#38257,#38258);
#34622=AXIS2_PLACEMENT_3D('',#47943,#38259,#38260);
#34623=AXIS2_PLACEMENT_3D('',#47944,#38261,#38262);
#34624=AXIS2_PLACEMENT_3D('',#47949,#38264,#38265);
#34625=AXIS2_PLACEMENT_3D('',#47951,#38266,#38267);
#34626=AXIS2_PLACEMENT_3D('',#47953,#38268,#38269);
#34627=AXIS2_PLACEMENT_3D('',#47957,#38271,#38272);
#34628=AXIS2_PLACEMENT_3D('',#47959,#38273,#38274);
#34629=AXIS2_PLACEMENT_3D('',#47960,#38275,#38276);
#34630=AXIS2_PLACEMENT_3D('',#47965,#38278,#38279);
#34631=AXIS2_PLACEMENT_3D('',#47967,#38280,#38281);
#34632=AXIS2_PLACEMENT_3D('',#47969,#38282,#38283);
#34633=AXIS2_PLACEMENT_3D('',#47973,#38285,#38286);
#34634=AXIS2_PLACEMENT_3D('',#47975,#38287,#38288);
#34635=AXIS2_PLACEMENT_3D('',#47976,#38289,#38290);
#34636=AXIS2_PLACEMENT_3D('',#47981,#38292,#38293);
#34637=AXIS2_PLACEMENT_3D('',#47983,#38294,#38295);
#34638=AXIS2_PLACEMENT_3D('',#47985,#38296,#38297);
#34639=AXIS2_PLACEMENT_3D('',#47989,#38299,#38300);
#34640=AXIS2_PLACEMENT_3D('',#47991,#38301,#38302);
#34641=AXIS2_PLACEMENT_3D('',#47992,#38303,#38304);
#34642=AXIS2_PLACEMENT_3D('',#47997,#38306,#38307);
#34643=AXIS2_PLACEMENT_3D('',#47999,#38308,#38309);
#34644=AXIS2_PLACEMENT_3D('',#48001,#38310,#38311);
#34645=AXIS2_PLACEMENT_3D('',#48005,#38313,#38314);
#34646=AXIS2_PLACEMENT_3D('',#48007,#38315,#38316);
#34647=AXIS2_PLACEMENT_3D('',#48008,#38317,#38318);
#34648=AXIS2_PLACEMENT_3D('',#48013,#38320,#38321);
#34649=AXIS2_PLACEMENT_3D('',#48015,#38322,#38323);
#34650=AXIS2_PLACEMENT_3D('',#48017,#38324,#38325);
#34651=AXIS2_PLACEMENT_3D('',#48021,#38327,#38328);
#34652=AXIS2_PLACEMENT_3D('',#48023,#38329,#38330);
#34653=AXIS2_PLACEMENT_3D('',#48024,#38331,#38332);
#34654=AXIS2_PLACEMENT_3D('',#48029,#38334,#38335);
#34655=AXIS2_PLACEMENT_3D('',#48031,#38336,#38337);
#34656=AXIS2_PLACEMENT_3D('',#48033,#38338,#38339);
#34657=AXIS2_PLACEMENT_3D('',#48037,#38341,#38342);
#34658=AXIS2_PLACEMENT_3D('',#48039,#38343,#38344);
#34659=AXIS2_PLACEMENT_3D('',#48040,#38345,#38346);
#34660=AXIS2_PLACEMENT_3D('',#48045,#38348,#38349);
#34661=AXIS2_PLACEMENT_3D('',#48047,#38350,#38351);
#34662=AXIS2_PLACEMENT_3D('',#48049,#38352,#38353);
#34663=AXIS2_PLACEMENT_3D('',#48053,#38355,#38356);
#34664=AXIS2_PLACEMENT_3D('',#48055,#38357,#38358);
#34665=AXIS2_PLACEMENT_3D('',#48056,#38359,#38360);
#34666=AXIS2_PLACEMENT_3D('',#48061,#38362,#38363);
#34667=AXIS2_PLACEMENT_3D('',#48063,#38364,#38365);
#34668=AXIS2_PLACEMENT_3D('',#48065,#38366,#38367);
#34669=AXIS2_PLACEMENT_3D('',#48069,#38369,#38370);
#34670=AXIS2_PLACEMENT_3D('',#48071,#38371,#38372);
#34671=AXIS2_PLACEMENT_3D('',#48072,#38373,#38374);
#34672=AXIS2_PLACEMENT_3D('',#48077,#38376,#38377);
#34673=AXIS2_PLACEMENT_3D('',#48079,#38378,#38379);
#34674=AXIS2_PLACEMENT_3D('',#48081,#38380,#38381);
#34675=AXIS2_PLACEMENT_3D('',#48085,#38383,#38384);
#34676=AXIS2_PLACEMENT_3D('',#48087,#38385,#38386);
#34677=AXIS2_PLACEMENT_3D('',#48088,#38387,#38388);
#34678=AXIS2_PLACEMENT_3D('',#48093,#38390,#38391);
#34679=AXIS2_PLACEMENT_3D('',#48095,#38392,#38393);
#34680=AXIS2_PLACEMENT_3D('',#48097,#38394,#38395);
#34681=AXIS2_PLACEMENT_3D('',#48101,#38397,#38398);
#34682=AXIS2_PLACEMENT_3D('',#48103,#38399,#38400);
#34683=AXIS2_PLACEMENT_3D('',#48104,#38401,#38402);
#34684=AXIS2_PLACEMENT_3D('',#48109,#38404,#38405);
#34685=AXIS2_PLACEMENT_3D('',#48111,#38406,#38407);
#34686=AXIS2_PLACEMENT_3D('',#48113,#38408,#38409);
#34687=AXIS2_PLACEMENT_3D('',#48117,#38411,#38412);
#34688=AXIS2_PLACEMENT_3D('',#48119,#38413,#38414);
#34689=AXIS2_PLACEMENT_3D('',#48120,#38415,#38416);
#34690=AXIS2_PLACEMENT_3D('',#48125,#38418,#38419);
#34691=AXIS2_PLACEMENT_3D('',#48127,#38420,#38421);
#34692=AXIS2_PLACEMENT_3D('',#48129,#38422,#38423);
#34693=AXIS2_PLACEMENT_3D('',#48133,#38425,#38426);
#34694=AXIS2_PLACEMENT_3D('',#48135,#38427,#38428);
#34695=AXIS2_PLACEMENT_3D('',#48136,#38429,#38430);
#34696=AXIS2_PLACEMENT_3D('',#48141,#38432,#38433);
#34697=AXIS2_PLACEMENT_3D('',#48143,#38434,#38435);
#34698=AXIS2_PLACEMENT_3D('',#48145,#38436,#38437);
#34699=AXIS2_PLACEMENT_3D('',#48149,#38439,#38440);
#34700=AXIS2_PLACEMENT_3D('',#48151,#38441,#38442);
#34701=AXIS2_PLACEMENT_3D('',#48152,#38443,#38444);
#34702=AXIS2_PLACEMENT_3D('',#48157,#38446,#38447);
#34703=AXIS2_PLACEMENT_3D('',#48159,#38448,#38449);
#34704=AXIS2_PLACEMENT_3D('',#48161,#38450,#38451);
#34705=AXIS2_PLACEMENT_3D('',#48165,#38453,#38454);
#34706=AXIS2_PLACEMENT_3D('',#48167,#38455,#38456);
#34707=AXIS2_PLACEMENT_3D('',#48168,#38457,#38458);
#34708=AXIS2_PLACEMENT_3D('',#48173,#38460,#38461);
#34709=AXIS2_PLACEMENT_3D('',#48175,#38462,#38463);
#34710=AXIS2_PLACEMENT_3D('',#48177,#38464,#38465);
#34711=AXIS2_PLACEMENT_3D('',#48181,#38467,#38468);
#34712=AXIS2_PLACEMENT_3D('',#48183,#38469,#38470);
#34713=AXIS2_PLACEMENT_3D('',#48184,#38471,#38472);
#34714=AXIS2_PLACEMENT_3D('',#48189,#38474,#38475);
#34715=AXIS2_PLACEMENT_3D('',#48191,#38476,#38477);
#34716=AXIS2_PLACEMENT_3D('',#48193,#38478,#38479);
#34717=AXIS2_PLACEMENT_3D('',#48197,#38481,#38482);
#34718=AXIS2_PLACEMENT_3D('',#48199,#38483,#38484);
#34719=AXIS2_PLACEMENT_3D('',#48200,#38485,#38486);
#34720=AXIS2_PLACEMENT_3D('',#48205,#38488,#38489);
#34721=AXIS2_PLACEMENT_3D('',#48207,#38490,#38491);
#34722=AXIS2_PLACEMENT_3D('',#48209,#38492,#38493);
#34723=AXIS2_PLACEMENT_3D('',#48213,#38495,#38496);
#34724=AXIS2_PLACEMENT_3D('',#48215,#38497,#38498);
#34725=AXIS2_PLACEMENT_3D('',#48216,#38499,#38500);
#34726=AXIS2_PLACEMENT_3D('',#48221,#38502,#38503);
#34727=AXIS2_PLACEMENT_3D('',#48223,#38504,#38505);
#34728=AXIS2_PLACEMENT_3D('',#48225,#38506,#38507);
#34729=AXIS2_PLACEMENT_3D('',#48229,#38509,#38510);
#34730=AXIS2_PLACEMENT_3D('',#48231,#38511,#38512);
#34731=AXIS2_PLACEMENT_3D('',#48232,#38513,#38514);
#34732=AXIS2_PLACEMENT_3D('',#48237,#38516,#38517);
#34733=AXIS2_PLACEMENT_3D('',#48239,#38518,#38519);
#34734=AXIS2_PLACEMENT_3D('',#48241,#38520,#38521);
#34735=AXIS2_PLACEMENT_3D('',#48245,#38523,#38524);
#34736=AXIS2_PLACEMENT_3D('',#48247,#38525,#38526);
#34737=AXIS2_PLACEMENT_3D('',#48248,#38527,#38528);
#34738=AXIS2_PLACEMENT_3D('',#48253,#38530,#38531);
#34739=AXIS2_PLACEMENT_3D('',#48255,#38532,#38533);
#34740=AXIS2_PLACEMENT_3D('',#48257,#38534,#38535);
#34741=AXIS2_PLACEMENT_3D('',#48261,#38537,#38538);
#34742=AXIS2_PLACEMENT_3D('',#48263,#38539,#38540);
#34743=AXIS2_PLACEMENT_3D('',#48264,#38541,#38542);
#34744=AXIS2_PLACEMENT_3D('',#48269,#38544,#38545);
#34745=AXIS2_PLACEMENT_3D('',#48271,#38546,#38547);
#34746=AXIS2_PLACEMENT_3D('',#48273,#38548,#38549);
#34747=AXIS2_PLACEMENT_3D('',#48277,#38551,#38552);
#34748=AXIS2_PLACEMENT_3D('',#48279,#38553,#38554);
#34749=AXIS2_PLACEMENT_3D('',#48280,#38555,#38556);
#34750=AXIS2_PLACEMENT_3D('',#48285,#38558,#38559);
#34751=AXIS2_PLACEMENT_3D('',#48287,#38560,#38561);
#34752=AXIS2_PLACEMENT_3D('',#48289,#38562,#38563);
#34753=AXIS2_PLACEMENT_3D('',#48293,#38565,#38566);
#34754=AXIS2_PLACEMENT_3D('',#48295,#38567,#38568);
#34755=AXIS2_PLACEMENT_3D('',#48296,#38569,#38570);
#34756=AXIS2_PLACEMENT_3D('',#48301,#38572,#38573);
#34757=AXIS2_PLACEMENT_3D('',#48303,#38574,#38575);
#34758=AXIS2_PLACEMENT_3D('',#48305,#38576,#38577);
#34759=AXIS2_PLACEMENT_3D('',#48309,#38579,#38580);
#34760=AXIS2_PLACEMENT_3D('',#48311,#38581,#38582);
#34761=AXIS2_PLACEMENT_3D('',#48312,#38583,#38584);
#34762=AXIS2_PLACEMENT_3D('',#48317,#38586,#38587);
#34763=AXIS2_PLACEMENT_3D('',#48319,#38588,#38589);
#34764=AXIS2_PLACEMENT_3D('',#48321,#38590,#38591);
#34765=AXIS2_PLACEMENT_3D('',#48325,#38593,#38594);
#34766=AXIS2_PLACEMENT_3D('',#48327,#38595,#38596);
#34767=AXIS2_PLACEMENT_3D('',#48328,#38597,#38598);
#34768=AXIS2_PLACEMENT_3D('',#48333,#38600,#38601);
#34769=AXIS2_PLACEMENT_3D('',#48335,#38602,#38603);
#34770=AXIS2_PLACEMENT_3D('',#48337,#38604,#38605);
#34771=AXIS2_PLACEMENT_3D('',#48341,#38607,#38608);
#34772=AXIS2_PLACEMENT_3D('',#48343,#38609,#38610);
#34773=AXIS2_PLACEMENT_3D('',#48344,#38611,#38612);
#34774=AXIS2_PLACEMENT_3D('',#48349,#38614,#38615);
#34775=AXIS2_PLACEMENT_3D('',#48351,#38616,#38617);
#34776=AXIS2_PLACEMENT_3D('',#48353,#38618,#38619);
#34777=AXIS2_PLACEMENT_3D('',#48357,#38621,#38622);
#34778=AXIS2_PLACEMENT_3D('',#48359,#38623,#38624);
#34779=AXIS2_PLACEMENT_3D('',#48360,#38625,#38626);
#34780=AXIS2_PLACEMENT_3D('',#48365,#38628,#38629);
#34781=AXIS2_PLACEMENT_3D('',#48367,#38630,#38631);
#34782=AXIS2_PLACEMENT_3D('',#48369,#38632,#38633);
#34783=AXIS2_PLACEMENT_3D('',#48373,#38635,#38636);
#34784=AXIS2_PLACEMENT_3D('',#48375,#38637,#38638);
#34785=AXIS2_PLACEMENT_3D('',#48376,#38639,#38640);
#34786=AXIS2_PLACEMENT_3D('',#48381,#38642,#38643);
#34787=AXIS2_PLACEMENT_3D('',#48383,#38644,#38645);
#34788=AXIS2_PLACEMENT_3D('',#48385,#38646,#38647);
#34789=AXIS2_PLACEMENT_3D('',#48389,#38649,#38650);
#34790=AXIS2_PLACEMENT_3D('',#48391,#38651,#38652);
#34791=AXIS2_PLACEMENT_3D('',#48392,#38653,#38654);
#34792=AXIS2_PLACEMENT_3D('',#48397,#38656,#38657);
#34793=AXIS2_PLACEMENT_3D('',#48399,#38658,#38659);
#34794=AXIS2_PLACEMENT_3D('',#48401,#38660,#38661);
#34795=AXIS2_PLACEMENT_3D('',#48405,#38663,#38664);
#34796=AXIS2_PLACEMENT_3D('',#48407,#38665,#38666);
#34797=AXIS2_PLACEMENT_3D('',#48408,#38667,#38668);
#34798=AXIS2_PLACEMENT_3D('',#48413,#38670,#38671);
#34799=AXIS2_PLACEMENT_3D('',#48415,#38672,#38673);
#34800=AXIS2_PLACEMENT_3D('',#48417,#38674,#38675);
#34801=AXIS2_PLACEMENT_3D('',#48421,#38677,#38678);
#34802=AXIS2_PLACEMENT_3D('',#48423,#38679,#38680);
#34803=AXIS2_PLACEMENT_3D('',#48424,#38681,#38682);
#34804=AXIS2_PLACEMENT_3D('',#48429,#38684,#38685);
#34805=AXIS2_PLACEMENT_3D('',#48431,#38686,#38687);
#34806=AXIS2_PLACEMENT_3D('',#48433,#38688,#38689);
#34807=AXIS2_PLACEMENT_3D('',#48437,#38691,#38692);
#34808=AXIS2_PLACEMENT_3D('',#48439,#38693,#38694);
#34809=AXIS2_PLACEMENT_3D('',#48440,#38695,#38696);
#34810=AXIS2_PLACEMENT_3D('',#48445,#38698,#38699);
#34811=AXIS2_PLACEMENT_3D('',#48447,#38700,#38701);
#34812=AXIS2_PLACEMENT_3D('',#48449,#38702,#38703);
#34813=AXIS2_PLACEMENT_3D('',#48453,#38705,#38706);
#34814=AXIS2_PLACEMENT_3D('',#48455,#38707,#38708);
#34815=AXIS2_PLACEMENT_3D('',#48456,#38709,#38710);
#34816=AXIS2_PLACEMENT_3D('',#48461,#38712,#38713);
#34817=AXIS2_PLACEMENT_3D('',#48463,#38714,#38715);
#34818=AXIS2_PLACEMENT_3D('',#48465,#38716,#38717);
#34819=AXIS2_PLACEMENT_3D('',#48469,#38719,#38720);
#34820=AXIS2_PLACEMENT_3D('',#48471,#38721,#38722);
#34821=AXIS2_PLACEMENT_3D('',#48472,#38723,#38724);
#34822=AXIS2_PLACEMENT_3D('',#48477,#38726,#38727);
#34823=AXIS2_PLACEMENT_3D('',#48479,#38728,#38729);
#34824=AXIS2_PLACEMENT_3D('',#48481,#38730,#38731);
#34825=AXIS2_PLACEMENT_3D('',#48485,#38733,#38734);
#34826=AXIS2_PLACEMENT_3D('',#48487,#38735,#38736);
#34827=AXIS2_PLACEMENT_3D('',#48488,#38737,#38738);
#34828=AXIS2_PLACEMENT_3D('',#48493,#38740,#38741);
#34829=AXIS2_PLACEMENT_3D('',#48495,#38742,#38743);
#34830=AXIS2_PLACEMENT_3D('',#48497,#38744,#38745);
#34831=AXIS2_PLACEMENT_3D('',#48501,#38747,#38748);
#34832=AXIS2_PLACEMENT_3D('',#48503,#38749,#38750);
#34833=AXIS2_PLACEMENT_3D('',#48504,#38751,#38752);
#34834=AXIS2_PLACEMENT_3D('',#48509,#38754,#38755);
#34835=AXIS2_PLACEMENT_3D('',#48511,#38756,#38757);
#34836=AXIS2_PLACEMENT_3D('',#48513,#38758,#38759);
#34837=AXIS2_PLACEMENT_3D('',#48517,#38761,#38762);
#34838=AXIS2_PLACEMENT_3D('',#48519,#38763,#38764);
#34839=AXIS2_PLACEMENT_3D('',#48520,#38765,#38766);
#34840=AXIS2_PLACEMENT_3D('',#48525,#38768,#38769);
#34841=AXIS2_PLACEMENT_3D('',#48527,#38770,#38771);
#34842=AXIS2_PLACEMENT_3D('',#48529,#38772,#38773);
#34843=AXIS2_PLACEMENT_3D('',#48533,#38775,#38776);
#34844=AXIS2_PLACEMENT_3D('',#48535,#38777,#38778);
#34845=AXIS2_PLACEMENT_3D('',#48536,#38779,#38780);
#34846=AXIS2_PLACEMENT_3D('',#48541,#38782,#38783);
#34847=AXIS2_PLACEMENT_3D('',#48543,#38784,#38785);
#34848=AXIS2_PLACEMENT_3D('',#48545,#38786,#38787);
#34849=AXIS2_PLACEMENT_3D('',#48549,#38789,#38790);
#34850=AXIS2_PLACEMENT_3D('',#48551,#38791,#38792);
#34851=AXIS2_PLACEMENT_3D('',#48552,#38793,#38794);
#34852=AXIS2_PLACEMENT_3D('',#48557,#38796,#38797);
#34853=AXIS2_PLACEMENT_3D('',#48559,#38798,#38799);
#34854=AXIS2_PLACEMENT_3D('',#48561,#38800,#38801);
#34855=AXIS2_PLACEMENT_3D('',#48565,#38803,#38804);
#34856=AXIS2_PLACEMENT_3D('',#48567,#38805,#38806);
#34857=AXIS2_PLACEMENT_3D('',#48568,#38807,#38808);
#34858=AXIS2_PLACEMENT_3D('',#48573,#38810,#38811);
#34859=AXIS2_PLACEMENT_3D('',#48575,#38812,#38813);
#34860=AXIS2_PLACEMENT_3D('',#48577,#38814,#38815);
#34861=AXIS2_PLACEMENT_3D('',#48581,#38817,#38818);
#34862=AXIS2_PLACEMENT_3D('',#48583,#38819,#38820);
#34863=AXIS2_PLACEMENT_3D('',#48584,#38821,#38822);
#34864=AXIS2_PLACEMENT_3D('',#48585,#38823,#38824);
#34865=AXIS2_PLACEMENT_3D('',#48588,#38825,#38826);
#34866=AXIS2_PLACEMENT_3D('',#48595,#38827,#38828);
#34867=AXIS2_PLACEMENT_3D('',#48600,#38829,#38830);
#34868=AXIS2_PLACEMENT_3D('',#48602,#38831,#38832);
#34869=AXIS2_PLACEMENT_3D('',#48608,#38833,#38834);
#34870=AXIS2_PLACEMENT_3D('',#48609,#38835,#38836);
#34871=AXIS2_PLACEMENT_3D('',#48611,#38837,#38838);
#34872=AXIS2_PLACEMENT_3D('',#48617,#38839,#38840);
#34873=AXIS2_PLACEMENT_3D('',#48618,#38841,#38842);
#34874=AXIS2_PLACEMENT_3D('',#48620,#38843,#38844);
#34875=AXIS2_PLACEMENT_3D('',#48626,#38845,#38846);
#34876=AXIS2_PLACEMENT_3D('',#48627,#38847,#38848);
#34877=AXIS2_PLACEMENT_3D('',#48629,#38849,#38850);
#34878=AXIS2_PLACEMENT_3D('',#48635,#38851,#38852);
#34879=AXIS2_PLACEMENT_3D('',#48636,#38853,#38854);
#34880=AXIS2_PLACEMENT_3D('',#48638,#38855,#38856);
#34881=AXIS2_PLACEMENT_3D('',#48644,#38857,#38858);
#34882=AXIS2_PLACEMENT_3D('',#48645,#38859,#38860);
#34883=AXIS2_PLACEMENT_3D('',#48647,#38861,#38862);
#34884=AXIS2_PLACEMENT_3D('',#48649,#38863,#38864);
#34885=AXIS2_PLACEMENT_3D('',#48654,#38865,#38866);
#34886=AXIS2_PLACEMENT_3D('',#48656,#38867,#38868);
#34887=AXIS2_PLACEMENT_3D('',#48658,#38869,#38870);
#34888=AXIS2_PLACEMENT_3D('',#48663,#38871,#38872);
#34889=AXIS2_PLACEMENT_3D('',#48665,#38873,#38874);
#34890=AXIS2_PLACEMENT_3D('',#48667,#38875,#38876);
#34891=AXIS2_PLACEMENT_3D('',#48672,#38877,#38878);
#34892=AXIS2_PLACEMENT_3D('',#48673,#38879,#38880);
#34893=AXIS2_PLACEMENT_3D('',#48674,#38881,#38882);
#34894=AXIS2_PLACEMENT_3D('',#48675,#38883,#38884);
#34895=AXIS2_PLACEMENT_3D('',#48679,#38886,#38887);
#34896=AXIS2_PLACEMENT_3D('',#48681,#38889,#38890);
#34897=AXIS2_PLACEMENT_3D('',#48684,#38892,#38893);
#34898=AXIS2_PLACEMENT_3D('',#48685,#38894,#38895);
#34899=AXIS2_PLACEMENT_3D('',#48688,#38897,#38898);
#34900=AXIS2_PLACEMENT_3D('',#48689,#38899,#38900);
#34901=AXIS2_PLACEMENT_3D('',#48692,#38902,#38903);
#34902=AXIS2_PLACEMENT_3D('',#48693,#38904,#38905);
#34903=AXIS2_PLACEMENT_3D('',#48696,#38907,#38908);
#34904=AXIS2_PLACEMENT_3D('',#48697,#38909,#38910);
#34905=AXIS2_PLACEMENT_3D('',#48700,#38912,#38913);
#34906=AXIS2_PLACEMENT_3D('',#48701,#38914,#38915);
#34907=AXIS2_PLACEMENT_3D('',#48703,#38916,#38917);
#34908=AXIS2_PLACEMENT_3D('',#48705,#38918,#38919);
#34909=AXIS2_PLACEMENT_3D('',#48707,#38920,#38921);
#34910=AXIS2_PLACEMENT_3D('',#48709,#38922,#38923);
#34911=AXIS2_PLACEMENT_3D('',#48711,#38924,#38925);
#34912=AXIS2_PLACEMENT_3D('',#48712,#38926,#38927);
#34913=AXIS2_PLACEMENT_3D('',#48720,#38932,#38933);
#34914=AXIS2_PLACEMENT_3D('',#48724,#38936,#38937);
#34915=AXIS2_PLACEMENT_3D('',#48730,#38941,#38942);
#34916=AXIS2_PLACEMENT_3D('',#48736,#38946,#38947);
#34917=AXIS2_PLACEMENT_3D('',#48740,#38950,#38951);
#34918=AXIS2_PLACEMENT_3D('',#48744,#38954,#38955);
#34919=AXIS2_PLACEMENT_3D('',#48747,#38958,#38959);
#34920=AXIS2_PLACEMENT_3D('',#48754,#38963,#38964);
#34921=AXIS2_PLACEMENT_3D('',#48757,#38967,#38968);
#34922=AXIS2_PLACEMENT_3D('',#48760,#38971,#38972);
#34923=AXIS2_PLACEMENT_3D('',#48763,#38975,#38976);
#34924=AXIS2_PLACEMENT_3D('',#48765,#38978,#38979);
#34925=AXIS2_PLACEMENT_3D('',#48766,#38980,#38981);
#34926=AXIS2_PLACEMENT_3D('',#48767,#38982,#38983);
#34927=AXIS2_PLACEMENT_3D('',#48774,#38987,#38988);
#34928=AXIS2_PLACEMENT_3D('',#48781,#38992,#38993);
#34929=AXIS2_PLACEMENT_3D('',#48788,#38997,#38998);
#34930=AXIS2_PLACEMENT_3D('',#48791,#39001,#39002);
#34931=AXIS2_PLACEMENT_3D('',#48798,#39006,#39007);
#34932=AXIS2_PLACEMENT_3D('',#48801,#39010,#39011);
#34933=AXIS2_PLACEMENT_3D('',#48804,#39014,#39015);
#34934=AXIS2_PLACEMENT_3D('',#48807,#39018,#39019);
#34935=AXIS2_PLACEMENT_3D('',#48810,#39022,#39023);
#34936=AXIS2_PLACEMENT_3D('',#48813,#39026,#39027);
#34937=AXIS2_PLACEMENT_3D('',#48816,#39030,#39031);
#34938=AXIS2_PLACEMENT_3D('',#48819,#39034,#39035);
#34939=AXIS2_PLACEMENT_3D('',#48820,#39036,#39037);
#34940=AXIS2_PLACEMENT_3D('',#48821,#39038,#39039);
#34941=AXIS2_PLACEMENT_3D('',#48822,#39040,#39041);
#34942=AXIS2_PLACEMENT_3D('',#48829,#39045,#39046);
#34943=AXIS2_PLACEMENT_3D('',#48837,#39051,#39052);
#34944=AXIS2_PLACEMENT_3D('',#48840,#39055,#39056);
#34945=AXIS2_PLACEMENT_3D('',#48847,#39060,#39061);
#34946=AXIS2_PLACEMENT_3D('',#48855,#39066,#39067);
#34947=AXIS2_PLACEMENT_3D('',#48858,#39070,#39071);
#34948=AXIS2_PLACEMENT_3D('',#48861,#39074,#39075);
#34949=AXIS2_PLACEMENT_3D('',#48866,#39079,#39080);
#34950=AXIS2_PLACEMENT_3D('',#48868,#39082,#39083);
#34951=AXIS2_PLACEMENT_3D('',#48872,#39086,#39087);
#34952=AXIS2_PLACEMENT_3D('',#48875,#39090,#39091);
#34953=AXIS2_PLACEMENT_3D('',#48876,#39092,#39093);
#34954=AXIS2_PLACEMENT_3D('',#48877,#39094,#39095);
#34955=AXIS2_PLACEMENT_3D('',#48884,#39099,#39100);
#34956=AXIS2_PLACEMENT_3D('',#48891,#39104,#39105);
#34957=AXIS2_PLACEMENT_3D('',#48898,#39109,#39110);
#34958=AXIS2_PLACEMENT_3D('',#48901,#39113,#39114);
#34959=AXIS2_PLACEMENT_3D('',#48908,#39118,#39119);
#34960=AXIS2_PLACEMENT_3D('',#48911,#39122,#39123);
#34961=AXIS2_PLACEMENT_3D('',#48914,#39126,#39127);
#34962=AXIS2_PLACEMENT_3D('',#48917,#39130,#39131);
#34963=AXIS2_PLACEMENT_3D('',#48920,#39134,#39135);
#34964=AXIS2_PLACEMENT_3D('',#48923,#39138,#39139);
#34965=AXIS2_PLACEMENT_3D('',#48926,#39142,#39143);
#34966=AXIS2_PLACEMENT_3D('',#48929,#39146,#39147);
#34967=AXIS2_PLACEMENT_3D('',#48930,#39148,#39149);
#34968=AXIS2_PLACEMENT_3D('',#48931,#39150,#39151);
#34969=AXIS2_PLACEMENT_3D('',#48932,#39152,#39153);
#34970=AXIS2_PLACEMENT_3D('',#48939,#39157,#39158);
#34971=AXIS2_PLACEMENT_3D('',#48946,#39162,#39163);
#34972=AXIS2_PLACEMENT_3D('',#48953,#39167,#39168);
#34973=AXIS2_PLACEMENT_3D('',#48956,#39171,#39172);
#34974=AXIS2_PLACEMENT_3D('',#48963,#39176,#39177);
#34975=AXIS2_PLACEMENT_3D('',#48966,#39180,#39181);
#34976=AXIS2_PLACEMENT_3D('',#48969,#39184,#39185);
#34977=AXIS2_PLACEMENT_3D('',#48972,#39188,#39189);
#34978=AXIS2_PLACEMENT_3D('',#48975,#39192,#39193);
#34979=AXIS2_PLACEMENT_3D('',#48978,#39196,#39197);
#34980=AXIS2_PLACEMENT_3D('',#48981,#39200,#39201);
#34981=AXIS2_PLACEMENT_3D('',#48984,#39204,#39205);
#34982=AXIS2_PLACEMENT_3D('',#48985,#39206,#39207);
#34983=AXIS2_PLACEMENT_3D('',#48986,#39208,#39209);
#34984=AXIS2_PLACEMENT_3D('',#48987,#39210,#39211);
#34985=AXIS2_PLACEMENT_3D('',#48995,#39216,#39217);
#34986=AXIS2_PLACEMENT_3D('',#48999,#39220,#39221);
#34987=AXIS2_PLACEMENT_3D('',#49005,#39225,#39226);
#34988=AXIS2_PLACEMENT_3D('',#49011,#39230,#39231);
#34989=AXIS2_PLACEMENT_3D('',#49015,#39234,#39235);
#34990=AXIS2_PLACEMENT_3D('',#49019,#39238,#39239);
#34991=AXIS2_PLACEMENT_3D('',#49022,#39242,#39243);
#34992=AXIS2_PLACEMENT_3D('',#49029,#39247,#39248);
#34993=AXIS2_PLACEMENT_3D('',#49032,#39251,#39252);
#34994=AXIS2_PLACEMENT_3D('',#49035,#39255,#39256);
#34995=AXIS2_PLACEMENT_3D('',#49038,#39259,#39260);
#34996=AXIS2_PLACEMENT_3D('',#49040,#39262,#39263);
#34997=AXIS2_PLACEMENT_3D('',#49041,#39264,#39265);
#34998=AXIS2_PLACEMENT_3D('',#49042,#39266,#39267);
#34999=AXIS2_PLACEMENT_3D('',#49049,#39271,#39272);
#35000=AXIS2_PLACEMENT_3D('',#49056,#39276,#39277);
#35001=AXIS2_PLACEMENT_3D('',#49063,#39281,#39282);
#35002=AXIS2_PLACEMENT_3D('',#49066,#39285,#39286);
#35003=AXIS2_PLACEMENT_3D('',#49073,#39290,#39291);
#35004=AXIS2_PLACEMENT_3D('',#49076,#39294,#39295);
#35005=AXIS2_PLACEMENT_3D('',#49079,#39298,#39299);
#35006=AXIS2_PLACEMENT_3D('',#49082,#39302,#39303);
#35007=AXIS2_PLACEMENT_3D('',#49085,#39306,#39307);
#35008=AXIS2_PLACEMENT_3D('',#49088,#39310,#39311);
#35009=AXIS2_PLACEMENT_3D('',#49091,#39314,#39315);
#35010=AXIS2_PLACEMENT_3D('',#49094,#39318,#39319);
#35011=AXIS2_PLACEMENT_3D('',#49095,#39320,#39321);
#35012=AXIS2_PLACEMENT_3D('',#49096,#39322,#39323);
#35013=AXIS2_PLACEMENT_3D('',#49097,#39324,#39325);
#35014=AXIS2_PLACEMENT_3D('',#49104,#39329,#39330);
#35015=AXIS2_PLACEMENT_3D('',#49112,#39335,#39336);
#35016=AXIS2_PLACEMENT_3D('',#49115,#39339,#39340);
#35017=AXIS2_PLACEMENT_3D('',#49122,#39344,#39345);
#35018=AXIS2_PLACEMENT_3D('',#49130,#39350,#39351);
#35019=AXIS2_PLACEMENT_3D('',#49133,#39354,#39355);
#35020=AXIS2_PLACEMENT_3D('',#49136,#39358,#39359);
#35021=AXIS2_PLACEMENT_3D('',#49141,#39363,#39364);
#35022=AXIS2_PLACEMENT_3D('',#49143,#39366,#39367);
#35023=AXIS2_PLACEMENT_3D('',#49147,#39370,#39371);
#35024=AXIS2_PLACEMENT_3D('',#49150,#39374,#39375);
#35025=AXIS2_PLACEMENT_3D('',#49151,#39376,#39377);
#35026=AXIS2_PLACEMENT_3D('',#49152,#39378,#39379);
#35027=AXIS2_PLACEMENT_3D('',#49159,#39383,#39384);
#35028=AXIS2_PLACEMENT_3D('',#49166,#39388,#39389);
#35029=AXIS2_PLACEMENT_3D('',#49173,#39393,#39394);
#35030=AXIS2_PLACEMENT_3D('',#49176,#39397,#39398);
#35031=AXIS2_PLACEMENT_3D('',#49183,#39402,#39403);
#35032=AXIS2_PLACEMENT_3D('',#49186,#39406,#39407);
#35033=AXIS2_PLACEMENT_3D('',#49189,#39410,#39411);
#35034=AXIS2_PLACEMENT_3D('',#49192,#39414,#39415);
#35035=AXIS2_PLACEMENT_3D('',#49195,#39418,#39419);
#35036=AXIS2_PLACEMENT_3D('',#49198,#39422,#39423);
#35037=AXIS2_PLACEMENT_3D('',#49201,#39426,#39427);
#35038=AXIS2_PLACEMENT_3D('',#49204,#39430,#39431);
#35039=AXIS2_PLACEMENT_3D('',#49205,#39432,#39433);
#35040=AXIS2_PLACEMENT_3D('',#49206,#39434,#39435);
#35041=AXIS2_PLACEMENT_3D('',#49207,#39436,#39437);
#35042=AXIS2_PLACEMENT_3D('',#49214,#39441,#39442);
#35043=AXIS2_PLACEMENT_3D('',#49221,#39446,#39447);
#35044=AXIS2_PLACEMENT_3D('',#49228,#39451,#39452);
#35045=AXIS2_PLACEMENT_3D('',#49231,#39455,#39456);
#35046=AXIS2_PLACEMENT_3D('',#49238,#39460,#39461);
#35047=AXIS2_PLACEMENT_3D('',#49241,#39464,#39465);
#35048=AXIS2_PLACEMENT_3D('',#49244,#39468,#39469);
#35049=AXIS2_PLACEMENT_3D('',#49247,#39472,#39473);
#35050=AXIS2_PLACEMENT_3D('',#49250,#39476,#39477);
#35051=AXIS2_PLACEMENT_3D('',#49253,#39480,#39481);
#35052=AXIS2_PLACEMENT_3D('',#49256,#39484,#39485);
#35053=AXIS2_PLACEMENT_3D('',#49259,#39488,#39489);
#35054=AXIS2_PLACEMENT_3D('',#49260,#39490,#39491);
#35055=AXIS2_PLACEMENT_3D('',#49261,#39492,#39493);
#35056=AXIS2_PLACEMENT_3D('',#49262,#39494,#39495);
#35057=AXIS2_PLACEMENT_3D('',#49270,#39500,#39501);
#35058=AXIS2_PLACEMENT_3D('',#49274,#39504,#39505);
#35059=AXIS2_PLACEMENT_3D('',#49280,#39509,#39510);
#35060=AXIS2_PLACEMENT_3D('',#49286,#39514,#39515);
#35061=AXIS2_PLACEMENT_3D('',#49290,#39518,#39519);
#35062=AXIS2_PLACEMENT_3D('',#49294,#39522,#39523);
#35063=AXIS2_PLACEMENT_3D('',#49297,#39526,#39527);
#35064=AXIS2_PLACEMENT_3D('',#49304,#39531,#39532);
#35065=AXIS2_PLACEMENT_3D('',#49307,#39535,#39536);
#35066=AXIS2_PLACEMENT_3D('',#49310,#39539,#39540);
#35067=AXIS2_PLACEMENT_3D('',#49313,#39543,#39544);
#35068=AXIS2_PLACEMENT_3D('',#49315,#39546,#39547);
#35069=AXIS2_PLACEMENT_3D('',#49316,#39548,#39549);
#35070=AXIS2_PLACEMENT_3D('',#49317,#39550,#39551);
#35071=AXIS2_PLACEMENT_3D('',#49324,#39555,#39556);
#35072=AXIS2_PLACEMENT_3D('',#49331,#39560,#39561);
#35073=AXIS2_PLACEMENT_3D('',#49338,#39565,#39566);
#35074=AXIS2_PLACEMENT_3D('',#49341,#39569,#39570);
#35075=AXIS2_PLACEMENT_3D('',#49348,#39574,#39575);
#35076=AXIS2_PLACEMENT_3D('',#49351,#39578,#39579);
#35077=AXIS2_PLACEMENT_3D('',#49354,#39582,#39583);
#35078=AXIS2_PLACEMENT_3D('',#49357,#39586,#39587);
#35079=AXIS2_PLACEMENT_3D('',#49360,#39590,#39591);
#35080=AXIS2_PLACEMENT_3D('',#49363,#39594,#39595);
#35081=AXIS2_PLACEMENT_3D('',#49366,#39598,#39599);
#35082=AXIS2_PLACEMENT_3D('',#49369,#39602,#39603);
#35083=AXIS2_PLACEMENT_3D('',#49370,#39604,#39605);
#35084=AXIS2_PLACEMENT_3D('',#49371,#39606,#39607);
#35085=AXIS2_PLACEMENT_3D('',#49372,#39608,#39609);
#35086=AXIS2_PLACEMENT_3D('',#49379,#39613,#39614);
#35087=AXIS2_PLACEMENT_3D('',#49387,#39619,#39620);
#35088=AXIS2_PLACEMENT_3D('',#49390,#39623,#39624);
#35089=AXIS2_PLACEMENT_3D('',#49397,#39628,#39629);
#35090=AXIS2_PLACEMENT_3D('',#49405,#39634,#39635);
#35091=AXIS2_PLACEMENT_3D('',#49408,#39638,#39639);
#35092=AXIS2_PLACEMENT_3D('',#49411,#39642,#39643);
#35093=AXIS2_PLACEMENT_3D('',#49416,#39647,#39648);
#35094=AXIS2_PLACEMENT_3D('',#49418,#39650,#39651);
#35095=AXIS2_PLACEMENT_3D('',#49422,#39654,#39655);
#35096=AXIS2_PLACEMENT_3D('',#49425,#39658,#39659);
#35097=AXIS2_PLACEMENT_3D('',#49426,#39660,#39661);
#35098=AXIS2_PLACEMENT_3D('',#49427,#39662,#39663);
#35099=AXIS2_PLACEMENT_3D('',#49434,#39667,#39668);
#35100=AXIS2_PLACEMENT_3D('',#49441,#39672,#39673);
#35101=AXIS2_PLACEMENT_3D('',#49448,#39677,#39678);
#35102=AXIS2_PLACEMENT_3D('',#49451,#39681,#39682);
#35103=AXIS2_PLACEMENT_3D('',#49458,#39686,#39687);
#35104=AXIS2_PLACEMENT_3D('',#49461,#39690,#39691);
#35105=AXIS2_PLACEMENT_3D('',#49464,#39694,#39695);
#35106=AXIS2_PLACEMENT_3D('',#49467,#39698,#39699);
#35107=AXIS2_PLACEMENT_3D('',#49470,#39702,#39703);
#35108=AXIS2_PLACEMENT_3D('',#49473,#39706,#39707);
#35109=AXIS2_PLACEMENT_3D('',#49476,#39710,#39711);
#35110=AXIS2_PLACEMENT_3D('',#49479,#39714,#39715);
#35111=AXIS2_PLACEMENT_3D('',#49480,#39716,#39717);
#35112=AXIS2_PLACEMENT_3D('',#49481,#39718,#39719);
#35113=AXIS2_PLACEMENT_3D('',#49482,#39720,#39721);
#35114=AXIS2_PLACEMENT_3D('',#49489,#39725,#39726);
#35115=AXIS2_PLACEMENT_3D('',#49496,#39730,#39731);
#35116=AXIS2_PLACEMENT_3D('',#49503,#39735,#39736);
#35117=AXIS2_PLACEMENT_3D('',#49506,#39739,#39740);
#35118=AXIS2_PLACEMENT_3D('',#49513,#39744,#39745);
#35119=AXIS2_PLACEMENT_3D('',#49516,#39748,#39749);
#35120=AXIS2_PLACEMENT_3D('',#49519,#39752,#39753);
#35121=AXIS2_PLACEMENT_3D('',#49522,#39756,#39757);
#35122=AXIS2_PLACEMENT_3D('',#49525,#39760,#39761);
#35123=AXIS2_PLACEMENT_3D('',#49528,#39764,#39765);
#35124=AXIS2_PLACEMENT_3D('',#49531,#39768,#39769);
#35125=AXIS2_PLACEMENT_3D('',#49534,#39772,#39773);
#35126=AXIS2_PLACEMENT_3D('',#49535,#39774,#39775);
#35127=AXIS2_PLACEMENT_3D('',#49536,#39776,#39777);
#35128=AXIS2_PLACEMENT_3D('',#49537,#39778,#39779);
#35129=AXIS2_PLACEMENT_3D('',#49545,#39784,#39785);
#35130=AXIS2_PLACEMENT_3D('',#49549,#39788,#39789);
#35131=AXIS2_PLACEMENT_3D('',#49555,#39793,#39794);
#35132=AXIS2_PLACEMENT_3D('',#49561,#39798,#39799);
#35133=AXIS2_PLACEMENT_3D('',#49565,#39802,#39803);
#35134=AXIS2_PLACEMENT_3D('',#49569,#39806,#39807);
#35135=AXIS2_PLACEMENT_3D('',#49572,#39810,#39811);
#35136=AXIS2_PLACEMENT_3D('',#49579,#39815,#39816);
#35137=AXIS2_PLACEMENT_3D('',#49582,#39819,#39820);
#35138=AXIS2_PLACEMENT_3D('',#49585,#39823,#39824);
#35139=AXIS2_PLACEMENT_3D('',#49588,#39827,#39828);
#35140=AXIS2_PLACEMENT_3D('',#49590,#39830,#39831);
#35141=AXIS2_PLACEMENT_3D('',#49591,#39832,#39833);
#35142=AXIS2_PLACEMENT_3D('',#49592,#39834,#39835);
#35143=AXIS2_PLACEMENT_3D('',#49599,#39839,#39840);
#35144=AXIS2_PLACEMENT_3D('',#49606,#39844,#39845);
#35145=AXIS2_PLACEMENT_3D('',#49613,#39849,#39850);
#35146=AXIS2_PLACEMENT_3D('',#49616,#39853,#39854);
#35147=AXIS2_PLACEMENT_3D('',#49623,#39858,#39859);
#35148=AXIS2_PLACEMENT_3D('',#49626,#39862,#39863);
#35149=AXIS2_PLACEMENT_3D('',#49629,#39866,#39867);
#35150=AXIS2_PLACEMENT_3D('',#49632,#39870,#39871);
#35151=AXIS2_PLACEMENT_3D('',#49635,#39874,#39875);
#35152=AXIS2_PLACEMENT_3D('',#49638,#39878,#39879);
#35153=AXIS2_PLACEMENT_3D('',#49641,#39882,#39883);
#35154=AXIS2_PLACEMENT_3D('',#49644,#39886,#39887);
#35155=AXIS2_PLACEMENT_3D('',#49645,#39888,#39889);
#35156=AXIS2_PLACEMENT_3D('',#49646,#39890,#39891);
#35157=AXIS2_PLACEMENT_3D('',#49647,#39892,#39893);
#35158=AXIS2_PLACEMENT_3D('',#49654,#39897,#39898);
#35159=AXIS2_PLACEMENT_3D('',#49662,#39903,#39904);
#35160=AXIS2_PLACEMENT_3D('',#49665,#39907,#39908);
#35161=AXIS2_PLACEMENT_3D('',#49672,#39912,#39913);
#35162=AXIS2_PLACEMENT_3D('',#49680,#39918,#39919);
#35163=AXIS2_PLACEMENT_3D('',#49683,#39922,#39923);
#35164=AXIS2_PLACEMENT_3D('',#49686,#39926,#39927);
#35165=AXIS2_PLACEMENT_3D('',#49691,#39931,#39932);
#35166=AXIS2_PLACEMENT_3D('',#49693,#39934,#39935);
#35167=AXIS2_PLACEMENT_3D('',#49697,#39938,#39939);
#35168=AXIS2_PLACEMENT_3D('',#49700,#39942,#39943);
#35169=AXIS2_PLACEMENT_3D('',#49701,#39944,#39945);
#35170=AXIS2_PLACEMENT_3D('',#49702,#39946,#39947);
#35171=AXIS2_PLACEMENT_3D('',#49709,#39951,#39952);
#35172=AXIS2_PLACEMENT_3D('',#49716,#39956,#39957);
#35173=AXIS2_PLACEMENT_3D('',#49723,#39961,#39962);
#35174=AXIS2_PLACEMENT_3D('',#49726,#39965,#39966);
#35175=AXIS2_PLACEMENT_3D('',#49733,#39970,#39971);
#35176=AXIS2_PLACEMENT_3D('',#49736,#39974,#39975);
#35177=AXIS2_PLACEMENT_3D('',#49739,#39978,#39979);
#35178=AXIS2_PLACEMENT_3D('',#49742,#39982,#39983);
#35179=AXIS2_PLACEMENT_3D('',#49745,#39986,#39987);
#35180=AXIS2_PLACEMENT_3D('',#49748,#39990,#39991);
#35181=AXIS2_PLACEMENT_3D('',#49751,#39994,#39995);
#35182=AXIS2_PLACEMENT_3D('',#49754,#39998,#39999);
#35183=AXIS2_PLACEMENT_3D('',#49755,#40000,#40001);
#35184=AXIS2_PLACEMENT_3D('',#49756,#40002,#40003);
#35185=AXIS2_PLACEMENT_3D('',#49757,#40004,#40005);
#35186=AXIS2_PLACEMENT_3D('',#49764,#40009,#40010);
#35187=AXIS2_PLACEMENT_3D('',#49771,#40014,#40015);
#35188=AXIS2_PLACEMENT_3D('',#49778,#40019,#40020);
#35189=AXIS2_PLACEMENT_3D('',#49781,#40023,#40024);
#35190=AXIS2_PLACEMENT_3D('',#49788,#40028,#40029);
#35191=AXIS2_PLACEMENT_3D('',#49791,#40032,#40033);
#35192=AXIS2_PLACEMENT_3D('',#49794,#40036,#40037);
#35193=AXIS2_PLACEMENT_3D('',#49797,#40040,#40041);
#35194=AXIS2_PLACEMENT_3D('',#49800,#40044,#40045);
#35195=AXIS2_PLACEMENT_3D('',#49803,#40048,#40049);
#35196=AXIS2_PLACEMENT_3D('',#49806,#40052,#40053);
#35197=AXIS2_PLACEMENT_3D('',#49809,#40056,#40057);
#35198=AXIS2_PLACEMENT_3D('',#49810,#40058,#40059);
#35199=AXIS2_PLACEMENT_3D('',#49811,#40060,#40061);
#35200=AXIS2_PLACEMENT_3D('',#49812,#40062,#40063);
#35201=AXIS2_PLACEMENT_3D('',#49820,#40068,#40069);
#35202=AXIS2_PLACEMENT_3D('',#49824,#40072,#40073);
#35203=AXIS2_PLACEMENT_3D('',#49830,#40077,#40078);
#35204=AXIS2_PLACEMENT_3D('',#49836,#40082,#40083);
#35205=AXIS2_PLACEMENT_3D('',#49840,#40086,#40087);
#35206=AXIS2_PLACEMENT_3D('',#49844,#40090,#40091);
#35207=AXIS2_PLACEMENT_3D('',#49847,#40094,#40095);
#35208=AXIS2_PLACEMENT_3D('',#49854,#40099,#40100);
#35209=AXIS2_PLACEMENT_3D('',#49857,#40103,#40104);
#35210=AXIS2_PLACEMENT_3D('',#49860,#40107,#40108);
#35211=AXIS2_PLACEMENT_3D('',#49863,#40111,#40112);
#35212=AXIS2_PLACEMENT_3D('',#49865,#40114,#40115);
#35213=AXIS2_PLACEMENT_3D('',#49866,#40116,#40117);
#35214=AXIS2_PLACEMENT_3D('',#49867,#40118,#40119);
#35215=AXIS2_PLACEMENT_3D('',#49874,#40123,#40124);
#35216=AXIS2_PLACEMENT_3D('',#49881,#40128,#40129);
#35217=AXIS2_PLACEMENT_3D('',#49888,#40133,#40134);
#35218=AXIS2_PLACEMENT_3D('',#49891,#40137,#40138);
#35219=AXIS2_PLACEMENT_3D('',#49898,#40142,#40143);
#35220=AXIS2_PLACEMENT_3D('',#49901,#40146,#40147);
#35221=AXIS2_PLACEMENT_3D('',#49904,#40150,#40151);
#35222=AXIS2_PLACEMENT_3D('',#49907,#40154,#40155);
#35223=AXIS2_PLACEMENT_3D('',#49910,#40158,#40159);
#35224=AXIS2_PLACEMENT_3D('',#49913,#40162,#40163);
#35225=AXIS2_PLACEMENT_3D('',#49916,#40166,#40167);
#35226=AXIS2_PLACEMENT_3D('',#49919,#40170,#40171);
#35227=AXIS2_PLACEMENT_3D('',#49920,#40172,#40173);
#35228=AXIS2_PLACEMENT_3D('',#49921,#40174,#40175);
#35229=AXIS2_PLACEMENT_3D('',#49922,#40176,#40177);
#35230=AXIS2_PLACEMENT_3D('',#49929,#40181,#40182);
#35231=AXIS2_PLACEMENT_3D('',#49937,#40187,#40188);
#35232=AXIS2_PLACEMENT_3D('',#49940,#40191,#40192);
#35233=AXIS2_PLACEMENT_3D('',#49947,#40196,#40197);
#35234=AXIS2_PLACEMENT_3D('',#49955,#40202,#40203);
#35235=AXIS2_PLACEMENT_3D('',#49958,#40206,#40207);
#35236=AXIS2_PLACEMENT_3D('',#49961,#40210,#40211);
#35237=AXIS2_PLACEMENT_3D('',#49966,#40215,#40216);
#35238=AXIS2_PLACEMENT_3D('',#49968,#40218,#40219);
#35239=AXIS2_PLACEMENT_3D('',#49972,#40222,#40223);
#35240=AXIS2_PLACEMENT_3D('',#49975,#40226,#40227);
#35241=AXIS2_PLACEMENT_3D('',#49976,#40228,#40229);
#35242=AXIS2_PLACEMENT_3D('',#49977,#40230,#40231);
#35243=AXIS2_PLACEMENT_3D('',#49984,#40235,#40236);
#35244=AXIS2_PLACEMENT_3D('',#49991,#40240,#40241);
#35245=AXIS2_PLACEMENT_3D('',#49998,#40245,#40246);
#35246=AXIS2_PLACEMENT_3D('',#50001,#40249,#40250);
#35247=AXIS2_PLACEMENT_3D('',#50008,#40254,#40255);
#35248=AXIS2_PLACEMENT_3D('',#50011,#40258,#40259);
#35249=AXIS2_PLACEMENT_3D('',#50014,#40262,#40263);
#35250=AXIS2_PLACEMENT_3D('',#50017,#40266,#40267);
#35251=AXIS2_PLACEMENT_3D('',#50020,#40270,#40271);
#35252=AXIS2_PLACEMENT_3D('',#50023,#40274,#40275);
#35253=AXIS2_PLACEMENT_3D('',#50026,#40278,#40279);
#35254=AXIS2_PLACEMENT_3D('',#50029,#40282,#40283);
#35255=AXIS2_PLACEMENT_3D('',#50030,#40284,#40285);
#35256=AXIS2_PLACEMENT_3D('',#50031,#40286,#40287);
#35257=AXIS2_PLACEMENT_3D('',#50032,#40288,#40289);
#35258=AXIS2_PLACEMENT_3D('',#50039,#40293,#40294);
#35259=AXIS2_PLACEMENT_3D('',#50046,#40298,#40299);
#35260=AXIS2_PLACEMENT_3D('',#50053,#40303,#40304);
#35261=AXIS2_PLACEMENT_3D('',#50056,#40307,#40308);
#35262=AXIS2_PLACEMENT_3D('',#50063,#40312,#40313);
#35263=AXIS2_PLACEMENT_3D('',#50066,#40316,#40317);
#35264=AXIS2_PLACEMENT_3D('',#50069,#40320,#40321);
#35265=AXIS2_PLACEMENT_3D('',#50072,#40324,#40325);
#35266=AXIS2_PLACEMENT_3D('',#50075,#40328,#40329);
#35267=AXIS2_PLACEMENT_3D('',#50078,#40332,#40333);
#35268=AXIS2_PLACEMENT_3D('',#50081,#40336,#40337);
#35269=AXIS2_PLACEMENT_3D('',#50084,#40340,#40341);
#35270=AXIS2_PLACEMENT_3D('',#50085,#40342,#40343);
#35271=AXIS2_PLACEMENT_3D('',#50086,#40344,#40345);
#35272=AXIS2_PLACEMENT_3D('',#50087,#40346,#40347);
#35273=AXIS2_PLACEMENT_3D('',#50095,#40352,#40353);
#35274=AXIS2_PLACEMENT_3D('',#50099,#40356,#40357);
#35275=AXIS2_PLACEMENT_3D('',#50105,#40361,#40362);
#35276=AXIS2_PLACEMENT_3D('',#50111,#40366,#40367);
#35277=AXIS2_PLACEMENT_3D('',#50115,#40370,#40371);
#35278=AXIS2_PLACEMENT_3D('',#50119,#40374,#40375);
#35279=AXIS2_PLACEMENT_3D('',#50122,#40378,#40379);
#35280=AXIS2_PLACEMENT_3D('',#50129,#40383,#40384);
#35281=AXIS2_PLACEMENT_3D('',#50132,#40387,#40388);
#35282=AXIS2_PLACEMENT_3D('',#50135,#40391,#40392);
#35283=AXIS2_PLACEMENT_3D('',#50138,#40395,#40396);
#35284=AXIS2_PLACEMENT_3D('',#50140,#40398,#40399);
#35285=AXIS2_PLACEMENT_3D('',#50141,#40400,#40401);
#35286=AXIS2_PLACEMENT_3D('',#50142,#40402,#40403);
#35287=AXIS2_PLACEMENT_3D('',#50149,#40407,#40408);
#35288=AXIS2_PLACEMENT_3D('',#50156,#40412,#40413);
#35289=AXIS2_PLACEMENT_3D('',#50163,#40417,#40418);
#35290=AXIS2_PLACEMENT_3D('',#50166,#40421,#40422);
#35291=AXIS2_PLACEMENT_3D('',#50173,#40426,#40427);
#35292=AXIS2_PLACEMENT_3D('',#50176,#40430,#40431);
#35293=AXIS2_PLACEMENT_3D('',#50179,#40434,#40435);
#35294=AXIS2_PLACEMENT_3D('',#50182,#40438,#40439);
#35295=AXIS2_PLACEMENT_3D('',#50185,#40442,#40443);
#35296=AXIS2_PLACEMENT_3D('',#50188,#40446,#40447);
#35297=AXIS2_PLACEMENT_3D('',#50191,#40450,#40451);
#35298=AXIS2_PLACEMENT_3D('',#50194,#40454,#40455);
#35299=AXIS2_PLACEMENT_3D('',#50195,#40456,#40457);
#35300=AXIS2_PLACEMENT_3D('',#50196,#40458,#40459);
#35301=AXIS2_PLACEMENT_3D('',#50197,#40460,#40461);
#35302=AXIS2_PLACEMENT_3D('',#50204,#40465,#40466);
#35303=AXIS2_PLACEMENT_3D('',#50212,#40471,#40472);
#35304=AXIS2_PLACEMENT_3D('',#50215,#40475,#40476);
#35305=AXIS2_PLACEMENT_3D('',#50222,#40480,#40481);
#35306=AXIS2_PLACEMENT_3D('',#50230,#40486,#40487);
#35307=AXIS2_PLACEMENT_3D('',#50233,#40490,#40491);
#35308=AXIS2_PLACEMENT_3D('',#50236,#40494,#40495);
#35309=AXIS2_PLACEMENT_3D('',#50241,#40499,#40500);
#35310=AXIS2_PLACEMENT_3D('',#50243,#40502,#40503);
#35311=AXIS2_PLACEMENT_3D('',#50247,#40506,#40507);
#35312=AXIS2_PLACEMENT_3D('',#50250,#40510,#40511);
#35313=AXIS2_PLACEMENT_3D('',#50251,#40512,#40513);
#35314=AXIS2_PLACEMENT_3D('',#50252,#40514,#40515);
#35315=AXIS2_PLACEMENT_3D('',#50259,#40519,#40520);
#35316=AXIS2_PLACEMENT_3D('',#50266,#40524,#40525);
#35317=AXIS2_PLACEMENT_3D('',#50273,#40529,#40530);
#35318=AXIS2_PLACEMENT_3D('',#50276,#40533,#40534);
#35319=AXIS2_PLACEMENT_3D('',#50283,#40538,#40539);
#35320=AXIS2_PLACEMENT_3D('',#50286,#40542,#40543);
#35321=AXIS2_PLACEMENT_3D('',#50289,#40546,#40547);
#35322=AXIS2_PLACEMENT_3D('',#50292,#40550,#40551);
#35323=AXIS2_PLACEMENT_3D('',#50295,#40554,#40555);
#35324=AXIS2_PLACEMENT_3D('',#50298,#40558,#40559);
#35325=AXIS2_PLACEMENT_3D('',#50301,#40562,#40563);
#35326=AXIS2_PLACEMENT_3D('',#50304,#40566,#40567);
#35327=AXIS2_PLACEMENT_3D('',#50305,#40568,#40569);
#35328=AXIS2_PLACEMENT_3D('',#50306,#40570,#40571);
#35329=AXIS2_PLACEMENT_3D('',#50307,#40572,#40573);
#35330=AXIS2_PLACEMENT_3D('',#50314,#40577,#40578);
#35331=AXIS2_PLACEMENT_3D('',#50321,#40582,#40583);
#35332=AXIS2_PLACEMENT_3D('',#50328,#40587,#40588);
#35333=AXIS2_PLACEMENT_3D('',#50331,#40591,#40592);
#35334=AXIS2_PLACEMENT_3D('',#50338,#40596,#40597);
#35335=AXIS2_PLACEMENT_3D('',#50341,#40600,#40601);
#35336=AXIS2_PLACEMENT_3D('',#50344,#40604,#40605);
#35337=AXIS2_PLACEMENT_3D('',#50347,#40608,#40609);
#35338=AXIS2_PLACEMENT_3D('',#50350,#40612,#40613);
#35339=AXIS2_PLACEMENT_3D('',#50353,#40616,#40617);
#35340=AXIS2_PLACEMENT_3D('',#50356,#40620,#40621);
#35341=AXIS2_PLACEMENT_3D('',#50359,#40624,#40625);
#35342=AXIS2_PLACEMENT_3D('',#50360,#40626,#40627);
#35343=AXIS2_PLACEMENT_3D('',#50361,#40628,#40629);
#35344=AXIS2_PLACEMENT_3D('',#50362,#40630,#40631);
#35345=AXIS2_PLACEMENT_3D('',#50370,#40636,#40637);
#35346=AXIS2_PLACEMENT_3D('',#50374,#40640,#40641);
#35347=AXIS2_PLACEMENT_3D('',#50380,#40645,#40646);
#35348=AXIS2_PLACEMENT_3D('',#50386,#40650,#40651);
#35349=AXIS2_PLACEMENT_3D('',#50390,#40654,#40655);
#35350=AXIS2_PLACEMENT_3D('',#50394,#40658,#40659);
#35351=AXIS2_PLACEMENT_3D('',#50397,#40662,#40663);
#35352=AXIS2_PLACEMENT_3D('',#50404,#40667,#40668);
#35353=AXIS2_PLACEMENT_3D('',#50407,#40671,#40672);
#35354=AXIS2_PLACEMENT_3D('',#50410,#40675,#40676);
#35355=AXIS2_PLACEMENT_3D('',#50413,#40679,#40680);
#35356=AXIS2_PLACEMENT_3D('',#50415,#40682,#40683);
#35357=AXIS2_PLACEMENT_3D('',#50416,#40684,#40685);
#35358=AXIS2_PLACEMENT_3D('',#50417,#40686,#40687);
#35359=AXIS2_PLACEMENT_3D('',#50424,#40691,#40692);
#35360=AXIS2_PLACEMENT_3D('',#50431,#40696,#40697);
#35361=AXIS2_PLACEMENT_3D('',#50438,#40701,#40702);
#35362=AXIS2_PLACEMENT_3D('',#50441,#40705,#40706);
#35363=AXIS2_PLACEMENT_3D('',#50448,#40710,#40711);
#35364=AXIS2_PLACEMENT_3D('',#50451,#40714,#40715);
#35365=AXIS2_PLACEMENT_3D('',#50454,#40718,#40719);
#35366=AXIS2_PLACEMENT_3D('',#50457,#40722,#40723);
#35367=AXIS2_PLACEMENT_3D('',#50460,#40726,#40727);
#35368=AXIS2_PLACEMENT_3D('',#50463,#40730,#40731);
#35369=AXIS2_PLACEMENT_3D('',#50466,#40734,#40735);
#35370=AXIS2_PLACEMENT_3D('',#50469,#40738,#40739);
#35371=AXIS2_PLACEMENT_3D('',#50470,#40740,#40741);
#35372=AXIS2_PLACEMENT_3D('',#50471,#40742,#40743);
#35373=AXIS2_PLACEMENT_3D('',#50472,#40744,#40745);
#35374=AXIS2_PLACEMENT_3D('',#50479,#40749,#40750);
#35375=AXIS2_PLACEMENT_3D('',#50487,#40755,#40756);
#35376=AXIS2_PLACEMENT_3D('',#50490,#40759,#40760);
#35377=AXIS2_PLACEMENT_3D('',#50497,#40764,#40765);
#35378=AXIS2_PLACEMENT_3D('',#50505,#40770,#40771);
#35379=AXIS2_PLACEMENT_3D('',#50508,#40774,#40775);
#35380=AXIS2_PLACEMENT_3D('',#50511,#40778,#40779);
#35381=AXIS2_PLACEMENT_3D('',#50516,#40783,#40784);
#35382=AXIS2_PLACEMENT_3D('',#50518,#40786,#40787);
#35383=AXIS2_PLACEMENT_3D('',#50522,#40790,#40791);
#35384=AXIS2_PLACEMENT_3D('',#50525,#40794,#40795);
#35385=AXIS2_PLACEMENT_3D('',#50526,#40796,#40797);
#35386=AXIS2_PLACEMENT_3D('',#50527,#40798,#40799);
#35387=AXIS2_PLACEMENT_3D('',#50534,#40803,#40804);
#35388=AXIS2_PLACEMENT_3D('',#50541,#40808,#40809);
#35389=AXIS2_PLACEMENT_3D('',#50548,#40813,#40814);
#35390=AXIS2_PLACEMENT_3D('',#50551,#40817,#40818);
#35391=AXIS2_PLACEMENT_3D('',#50558,#40822,#40823);
#35392=AXIS2_PLACEMENT_3D('',#50561,#40826,#40827);
#35393=AXIS2_PLACEMENT_3D('',#50564,#40830,#40831);
#35394=AXIS2_PLACEMENT_3D('',#50567,#40834,#40835);
#35395=AXIS2_PLACEMENT_3D('',#50570,#40838,#40839);
#35396=AXIS2_PLACEMENT_3D('',#50573,#40842,#40843);
#35397=AXIS2_PLACEMENT_3D('',#50576,#40846,#40847);
#35398=AXIS2_PLACEMENT_3D('',#50579,#40850,#40851);
#35399=AXIS2_PLACEMENT_3D('',#50580,#40852,#40853);
#35400=AXIS2_PLACEMENT_3D('',#50581,#40854,#40855);
#35401=AXIS2_PLACEMENT_3D('',#50582,#40856,#40857);
#35402=AXIS2_PLACEMENT_3D('',#50589,#40861,#40862);
#35403=AXIS2_PLACEMENT_3D('',#50596,#40866,#40867);
#35404=AXIS2_PLACEMENT_3D('',#50603,#40871,#40872);
#35405=AXIS2_PLACEMENT_3D('',#50606,#40875,#40876);
#35406=AXIS2_PLACEMENT_3D('',#50613,#40880,#40881);
#35407=AXIS2_PLACEMENT_3D('',#50616,#40884,#40885);
#35408=AXIS2_PLACEMENT_3D('',#50619,#40888,#40889);
#35409=AXIS2_PLACEMENT_3D('',#50622,#40892,#40893);
#35410=AXIS2_PLACEMENT_3D('',#50625,#40896,#40897);
#35411=AXIS2_PLACEMENT_3D('',#50628,#40900,#40901);
#35412=AXIS2_PLACEMENT_3D('',#50631,#40904,#40905);
#35413=AXIS2_PLACEMENT_3D('',#50634,#40908,#40909);
#35414=AXIS2_PLACEMENT_3D('',#50635,#40910,#40911);
#35415=AXIS2_PLACEMENT_3D('',#50636,#40912,#40913);
#35416=AXIS2_PLACEMENT_3D('',#50637,#40914,#40915);
#35417=AXIS2_PLACEMENT_3D('',#50645,#40920,#40921);
#35418=AXIS2_PLACEMENT_3D('',#50649,#40924,#40925);
#35419=AXIS2_PLACEMENT_3D('',#50655,#40929,#40930);
#35420=AXIS2_PLACEMENT_3D('',#50661,#40934,#40935);
#35421=AXIS2_PLACEMENT_3D('',#50665,#40938,#40939);
#35422=AXIS2_PLACEMENT_3D('',#50669,#40942,#40943);
#35423=AXIS2_PLACEMENT_3D('',#50672,#40946,#40947);
#35424=AXIS2_PLACEMENT_3D('',#50679,#40951,#40952);
#35425=AXIS2_PLACEMENT_3D('',#50682,#40955,#40956);
#35426=AXIS2_PLACEMENT_3D('',#50685,#40959,#40960);
#35427=AXIS2_PLACEMENT_3D('',#50688,#40963,#40964);
#35428=AXIS2_PLACEMENT_3D('',#50690,#40966,#40967);
#35429=AXIS2_PLACEMENT_3D('',#50691,#40968,#40969);
#35430=AXIS2_PLACEMENT_3D('',#50692,#40970,#40971);
#35431=AXIS2_PLACEMENT_3D('',#50699,#40975,#40976);
#35432=AXIS2_PLACEMENT_3D('',#50706,#40980,#40981);
#35433=AXIS2_PLACEMENT_3D('',#50713,#40985,#40986);
#35434=AXIS2_PLACEMENT_3D('',#50716,#40989,#40990);
#35435=AXIS2_PLACEMENT_3D('',#50723,#40994,#40995);
#35436=AXIS2_PLACEMENT_3D('',#50726,#40998,#40999);
#35437=AXIS2_PLACEMENT_3D('',#50729,#41002,#41003);
#35438=AXIS2_PLACEMENT_3D('',#50732,#41006,#41007);
#35439=AXIS2_PLACEMENT_3D('',#50735,#41010,#41011);
#35440=AXIS2_PLACEMENT_3D('',#50738,#41014,#41015);
#35441=AXIS2_PLACEMENT_3D('',#50741,#41018,#41019);
#35442=AXIS2_PLACEMENT_3D('',#50744,#41022,#41023);
#35443=AXIS2_PLACEMENT_3D('',#50745,#41024,#41025);
#35444=AXIS2_PLACEMENT_3D('',#50746,#41026,#41027);
#35445=AXIS2_PLACEMENT_3D('',#50747,#41028,#41029);
#35446=AXIS2_PLACEMENT_3D('',#50754,#41033,#41034);
#35447=AXIS2_PLACEMENT_3D('',#50762,#41039,#41040);
#35448=AXIS2_PLACEMENT_3D('',#50765,#41043,#41044);
#35449=AXIS2_PLACEMENT_3D('',#50772,#41048,#41049);
#35450=AXIS2_PLACEMENT_3D('',#50780,#41054,#41055);
#35451=AXIS2_PLACEMENT_3D('',#50783,#41058,#41059);
#35452=AXIS2_PLACEMENT_3D('',#50786,#41062,#41063);
#35453=AXIS2_PLACEMENT_3D('',#50791,#41067,#41068);
#35454=AXIS2_PLACEMENT_3D('',#50793,#41070,#41071);
#35455=AXIS2_PLACEMENT_3D('',#50797,#41074,#41075);
#35456=AXIS2_PLACEMENT_3D('',#50800,#41078,#41079);
#35457=AXIS2_PLACEMENT_3D('',#50801,#41080,#41081);
#35458=AXIS2_PLACEMENT_3D('',#50802,#41082,#41083);
#35459=AXIS2_PLACEMENT_3D('',#50809,#41087,#41088);
#35460=AXIS2_PLACEMENT_3D('',#50816,#41092,#41093);
#35461=AXIS2_PLACEMENT_3D('',#50823,#41097,#41098);
#35462=AXIS2_PLACEMENT_3D('',#50826,#41101,#41102);
#35463=AXIS2_PLACEMENT_3D('',#50833,#41106,#41107);
#35464=AXIS2_PLACEMENT_3D('',#50836,#41110,#41111);
#35465=AXIS2_PLACEMENT_3D('',#50839,#41114,#41115);
#35466=AXIS2_PLACEMENT_3D('',#50842,#41118,#41119);
#35467=AXIS2_PLACEMENT_3D('',#50845,#41122,#41123);
#35468=AXIS2_PLACEMENT_3D('',#50848,#41126,#41127);
#35469=AXIS2_PLACEMENT_3D('',#50851,#41130,#41131);
#35470=AXIS2_PLACEMENT_3D('',#50854,#41134,#41135);
#35471=AXIS2_PLACEMENT_3D('',#50855,#41136,#41137);
#35472=AXIS2_PLACEMENT_3D('',#50856,#41138,#41139);
#35473=AXIS2_PLACEMENT_3D('',#50857,#41140,#41141);
#35474=AXIS2_PLACEMENT_3D('',#50864,#41145,#41146);
#35475=AXIS2_PLACEMENT_3D('',#50871,#41150,#41151);
#35476=AXIS2_PLACEMENT_3D('',#50878,#41155,#41156);
#35477=AXIS2_PLACEMENT_3D('',#50881,#41159,#41160);
#35478=AXIS2_PLACEMENT_3D('',#50888,#41164,#41165);
#35479=AXIS2_PLACEMENT_3D('',#50891,#41168,#41169);
#35480=AXIS2_PLACEMENT_3D('',#50894,#41172,#41173);
#35481=AXIS2_PLACEMENT_3D('',#50897,#41176,#41177);
#35482=AXIS2_PLACEMENT_3D('',#50900,#41180,#41181);
#35483=AXIS2_PLACEMENT_3D('',#50903,#41184,#41185);
#35484=AXIS2_PLACEMENT_3D('',#50906,#41188,#41189);
#35485=AXIS2_PLACEMENT_3D('',#50909,#41192,#41193);
#35486=AXIS2_PLACEMENT_3D('',#50910,#41194,#41195);
#35487=AXIS2_PLACEMENT_3D('',#50911,#41196,#41197);
#35488=AXIS2_PLACEMENT_3D('',#50912,#41198,#41199);
#35489=AXIS2_PLACEMENT_3D('',#50920,#41204,#41205);
#35490=AXIS2_PLACEMENT_3D('',#50924,#41208,#41209);
#35491=AXIS2_PLACEMENT_3D('',#50930,#41213,#41214);
#35492=AXIS2_PLACEMENT_3D('',#50936,#41218,#41219);
#35493=AXIS2_PLACEMENT_3D('',#50940,#41222,#41223);
#35494=AXIS2_PLACEMENT_3D('',#50944,#41226,#41227);
#35495=AXIS2_PLACEMENT_3D('',#50947,#41230,#41231);
#35496=AXIS2_PLACEMENT_3D('',#50954,#41235,#41236);
#35497=AXIS2_PLACEMENT_3D('',#50957,#41239,#41240);
#35498=AXIS2_PLACEMENT_3D('',#50960,#41243,#41244);
#35499=AXIS2_PLACEMENT_3D('',#50963,#41247,#41248);
#35500=AXIS2_PLACEMENT_3D('',#50965,#41250,#41251);
#35501=AXIS2_PLACEMENT_3D('',#50966,#41252,#41253);
#35502=AXIS2_PLACEMENT_3D('',#50967,#41254,#41255);
#35503=AXIS2_PLACEMENT_3D('',#50974,#41259,#41260);
#35504=AXIS2_PLACEMENT_3D('',#50981,#41264,#41265);
#35505=AXIS2_PLACEMENT_3D('',#50988,#41269,#41270);
#35506=AXIS2_PLACEMENT_3D('',#50991,#41273,#41274);
#35507=AXIS2_PLACEMENT_3D('',#50998,#41278,#41279);
#35508=AXIS2_PLACEMENT_3D('',#51001,#41282,#41283);
#35509=AXIS2_PLACEMENT_3D('',#51004,#41286,#41287);
#35510=AXIS2_PLACEMENT_3D('',#51007,#41290,#41291);
#35511=AXIS2_PLACEMENT_3D('',#51010,#41294,#41295);
#35512=AXIS2_PLACEMENT_3D('',#51013,#41298,#41299);
#35513=AXIS2_PLACEMENT_3D('',#51016,#41302,#41303);
#35514=AXIS2_PLACEMENT_3D('',#51019,#41306,#41307);
#35515=AXIS2_PLACEMENT_3D('',#51020,#41308,#41309);
#35516=AXIS2_PLACEMENT_3D('',#51021,#41310,#41311);
#35517=AXIS2_PLACEMENT_3D('',#51022,#41312,#41313);
#35518=AXIS2_PLACEMENT_3D('',#51029,#41317,#41318);
#35519=AXIS2_PLACEMENT_3D('',#51037,#41323,#41324);
#35520=AXIS2_PLACEMENT_3D('',#51040,#41327,#41328);
#35521=AXIS2_PLACEMENT_3D('',#51047,#41332,#41333);
#35522=AXIS2_PLACEMENT_3D('',#51055,#41338,#41339);
#35523=AXIS2_PLACEMENT_3D('',#51058,#41342,#41343);
#35524=AXIS2_PLACEMENT_3D('',#51061,#41346,#41347);
#35525=AXIS2_PLACEMENT_3D('',#51066,#41351,#41352);
#35526=AXIS2_PLACEMENT_3D('',#51068,#41354,#41355);
#35527=AXIS2_PLACEMENT_3D('',#51072,#41358,#41359);
#35528=AXIS2_PLACEMENT_3D('',#51075,#41362,#41363);
#35529=AXIS2_PLACEMENT_3D('',#51076,#41364,#41365);
#35530=AXIS2_PLACEMENT_3D('',#51077,#41366,#41367);
#35531=AXIS2_PLACEMENT_3D('',#51084,#41371,#41372);
#35532=AXIS2_PLACEMENT_3D('',#51091,#41376,#41377);
#35533=AXIS2_PLACEMENT_3D('',#51098,#41381,#41382);
#35534=AXIS2_PLACEMENT_3D('',#51101,#41385,#41386);
#35535=AXIS2_PLACEMENT_3D('',#51108,#41390,#41391);
#35536=AXIS2_PLACEMENT_3D('',#51111,#41394,#41395);
#35537=AXIS2_PLACEMENT_3D('',#51114,#41398,#41399);
#35538=AXIS2_PLACEMENT_3D('',#51117,#41402,#41403);
#35539=AXIS2_PLACEMENT_3D('',#51120,#41406,#41407);
#35540=AXIS2_PLACEMENT_3D('',#51123,#41410,#41411);
#35541=AXIS2_PLACEMENT_3D('',#51126,#41414,#41415);
#35542=AXIS2_PLACEMENT_3D('',#51129,#41418,#41419);
#35543=AXIS2_PLACEMENT_3D('',#51130,#41420,#41421);
#35544=AXIS2_PLACEMENT_3D('',#51131,#41422,#41423);
#35545=AXIS2_PLACEMENT_3D('',#51132,#41424,#41425);
#35546=AXIS2_PLACEMENT_3D('',#51139,#41429,#41430);
#35547=AXIS2_PLACEMENT_3D('',#51146,#41434,#41435);
#35548=AXIS2_PLACEMENT_3D('',#51153,#41439,#41440);
#35549=AXIS2_PLACEMENT_3D('',#51156,#41443,#41444);
#35550=AXIS2_PLACEMENT_3D('',#51163,#41448,#41449);
#35551=AXIS2_PLACEMENT_3D('',#51166,#41452,#41453);
#35552=AXIS2_PLACEMENT_3D('',#51169,#41456,#41457);
#35553=AXIS2_PLACEMENT_3D('',#51172,#41460,#41461);
#35554=AXIS2_PLACEMENT_3D('',#51175,#41464,#41465);
#35555=AXIS2_PLACEMENT_3D('',#51178,#41468,#41469);
#35556=AXIS2_PLACEMENT_3D('',#51181,#41472,#41473);
#35557=AXIS2_PLACEMENT_3D('',#51184,#41476,#41477);
#35558=AXIS2_PLACEMENT_3D('',#51185,#41478,#41479);
#35559=AXIS2_PLACEMENT_3D('',#51186,#41480,#41481);
#35560=AXIS2_PLACEMENT_3D('',#51187,#41482,#41483);
#35561=AXIS2_PLACEMENT_3D('',#51195,#41488,#41489);
#35562=AXIS2_PLACEMENT_3D('',#51199,#41492,#41493);
#35563=AXIS2_PLACEMENT_3D('',#51205,#41497,#41498);
#35564=AXIS2_PLACEMENT_3D('',#51211,#41502,#41503);
#35565=AXIS2_PLACEMENT_3D('',#51215,#41506,#41507);
#35566=AXIS2_PLACEMENT_3D('',#51219,#41510,#41511);
#35567=AXIS2_PLACEMENT_3D('',#51222,#41514,#41515);
#35568=AXIS2_PLACEMENT_3D('',#51229,#41519,#41520);
#35569=AXIS2_PLACEMENT_3D('',#51232,#41523,#41524);
#35570=AXIS2_PLACEMENT_3D('',#51235,#41527,#41528);
#35571=AXIS2_PLACEMENT_3D('',#51238,#41531,#41532);
#35572=AXIS2_PLACEMENT_3D('',#51240,#41534,#41535);
#35573=AXIS2_PLACEMENT_3D('',#51241,#41536,#41537);
#35574=AXIS2_PLACEMENT_3D('',#51242,#41538,#41539);
#35575=AXIS2_PLACEMENT_3D('',#51249,#41543,#41544);
#35576=AXIS2_PLACEMENT_3D('',#51256,#41548,#41549);
#35577=AXIS2_PLACEMENT_3D('',#51263,#41553,#41554);
#35578=AXIS2_PLACEMENT_3D('',#51266,#41557,#41558);
#35579=AXIS2_PLACEMENT_3D('',#51273,#41562,#41563);
#35580=AXIS2_PLACEMENT_3D('',#51276,#41566,#41567);
#35581=AXIS2_PLACEMENT_3D('',#51279,#41570,#41571);
#35582=AXIS2_PLACEMENT_3D('',#51282,#41574,#41575);
#35583=AXIS2_PLACEMENT_3D('',#51285,#41578,#41579);
#35584=AXIS2_PLACEMENT_3D('',#51288,#41582,#41583);
#35585=AXIS2_PLACEMENT_3D('',#51291,#41586,#41587);
#35586=AXIS2_PLACEMENT_3D('',#51294,#41590,#41591);
#35587=AXIS2_PLACEMENT_3D('',#51295,#41592,#41593);
#35588=AXIS2_PLACEMENT_3D('',#51296,#41594,#41595);
#35589=AXIS2_PLACEMENT_3D('',#51297,#41596,#41597);
#35590=AXIS2_PLACEMENT_3D('',#51304,#41601,#41602);
#35591=AXIS2_PLACEMENT_3D('',#51312,#41607,#41608);
#35592=AXIS2_PLACEMENT_3D('',#51315,#41611,#41612);
#35593=AXIS2_PLACEMENT_3D('',#51322,#41616,#41617);
#35594=AXIS2_PLACEMENT_3D('',#51330,#41622,#41623);
#35595=AXIS2_PLACEMENT_3D('',#51333,#41626,#41627);
#35596=AXIS2_PLACEMENT_3D('',#51336,#41630,#41631);
#35597=AXIS2_PLACEMENT_3D('',#51341,#41635,#41636);
#35598=AXIS2_PLACEMENT_3D('',#51343,#41638,#41639);
#35599=AXIS2_PLACEMENT_3D('',#51347,#41642,#41643);
#35600=AXIS2_PLACEMENT_3D('',#51350,#41646,#41647);
#35601=AXIS2_PLACEMENT_3D('',#51351,#41648,#41649);
#35602=AXIS2_PLACEMENT_3D('',#51352,#41650,#41651);
#35603=AXIS2_PLACEMENT_3D('',#51359,#41655,#41656);
#35604=AXIS2_PLACEMENT_3D('',#51366,#41660,#41661);
#35605=AXIS2_PLACEMENT_3D('',#51373,#41665,#41666);
#35606=AXIS2_PLACEMENT_3D('',#51376,#41669,#41670);
#35607=AXIS2_PLACEMENT_3D('',#51383,#41674,#41675);
#35608=AXIS2_PLACEMENT_3D('',#51386,#41678,#41679);
#35609=AXIS2_PLACEMENT_3D('',#51389,#41682,#41683);
#35610=AXIS2_PLACEMENT_3D('',#51392,#41686,#41687);
#35611=AXIS2_PLACEMENT_3D('',#51395,#41690,#41691);
#35612=AXIS2_PLACEMENT_3D('',#51398,#41694,#41695);
#35613=AXIS2_PLACEMENT_3D('',#51401,#41698,#41699);
#35614=AXIS2_PLACEMENT_3D('',#51404,#41702,#41703);
#35615=AXIS2_PLACEMENT_3D('',#51405,#41704,#41705);
#35616=AXIS2_PLACEMENT_3D('',#51406,#41706,#41707);
#35617=AXIS2_PLACEMENT_3D('',#51407,#41708,#41709);
#35618=AXIS2_PLACEMENT_3D('',#51414,#41713,#41714);
#35619=AXIS2_PLACEMENT_3D('',#51421,#41718,#41719);
#35620=AXIS2_PLACEMENT_3D('',#51428,#41723,#41724);
#35621=AXIS2_PLACEMENT_3D('',#51431,#41727,#41728);
#35622=AXIS2_PLACEMENT_3D('',#51438,#41732,#41733);
#35623=AXIS2_PLACEMENT_3D('',#51441,#41736,#41737);
#35624=AXIS2_PLACEMENT_3D('',#51444,#41740,#41741);
#35625=AXIS2_PLACEMENT_3D('',#51447,#41744,#41745);
#35626=AXIS2_PLACEMENT_3D('',#51450,#41748,#41749);
#35627=AXIS2_PLACEMENT_3D('',#51453,#41752,#41753);
#35628=AXIS2_PLACEMENT_3D('',#51456,#41756,#41757);
#35629=AXIS2_PLACEMENT_3D('',#51459,#41760,#41761);
#35630=AXIS2_PLACEMENT_3D('',#51460,#41762,#41763);
#35631=AXIS2_PLACEMENT_3D('',#51461,#41764,#41765);
#35632=AXIS2_PLACEMENT_3D('',#51462,#41766,#41767);
#35633=AXIS2_PLACEMENT_3D('',#51470,#41772,#41773);
#35634=AXIS2_PLACEMENT_3D('',#51474,#41776,#41777);
#35635=AXIS2_PLACEMENT_3D('',#51480,#41781,#41782);
#35636=AXIS2_PLACEMENT_3D('',#51486,#41786,#41787);
#35637=AXIS2_PLACEMENT_3D('',#51490,#41790,#41791);
#35638=AXIS2_PLACEMENT_3D('',#51494,#41794,#41795);
#35639=AXIS2_PLACEMENT_3D('',#51497,#41798,#41799);
#35640=AXIS2_PLACEMENT_3D('',#51504,#41803,#41804);
#35641=AXIS2_PLACEMENT_3D('',#51507,#41807,#41808);
#35642=AXIS2_PLACEMENT_3D('',#51510,#41811,#41812);
#35643=AXIS2_PLACEMENT_3D('',#51513,#41815,#41816);
#35644=AXIS2_PLACEMENT_3D('',#51515,#41818,#41819);
#35645=AXIS2_PLACEMENT_3D('',#51516,#41820,#41821);
#35646=AXIS2_PLACEMENT_3D('',#51517,#41822,#41823);
#35647=AXIS2_PLACEMENT_3D('',#51524,#41827,#41828);
#35648=AXIS2_PLACEMENT_3D('',#51531,#41832,#41833);
#35649=AXIS2_PLACEMENT_3D('',#51538,#41837,#41838);
#35650=AXIS2_PLACEMENT_3D('',#51541,#41841,#41842);
#35651=AXIS2_PLACEMENT_3D('',#51548,#41846,#41847);
#35652=AXIS2_PLACEMENT_3D('',#51551,#41850,#41851);
#35653=AXIS2_PLACEMENT_3D('',#51554,#41854,#41855);
#35654=AXIS2_PLACEMENT_3D('',#51557,#41858,#41859);
#35655=AXIS2_PLACEMENT_3D('',#51560,#41862,#41863);
#35656=AXIS2_PLACEMENT_3D('',#51563,#41866,#41867);
#35657=AXIS2_PLACEMENT_3D('',#51566,#41870,#41871);
#35658=AXIS2_PLACEMENT_3D('',#51569,#41874,#41875);
#35659=AXIS2_PLACEMENT_3D('',#51570,#41876,#41877);
#35660=AXIS2_PLACEMENT_3D('',#51571,#41878,#41879);
#35661=AXIS2_PLACEMENT_3D('',#51572,#41880,#41881);
#35662=AXIS2_PLACEMENT_3D('',#51579,#41885,#41886);
#35663=AXIS2_PLACEMENT_3D('',#51587,#41891,#41892);
#35664=AXIS2_PLACEMENT_3D('',#51590,#41895,#41896);
#35665=AXIS2_PLACEMENT_3D('',#51597,#41900,#41901);
#35666=AXIS2_PLACEMENT_3D('',#51605,#41906,#41907);
#35667=AXIS2_PLACEMENT_3D('',#51608,#41910,#41911);
#35668=AXIS2_PLACEMENT_3D('',#51611,#41914,#41915);
#35669=AXIS2_PLACEMENT_3D('',#51616,#41919,#41920);
#35670=AXIS2_PLACEMENT_3D('',#51618,#41922,#41923);
#35671=AXIS2_PLACEMENT_3D('',#51622,#41926,#41927);
#35672=AXIS2_PLACEMENT_3D('',#51625,#41930,#41931);
#35673=AXIS2_PLACEMENT_3D('',#51626,#41932,#41933);
#35674=AXIS2_PLACEMENT_3D('',#51627,#41934,#41935);
#35675=AXIS2_PLACEMENT_3D('',#51634,#41939,#41940);
#35676=AXIS2_PLACEMENT_3D('',#51641,#41944,#41945);
#35677=AXIS2_PLACEMENT_3D('',#51648,#41949,#41950);
#35678=AXIS2_PLACEMENT_3D('',#51651,#41953,#41954);
#35679=AXIS2_PLACEMENT_3D('',#51658,#41958,#41959);
#35680=AXIS2_PLACEMENT_3D('',#51661,#41962,#41963);
#35681=AXIS2_PLACEMENT_3D('',#51664,#41966,#41967);
#35682=AXIS2_PLACEMENT_3D('',#51667,#41970,#41971);
#35683=AXIS2_PLACEMENT_3D('',#51670,#41974,#41975);
#35684=AXIS2_PLACEMENT_3D('',#51673,#41978,#41979);
#35685=AXIS2_PLACEMENT_3D('',#51676,#41982,#41983);
#35686=AXIS2_PLACEMENT_3D('',#51679,#41986,#41987);
#35687=AXIS2_PLACEMENT_3D('',#51680,#41988,#41989);
#35688=AXIS2_PLACEMENT_3D('',#51681,#41990,#41991);
#35689=AXIS2_PLACEMENT_3D('',#51682,#41992,#41993);
#35690=AXIS2_PLACEMENT_3D('',#51689,#41997,#41998);
#35691=AXIS2_PLACEMENT_3D('',#51696,#42002,#42003);
#35692=AXIS2_PLACEMENT_3D('',#51703,#42007,#42008);
#35693=AXIS2_PLACEMENT_3D('',#51706,#42011,#42012);
#35694=AXIS2_PLACEMENT_3D('',#51713,#42016,#42017);
#35695=AXIS2_PLACEMENT_3D('',#51716,#42020,#42021);
#35696=AXIS2_PLACEMENT_3D('',#51719,#42024,#42025);
#35697=AXIS2_PLACEMENT_3D('',#51722,#42028,#42029);
#35698=AXIS2_PLACEMENT_3D('',#51725,#42032,#42033);
#35699=AXIS2_PLACEMENT_3D('',#51728,#42036,#42037);
#35700=AXIS2_PLACEMENT_3D('',#51731,#42040,#42041);
#35701=AXIS2_PLACEMENT_3D('',#51734,#42044,#42045);
#35702=AXIS2_PLACEMENT_3D('',#51735,#42046,#42047);
#35703=AXIS2_PLACEMENT_3D('',#51736,#42048,#42049);
#35704=AXIS2_PLACEMENT_3D('',#51737,#42050,#42051);
#35705=AXIS2_PLACEMENT_3D('',#51745,#42056,#42057);
#35706=AXIS2_PLACEMENT_3D('',#51749,#42060,#42061);
#35707=AXIS2_PLACEMENT_3D('',#51755,#42065,#42066);
#35708=AXIS2_PLACEMENT_3D('',#51761,#42070,#42071);
#35709=AXIS2_PLACEMENT_3D('',#51765,#42074,#42075);
#35710=AXIS2_PLACEMENT_3D('',#51769,#42078,#42079);
#35711=AXIS2_PLACEMENT_3D('',#51772,#42082,#42083);
#35712=AXIS2_PLACEMENT_3D('',#51779,#42087,#42088);
#35713=AXIS2_PLACEMENT_3D('',#51782,#42091,#42092);
#35714=AXIS2_PLACEMENT_3D('',#51785,#42095,#42096);
#35715=AXIS2_PLACEMENT_3D('',#51788,#42099,#42100);
#35716=AXIS2_PLACEMENT_3D('',#51790,#42102,#42103);
#35717=AXIS2_PLACEMENT_3D('',#51791,#42104,#42105);
#35718=AXIS2_PLACEMENT_3D('',#51792,#42106,#42107);
#35719=AXIS2_PLACEMENT_3D('',#51799,#42111,#42112);
#35720=AXIS2_PLACEMENT_3D('',#51806,#42116,#42117);
#35721=AXIS2_PLACEMENT_3D('',#51813,#42121,#42122);
#35722=AXIS2_PLACEMENT_3D('',#51816,#42125,#42126);
#35723=AXIS2_PLACEMENT_3D('',#51823,#42130,#42131);
#35724=AXIS2_PLACEMENT_3D('',#51826,#42134,#42135);
#35725=AXIS2_PLACEMENT_3D('',#51829,#42138,#42139);
#35726=AXIS2_PLACEMENT_3D('',#51832,#42142,#42143);
#35727=AXIS2_PLACEMENT_3D('',#51835,#42146,#42147);
#35728=AXIS2_PLACEMENT_3D('',#51838,#42150,#42151);
#35729=AXIS2_PLACEMENT_3D('',#51841,#42154,#42155);
#35730=AXIS2_PLACEMENT_3D('',#51844,#42158,#42159);
#35731=AXIS2_PLACEMENT_3D('',#51845,#42160,#42161);
#35732=AXIS2_PLACEMENT_3D('',#51846,#42162,#42163);
#35733=AXIS2_PLACEMENT_3D('',#51847,#42164,#42165);
#35734=AXIS2_PLACEMENT_3D('',#51854,#42169,#42170);
#35735=AXIS2_PLACEMENT_3D('',#51862,#42175,#42176);
#35736=AXIS2_PLACEMENT_3D('',#51865,#42179,#42180);
#35737=AXIS2_PLACEMENT_3D('',#51872,#42184,#42185);
#35738=AXIS2_PLACEMENT_3D('',#51880,#42190,#42191);
#35739=AXIS2_PLACEMENT_3D('',#51883,#42194,#42195);
#35740=AXIS2_PLACEMENT_3D('',#51886,#42198,#42199);
#35741=AXIS2_PLACEMENT_3D('',#51891,#42203,#42204);
#35742=AXIS2_PLACEMENT_3D('',#51893,#42206,#42207);
#35743=AXIS2_PLACEMENT_3D('',#51897,#42210,#42211);
#35744=AXIS2_PLACEMENT_3D('',#51900,#42214,#42215);
#35745=AXIS2_PLACEMENT_3D('',#51901,#42216,#42217);
#35746=AXIS2_PLACEMENT_3D('',#51902,#42218,#42219);
#35747=AXIS2_PLACEMENT_3D('',#51909,#42223,#42224);
#35748=AXIS2_PLACEMENT_3D('',#51916,#42228,#42229);
#35749=AXIS2_PLACEMENT_3D('',#51923,#42233,#42234);
#35750=AXIS2_PLACEMENT_3D('',#51926,#42237,#42238);
#35751=AXIS2_PLACEMENT_3D('',#51933,#42242,#42243);
#35752=AXIS2_PLACEMENT_3D('',#51936,#42246,#42247);
#35753=AXIS2_PLACEMENT_3D('',#51939,#42250,#42251);
#35754=AXIS2_PLACEMENT_3D('',#51942,#42254,#42255);
#35755=AXIS2_PLACEMENT_3D('',#51945,#42258,#42259);
#35756=AXIS2_PLACEMENT_3D('',#51948,#42262,#42263);
#35757=AXIS2_PLACEMENT_3D('',#51951,#42266,#42267);
#35758=AXIS2_PLACEMENT_3D('',#51954,#42270,#42271);
#35759=AXIS2_PLACEMENT_3D('',#51955,#42272,#42273);
#35760=AXIS2_PLACEMENT_3D('',#51956,#42274,#42275);
#35761=AXIS2_PLACEMENT_3D('',#51957,#42276,#42277);
#35762=AXIS2_PLACEMENT_3D('',#51964,#42281,#42282);
#35763=AXIS2_PLACEMENT_3D('',#51971,#42286,#42287);
#35764=AXIS2_PLACEMENT_3D('',#51978,#42291,#42292);
#35765=AXIS2_PLACEMENT_3D('',#51981,#42295,#42296);
#35766=AXIS2_PLACEMENT_3D('',#51988,#42300,#42301);
#35767=AXIS2_PLACEMENT_3D('',#51991,#42304,#42305);
#35768=AXIS2_PLACEMENT_3D('',#51994,#42308,#42309);
#35769=AXIS2_PLACEMENT_3D('',#51997,#42312,#42313);
#35770=AXIS2_PLACEMENT_3D('',#52000,#42316,#42317);
#35771=AXIS2_PLACEMENT_3D('',#52003,#42320,#42321);
#35772=AXIS2_PLACEMENT_3D('',#52006,#42324,#42325);
#35773=AXIS2_PLACEMENT_3D('',#52009,#42328,#42329);
#35774=AXIS2_PLACEMENT_3D('',#52010,#42330,#42331);
#35775=AXIS2_PLACEMENT_3D('',#52011,#42332,#42333);
#35776=AXIS2_PLACEMENT_3D('',#52012,#42334,#42335);
#35777=AXIS2_PLACEMENT_3D('',#52020,#42340,#42341);
#35778=AXIS2_PLACEMENT_3D('',#52024,#42344,#42345);
#35779=AXIS2_PLACEMENT_3D('',#52030,#42349,#42350);
#35780=AXIS2_PLACEMENT_3D('',#52036,#42354,#42355);
#35781=AXIS2_PLACEMENT_3D('',#52040,#42358,#42359);
#35782=AXIS2_PLACEMENT_3D('',#52044,#42362,#42363);
#35783=AXIS2_PLACEMENT_3D('',#52047,#42366,#42367);
#35784=AXIS2_PLACEMENT_3D('',#52054,#42371,#42372);
#35785=AXIS2_PLACEMENT_3D('',#52057,#42375,#42376);
#35786=AXIS2_PLACEMENT_3D('',#52060,#42379,#42380);
#35787=AXIS2_PLACEMENT_3D('',#52063,#42383,#42384);
#35788=AXIS2_PLACEMENT_3D('',#52065,#42386,#42387);
#35789=AXIS2_PLACEMENT_3D('',#52066,#42388,#42389);
#35790=AXIS2_PLACEMENT_3D('',#52067,#42390,#42391);
#35791=AXIS2_PLACEMENT_3D('',#52074,#42395,#42396);
#35792=AXIS2_PLACEMENT_3D('',#52081,#42400,#42401);
#35793=AXIS2_PLACEMENT_3D('',#52088,#42405,#42406);
#35794=AXIS2_PLACEMENT_3D('',#52091,#42409,#42410);
#35795=AXIS2_PLACEMENT_3D('',#52098,#42414,#42415);
#35796=AXIS2_PLACEMENT_3D('',#52101,#42418,#42419);
#35797=AXIS2_PLACEMENT_3D('',#52104,#42422,#42423);
#35798=AXIS2_PLACEMENT_3D('',#52107,#42426,#42427);
#35799=AXIS2_PLACEMENT_3D('',#52110,#42430,#42431);
#35800=AXIS2_PLACEMENT_3D('',#52113,#42434,#42435);
#35801=AXIS2_PLACEMENT_3D('',#52116,#42438,#42439);
#35802=AXIS2_PLACEMENT_3D('',#52119,#42442,#42443);
#35803=AXIS2_PLACEMENT_3D('',#52120,#42444,#42445);
#35804=AXIS2_PLACEMENT_3D('',#52121,#42446,#42447);
#35805=AXIS2_PLACEMENT_3D('',#52122,#42448,#42449);
#35806=AXIS2_PLACEMENT_3D('',#52129,#42453,#42454);
#35807=AXIS2_PLACEMENT_3D('',#52137,#42459,#42460);
#35808=AXIS2_PLACEMENT_3D('',#52140,#42463,#42464);
#35809=AXIS2_PLACEMENT_3D('',#52147,#42468,#42469);
#35810=AXIS2_PLACEMENT_3D('',#52155,#42474,#42475);
#35811=AXIS2_PLACEMENT_3D('',#52158,#42478,#42479);
#35812=AXIS2_PLACEMENT_3D('',#52161,#42482,#42483);
#35813=AXIS2_PLACEMENT_3D('',#52166,#42487,#42488);
#35814=AXIS2_PLACEMENT_3D('',#52168,#42490,#42491);
#35815=AXIS2_PLACEMENT_3D('',#52172,#42494,#42495);
#35816=AXIS2_PLACEMENT_3D('',#52175,#42498,#42499);
#35817=AXIS2_PLACEMENT_3D('',#52176,#42500,#42501);
#35818=AXIS2_PLACEMENT_3D('',#52177,#42502,#42503);
#35819=AXIS2_PLACEMENT_3D('',#52184,#42507,#42508);
#35820=AXIS2_PLACEMENT_3D('',#52191,#42512,#42513);
#35821=AXIS2_PLACEMENT_3D('',#52198,#42517,#42518);
#35822=AXIS2_PLACEMENT_3D('',#52201,#42521,#42522);
#35823=AXIS2_PLACEMENT_3D('',#52208,#42526,#42527);
#35824=AXIS2_PLACEMENT_3D('',#52211,#42530,#42531);
#35825=AXIS2_PLACEMENT_3D('',#52214,#42534,#42535);
#35826=AXIS2_PLACEMENT_3D('',#52217,#42538,#42539);
#35827=AXIS2_PLACEMENT_3D('',#52220,#42542,#42543);
#35828=AXIS2_PLACEMENT_3D('',#52223,#42546,#42547);
#35829=AXIS2_PLACEMENT_3D('',#52226,#42550,#42551);
#35830=AXIS2_PLACEMENT_3D('',#52229,#42554,#42555);
#35831=AXIS2_PLACEMENT_3D('',#52230,#42556,#42557);
#35832=AXIS2_PLACEMENT_3D('',#52231,#42558,#42559);
#35833=AXIS2_PLACEMENT_3D('',#52232,#42560,#42561);
#35834=AXIS2_PLACEMENT_3D('',#52239,#42565,#42566);
#35835=AXIS2_PLACEMENT_3D('',#52246,#42570,#42571);
#35836=AXIS2_PLACEMENT_3D('',#52253,#42575,#42576);
#35837=AXIS2_PLACEMENT_3D('',#52256,#42579,#42580);
#35838=AXIS2_PLACEMENT_3D('',#52263,#42584,#42585);
#35839=AXIS2_PLACEMENT_3D('',#52266,#42588,#42589);
#35840=AXIS2_PLACEMENT_3D('',#52269,#42592,#42593);
#35841=AXIS2_PLACEMENT_3D('',#52272,#42596,#42597);
#35842=AXIS2_PLACEMENT_3D('',#52275,#42600,#42601);
#35843=AXIS2_PLACEMENT_3D('',#52278,#42604,#42605);
#35844=AXIS2_PLACEMENT_3D('',#52281,#42608,#42609);
#35845=AXIS2_PLACEMENT_3D('',#52284,#42612,#42613);
#35846=AXIS2_PLACEMENT_3D('',#52285,#42614,#42615);
#35847=AXIS2_PLACEMENT_3D('',#52286,#42616,#42617);
#35848=AXIS2_PLACEMENT_3D('',#52287,#42618,#42619);
#35849=AXIS2_PLACEMENT_3D('',#52295,#42624,#42625);
#35850=AXIS2_PLACEMENT_3D('',#52299,#42628,#42629);
#35851=AXIS2_PLACEMENT_3D('',#52305,#42633,#42634);
#35852=AXIS2_PLACEMENT_3D('',#52311,#42638,#42639);
#35853=AXIS2_PLACEMENT_3D('',#52315,#42642,#42643);
#35854=AXIS2_PLACEMENT_3D('',#52319,#42646,#42647);
#35855=AXIS2_PLACEMENT_3D('',#52322,#42650,#42651);
#35856=AXIS2_PLACEMENT_3D('',#52329,#42655,#42656);
#35857=AXIS2_PLACEMENT_3D('',#52332,#42659,#42660);
#35858=AXIS2_PLACEMENT_3D('',#52335,#42663,#42664);
#35859=AXIS2_PLACEMENT_3D('',#52338,#42667,#42668);
#35860=AXIS2_PLACEMENT_3D('',#52340,#42670,#42671);
#35861=AXIS2_PLACEMENT_3D('',#52341,#42672,#42673);
#35862=AXIS2_PLACEMENT_3D('',#52342,#42674,#42675);
#35863=AXIS2_PLACEMENT_3D('',#52349,#42679,#42680);
#35864=AXIS2_PLACEMENT_3D('',#52356,#42684,#42685);
#35865=AXIS2_PLACEMENT_3D('',#52363,#42689,#42690);
#35866=AXIS2_PLACEMENT_3D('',#52366,#42693,#42694);
#35867=AXIS2_PLACEMENT_3D('',#52373,#42698,#42699);
#35868=AXIS2_PLACEMENT_3D('',#52376,#42702,#42703);
#35869=AXIS2_PLACEMENT_3D('',#52379,#42706,#42707);
#35870=AXIS2_PLACEMENT_3D('',#52382,#42710,#42711);
#35871=AXIS2_PLACEMENT_3D('',#52385,#42714,#42715);
#35872=AXIS2_PLACEMENT_3D('',#52388,#42718,#42719);
#35873=AXIS2_PLACEMENT_3D('',#52391,#42722,#42723);
#35874=AXIS2_PLACEMENT_3D('',#52394,#42726,#42727);
#35875=AXIS2_PLACEMENT_3D('',#52395,#42728,#42729);
#35876=AXIS2_PLACEMENT_3D('',#52396,#42730,#42731);
#35877=AXIS2_PLACEMENT_3D('',#52397,#42732,#42733);
#35878=AXIS2_PLACEMENT_3D('',#52404,#42737,#42738);
#35879=AXIS2_PLACEMENT_3D('',#52412,#42743,#42744);
#35880=AXIS2_PLACEMENT_3D('',#52415,#42747,#42748);
#35881=AXIS2_PLACEMENT_3D('',#52422,#42752,#42753);
#35882=AXIS2_PLACEMENT_3D('',#52430,#42758,#42759);
#35883=AXIS2_PLACEMENT_3D('',#52433,#42762,#42763);
#35884=AXIS2_PLACEMENT_3D('',#52436,#42766,#42767);
#35885=AXIS2_PLACEMENT_3D('',#52441,#42771,#42772);
#35886=AXIS2_PLACEMENT_3D('',#52443,#42774,#42775);
#35887=AXIS2_PLACEMENT_3D('',#52447,#42778,#42779);
#35888=AXIS2_PLACEMENT_3D('',#52450,#42782,#42783);
#35889=AXIS2_PLACEMENT_3D('',#52451,#42784,#42785);
#35890=AXIS2_PLACEMENT_3D('',#52452,#42786,#42787);
#35891=AXIS2_PLACEMENT_3D('',#52459,#42791,#42792);
#35892=AXIS2_PLACEMENT_3D('',#52466,#42796,#42797);
#35893=AXIS2_PLACEMENT_3D('',#52473,#42801,#42802);
#35894=AXIS2_PLACEMENT_3D('',#52476,#42805,#42806);
#35895=AXIS2_PLACEMENT_3D('',#52483,#42810,#42811);
#35896=AXIS2_PLACEMENT_3D('',#52486,#42814,#42815);
#35897=AXIS2_PLACEMENT_3D('',#52489,#42818,#42819);
#35898=AXIS2_PLACEMENT_3D('',#52492,#42822,#42823);
#35899=AXIS2_PLACEMENT_3D('',#52495,#42826,#42827);
#35900=AXIS2_PLACEMENT_3D('',#52498,#42830,#42831);
#35901=AXIS2_PLACEMENT_3D('',#52501,#42834,#42835);
#35902=AXIS2_PLACEMENT_3D('',#52504,#42838,#42839);
#35903=AXIS2_PLACEMENT_3D('',#52505,#42840,#42841);
#35904=AXIS2_PLACEMENT_3D('',#52506,#42842,#42843);
#35905=AXIS2_PLACEMENT_3D('',#52507,#42844,#42845);
#35906=AXIS2_PLACEMENT_3D('',#52514,#42849,#42850);
#35907=AXIS2_PLACEMENT_3D('',#52521,#42854,#42855);
#35908=AXIS2_PLACEMENT_3D('',#52528,#42859,#42860);
#35909=AXIS2_PLACEMENT_3D('',#52531,#42863,#42864);
#35910=AXIS2_PLACEMENT_3D('',#52538,#42868,#42869);
#35911=AXIS2_PLACEMENT_3D('',#52541,#42872,#42873);
#35912=AXIS2_PLACEMENT_3D('',#52544,#42876,#42877);
#35913=AXIS2_PLACEMENT_3D('',#52547,#42880,#42881);
#35914=AXIS2_PLACEMENT_3D('',#52550,#42884,#42885);
#35915=AXIS2_PLACEMENT_3D('',#52553,#42888,#42889);
#35916=AXIS2_PLACEMENT_3D('',#52556,#42892,#42893);
#35917=AXIS2_PLACEMENT_3D('',#52559,#42896,#42897);
#35918=AXIS2_PLACEMENT_3D('',#52560,#42898,#42899);
#35919=AXIS2_PLACEMENT_3D('',#52561,#42900,#42901);
#35920=AXIS2_PLACEMENT_3D('',#52562,#42902,#42903);
#35921=AXIS2_PLACEMENT_3D('',#52565,#42904,#42905);
#35922=AXIS2_PLACEMENT_3D('',#52566,#42906,#42907);
#35923=AXIS2_PLACEMENT_3D('',#52570,#42909,#42910);
#35924=AXIS2_PLACEMENT_3D('',#52571,#42911,#42912);
#35925=AXIS2_PLACEMENT_3D('',#52572,#42913,#42914);
#35926=AXIS2_PLACEMENT_3D('',#52576,#42916,#42917);
#35927=AXIS2_PLACEMENT_3D('',#52577,#42918,#42919);
#35928=AXIS2_PLACEMENT_3D('',#52578,#42920,#42921);
#35929=AXIS2_PLACEMENT_3D('',#52580,#42922,#42923);
#35930=AXIS2_PLACEMENT_3D('',#52582,#42925,#42926);
#35931=AXIS2_PLACEMENT_3D('',#52589,#42930,#42931);
#35932=AXIS2_PLACEMENT_3D('',#52596,#42935,#42936);
#35933=AXIS2_PLACEMENT_3D('',#52603,#42940,#42941);
#35934=AXIS2_PLACEMENT_3D('',#52606,#42944,#42945);
#35935=AXIS2_PLACEMENT_3D('',#52613,#42949,#42950);
#35936=AXIS2_PLACEMENT_3D('',#52616,#42953,#42954);
#35937=AXIS2_PLACEMENT_3D('',#52619,#42957,#42958);
#35938=AXIS2_PLACEMENT_3D('',#52622,#42961,#42962);
#35939=AXIS2_PLACEMENT_3D('',#52625,#42965,#42966);
#35940=AXIS2_PLACEMENT_3D('',#52628,#42969,#42970);
#35941=AXIS2_PLACEMENT_3D('',#52631,#42973,#42974);
#35942=AXIS2_PLACEMENT_3D('',#52634,#42977,#42978);
#35943=AXIS2_PLACEMENT_3D('',#52635,#42979,#42980);
#35944=AXIS2_PLACEMENT_3D('',#52636,#42981,#42982);
#35945=AXIS2_PLACEMENT_3D('',#52637,#42983,#42984);
#35946=AXIS2_PLACEMENT_3D('',#52644,#42988,#42989);
#35947=AXIS2_PLACEMENT_3D('',#52651,#42993,#42994);
#35948=AXIS2_PLACEMENT_3D('',#52658,#42998,#42999);
#35949=AXIS2_PLACEMENT_3D('',#52661,#43002,#43003);
#35950=AXIS2_PLACEMENT_3D('',#52668,#43007,#43008);
#35951=AXIS2_PLACEMENT_3D('',#52671,#43011,#43012);
#35952=AXIS2_PLACEMENT_3D('',#52674,#43015,#43016);
#35953=AXIS2_PLACEMENT_3D('',#52677,#43019,#43020);
#35954=AXIS2_PLACEMENT_3D('',#52680,#43023,#43024);
#35955=AXIS2_PLACEMENT_3D('',#52683,#43027,#43028);
#35956=AXIS2_PLACEMENT_3D('',#52686,#43031,#43032);
#35957=AXIS2_PLACEMENT_3D('',#52689,#43035,#43036);
#35958=AXIS2_PLACEMENT_3D('',#52690,#43037,#43038);
#35959=AXIS2_PLACEMENT_3D('',#52691,#43039,#43040);
#35960=AXIS2_PLACEMENT_3D('',#52692,#43041,#43042);
#35961=AXIS2_PLACEMENT_3D('',#52695,#43043,#43044);
#35962=AXIS2_PLACEMENT_3D('',#52696,#43045,#43046);
#35963=AXIS2_PLACEMENT_3D('',#52700,#43048,#43049);
#35964=AXIS2_PLACEMENT_3D('',#52701,#43050,#43051);
#35965=AXIS2_PLACEMENT_3D('',#52702,#43052,#43053);
#35966=AXIS2_PLACEMENT_3D('',#52706,#43055,#43056);
#35967=AXIS2_PLACEMENT_3D('',#52707,#43057,#43058);
#35968=AXIS2_PLACEMENT_3D('',#52708,#43059,#43060);
#35969=AXIS2_PLACEMENT_3D('',#52710,#43062,#43063);
#35970=AXIS2_PLACEMENT_3D('',#52712,#43064,#43065);
#35971=AXIS2_PLACEMENT_3D('',#52714,#43067,#43068);
#35972=AXIS2_PLACEMENT_3D('',#52716,#43069,#43070);
#35973=AXIS2_PLACEMENT_3D('',#52717,#43071,#43072);
#35974=AXIS2_PLACEMENT_3D('',#52719,#43073,#43074);
#35975=AXIS2_PLACEMENT_3D('',#52721,#43076,#43077);
#35976=AXIS2_PLACEMENT_3D('',#52724,#43079,#43080);
#35977=AXIS2_PLACEMENT_3D('',#52725,#43081,#43082);
#35978=AXIS2_PLACEMENT_3D('',#52727,#43084,#43085);
#35979=AXIS2_PLACEMENT_3D('',#52728,#43086,#43087);
#35980=AXIS2_PLACEMENT_3D('',#52729,#43088,#43089);
#35981=AXIS2_PLACEMENT_3D('',#52730,#43090,#43091);
#35982=AXIS2_PLACEMENT_3D('',#52731,#43092,#43093);
#35983=AXIS2_PLACEMENT_3D('',#52732,#43094,#43095);
#35984=AXIS2_PLACEMENT_3D('',#52733,#43096,#43097);
#35985=AXIS2_PLACEMENT_3D('',#52734,#43098,#43099);
#35986=AXIS2_PLACEMENT_3D('',#52735,#43100,#43101);
#35987=AXIS2_PLACEMENT_3D('',#52736,#43102,#43103);
#35988=AXIS2_PLACEMENT_3D('',#52737,#43104,#43105);
#35989=AXIS2_PLACEMENT_3D('',#52738,#43106,#43107);
#35990=AXIS2_PLACEMENT_3D('',#52739,#43108,#43109);
#35991=AXIS2_PLACEMENT_3D('',#52740,#43110,#43111);
#35992=AXIS2_PLACEMENT_3D('',#52741,#43112,#43113);
#35993=AXIS2_PLACEMENT_3D('',#52742,#43114,#43115);
#35994=AXIS2_PLACEMENT_3D('',#52743,#43116,#43117);
#35995=AXIS2_PLACEMENT_3D('',#52744,#43118,#43119);
#35996=AXIS2_PLACEMENT_3D('',#52745,#43120,#43121);
#35997=AXIS2_PLACEMENT_3D('',#52746,#43122,#43123);
#35998=AXIS2_PLACEMENT_3D('',#52747,#43124,#43125);
#35999=AXIS2_PLACEMENT_3D('',#52748,#43126,#43127);
#36000=AXIS2_PLACEMENT_3D('',#52749,#43128,#43129);
#36001=AXIS2_PLACEMENT_3D('',#52750,#43130,#43131);
#36002=AXIS2_PLACEMENT_3D('',#52751,#43132,#43133);
#36003=AXIS2_PLACEMENT_3D('',#52752,#43134,#43135);
#36004=AXIS2_PLACEMENT_3D('',#52753,#43136,#43137);
#36005=AXIS2_PLACEMENT_3D('',#52754,#43138,#43139);
#36006=AXIS2_PLACEMENT_3D('',#52755,#43140,#43141);
#36007=AXIS2_PLACEMENT_3D('',#52756,#43142,#43143);
#36008=AXIS2_PLACEMENT_3D('',#52757,#43144,#43145);
#36009=AXIS2_PLACEMENT_3D('',#52758,#43146,#43147);
#36010=AXIS2_PLACEMENT_3D('',#52759,#43148,#43149);
#36011=AXIS2_PLACEMENT_3D('',#52760,#43150,#43151);
#36012=AXIS2_PLACEMENT_3D('',#52761,#43152,#43153);
#36013=AXIS2_PLACEMENT_3D('',#52762,#43154,#43155);
#36014=AXIS2_PLACEMENT_3D('',#52763,#43156,#43157);
#36015=AXIS2_PLACEMENT_3D('',#52764,#43158,#43159);
#36016=AXIS2_PLACEMENT_3D('',#52765,#43160,#43161);
#36017=AXIS2_PLACEMENT_3D('',#52766,#43162,#43163);
#36018=AXIS2_PLACEMENT_3D('',#52767,#43164,#43165);
#36019=AXIS2_PLACEMENT_3D('',#52768,#43166,#43167);
#36020=AXIS2_PLACEMENT_3D('',#52769,#43168,#43169);
#36021=AXIS2_PLACEMENT_3D('',#52770,#43170,#43171);
#36022=AXIS2_PLACEMENT_3D('',#52771,#43172,#43173);
#36023=AXIS2_PLACEMENT_3D('',#52772,#43174,#43175);
#36024=AXIS2_PLACEMENT_3D('',#52773,#43176,#43177);
#36025=AXIS2_PLACEMENT_3D('',#52774,#43178,#43179);
#36026=AXIS2_PLACEMENT_3D('',#52775,#43180,#43181);
#36027=AXIS2_PLACEMENT_3D('',#52776,#43182,#43183);
#36028=AXIS2_PLACEMENT_3D('',#52777,#43184,#43185);
#36029=AXIS2_PLACEMENT_3D('',#52778,#43186,#43187);
#36030=AXIS2_PLACEMENT_3D('',#52779,#43188,#43189);
#36031=AXIS2_PLACEMENT_3D('',#52780,#43190,#43191);
#36032=AXIS2_PLACEMENT_3D('',#52781,#43192,#43193);
#36033=AXIS2_PLACEMENT_3D('',#52782,#43194,#43195);
#36034=AXIS2_PLACEMENT_3D('',#52783,#43196,#43197);
#36035=AXIS2_PLACEMENT_3D('',#52784,#43198,#43199);
#36036=AXIS2_PLACEMENT_3D('',#52785,#43200,#43201);
#36037=AXIS2_PLACEMENT_3D('',#52786,#43202,#43203);
#36038=AXIS2_PLACEMENT_3D('',#52787,#43204,#43205);
#36039=AXIS2_PLACEMENT_3D('',#52788,#43206,#43207);
#36040=AXIS2_PLACEMENT_3D('',#52789,#43208,#43209);
#36041=AXIS2_PLACEMENT_3D('',#52790,#43210,#43211);
#36042=AXIS2_PLACEMENT_3D('',#52791,#43212,#43213);
#36043=AXIS2_PLACEMENT_3D('',#52792,#43214,#43215);
#36044=AXIS2_PLACEMENT_3D('',#52793,#43216,#43217);
#36045=AXIS2_PLACEMENT_3D('',#52794,#43218,#43219);
#36046=AXIS2_PLACEMENT_3D('',#52795,#43220,#43221);
#36047=AXIS2_PLACEMENT_3D('',#52796,#43222,#43223);
#36048=AXIS2_PLACEMENT_3D('',#52797,#43224,#43225);
#36049=AXIS2_PLACEMENT_3D('',#52798,#43226,#43227);
#36050=AXIS2_PLACEMENT_3D('',#52799,#43228,#43229);
#36051=AXIS2_PLACEMENT_3D('',#52800,#43230,#43231);
#36052=AXIS2_PLACEMENT_3D('',#52801,#43232,#43233);
#36053=AXIS2_PLACEMENT_3D('',#52802,#43234,#43235);
#36054=AXIS2_PLACEMENT_3D('',#52803,#43236,#43237);
#36055=AXIS2_PLACEMENT_3D('',#52804,#43238,#43239);
#36056=AXIS2_PLACEMENT_3D('',#52805,#43240,#43241);
#36057=AXIS2_PLACEMENT_3D('',#52806,#43242,#43243);
#36058=AXIS2_PLACEMENT_3D('',#52807,#43244,#43245);
#36059=AXIS2_PLACEMENT_3D('',#52808,#43246,#43247);
#36060=AXIS2_PLACEMENT_3D('',#52809,#43248,#43249);
#36061=AXIS2_PLACEMENT_3D('',#52810,#43250,#43251);
#36062=AXIS2_PLACEMENT_3D('',#52811,#43252,#43253);
#36063=AXIS2_PLACEMENT_3D('',#52812,#43254,#43255);
#36064=AXIS2_PLACEMENT_3D('',#52813,#43256,#43257);
#36065=AXIS2_PLACEMENT_3D('',#52814,#43258,#43259);
#36066=AXIS2_PLACEMENT_3D('',#52815,#43260,#43261);
#36067=AXIS2_PLACEMENT_3D('',#52816,#43262,#43263);
#36068=AXIS2_PLACEMENT_3D('',#52817,#43264,#43265);
#36069=AXIS2_PLACEMENT_3D('',#52818,#43266,#43267);
#36070=AXIS2_PLACEMENT_3D('',#52819,#43268,#43269);
#36071=AXIS2_PLACEMENT_3D('',#52820,#43270,#43271);
#36072=AXIS2_PLACEMENT_3D('',#52821,#43272,#43273);
#36073=AXIS2_PLACEMENT_3D('',#52822,#43274,#43275);
#36074=AXIS2_PLACEMENT_3D('',#52823,#43276,#43277);
#36075=AXIS2_PLACEMENT_3D('',#52824,#43278,#43279);
#36076=AXIS2_PLACEMENT_3D('',#52825,#43280,#43281);
#36077=AXIS2_PLACEMENT_3D('',#52826,#43282,#43283);
#36078=AXIS2_PLACEMENT_3D('',#52827,#43284,#43285);
#36079=AXIS2_PLACEMENT_3D('',#52828,#43286,#43287);
#36080=AXIS2_PLACEMENT_3D('',#52829,#43288,#43289);
#36081=AXIS2_PLACEMENT_3D('',#52830,#43290,#43291);
#36082=AXIS2_PLACEMENT_3D('',#52831,#43292,#43293);
#36083=AXIS2_PLACEMENT_3D('',#52832,#43294,#43295);
#36084=AXIS2_PLACEMENT_3D('',#52833,#43296,#43297);
#36085=AXIS2_PLACEMENT_3D('',#52834,#43298,#43299);
#36086=AXIS2_PLACEMENT_3D('',#52835,#43300,#43301);
#36087=AXIS2_PLACEMENT_3D('',#52836,#43302,#43303);
#36088=AXIS2_PLACEMENT_3D('',#52837,#43304,#43305);
#36089=AXIS2_PLACEMENT_3D('',#52838,#43306,#43307);
#36090=AXIS2_PLACEMENT_3D('',#52839,#43308,#43309);
#36091=AXIS2_PLACEMENT_3D('',#52840,#43310,#43311);
#36092=AXIS2_PLACEMENT_3D('',#52841,#43312,#43313);
#36093=AXIS2_PLACEMENT_3D('',#52842,#43314,#43315);
#36094=AXIS2_PLACEMENT_3D('',#52843,#43316,#43317);
#36095=AXIS2_PLACEMENT_3D('',#52844,#43318,#43319);
#36096=AXIS2_PLACEMENT_3D('',#52845,#43320,#43321);
#36097=AXIS2_PLACEMENT_3D('',#52846,#43322,#43323);
#36098=AXIS2_PLACEMENT_3D('',#52847,#43324,#43325);
#36099=AXIS2_PLACEMENT_3D('',#52848,#43326,#43327);
#36100=AXIS2_PLACEMENT_3D('',#52849,#43328,#43329);
#36101=AXIS2_PLACEMENT_3D('',#52850,#43330,#43331);
#36102=AXIS2_PLACEMENT_3D('',#52851,#43332,#43333);
#36103=AXIS2_PLACEMENT_3D('',#52852,#43334,#43335);
#36104=AXIS2_PLACEMENT_3D('',#52853,#43336,#43337);
#36105=AXIS2_PLACEMENT_3D('',#52854,#43338,#43339);
#36106=AXIS2_PLACEMENT_3D('',#52855,#43340,#43341);
#36107=AXIS2_PLACEMENT_3D('',#52856,#43342,#43343);
#36108=AXIS2_PLACEMENT_3D('',#52857,#43344,#43345);
#36109=AXIS2_PLACEMENT_3D('',#52858,#43346,#43347);
#36110=AXIS2_PLACEMENT_3D('',#52859,#43348,#43349);
#36111=AXIS2_PLACEMENT_3D('',#52860,#43350,#43351);
#36112=AXIS2_PLACEMENT_3D('',#52861,#43352,#43353);
#36113=AXIS2_PLACEMENT_3D('',#52862,#43354,#43355);
#36114=AXIS2_PLACEMENT_3D('',#52863,#43356,#43357);
#36115=AXIS2_PLACEMENT_3D('',#52864,#43358,#43359);
#36116=AXIS2_PLACEMENT_3D('',#52865,#43360,#43361);
#36117=AXIS2_PLACEMENT_3D('',#52866,#43362,#43363);
#36118=AXIS2_PLACEMENT_3D('',#52867,#43364,#43365);
#36119=AXIS2_PLACEMENT_3D('',#52868,#43366,#43367);
#36120=AXIS2_PLACEMENT_3D('',#52869,#43368,#43369);
#36121=AXIS2_PLACEMENT_3D('',#52870,#43370,#43371);
#36122=AXIS2_PLACEMENT_3D('',#52871,#43372,#43373);
#36123=AXIS2_PLACEMENT_3D('',#52874,#43375,#43376);
#36124=AXIS2_PLACEMENT_3D('',#52875,#43377,#43378);
#36125=AXIS2_PLACEMENT_3D('',#52878,#43380,#43381);
#36126=AXIS2_PLACEMENT_3D('',#52879,#43382,#43383);
#36127=AXIS2_PLACEMENT_3D('',#52882,#43385,#43386);
#36128=AXIS2_PLACEMENT_3D('',#52883,#43387,#43388);
#36129=AXIS2_PLACEMENT_3D('',#52886,#43390,#43391);
#36130=AXIS2_PLACEMENT_3D('',#52887,#43392,#43393);
#36131=AXIS2_PLACEMENT_3D('',#52890,#43395,#43396);
#36132=AXIS2_PLACEMENT_3D('',#52891,#43397,#43398);
#36133=AXIS2_PLACEMENT_3D('',#52893,#43399,#43400);
#36134=AXIS2_PLACEMENT_3D('',#52896,#43402,#43403);
#36135=AXIS2_PLACEMENT_3D('',#52897,#43404,#43405);
#36136=AXIS2_PLACEMENT_3D('',#52900,#43407,#43408);
#36137=AXIS2_PLACEMENT_3D('',#52901,#43409,#43410);
#36138=AXIS2_PLACEMENT_3D('',#52904,#43412,#43413);
#36139=AXIS2_PLACEMENT_3D('',#52905,#43414,#43415);
#36140=AXIS2_PLACEMENT_3D('',#52908,#43417,#43418);
#36141=AXIS2_PLACEMENT_3D('',#52909,#43419,#43420);
#36142=AXIS2_PLACEMENT_3D('',#52912,#43422,#43423);
#36143=AXIS2_PLACEMENT_3D('',#52913,#43424,#43425);
#36144=AXIS2_PLACEMENT_3D('',#52914,#43426,#43427);
#36145=AXIS2_PLACEMENT_3D('',#52915,#43428,#43429);
#36146=AXIS2_PLACEMENT_3D('',#52916,#43430,#43431);
#36147=AXIS2_PLACEMENT_3D('',#52919,#43433,#43434);
#36148=AXIS2_PLACEMENT_3D('',#52920,#43435,#43436);
#36149=AXIS2_PLACEMENT_3D('',#52921,#43437,#43438);
#36150=AXIS2_PLACEMENT_3D('',#52924,#43440,#43441);
#36151=AXIS2_PLACEMENT_3D('',#52925,#43442,#43443);
#36152=AXIS2_PLACEMENT_3D('',#52926,#43444,#43445);
#36153=AXIS2_PLACEMENT_3D('',#52929,#43447,#43448);
#36154=AXIS2_PLACEMENT_3D('',#52930,#43449,#43450);
#36155=AXIS2_PLACEMENT_3D('',#52932,#43451,#43452);
#36156=AXIS2_PLACEMENT_3D('',#52933,#43453,#43454);
#36157=AXIS2_PLACEMENT_3D('',#52936,#43456,#43457);
#36158=AXIS2_PLACEMENT_3D('',#52937,#43458,#43459);
#36159=AXIS2_PLACEMENT_3D('',#52939,#43461,#43462);
#36160=AXIS2_PLACEMENT_3D('',#52941,#43463,#43464);
#36161=AXIS2_PLACEMENT_3D('',#52943,#43466,#43467);
#36162=AXIS2_PLACEMENT_3D('',#52945,#43468,#43469);
#36163=AXIS2_PLACEMENT_3D('',#52946,#43470,#43471);
#36164=AXIS2_PLACEMENT_3D('',#52949,#43473,#43474);
#36165=AXIS2_PLACEMENT_3D('',#52950,#43475,#43476);
#37663=DIRECTION('axis',(0.,0.,1.));
#37664=DIRECTION('refdir',(1.,0.,0.));
#37665=DIRECTION('center_axis',(1.,0.,3.3469968371114E-15));
#37666=DIRECTION('ref_axis',(0.,-1.,-3.0444058251673E-17));
#37667=DIRECTION('center_axis',(-1.,0.,0.));
#37668=DIRECTION('ref_axis',(0.,-1.,0.));
#37669=DIRECTION('center_axis',(-1.,0.,0.));
#37670=DIRECTION('ref_axis',(0.,-1.,0.));
#37671=DIRECTION('',(-0.85065080835204,-0.525731112119134,-2.92751444600949E-15));
#37672=DIRECTION('center_axis',(1.,0.,0.));
#37673=DIRECTION('ref_axis',(0.,-1.,-6.12323399573677E-17));
#37674=DIRECTION('center_axis',(1.,0.,0.));
#37675=DIRECTION('ref_axis',(0.,-1.,-6.12323399573677E-17));
#37676=DIRECTION('center_axis',(1.,0.,0.));
#37677=DIRECTION('ref_axis',(0.,1.,0.));
#37678=DIRECTION('',(-0.447213595499958,0.894427190999916,1.09535739652841E-16));
#37679=DIRECTION('center_axis',(-1.,0.,0.));
#37680=DIRECTION('ref_axis',(0.,-1.,-6.12323399573676E-17));
#37681=DIRECTION('center_axis',(-1.,0.,0.));
#37682=DIRECTION('ref_axis',(0.,-1.,-6.12323399573676E-17));
#37683=DIRECTION('center_axis',(1.,0.,0.));
#37684=DIRECTION('ref_axis',(0.,1.,0.));
#37685=DIRECTION('center_axis',(1.,0.,0.));
#37686=DIRECTION('ref_axis',(0.,0.,-1.));
#37687=DIRECTION('',(-1.,0.,0.));
#37688=DIRECTION('center_axis',(1.,0.,-1.02545205978024E-14));
#37689=DIRECTION('ref_axis',(0.,-1.,-3.10083423275242E-17));
#37690=DIRECTION('',(-0.229752920547362,-0.97324898946773,2.20663859235035E-15));
#37691=DIRECTION('center_axis',(1.,0.,0.));
#37692=DIRECTION('ref_axis',(0.,-1.,0.));
#37693=DIRECTION('center_axis',(-1.,0.,0.));
#37694=DIRECTION('ref_axis',(0.,0.,1.));
#37695=DIRECTION('center_axis',(1.,0.,0.));
#37696=DIRECTION('ref_axis',(0.,0.,-1.));
#37697=DIRECTION('center_axis',(-1.,0.,0.));
#37698=DIRECTION('ref_axis',(0.,-1.,0.));
#37699=DIRECTION('center_axis',(-1.,0.,0.));
#37700=DIRECTION('ref_axis',(0.,-1.,0.));
#37701=DIRECTION('',(0.707106781186548,-0.707106781186548,8.65956056235493E-17));
#37702=DIRECTION('center_axis',(1.,0.,0.));
#37703=DIRECTION('ref_axis',(0.,-1.,0.));
#37704=DIRECTION('center_axis',(1.,0.,0.));
#37705=DIRECTION('ref_axis',(0.,-1.,0.));
#37706=DIRECTION('center_axis',(1.,0.,0.));
#37707=DIRECTION('ref_axis',(0.,1.,0.));
#37708=DIRECTION('center_axis',(1.,0.,0.));
#37709=DIRECTION('ref_axis',(0.,0.,-1.));
#37710=DIRECTION('',(-1.,0.,0.));
#37711=DIRECTION('center_axis',(-1.,0.,0.));
#37712=DIRECTION('ref_axis',(0.,0.,1.));
#37713=DIRECTION('center_axis',(1.,0.,0.));
#37714=DIRECTION('ref_axis',(0.,0.,-1.));
#37715=DIRECTION('center_axis',(-1.,0.,-5.60335109986454E-15));
#37716=DIRECTION('ref_axis',(0.,-1.,-3.10254273231018E-17));
#37717=DIRECTION('center_axis',(-1.,0.,0.));
#37718=DIRECTION('ref_axis',(0.,-1.,0.));
#37719=DIRECTION('',(-0.38268343236509,0.923879532511287,-2.00250326312286E-15));
#37720=DIRECTION('center_axis',(1.,0.,0.));
#37721=DIRECTION('ref_axis',(0.,-1.,-6.12323399573677E-17));
#37722=DIRECTION('center_axis',(1.,0.,0.));
#37723=DIRECTION('ref_axis',(0.,-1.,-6.12323399573677E-17));
#37724=DIRECTION('center_axis',(-1.,0.,0.));
#37725=DIRECTION('ref_axis',(0.,1.,0.));
#37726=DIRECTION('',(-0.707106781186547,-0.707106781186548,-8.65956056235494E-17));
#37727=DIRECTION('center_axis',(-1.,0.,0.));
#37728=DIRECTION('ref_axis',(0.,-1.,-6.12323399573677E-17));
#37729=DIRECTION('center_axis',(-1.,0.,0.));
#37730=DIRECTION('ref_axis',(0.,-1.,-6.12323399573677E-17));
#37731=DIRECTION('center_axis',(1.,0.,0.));
#37732=DIRECTION('ref_axis',(0.,0.,-1.));
#37733=DIRECTION('center_axis',(1.,0.,0.));
#37734=DIRECTION('ref_axis',(0.,0.,-1.));
#37735=DIRECTION('center_axis',(-1.,0.,-2.93398870229358E-17));
#37736=DIRECTION('ref_axis',(0.,-1.,-6.12323399573676E-17));
#37737=DIRECTION('',(-0.901819525133682,0.43211288350113,5.29185659649989E-17));
#37738=DIRECTION('center_axis',(1.,0.,0.));
#37739=DIRECTION('ref_axis',(0.,-1.,-6.12323399573677E-17));
#37740=DIRECTION('center_axis',(1.,0.,0.));
#37741=DIRECTION('ref_axis',(0.,-1.,-6.12323399573677E-17));
#37742=DIRECTION('center_axis',(-1.,0.,0.));
#37743=DIRECTION('ref_axis',(0.,1.,0.));
#37744=DIRECTION('',(-0.994144463069456,-0.108059180768419,-1.3233432984653E-17));
#37745=DIRECTION('center_axis',(1.,0.,0.));
#37746=DIRECTION('ref_axis',(0.,0.,-1.));
#37747=DIRECTION('center_axis',(-1.,0.,-1.54843166437498E-16));
#37748=DIRECTION('ref_axis',(0.,-1.,-6.12323399573677E-17));
#37749=DIRECTION('center_axis',(-1.,0.,0.));
#37750=DIRECTION('ref_axis',(0.,-1.,-6.12323399573677E-17));
#37751=DIRECTION('center_axis',(-1.,0.,0.));
#37752=DIRECTION('ref_axis',(0.,-1.,-6.12323399573677E-17));
#37753=DIRECTION('',(-0.367738219294597,0.929929353268322,1.1388350059132E-16));
#37754=DIRECTION('center_axis',(1.,0.,0.));
#37755=DIRECTION('ref_axis',(0.,-1.,-6.12323399573677E-17));
#37756=DIRECTION('center_axis',(1.,0.,0.));
#37757=DIRECTION('ref_axis',(0.,-1.,-6.12323399573677E-17));
#37758=DIRECTION('center_axis',(-1.,0.,0.));
#37759=DIRECTION('ref_axis',(0.,1.,0.));
#37760=DIRECTION('',(-0.554700196225228,-0.832050294337845,-1.01896772969045E-16));
#37761=DIRECTION('center_axis',(-1.,0.,0.));
#37762=DIRECTION('ref_axis',(0.,-1.,-6.12323399573677E-17));
#37763=DIRECTION('center_axis',(-1.,0.,0.));
#37764=DIRECTION('ref_axis',(0.,-1.,-6.12323399573677E-17));
#37765=DIRECTION('center_axis',(-1.,0.,0.));
#37766=DIRECTION('ref_axis',(0.,1.,0.));
#37767=DIRECTION('center_axis',(1.,0.,0.));
#37768=DIRECTION('ref_axis',(0.,0.,-1.));
#37769=DIRECTION('',(-0.164398987305358,-0.986393923832144,-1.20798416151943E-16));
#37770=DIRECTION('center_axis',(-1.,0.,-6.47285581734468E-17));
#37771=DIRECTION('ref_axis',(0.,-1.,-6.12323399573677E-17));
#37772=DIRECTION('',(-0.687215388498205,0.726453721727173,8.89649225041859E-17));
#37773=DIRECTION('center_axis',(1.,0.,0.));
#37774=DIRECTION('ref_axis',(0.,-1.,-6.12323399573677E-17));
#37775=DIRECTION('center_axis',(1.,0.,0.));
#37776=DIRECTION('ref_axis',(0.,-1.,-6.12323399573677E-17));
#37777=DIRECTION('center_axis',(-1.,0.,0.));
#37778=DIRECTION('ref_axis',(0.,1.,0.));
#37779=DIRECTION('',(-0.800000000000001,-0.599999999999999,-7.34788079488411E-17));
#37780=DIRECTION('center_axis',(-1.,0.,0.));
#37781=DIRECTION('ref_axis',(0.,-1.,-6.12323399573677E-17));
#37782=DIRECTION('center_axis',(-1.,0.,0.));
#37783=DIRECTION('ref_axis',(0.,-1.,-6.12323399573677E-17));
#37784=DIRECTION('center_axis',(-1.,0.,-3.35417469620003E-17));
#37785=DIRECTION('ref_axis',(0.,-1.,-6.12323399573677E-17));
#37786=DIRECTION('',(-0.877037421408632,0.480422065947118,5.8834734530191E-17));
#37787=DIRECTION('center_axis',(1.,0.,0.));
#37788=DIRECTION('ref_axis',(0.,-1.,-6.12323399573677E-17));
#37789=DIRECTION('center_axis',(1.,0.,0.));
#37790=DIRECTION('ref_axis',(0.,-1.,-6.12323399573677E-17));
#37791=DIRECTION('center_axis',(-1.,0.,0.));
#37792=DIRECTION('ref_axis',(0.,1.,0.));
#37793=DIRECTION('',(-0.936329177569044,-0.351123441588392,-4.30002198846827E-17));
#37794=DIRECTION('center_axis',(-1.,0.,0.));
#37795=DIRECTION('ref_axis',(0.,-1.,-6.12323399573676E-17));
#37796=DIRECTION('center_axis',(-1.,0.,0.));
#37797=DIRECTION('ref_axis',(0.,-1.,-6.12323399573676E-17));
#37798=DIRECTION('center_axis',(-1.,0.,8.59032469848147E-15));
#37799=DIRECTION('ref_axis',(0.,-1.,-3.0596396085212E-17));
#37800=DIRECTION('',(-0.983953550115309,0.17842480549374,8.47979037642802E-15));
#37801=DIRECTION('center_axis',(1.,0.,0.));
#37802=DIRECTION('ref_axis',(0.,-1.,0.));
#37803=DIRECTION('center_axis',(1.,0.,0.));
#37804=DIRECTION('ref_axis',(0.,-1.,0.));
#37805=DIRECTION('center_axis',(1.,0.,0.));
#37806=DIRECTION('ref_axis',(0.,1.,0.));
#37807=DIRECTION('',(-1.,0.,0.));
#37808=DIRECTION('center_axis',(1.,0.,0.));
#37809=DIRECTION('ref_axis',(0.,1.,0.));
#37810=DIRECTION('center_axis',(0.707106781186548,-0.070359754473029,-0.703597544730291));
#37811=DIRECTION('ref_axis',(0.707106781186547,0.0703597544730292,0.703597544730293));
#37812=DIRECTION('',(-1.,0.,0.));
#37813=DIRECTION('center_axis',(-0.707106781186548,-0.0703597544730291,
-0.703597544730292));
#37814=DIRECTION('ref_axis',(-0.707106781186547,0.0703597544730291,0.703597544730292));
#37815=DIRECTION('center_axis',(-1.,0.,0.));
#37816=DIRECTION('ref_axis',(0.,1.,0.));
#37817=DIRECTION('',(-1.,0.,0.));
#37818=DIRECTION('center_axis',(1.,0.,0.));
#37819=DIRECTION('ref_axis',(0.,0.,-1.));
#37820=DIRECTION('center_axis',(-1.,0.,0.));
#37821=DIRECTION('ref_axis',(0.,1.,0.));
#37822=DIRECTION('center_axis',(-0.707106781186547,-0.0703597544730291,
0.703597544730292));
#37823=DIRECTION('ref_axis',(-0.707106781186548,0.0703597544730291,-0.703597544730291));
#37824=DIRECTION('',(1.,0.,0.));
#37825=DIRECTION('center_axis',(0.707106781186548,-0.070359754473029,0.703597544730291));
#37826=DIRECTION('ref_axis',(0.707106781186547,0.0703597544730292,-0.703597544730293));
#37827=DIRECTION('center_axis',(1.,0.,0.));
#37828=DIRECTION('ref_axis',(0.,1.,0.));
#37829=DIRECTION('',(-1.,0.,0.));
#37830=DIRECTION('center_axis',(-0.707106781186548,-0.703597544730292,0.0703597544730291));
#37831=DIRECTION('ref_axis',(-0.707106781186547,0.703597544730292,-0.0703597544730291));
#37832=DIRECTION('center_axis',(-1.,0.,0.));
#37833=DIRECTION('ref_axis',(0.,1.,0.));
#37834=DIRECTION('center_axis',(-0.707106781186547,0.703597544730292,0.0703597544730291));
#37835=DIRECTION('ref_axis',(0.707106781186548,0.703597544730291,0.070359754473029));
#37836=DIRECTION('',(1.,0.,0.));
#37837=DIRECTION('center_axis',(0.707106781186548,0.703597544730291,0.070359754473029));
#37838=DIRECTION('ref_axis',(-0.707106781186547,0.703597544730293,0.0703597544730292));
#37839=DIRECTION('center_axis',(1.,0.,0.));
#37840=DIRECTION('ref_axis',(0.,1.,0.));
#37841=DIRECTION('center_axis',(0.707106781186548,-0.703597544730291,0.070359754473029));
#37842=DIRECTION('ref_axis',(0.707106781186547,0.703597544730293,-0.0703597544730292));
#37843=DIRECTION('',(-1.,0.,0.));
#37844=DIRECTION('center_axis',(-0.707106781186548,-0.707052400311326,0.00876944775867132));
#37845=DIRECTION('ref_axis',(-0.707106781186547,0.707052400311326,-0.00876944775867133));
#37846=DIRECTION('center_axis',(-1.,0.,0.));
#37847=DIRECTION('ref_axis',(0.,1.,0.));
#37848=DIRECTION('center_axis',(-0.707106781186548,0.694787886990046,0.131414580971466));
#37849=DIRECTION('ref_axis',(0.707106781186547,0.694787886990047,0.131414580971466));
#37850=DIRECTION('',(1.,0.,0.));
#37851=DIRECTION('center_axis',(0.707106781186549,0.694787886990045,0.131414580971465));
#37852=DIRECTION('ref_axis',(-0.707106781186546,0.694787886990049,0.131414580971466));
#37853=DIRECTION('center_axis',(1.,0.,0.));
#37854=DIRECTION('ref_axis',(0.,1.,0.));
#37855=DIRECTION('center_axis',(0.707106781186549,-0.707052400311325,0.00876944775867131));
#37856=DIRECTION('ref_axis',(0.707106781186546,0.707052400311328,-0.00876944775867135));
#37857=DIRECTION('',(-1.,0.,0.));
#37858=DIRECTION('center_axis',(-0.707106781186545,-0.705126160196082,-0.0528875997482674));
#37859=DIRECTION('ref_axis',(-0.70710678118655,0.705126160196077,0.052887599748267));
#37860=DIRECTION('center_axis',(-1.,0.,0.));
#37861=DIRECTION('ref_axis',(0.,1.,0.));
#37862=DIRECTION('center_axis',(-0.707106781186538,0.68069047390542,0.191469263158419));
#37863=DIRECTION('ref_axis',(0.707106781186557,0.680690473905402,0.191469263158414));
#37864=DIRECTION('',(1.,0.,0.));
#37865=DIRECTION('center_axis',(0.707106781186543,0.680690473905416,0.191469263158417));
#37866=DIRECTION('ref_axis',(-0.707106781186552,0.680690473905407,0.191469263158415));
#37867=DIRECTION('center_axis',(1.,0.,0.));
#37868=DIRECTION('ref_axis',(0.,1.,0.));
#37869=DIRECTION('center_axis',(0.70710678118655,-0.705126160196078,-0.0528875997482671));
#37870=DIRECTION('ref_axis',(0.707106781186546,0.705126160196081,0.0528875997482674));
#37871=DIRECTION('',(-1.,0.,0.));
#37872=DIRECTION('center_axis',(-0.70710678118655,-0.697833484234922,-0.114142140686715));
#37873=DIRECTION('ref_axis',(-0.707106781186545,0.697833484234926,0.114142140686716));
#37874=DIRECTION('center_axis',(-1.,0.,0.));
#37875=DIRECTION('ref_axis',(0.,1.,0.));
#37876=DIRECTION('center_axis',(-0.707106781186541,0.661412595302216,0.250066748640431));
#37877=DIRECTION('ref_axis',(0.707106781186554,0.661412595302203,0.250066748640426));
#37878=DIRECTION('',(1.,0.,0.));
#37879=DIRECTION('center_axis',(0.707106781186545,0.661412595302212,0.25006674864043));
#37880=DIRECTION('ref_axis',(-0.70710678118655,0.661412595302208,0.250066748640428));
#37881=DIRECTION('center_axis',(1.,0.,0.));
#37882=DIRECTION('ref_axis',(0.,1.,0.));
#37883=DIRECTION('center_axis',(0.707106781186551,-0.697833484234921,-0.114142140686715));
#37884=DIRECTION('ref_axis',(0.707106781186544,0.697833484234928,0.114142140686716));
#37885=DIRECTION('',(-1.,0.,0.));
#37886=DIRECTION('center_axis',(-0.707106781186539,-0.685229874095371,-0.174527991013631));
#37887=DIRECTION('ref_axis',(-0.707106781186556,0.685229874095354,0.174527991013627));
#37888=DIRECTION('center_axis',(-1.,0.,0.));
#37889=DIRECTION('ref_axis',(0.,1.,0.));
#37890=DIRECTION('center_axis',(-0.707106781186553,0.637100967476909,0.306761075170854));
#37891=DIRECTION('ref_axis',(0.707106781186542,0.637100967476919,0.306761075170859));
#37892=DIRECTION('',(1.,0.,0.));
#37893=DIRECTION('center_axis',(0.707106781186549,0.637100967476913,0.306761075170856));
#37894=DIRECTION('ref_axis',(-0.707106781186546,0.637100967476915,0.306761075170857));
#37895=DIRECTION('center_axis',(1.,0.,0.));
#37896=DIRECTION('ref_axis',(0.,1.,0.));
#37897=DIRECTION('center_axis',(0.707106781186534,-0.685229874095376,-0.174527991013633));
#37898=DIRECTION('ref_axis',(0.707106781186561,0.68522987409535,0.174527991013626));
#37899=DIRECTION('',(-1.,0.,0.));
#37900=DIRECTION('center_axis',(-0.707106781186562,-0.667411250860812,-0.233585577946042));
#37901=DIRECTION('ref_axis',(-0.707106781186534,0.667411250860838,0.233585577946052));
#37902=DIRECTION('center_axis',(-1.,0.,0.));
#37903=DIRECTION('ref_axis',(0.,1.,0.));
#37904=DIRECTION('center_axis',(-0.707106781186546,0.607940616597039,0.361120764691834));
#37905=DIRECTION('ref_axis',(0.707106781186549,0.607940616597036,0.361120764691832));
#37906=DIRECTION('',(1.,0.,0.));
#37907=DIRECTION('center_axis',(0.707106781186553,0.607940616597033,0.36112076469183));
#37908=DIRECTION('ref_axis',(-0.707106781186542,0.607940616597042,0.361120764691836));
#37909=DIRECTION('center_axis',(1.,0.,0.));
#37910=DIRECTION('ref_axis',(0.,1.,0.));
#37911=DIRECTION('center_axis',(0.707106781186557,-0.667411250860816,-0.233585577946044));
#37912=DIRECTION('ref_axis',(0.707106781186538,0.667411250860834,0.23358557794605));
#37913=DIRECTION('',(-1.,0.,0.));
#37914=DIRECTION('center_axis',(-0.707106781186555,-0.644513225013298,-0.290865437587464));
#37915=DIRECTION('ref_axis',(-0.70710678118654,0.644513225013312,0.29086543758747));
#37916=DIRECTION('center_axis',(-1.,0.,0.));
#37917=DIRECTION('ref_axis',(0.,1.,0.));
#37918=DIRECTION('center_axis',(-0.707106781186541,0.574153470540282,0.412732107142829));
#37919=DIRECTION('ref_axis',(0.707106781186554,0.574153470540271,0.412732107142821));
#37920=DIRECTION('',(1.,0.,0.));
#37921=DIRECTION('center_axis',(0.707106781186542,0.57415347054028,0.412732107142828));
#37922=DIRECTION('ref_axis',(-0.707106781186553,0.574153470540272,0.412732107142822));
#37923=DIRECTION('center_axis',(1.,0.,0.));
#37924=DIRECTION('ref_axis',(0.,1.,0.));
#37925=DIRECTION('center_axis',(0.707106781186557,-0.644513225013297,-0.290865437587463));
#37926=DIRECTION('ref_axis',(0.707106781186538,0.644513225013314,0.290865437587471));
#37927=DIRECTION('',(-1.,0.,0.));
#37928=DIRECTION('center_axis',(-0.707106781186539,-0.616710064355716,-0.345931635619497));
#37929=DIRECTION('ref_axis',(-0.707106781186556,0.616710064355701,0.345931635619489));
#37930=DIRECTION('center_axis',(-1.,0.,0.));
#37931=DIRECTION('ref_axis',(0.,1.,0.));
#37932=DIRECTION('center_axis',(-0.707106781186546,0.535996669889361,0.461202309044001));
#37933=DIRECTION('ref_axis',(0.707106781186549,0.535996669889358,0.461202309043999));
#37934=DIRECTION('',(1.,0.,0.));
#37935=DIRECTION('center_axis',(0.707106781186547,0.53599666988936,0.461202309044));
#37936=DIRECTION('ref_axis',(-0.707106781186548,0.535996669889359,0.461202309044));
#37937=DIRECTION('center_axis',(1.,0.,0.));
#37938=DIRECTION('ref_axis',(0.,1.,0.));
#37939=DIRECTION('center_axis',(0.707106781186546,-0.61671006435571,-0.345931635619494));
#37940=DIRECTION('ref_axis',(0.707106781186549,0.616710064355707,0.345931635619493));
#37941=DIRECTION('',(-1.,0.,0.));
#37942=DIRECTION('center_axis',(-0.70710678118654,-0.584213367728653,-0.398365085025227));
#37943=DIRECTION('ref_axis',(-0.707106781186555,0.584213367728641,0.398365085025218));
#37944=DIRECTION('center_axis',(-1.,0.,0.));
#37945=DIRECTION('ref_axis',(0.,1.,0.));
#37946=DIRECTION('center_axis',(-0.70710678118654,0.493760610936952,0.506162482891787));
#37947=DIRECTION('ref_axis',(0.707106781186555,0.493760610936941,0.506162482891777));
#37948=DIRECTION('',(1.,0.,0.));
#37949=DIRECTION('center_axis',(0.707106781186551,0.493760610936944,0.50616248289178));
#37950=DIRECTION('ref_axis',(-0.707106781186545,0.493760610936949,0.506162482891784));
#37951=DIRECTION('center_axis',(1.,0.,0.));
#37952=DIRECTION('ref_axis',(0.,1.,0.));
#37953=DIRECTION('center_axis',(0.707106781186542,-0.584213367728652,-0.398365085025226));
#37954=DIRECTION('ref_axis',(0.707106781186553,0.584213367728642,0.398365085025219));
#37955=DIRECTION('',(-1.,0.,0.));
#37956=DIRECTION('center_axis',(-0.70710678118655,-0.547270454615492,-0.447766735594494));
#37957=DIRECTION('ref_axis',(-0.707106781186545,0.547270454615496,0.447766735594497));
#37958=DIRECTION('center_axis',(-1.,0.,0.));
#37959=DIRECTION('ref_axis',(0.,1.,0.));
#37960=DIRECTION('center_axis',(-0.70710678118655,0.447766735594494,0.547270454615492));
#37961=DIRECTION('ref_axis',(0.707106781186545,0.447766735594497,0.547270454615496));
#37962=DIRECTION('',(1.,0.,0.));
#37963=DIRECTION('center_axis',(0.707106781186552,0.447766735594493,0.547270454615491));
#37964=DIRECTION('ref_axis',(-0.707106781186544,0.447766735594498,0.547270454615497));
#37965=DIRECTION('center_axis',(1.,0.,0.));
#37966=DIRECTION('ref_axis',(0.,1.,0.));
#37967=DIRECTION('center_axis',(0.707106781186552,-0.547270454615491,-0.447766735594493));
#37968=DIRECTION('ref_axis',(0.707106781186544,0.547270454615497,0.447766735594498));
#37969=DIRECTION('',(-1.,0.,0.));
#37970=DIRECTION('center_axis',(-0.707106781186558,-0.506162482891774,-0.493760610936939));
#37971=DIRECTION('ref_axis',(-0.707106781186537,0.506162482891789,0.493760610936954));
#37972=DIRECTION('center_axis',(-1.,0.,0.));
#37973=DIRECTION('ref_axis',(0.,1.,0.));
#37974=DIRECTION('center_axis',(-0.707106781186547,0.398365085025223,0.584213367728647));
#37975=DIRECTION('ref_axis',(0.707106781186548,0.398365085025222,0.584213367728647));
#37976=DIRECTION('',(1.,0.,0.));
#37977=DIRECTION('center_axis',(0.707106781186549,0.398365085025222,0.584213367728646));
#37978=DIRECTION('ref_axis',(-0.707106781186546,0.398365085025223,0.584213367728648));
#37979=DIRECTION('center_axis',(1.,0.,0.));
#37980=DIRECTION('ref_axis',(0.,1.,0.));
#37981=DIRECTION('center_axis',(0.707106781186551,-0.50616248289178,-0.493760610936944));
#37982=DIRECTION('ref_axis',(0.707106781186544,0.506162482891784,0.493760610936949));
#37983=DIRECTION('',(-1.,0.,0.));
#37984=DIRECTION('center_axis',(-0.707106781186551,-0.461202309043998,-0.535996669889357));
#37985=DIRECTION('ref_axis',(-0.707106781186545,0.461202309044002,0.535996669889362));
#37986=DIRECTION('center_axis',(-1.,0.,0.));
#37987=DIRECTION('ref_axis',(0.,1.,0.));
#37988=DIRECTION('center_axis',(-0.707106781186545,0.345931635619495,0.616710064355711));
#37989=DIRECTION('ref_axis',(0.70710678118655,0.345931635619492,0.616710064355706));
#37990=DIRECTION('',(1.,0.,0.));
#37991=DIRECTION('center_axis',(0.707106781186546,0.345931635619494,0.61671006435571));
#37992=DIRECTION('ref_axis',(-0.707106781186549,0.345931635619493,0.616710064355707));
#37993=DIRECTION('center_axis',(1.,0.,0.));
#37994=DIRECTION('ref_axis',(0.,1.,0.));
#37995=DIRECTION('center_axis',(0.707106781186552,-0.461202309043997,-0.535996669889356));
#37996=DIRECTION('ref_axis',(0.707106781186543,0.461202309044003,0.535996669889363));
#37997=DIRECTION('',(-1.,0.,0.));
#37998=DIRECTION('center_axis',(-0.707106781186541,-0.412732107142829,-0.574153470540282));
#37999=DIRECTION('ref_axis',(-0.707106781186554,0.412732107142821,0.57415347054027));
#38000=DIRECTION('center_axis',(-1.,0.,0.));
#38001=DIRECTION('ref_axis',(0.,1.,0.));
#38002=DIRECTION('center_axis',(-0.707106781186549,0.290865437587466,0.644513225013304));
#38003=DIRECTION('ref_axis',(0.707106781186546,0.290865437587468,0.644513225013307));
#38004=DIRECTION('',(1.,0.,0.));
#38005=DIRECTION('center_axis',(0.707106781186551,0.290865437587466,0.644513225013302));
#38006=DIRECTION('ref_axis',(-0.707106781186544,0.290865437587468,0.644513225013308));
#38007=DIRECTION('center_axis',(1.,0.,0.));
#38008=DIRECTION('ref_axis',(0.,1.,0.));
#38009=DIRECTION('center_axis',(0.707106781186555,-0.412732107142821,-0.57415347054027));
#38010=DIRECTION('ref_axis',(0.70710678118654,0.412732107142829,0.574153470540282));
#38011=DIRECTION('',(-1.,0.,0.));
#38012=DIRECTION('center_axis',(-0.707106781186551,-0.361120764691831,-0.607940616597034));
#38013=DIRECTION('ref_axis',(-0.707106781186544,0.361120764691835,0.60794061659704));
#38014=DIRECTION('center_axis',(-1.,0.,0.));
#38015=DIRECTION('ref_axis',(0.,1.,0.));
#38016=DIRECTION('center_axis',(-0.70710678118655,0.233585577946046,0.667411250860823));
#38017=DIRECTION('ref_axis',(0.707106781186545,0.233585577946048,0.667411250860827));
#38018=DIRECTION('',(1.,0.,0.));
#38019=DIRECTION('center_axis',(0.707106781186551,0.233585577946046,0.667411250860822));
#38020=DIRECTION('ref_axis',(-0.707106781186544,0.233585577946048,0.667411250860829));
#38021=DIRECTION('center_axis',(1.,0.,0.));
#38022=DIRECTION('ref_axis',(0.,1.,0.));
#38023=DIRECTION('center_axis',(0.707106781186553,-0.36112076469183,-0.607940616597033));
#38024=DIRECTION('ref_axis',(0.707106781186542,0.361120764691836,0.607940616597042));
#38025=DIRECTION('',(-1.,0.,0.));
#38026=DIRECTION('center_axis',(-0.707106781186547,-0.306761075170857,-0.637100967476915));
#38027=DIRECTION('ref_axis',(-0.707106781186548,0.306761075170857,0.637100967476914));
#38028=DIRECTION('center_axis',(-1.,0.,0.));
#38029=DIRECTION('ref_axis',(0.,1.,0.));
#38030=DIRECTION('center_axis',(-0.707106781186539,0.174527991013632,0.685229874095371));
#38031=DIRECTION('ref_axis',(0.707106781186556,0.174527991013627,0.685229874095354));
#38032=DIRECTION('',(1.,0.,0.));
#38033=DIRECTION('center_axis',(0.70710678118654,0.174527991013631,0.68522987409537));
#38034=DIRECTION('ref_axis',(-0.707106781186555,0.174527991013628,0.685229874095355));
#38035=DIRECTION('center_axis',(1.,0.,0.));
#38036=DIRECTION('ref_axis',(0.,1.,0.));
#38037=DIRECTION('center_axis',(0.707106781186549,-0.306761075170856,-0.637100967476913));
#38038=DIRECTION('ref_axis',(0.707106781186547,0.306761075170857,0.637100967476915));
#38039=DIRECTION('',(-1.,0.,0.));
#38040=DIRECTION('center_axis',(-0.707106781186544,-0.25006674864043,-0.661412595302213));
#38041=DIRECTION('ref_axis',(-0.707106781186551,0.250066748640427,0.661412595302206));
#38042=DIRECTION('center_axis',(-1.,0.,0.));
#38043=DIRECTION('ref_axis',(0.,1.,0.));
#38044=DIRECTION('center_axis',(-0.707106781186546,0.114142140686716,0.697833484234925));
#38045=DIRECTION('ref_axis',(0.707106781186548,0.114142140686716,0.697833484234923));
#38046=DIRECTION('',(1.,0.,0.));
#38047=DIRECTION('center_axis',(0.707106781186548,0.114142140686716,0.697833484234924));
#38048=DIRECTION('ref_axis',(-0.707106781186547,0.114142140686716,0.697833484234925));
#38049=DIRECTION('center_axis',(1.,0.,0.));
#38050=DIRECTION('ref_axis',(0.,1.,0.));
#38051=DIRECTION('center_axis',(0.707106781186545,-0.25006674864043,-0.661412595302212));
#38052=DIRECTION('ref_axis',(0.70710678118655,0.250066748640428,0.661412595302208));
#38053=DIRECTION('',(-1.,0.,0.));
#38054=DIRECTION('center_axis',(-0.707106781186544,-0.191469263158417,-0.680690473905414));
#38055=DIRECTION('ref_axis',(-0.707106781186551,0.191469263158415,0.680690473905408));
#38056=DIRECTION('center_axis',(-1.,0.,0.));
#38057=DIRECTION('ref_axis',(0.,1.,0.));
#38058=DIRECTION('center_axis',(-0.707106781186545,0.0528875997482675,0.705126160196082));
#38059=DIRECTION('ref_axis',(0.70710678118655,0.0528875997482671,0.705126160196077));
#38060=DIRECTION('',(1.,0.,0.));
#38061=DIRECTION('center_axis',(0.707106781186546,0.0528875997482674,0.705126160196081));
#38062=DIRECTION('ref_axis',(-0.707106781186549,0.0528875997482673,0.705126160196078));
#38063=DIRECTION('center_axis',(1.,0.,0.));
#38064=DIRECTION('ref_axis',(0.,1.,0.));
#38065=DIRECTION('center_axis',(0.707106781186546,-0.191469263158417,-0.680690473905413));
#38066=DIRECTION('ref_axis',(0.707106781186549,0.191469263158416,0.68069047390541));
#38067=DIRECTION('',(-1.,0.,0.));
#38068=DIRECTION('center_axis',(-0.707106781186545,-0.131414580971466,-0.694787886990049));
#38069=DIRECTION('ref_axis',(-0.70710678118655,0.131414580971465,0.694787886990044));
#38070=DIRECTION('center_axis',(-1.,0.,0.));
#38071=DIRECTION('ref_axis',(0.,1.,0.));
#38072=DIRECTION('center_axis',(-0.707106781186548,-0.00876944775867119,
0.707052400311326));
#38073=DIRECTION('ref_axis',(-0.707106781186547,0.00876944775867126,-0.707052400311326));
#38074=DIRECTION('',(1.,0.,0.));
#38075=DIRECTION('center_axis',(0.707106781186549,-0.00876944775867117,
0.707052400311324));
#38076=DIRECTION('ref_axis',(0.707106781186546,0.00876944775867128,-0.707052400311328));
#38077=DIRECTION('center_axis',(1.,0.,0.));
#38078=DIRECTION('ref_axis',(0.,1.,0.));
#38079=DIRECTION('center_axis',(0.707106781186545,-0.131414580971466,-0.694787886990049));
#38080=DIRECTION('ref_axis',(0.70710678118655,0.131414580971465,0.694787886990044));
#38081=DIRECTION('',(-1.,0.,0.));
#38082=DIRECTION('center_axis',(-0.707106781186548,-0.00876944775867143,
-0.707052400311326));
#38083=DIRECTION('ref_axis',(-0.707106781186547,0.00876944775867142,0.707052400311326));
#38084=DIRECTION('center_axis',(-1.,0.,0.));
#38085=DIRECTION('ref_axis',(0.,1.,0.));
#38086=DIRECTION('center_axis',(-0.707106781186548,-0.131414580971466,0.694787886990046));
#38087=DIRECTION('ref_axis',(-0.707106781186547,0.131414580971466,-0.694787886990047));
#38088=DIRECTION('',(1.,0.,0.));
#38089=DIRECTION('center_axis',(0.707106781186549,-0.131414580971465,0.694787886990045));
#38090=DIRECTION('ref_axis',(0.707106781186546,0.131414580971466,-0.694787886990049));
#38091=DIRECTION('center_axis',(1.,0.,0.));
#38092=DIRECTION('ref_axis',(0.,1.,0.));
#38093=DIRECTION('center_axis',(0.707106781186549,-0.00876944775867141,
-0.707052400311324));
#38094=DIRECTION('ref_axis',(0.707106781186546,0.00876944775867144,0.707052400311328));
#38095=DIRECTION('',(-1.,0.,0.));
#38096=DIRECTION('center_axis',(-0.707106781186548,0.0528875997482672,-0.705126160196079));
#38097=DIRECTION('ref_axis',(0.707106781186547,0.0528875997482672,-0.70512616019608));
#38098=DIRECTION('center_axis',(-1.,0.,0.));
#38099=DIRECTION('ref_axis',(0.,1.,0.));
#38100=DIRECTION('center_axis',(-0.707106781186538,-0.191469263158419,0.68069047390542));
#38101=DIRECTION('ref_axis',(-0.707106781186557,0.191469263158414,-0.680690473905402));
#38102=DIRECTION('',(1.,0.,0.));
#38103=DIRECTION('center_axis',(0.707106781186546,-0.191469263158417,0.680690473905413));
#38104=DIRECTION('ref_axis',(0.707106781186549,0.191469263158416,-0.68069047390541));
#38105=DIRECTION('center_axis',(1.,0.,0.));
#38106=DIRECTION('ref_axis',(0.,1.,0.));
#38107=DIRECTION('center_axis',(0.707106781186549,0.0528875997482671,-0.705126160196077));
#38108=DIRECTION('ref_axis',(-0.707106781186546,0.0528875997482673,-0.705126160196081));
#38109=DIRECTION('',(-1.,0.,0.));
#38110=DIRECTION('center_axis',(-0.70710678118655,0.114142140686715,-0.697833484234922));
#38111=DIRECTION('ref_axis',(0.707106781186545,0.114142140686716,-0.697833484234926));
#38112=DIRECTION('center_axis',(-1.,0.,0.));
#38113=DIRECTION('ref_axis',(0.,1.,0.));
#38114=DIRECTION('center_axis',(-0.707106781186544,-0.25006674864043,0.661412595302213));
#38115=DIRECTION('ref_axis',(-0.707106781186551,0.250066748640427,-0.661412595302206));
#38116=DIRECTION('',(1.,0.,0.));
#38117=DIRECTION('center_axis',(0.707106781186545,-0.25006674864043,0.661412595302212));
#38118=DIRECTION('ref_axis',(0.70710678118655,0.250066748640428,-0.661412595302208));
#38119=DIRECTION('center_axis',(1.,0.,0.));
#38120=DIRECTION('ref_axis',(0.,1.,0.));
#38121=DIRECTION('center_axis',(0.707106781186545,0.114142140686716,-0.697833484234927));
#38122=DIRECTION('ref_axis',(-0.70710678118655,0.114142140686715,-0.697833484234922));
#38123=DIRECTION('',(-1.,0.,0.));
#38124=DIRECTION('center_axis',(-0.707106781186539,0.174527991013631,-0.685229874095371));
#38125=DIRECTION('ref_axis',(0.707106781186556,0.174527991013627,-0.685229874095354));
#38126=DIRECTION('center_axis',(-1.,0.,0.));
#38127=DIRECTION('ref_axis',(0.,1.,0.));
#38128=DIRECTION('center_axis',(-0.707106781186553,-0.306761075170854,0.637100967476909));
#38129=DIRECTION('ref_axis',(-0.707106781186542,0.306761075170859,-0.637100967476919));
#38130=DIRECTION('',(1.,0.,0.));
#38131=DIRECTION('center_axis',(0.707106781186549,-0.306761075170856,0.637100967476913));
#38132=DIRECTION('ref_axis',(0.707106781186546,0.306761075170857,-0.637100967476915));
#38133=DIRECTION('center_axis',(1.,0.,0.));
#38134=DIRECTION('ref_axis',(0.,1.,0.));
#38135=DIRECTION('center_axis',(0.707106781186534,0.174527991013633,-0.685229874095376));
#38136=DIRECTION('ref_axis',(-0.707106781186561,0.174527991013626,-0.68522987409535));
#38137=DIRECTION('',(-1.,0.,0.));
#38138=DIRECTION('center_axis',(-0.70710678118655,0.233585577946046,-0.667411250860823));
#38139=DIRECTION('ref_axis',(0.707106781186545,0.233585577946048,-0.667411250860827));
#38140=DIRECTION('center_axis',(-1.,0.,0.));
#38141=DIRECTION('ref_axis',(0.,1.,0.));
#38142=DIRECTION('center_axis',(-0.70710678118654,-0.361120764691837,0.607940616597043));
#38143=DIRECTION('ref_axis',(-0.707106781186555,0.361120764691829,-0.607940616597031));
#38144=DIRECTION('',(1.,0.,0.));
#38145=DIRECTION('center_axis',(0.707106781186547,-0.361120764691833,0.607940616597037));
#38146=DIRECTION('ref_axis',(0.707106781186548,0.361120764691833,-0.607940616597037));
#38147=DIRECTION('center_axis',(1.,0.,0.));
#38148=DIRECTION('ref_axis',(0.,1.,0.));
#38149=DIRECTION('center_axis',(0.707106781186551,0.233585577946046,-0.667411250860822));
#38150=DIRECTION('ref_axis',(-0.707106781186544,0.233585577946048,-0.667411250860829));
#38151=DIRECTION('',(-1.,0.,0.));
#38152=DIRECTION('center_axis',(-0.707106781186549,0.290865437587466,-0.644513225013304));
#38153=DIRECTION('ref_axis',(0.707106781186546,0.290865437587468,-0.644513225013307));
#38154=DIRECTION('center_axis',(-1.,0.,0.));
#38155=DIRECTION('ref_axis',(0.,1.,0.));
#38156=DIRECTION('center_axis',(-0.707106781186541,-0.412732107142829,0.574153470540282));
#38157=DIRECTION('ref_axis',(-0.707106781186554,0.412732107142821,-0.57415347054027));
#38158=DIRECTION('',(1.,0.,0.));
#38159=DIRECTION('center_axis',(0.707106781186542,-0.412732107142828,0.57415347054028));
#38160=DIRECTION('ref_axis',(0.707106781186553,0.412732107142822,-0.574153470540272));
#38161=DIRECTION('center_axis',(1.,0.,0.));
#38162=DIRECTION('ref_axis',(0.,1.,0.));
#38163=DIRECTION('center_axis',(0.707106781186551,0.290865437587465,-0.644513225013302));
#38164=DIRECTION('ref_axis',(-0.707106781186544,0.290865437587468,-0.644513225013308));
#38165=DIRECTION('',(-1.,0.,0.));
#38166=DIRECTION('center_axis',(-0.707106781186545,0.345931635619494,-0.616710064355711));
#38167=DIRECTION('ref_axis',(0.70710678118655,0.345931635619492,-0.616710064355706));
#38168=DIRECTION('center_axis',(-1.,0.,0.));
#38169=DIRECTION('ref_axis',(0.,1.,0.));
#38170=DIRECTION('center_axis',(-0.707106781186546,-0.461202309044001,0.535996669889361));
#38171=DIRECTION('ref_axis',(-0.707106781186549,0.461202309043999,-0.535996669889358));
#38172=DIRECTION('',(1.,0.,0.));
#38173=DIRECTION('center_axis',(0.707106781186547,-0.461202309044,0.53599666988936));
#38174=DIRECTION('ref_axis',(0.707106781186548,0.461202309044,-0.535996669889359));
#38175=DIRECTION('center_axis',(1.,0.,0.));
#38176=DIRECTION('ref_axis',(0.,1.,0.));
#38177=DIRECTION('center_axis',(0.707106781186546,0.345931635619494,-0.61671006435571));
#38178=DIRECTION('ref_axis',(-0.707106781186549,0.345931635619492,-0.616710064355708));
#38179=DIRECTION('',(-1.,0.,0.));
#38180=DIRECTION('center_axis',(-0.70710678118654,0.398365085025227,-0.584213367728653));
#38181=DIRECTION('ref_axis',(0.707106781186555,0.398365085025218,-0.584213367728641));
#38182=DIRECTION('center_axis',(-1.,0.,0.));
#38183=DIRECTION('ref_axis',(0.,1.,0.));
#38184=DIRECTION('center_axis',(-0.707106781186549,-0.506162482891781,0.493760610936946));
#38185=DIRECTION('ref_axis',(-0.707106781186546,0.506162482891783,-0.493760610936947));
#38186=DIRECTION('',(1.,0.,0.));
#38187=DIRECTION('center_axis',(0.707106781186551,-0.50616248289178,0.493760610936944));
#38188=DIRECTION('ref_axis',(0.707106781186544,0.506162482891784,-0.493760610936949));
#38189=DIRECTION('center_axis',(1.,0.,0.));
#38190=DIRECTION('ref_axis',(0.,1.,0.));
#38191=DIRECTION('center_axis',(0.707106781186542,0.398365085025226,-0.584213367728652));
#38192=DIRECTION('ref_axis',(-0.707106781186554,0.398365085025219,-0.584213367728642));
#38193=DIRECTION('',(-1.,0.,0.));
#38194=DIRECTION('center_axis',(-0.70710678118655,0.447766735594494,-0.547270454615492));
#38195=DIRECTION('ref_axis',(0.707106781186545,0.447766735594497,-0.547270454615496));
#38196=DIRECTION('center_axis',(-1.,0.,0.));
#38197=DIRECTION('ref_axis',(0.,1.,0.));
#38198=DIRECTION('center_axis',(-0.70710678118655,-0.547270454615492,0.447766735594494));
#38199=DIRECTION('ref_axis',(-0.707106781186545,0.547270454615496,-0.447766735594497));
#38200=DIRECTION('',(1.,0.,0.));
#38201=DIRECTION('center_axis',(0.707106781186552,-0.547270454615491,0.447766735594493));
#38202=DIRECTION('ref_axis',(0.707106781186544,0.547270454615497,-0.447766735594498));
#38203=DIRECTION('center_axis',(1.,0.,0.));
#38204=DIRECTION('ref_axis',(0.,1.,0.));
#38205=DIRECTION('center_axis',(0.707106781186551,0.447766735594493,-0.547270454615491));
#38206=DIRECTION('ref_axis',(-0.707106781186544,0.447766735594498,-0.547270454615497));
#38207=DIRECTION('',(-1.,0.,0.));
#38208=DIRECTION('center_axis',(-0.707106781186558,0.493760610936939,-0.506162482891774));
#38209=DIRECTION('ref_axis',(0.707106781186537,0.493760610936954,-0.50616248289179));
#38210=DIRECTION('center_axis',(-1.,0.,0.));
#38211=DIRECTION('ref_axis',(0.,1.,0.));
#38212=DIRECTION('center_axis',(-0.707106781186547,-0.584213367728647,0.398365085025223));
#38213=DIRECTION('ref_axis',(-0.707106781186548,0.584213367728646,-0.398365085025223));
#38214=DIRECTION('',(1.,0.,0.));
#38215=DIRECTION('center_axis',(0.707106781186549,-0.584213367728646,0.398365085025222));
#38216=DIRECTION('ref_axis',(0.707106781186546,0.584213367728648,-0.398365085025223));
#38217=DIRECTION('center_axis',(1.,0.,0.));
#38218=DIRECTION('ref_axis',(0.,1.,0.));
#38219=DIRECTION('center_axis',(0.70710678118656,0.493760610936938,-0.506162482891773));
#38220=DIRECTION('ref_axis',(-0.707106781186535,0.493760610936955,-0.506162482891791));
#38221=DIRECTION('',(-1.,0.,0.));
#38222=DIRECTION('center_axis',(-0.707106781186541,0.535996669889364,-0.461202309044004));
#38223=DIRECTION('ref_axis',(0.707106781186554,0.535996669889354,-0.461202309043996));
#38224=DIRECTION('center_axis',(-1.,0.,0.));
#38225=DIRECTION('ref_axis',(0.,1.,0.));
#38226=DIRECTION('center_axis',(-0.707106781186545,-0.616710064355711,0.345931635619495));
#38227=DIRECTION('ref_axis',(-0.70710678118655,0.616710064355706,-0.345931635619492));
#38228=DIRECTION('',(1.,0.,0.));
#38229=DIRECTION('center_axis',(0.707106781186546,-0.61671006435571,0.345931635619494));
#38230=DIRECTION('ref_axis',(0.707106781186549,0.616710064355707,-0.345931635619493));
#38231=DIRECTION('center_axis',(1.,0.,0.));
#38232=DIRECTION('ref_axis',(0.,1.,0.));
#38233=DIRECTION('center_axis',(0.707106781186552,0.535996669889356,-0.461202309043997));
#38234=DIRECTION('ref_axis',(-0.707106781186543,0.535996669889363,-0.461202309044003));
#38235=DIRECTION('',(-1.,0.,0.));
#38236=DIRECTION('center_axis',(-0.707106781186546,0.574153470540278,-0.412732107142826));
#38237=DIRECTION('ref_axis',(0.707106781186549,0.574153470540275,-0.412732107142824));
#38238=DIRECTION('center_axis',(-1.,0.,0.));
#38239=DIRECTION('ref_axis',(0.,1.,0.));
#38240=DIRECTION('center_axis',(-0.707106781186555,-0.644513225013298,0.290865437587464));
#38241=DIRECTION('ref_axis',(-0.70710678118654,0.644513225013312,-0.29086543758747));
#38242=DIRECTION('',(1.,0.,0.));
#38243=DIRECTION('center_axis',(0.707106781186551,-0.644513225013302,0.290865437587466));
#38244=DIRECTION('ref_axis',(0.707106781186544,0.644513225013308,-0.290865437587468));
#38245=DIRECTION('center_axis',(1.,0.,0.));
#38246=DIRECTION('ref_axis',(0.,1.,0.));
#38247=DIRECTION('center_axis',(0.707106781186547,0.574153470540276,-0.412732107142825));
#38248=DIRECTION('ref_axis',(-0.707106781186548,0.574153470540276,-0.412732107142825));
#38249=DIRECTION('',(-1.,0.,0.));
#38250=DIRECTION('center_axis',(-0.707106781186546,0.607940616597039,-0.361120764691834));
#38251=DIRECTION('ref_axis',(0.707106781186549,0.607940616597036,-0.361120764691832));
#38252=DIRECTION('center_axis',(-1.,0.,0.));
#38253=DIRECTION('ref_axis',(0.,1.,0.));
#38254=DIRECTION('center_axis',(-0.707106781186556,-0.667411250860817,0.233585577946044));
#38255=DIRECTION('ref_axis',(-0.707106781186539,0.667411250860833,-0.23358557794605));
#38256=DIRECTION('',(1.,0.,0.));
#38257=DIRECTION('center_axis',(0.707106781186557,-0.667411250860816,0.233585577946044));
#38258=DIRECTION('ref_axis',(0.707106781186538,0.667411250860834,-0.23358557794605));
#38259=DIRECTION('center_axis',(1.,0.,0.));
#38260=DIRECTION('ref_axis',(0.,1.,0.));
#38261=DIRECTION('center_axis',(0.707106781186547,0.607940616597037,-0.361120764691833));
#38262=DIRECTION('ref_axis',(-0.707106781186548,0.607940616597037,-0.361120764691833));
#38263=DIRECTION('',(-1.,0.,0.));
#38264=DIRECTION('center_axis',(-0.707106781186541,0.63710096747692,-0.30676107517086));
#38265=DIRECTION('ref_axis',(0.707106781186554,0.637100967476909,-0.306761075170854));
#38266=DIRECTION('center_axis',(-1.,0.,0.));
#38267=DIRECTION('ref_axis',(0.,1.,0.));
#38268=DIRECTION('center_axis',(-0.707106781186539,-0.685229874095371,0.174527991013632));
#38269=DIRECTION('ref_axis',(-0.707106781186556,0.685229874095354,-0.174527991013627));
#38270=DIRECTION('',(1.,0.,0.));
#38271=DIRECTION('center_axis',(0.70710678118654,-0.68522987409537,0.174527991013631));
#38272=DIRECTION('ref_axis',(0.707106781186555,0.685229874095355,-0.174527991013628));
#38273=DIRECTION('center_axis',(1.,0.,0.));
#38274=DIRECTION('ref_axis',(0.,1.,0.));
#38275=DIRECTION('center_axis',(0.707106781186549,0.637100967476913,-0.306761075170856));
#38276=DIRECTION('ref_axis',(-0.707106781186547,0.637100967476915,-0.306761075170857));
#38277=DIRECTION('',(-1.,0.,0.));
#38278=DIRECTION('center_axis',(-0.707106781186547,0.66141259530221,-0.250066748640429));
#38279=DIRECTION('ref_axis',(0.707106781186548,0.661412595302209,-0.250066748640429));
#38280=DIRECTION('center_axis',(-1.,0.,0.));
#38281=DIRECTION('ref_axis',(0.,1.,0.));
#38282=DIRECTION('center_axis',(-0.707106781186546,-0.697833484234925,0.114142140686716));
#38283=DIRECTION('ref_axis',(-0.707106781186549,0.697833484234923,-0.114142140686716));
#38284=DIRECTION('',(1.,0.,0.));
#38285=DIRECTION('center_axis',(0.707106781186548,-0.697833484234924,0.114142140686716));
#38286=DIRECTION('ref_axis',(0.707106781186547,0.697833484234924,-0.114142140686716));
#38287=DIRECTION('center_axis',(1.,0.,0.));
#38288=DIRECTION('ref_axis',(0.,1.,0.));
#38289=DIRECTION('center_axis',(0.707106781186545,0.661412595302212,-0.25006674864043));
#38290=DIRECTION('ref_axis',(-0.70710678118655,0.661412595302207,-0.250066748640428));
#38291=DIRECTION('',(-1.,0.,0.));
#38292=DIRECTION('center_axis',(-0.707106781186541,0.680690473905417,-0.191469263158418));
#38293=DIRECTION('ref_axis',(0.707106781186554,0.680690473905405,-0.191469263158415));
#38294=DIRECTION('center_axis',(-1.,0.,0.));
#38295=DIRECTION('ref_axis',(0.,1.,0.));
#38296=DIRECTION('center_axis',(-0.707106781186551,-0.705126160196076,0.0528875997482672));
#38297=DIRECTION('ref_axis',(-0.707106781186544,0.705126160196083,-0.0528875997482678));
#38298=DIRECTION('',(1.,0.,0.));
#38299=DIRECTION('center_axis',(0.707106781186553,-0.705126160196074,0.0528875997482671));
#38300=DIRECTION('ref_axis',(0.707106781186542,0.705126160196085,-0.0528875997482679));
#38301=DIRECTION('center_axis',(1.,0.,0.));
#38302=DIRECTION('ref_axis',(0.,1.,0.));
#38303=DIRECTION('center_axis',(0.707106781186543,0.680690473905416,-0.191469263158418));
#38304=DIRECTION('ref_axis',(-0.707106781186552,0.680690473905407,-0.191469263158415));
#38305=DIRECTION('',(-1.,0.,0.));
#38306=DIRECTION('center_axis',(-0.707106781186546,0.694787886990048,-0.131414580971466));
#38307=DIRECTION('ref_axis',(0.707106781186549,0.694787886990046,-0.131414580971466));
#38308=DIRECTION('center_axis',(-1.,0.,0.));
#38309=DIRECTION('ref_axis',(0.,1.,0.));
#38310=DIRECTION('center_axis',(-0.707106781186549,-0.707052400311325,-0.00876944775867129));
#38311=DIRECTION('ref_axis',(-0.707106781186546,0.707052400311328,0.00876944775867133));
#38312=DIRECTION('',(1.,0.,0.));
#38313=DIRECTION('center_axis',(0.707106781186549,-0.707052400311325,-0.00876944775867129));
#38314=DIRECTION('ref_axis',(0.707106781186546,0.707052400311328,0.00876944775867133));
#38315=DIRECTION('center_axis',(1.,0.,0.));
#38316=DIRECTION('ref_axis',(0.,1.,0.));
#38317=DIRECTION('center_axis',(0.707106781186546,0.694787886990048,-0.131414580971466));
#38318=DIRECTION('ref_axis',(-0.707106781186549,0.694787886990046,-0.131414580971466));
#38319=DIRECTION('',(-1.,0.,0.));
#38320=DIRECTION('center_axis',(-0.707106781186548,0.703597544730292,-0.0703597544730292));
#38321=DIRECTION('ref_axis',(0.707106781186547,0.703597544730292,-0.0703597544730292));
#38322=DIRECTION('center_axis',(-1.,0.,0.));
#38323=DIRECTION('ref_axis',(0.,1.,0.));
#38324=DIRECTION('center_axis',(-0.707106781186548,-0.703597544730292,-0.070359754473029));
#38325=DIRECTION('ref_axis',(-0.707106781186547,0.703597544730292,0.070359754473029));
#38326=DIRECTION('',(1.,0.,0.));
#38327=DIRECTION('center_axis',(0.707106781186549,-0.70359754473029,-0.0703597544730288));
#38328=DIRECTION('ref_axis',(0.707106781186546,0.703597544730294,0.0703597544730292));
#38329=DIRECTION('center_axis',(1.,0.,0.));
#38330=DIRECTION('ref_axis',(0.,1.,0.));
#38331=DIRECTION('center_axis',(0.707106781186548,0.703597544730291,-0.0703597544730291));
#38332=DIRECTION('ref_axis',(-0.707106781186547,0.703597544730293,-0.0703597544730293));
#38333=DIRECTION('',(-1.,0.,0.));
#38334=DIRECTION('center_axis',(-0.707106781186548,0.707052400311326,-0.00876944775867148));
#38335=DIRECTION('ref_axis',(0.707106781186547,0.707052400311326,-0.00876944775867149));
#38336=DIRECTION('center_axis',(-1.,0.,0.));
#38337=DIRECTION('ref_axis',(0.,1.,0.));
#38338=DIRECTION('center_axis',(-0.707106781186548,-0.694787886990046,-0.131414580971466));
#38339=DIRECTION('ref_axis',(-0.707106781186547,0.694787886990047,0.131414580971466));
#38340=DIRECTION('',(1.,0.,0.));
#38341=DIRECTION('center_axis',(0.707106781186549,-0.694787886990045,-0.131414580971465));
#38342=DIRECTION('ref_axis',(0.707106781186546,0.694787886990049,0.131414580971466));
#38343=DIRECTION('center_axis',(1.,0.,0.));
#38344=DIRECTION('ref_axis',(0.,1.,0.));
#38345=DIRECTION('center_axis',(0.707106781186549,0.707052400311325,-0.00876944775867146));
#38346=DIRECTION('ref_axis',(-0.707106781186546,0.707052400311328,-0.0087694477586715));
#38347=DIRECTION('',(-1.,0.,0.));
#38348=DIRECTION('center_axis',(-0.707106781186545,0.705126160196082,0.0528875997482672));
#38349=DIRECTION('ref_axis',(0.70710678118655,0.705126160196077,0.0528875997482668));
#38350=DIRECTION('center_axis',(-1.,0.,0.));
#38351=DIRECTION('ref_axis',(0.,1.,0.));
#38352=DIRECTION('center_axis',(-0.707106781186538,-0.68069047390542,-0.191469263158418));
#38353=DIRECTION('ref_axis',(-0.707106781186557,0.680690473905402,0.191469263158413));
#38354=DIRECTION('',(1.,0.,0.));
#38355=DIRECTION('center_axis',(0.707106781186543,-0.680690473905416,-0.191469263158417));
#38356=DIRECTION('ref_axis',(0.707106781186552,0.680690473905407,0.191469263158415));
#38357=DIRECTION('center_axis',(1.,0.,0.));
#38358=DIRECTION('ref_axis',(0.,1.,0.));
#38359=DIRECTION('center_axis',(0.70710678118655,0.705126160196078,0.0528875997482669));
#38360=DIRECTION('ref_axis',(-0.707106781186546,0.705126160196081,0.0528875997482672));
#38361=DIRECTION('',(-1.,0.,0.));
#38362=DIRECTION('center_axis',(-0.707106781186546,0.697833484234925,0.114142140686716));
#38363=DIRECTION('ref_axis',(0.707106781186548,0.697833484234923,0.114142140686716));
#38364=DIRECTION('center_axis',(-1.,0.,0.));
#38365=DIRECTION('ref_axis',(0.,1.,0.));
#38366=DIRECTION('center_axis',(-0.707106781186544,-0.661412595302213,-0.25006674864043));
#38367=DIRECTION('ref_axis',(-0.707106781186551,0.661412595302206,0.250066748640427));
#38368=DIRECTION('',(1.,0.,0.));
#38369=DIRECTION('center_axis',(0.707106781186545,-0.661412595302212,-0.25006674864043));
#38370=DIRECTION('ref_axis',(0.70710678118655,0.661412595302208,0.250066748640428));
#38371=DIRECTION('center_axis',(1.,0.,0.));
#38372=DIRECTION('ref_axis',(0.,1.,0.));
#38373=DIRECTION('center_axis',(0.707106781186551,0.697833484234921,0.114142140686715));
#38374=DIRECTION('ref_axis',(-0.707106781186544,0.697833484234928,0.114142140686716));
#38375=DIRECTION('',(-1.,0.,0.));
#38376=DIRECTION('center_axis',(-0.707106781186533,0.685229874095377,0.174527991013633));
#38377=DIRECTION('ref_axis',(0.707106781186563,0.685229874095348,0.174527991013626));
#38378=DIRECTION('center_axis',(-1.,0.,0.));
#38379=DIRECTION('ref_axis',(0.,1.,0.));
#38380=DIRECTION('center_axis',(-0.707106781186553,-0.637100967476909,-0.306761075170854));
#38381=DIRECTION('ref_axis',(-0.707106781186542,0.637100967476919,0.306761075170859));
#38382=DIRECTION('',(1.,0.,0.));
#38383=DIRECTION('center_axis',(0.707106781186549,-0.637100967476913,-0.306761075170856));
#38384=DIRECTION('ref_axis',(0.707106781186546,0.637100967476915,0.306761075170857));
#38385=DIRECTION('center_axis',(1.,0.,0.));
#38386=DIRECTION('ref_axis',(0.,1.,0.));
#38387=DIRECTION('center_axis',(0.707106781186534,0.685229874095376,0.174527991013633));
#38388=DIRECTION('ref_axis',(-0.707106781186561,0.68522987409535,0.174527991013626));
#38389=DIRECTION('',(-1.,0.,0.));
#38390=DIRECTION('center_axis',(-0.707106781186556,0.667411250860817,0.233585577946044));
#38391=DIRECTION('ref_axis',(0.707106781186539,0.667411250860833,0.233585577946049));
#38392=DIRECTION('center_axis',(-1.,0.,0.));
#38393=DIRECTION('ref_axis',(0.,1.,0.));
#38394=DIRECTION('center_axis',(-0.707106781186546,-0.607940616597039,-0.361120764691834));
#38395=DIRECTION('ref_axis',(-0.707106781186549,0.607940616597036,0.361120764691832));
#38396=DIRECTION('',(1.,0.,0.));
#38397=DIRECTION('center_axis',(0.707106781186547,-0.607940616597037,-0.361120764691833));
#38398=DIRECTION('ref_axis',(0.707106781186548,0.607940616597037,0.361120764691833));
#38399=DIRECTION('center_axis',(1.,0.,0.));
#38400=DIRECTION('ref_axis',(0.,1.,0.));
#38401=DIRECTION('center_axis',(0.707106781186557,0.667411250860816,0.233585577946044));
#38402=DIRECTION('ref_axis',(-0.707106781186538,0.667411250860834,0.23358557794605));
#38403=DIRECTION('',(-1.,0.,0.));
#38404=DIRECTION('center_axis',(-0.707106781186549,0.644513225013304,0.290865437587466));
#38405=DIRECTION('ref_axis',(0.707106781186546,0.644513225013307,0.290865437587467));
#38406=DIRECTION('center_axis',(-1.,0.,0.));
#38407=DIRECTION('ref_axis',(0.,1.,0.));
#38408=DIRECTION('center_axis',(-0.707106781186541,-0.574153470540282,-0.412732107142829));
#38409=DIRECTION('ref_axis',(-0.707106781186554,0.574153470540271,0.412732107142821));
#38410=DIRECTION('',(1.,0.,0.));
#38411=DIRECTION('center_axis',(0.707106781186542,-0.574153470540281,-0.412732107142828));
#38412=DIRECTION('ref_axis',(0.707106781186553,0.574153470540272,0.412732107142822));
#38413=DIRECTION('center_axis',(1.,0.,0.));
#38414=DIRECTION('ref_axis',(0.,1.,0.));
#38415=DIRECTION('center_axis',(0.707106781186551,0.644513225013302,0.290865437587465));
#38416=DIRECTION('ref_axis',(-0.707106781186544,0.644513225013308,0.290865437587468));
#38417=DIRECTION('',(-1.,0.,0.));
#38418=DIRECTION('center_axis',(-0.707106781186545,0.616710064355711,0.345931635619494));
#38419=DIRECTION('ref_axis',(0.70710678118655,0.616710064355706,0.345931635619492));
#38420=DIRECTION('center_axis',(-1.,0.,0.));
#38421=DIRECTION('ref_axis',(0.,1.,0.));
#38422=DIRECTION('center_axis',(-0.707106781186546,-0.535996669889361,-0.461202309044001));
#38423=DIRECTION('ref_axis',(-0.707106781186549,0.535996669889358,0.461202309043999));
#38424=DIRECTION('',(1.,0.,0.));
#38425=DIRECTION('center_axis',(0.707106781186547,-0.53599666988936,-0.461202309044));
#38426=DIRECTION('ref_axis',(0.707106781186548,0.535996669889359,0.461202309044));
#38427=DIRECTION('center_axis',(1.,0.,0.));
#38428=DIRECTION('ref_axis',(0.,1.,0.));
#38429=DIRECTION('center_axis',(0.707106781186546,0.61671006435571,0.345931635619494));
#38430=DIRECTION('ref_axis',(-0.707106781186549,0.616710064355708,0.345931635619492));
#38431=DIRECTION('',(-1.,0.,0.));
#38432=DIRECTION('center_axis',(-0.70710678118654,0.584213367728653,0.398365085025227));
#38433=DIRECTION('ref_axis',(0.707106781186555,0.584213367728641,0.398365085025218));
#38434=DIRECTION('center_axis',(-1.,0.,0.));
#38435=DIRECTION('ref_axis',(0.,1.,0.));
#38436=DIRECTION('center_axis',(-0.70710678118654,-0.493760610936952,-0.506162482891787));
#38437=DIRECTION('ref_axis',(-0.707106781186555,0.493760610936941,0.506162482891777));
#38438=DIRECTION('',(1.,0.,0.));
#38439=DIRECTION('center_axis',(0.707106781186551,-0.493760610936944,-0.50616248289178));
#38440=DIRECTION('ref_axis',(0.707106781186545,0.493760610936949,0.506162482891784));
#38441=DIRECTION('center_axis',(1.,0.,0.));
#38442=DIRECTION('ref_axis',(0.,1.,0.));
#38443=DIRECTION('center_axis',(0.707106781186542,0.584213367728652,0.398365085025226));
#38444=DIRECTION('ref_axis',(-0.707106781186553,0.584213367728642,0.398365085025219));
#38445=DIRECTION('',(-1.,0.,0.));
#38446=DIRECTION('center_axis',(-0.707106781186558,0.547270454615486,0.447766735594489));
#38447=DIRECTION('ref_axis',(0.707106781186537,0.547270454615502,0.447766735594502));
#38448=DIRECTION('center_axis',(-1.,0.,0.));
#38449=DIRECTION('ref_axis',(0.,1.,0.));
#38450=DIRECTION('center_axis',(-0.70710678118655,-0.447766735594494,-0.547270454615492));
#38451=DIRECTION('ref_axis',(-0.707106781186545,0.447766735594497,0.547270454615496));
#38452=DIRECTION('',(1.,0.,0.));
#38453=DIRECTION('center_axis',(0.707106781186551,-0.447766735594493,-0.547270454615491));
#38454=DIRECTION('ref_axis',(0.707106781186544,0.447766735594498,0.547270454615497));
#38455=DIRECTION('center_axis',(1.,0.,0.));
#38456=DIRECTION('ref_axis',(0.,1.,0.));
#38457=DIRECTION('center_axis',(0.707106781186551,0.547270454615491,0.447766735594493));
#38458=DIRECTION('ref_axis',(-0.707106781186544,0.547270454615497,0.447766735594498));
#38459=DIRECTION('',(-1.,0.,0.));
#38460=DIRECTION('center_axis',(-0.707106781186558,0.506162482891774,0.493760610936939));
#38461=DIRECTION('ref_axis',(0.707106781186537,0.506162482891789,0.493760610936954));
#38462=DIRECTION('center_axis',(-1.,0.,0.));
#38463=DIRECTION('ref_axis',(0.,1.,0.));
#38464=DIRECTION('center_axis',(-0.707106781186547,-0.398365085025223,-0.584213367728647));
#38465=DIRECTION('ref_axis',(-0.707106781186548,0.398365085025223,0.584213367728646));
#38466=DIRECTION('',(1.,0.,0.));
#38467=DIRECTION('center_axis',(0.707106781186549,-0.398365085025222,-0.584213367728646));
#38468=DIRECTION('ref_axis',(0.707106781186546,0.398365085025223,0.584213367728648));
#38469=DIRECTION('center_axis',(1.,0.,0.));
#38470=DIRECTION('ref_axis',(0.,1.,0.));
#38471=DIRECTION('center_axis',(0.70710678118656,0.506162482891773,0.493760610936938));
#38472=DIRECTION('ref_axis',(-0.707106781186535,0.506162482891791,0.493760610936955));
#38473=DIRECTION('',(-1.,0.,0.));
#38474=DIRECTION('center_axis',(-0.707106781186541,0.461202309044004,0.535996669889364));
#38475=DIRECTION('ref_axis',(0.707106781186554,0.461202309043996,0.535996669889354));
#38476=DIRECTION('center_axis',(-1.,0.,0.));
#38477=DIRECTION('ref_axis',(0.,1.,0.));
#38478=DIRECTION('center_axis',(-0.707106781186545,-0.345931635619495,-0.616710064355711));
#38479=DIRECTION('ref_axis',(-0.70710678118655,0.345931635619492,0.616710064355706));
#38480=DIRECTION('',(1.,0.,0.));
#38481=DIRECTION('center_axis',(0.707106781186546,-0.345931635619494,-0.61671006435571));
#38482=DIRECTION('ref_axis',(0.707106781186549,0.345931635619493,0.616710064355707));
#38483=DIRECTION('center_axis',(1.,0.,0.));
#38484=DIRECTION('ref_axis',(0.,1.,0.));
#38485=DIRECTION('center_axis',(0.707106781186552,0.461202309043997,0.535996669889356));
#38486=DIRECTION('ref_axis',(-0.707106781186543,0.461202309044003,0.535996669889363));
#38487=DIRECTION('',(-1.,0.,0.));
#38488=DIRECTION('center_axis',(-0.707106781186536,0.412732107142832,0.574153470540286));
#38489=DIRECTION('ref_axis',(0.707106781186559,0.412732107142818,0.574153470540266));
#38490=DIRECTION('center_axis',(-1.,0.,0.));
#38491=DIRECTION('ref_axis',(0.,1.,0.));
#38492=DIRECTION('center_axis',(-0.707106781186549,-0.290865437587467,-0.644513225013303));
#38493=DIRECTION('ref_axis',(-0.707106781186546,0.290865437587468,0.644513225013307));
#38494=DIRECTION('',(1.,0.,0.));
#38495=DIRECTION('center_axis',(0.707106781186551,-0.290865437587466,-0.644513225013302));
#38496=DIRECTION('ref_axis',(0.707106781186544,0.290865437587469,0.644513225013308));
#38497=DIRECTION('center_axis',(1.,0.,0.));
#38498=DIRECTION('ref_axis',(0.,1.,0.));
#38499=DIRECTION('center_axis',(0.707106781186547,0.412732107142825,0.574153470540276));
#38500=DIRECTION('ref_axis',(-0.707106781186548,0.412732107142825,0.574153470540276));
#38501=DIRECTION('',(-1.,0.,0.));
#38502=DIRECTION('center_axis',(-0.707106781186546,0.361120764691834,0.607940616597038));
#38503=DIRECTION('ref_axis',(0.707106781186549,0.361120764691833,0.607940616597036));
#38504=DIRECTION('center_axis',(-1.,0.,0.));
#38505=DIRECTION('ref_axis',(0.,1.,0.));
#38506=DIRECTION('center_axis',(-0.70710678118655,-0.233585577946047,-0.667411250860823));
#38507=DIRECTION('ref_axis',(-0.707106781186545,0.233585577946048,0.667411250860827));
#38508=DIRECTION('',(1.,0.,0.));
#38509=DIRECTION('center_axis',(0.707106781186551,-0.233585577946046,-0.667411250860821));
#38510=DIRECTION('ref_axis',(0.707106781186544,0.233585577946049,0.667411250860829));
#38511=DIRECTION('center_axis',(1.,0.,0.));
#38512=DIRECTION('ref_axis',(0.,1.,0.));
#38513=DIRECTION('center_axis',(0.707106781186547,0.361120764691833,0.607940616597037));
#38514=DIRECTION('ref_axis',(-0.707106781186548,0.361120764691833,0.607940616597037));
#38515=DIRECTION('',(-1.,0.,0.));
#38516=DIRECTION('center_axis',(-0.707106781186547,0.306761075170857,0.637100967476914));
#38517=DIRECTION('ref_axis',(0.707106781186548,0.306761075170857,0.637100967476913));
#38518=DIRECTION('center_axis',(-1.,0.,0.));
#38519=DIRECTION('ref_axis',(0.,1.,0.));
#38520=DIRECTION('center_axis',(-0.707106781186545,-0.17452799101363,-0.685229874095365));
#38521=DIRECTION('ref_axis',(-0.707106781186551,0.174527991013629,0.68522987409536));
#38522=DIRECTION('',(1.,0.,0.));
#38523=DIRECTION('center_axis',(0.707106781186546,-0.17452799101363,-0.685229874095364));
#38524=DIRECTION('ref_axis',(0.707106781186549,0.174527991013629,0.685229874095361));
#38525=DIRECTION('center_axis',(1.,0.,0.));
#38526=DIRECTION('ref_axis',(0.,1.,0.));
#38527=DIRECTION('center_axis',(0.707106781186549,0.306761075170857,0.637100967476913));
#38528=DIRECTION('ref_axis',(-0.707106781186546,0.306761075170858,0.637100967476915));
#38529=DIRECTION('',(-1.,0.,0.));
#38530=DIRECTION('center_axis',(-0.707106781186547,0.250066748640429,0.661412595302211));
#38531=DIRECTION('ref_axis',(0.707106781186548,0.250066748640428,0.661412595302209));
#38532=DIRECTION('center_axis',(-1.,0.,0.));
#38533=DIRECTION('ref_axis',(0.,1.,0.));
#38534=DIRECTION('center_axis',(-0.70710678118655,-0.114142140686715,-0.697833484234922));
#38535=DIRECTION('ref_axis',(-0.707106781186545,0.114142140686716,0.697833484234926));
#38536=DIRECTION('',(1.,0.,0.));
#38537=DIRECTION('center_axis',(0.707106781186545,-0.114142140686716,-0.697833484234927));
#38538=DIRECTION('ref_axis',(0.70710678118655,0.114142140686715,0.697833484234922));
#38539=DIRECTION('center_axis',(1.,0.,0.));
#38540=DIRECTION('ref_axis',(0.,1.,0.));
#38541=DIRECTION('center_axis',(0.707106781186545,0.25006674864043,0.661412595302212));
#38542=DIRECTION('ref_axis',(-0.70710678118655,0.250066748640428,0.661412595302208));
#38543=DIRECTION('',(-1.,0.,0.));
#38544=DIRECTION('center_axis',(-0.707106781186541,0.191469263158418,0.680690473905417));
#38545=DIRECTION('ref_axis',(0.707106781186554,0.191469263158414,0.680690473905405));
#38546=DIRECTION('center_axis',(-1.,0.,0.));
#38547=DIRECTION('ref_axis',(0.,1.,0.));
#38548=DIRECTION('center_axis',(-0.707106781186545,-0.0528875997482674,
-0.705126160196082));
#38549=DIRECTION('ref_axis',(-0.70710678118655,0.052887599748267,0.705126160196077));
#38550=DIRECTION('',(1.,0.,0.));
#38551=DIRECTION('center_axis',(0.707106781186546,-0.0528875997482673,-0.705126160196081));
#38552=DIRECTION('ref_axis',(0.707106781186549,0.0528875997482671,0.705126160196078));
#38553=DIRECTION('center_axis',(1.,0.,0.));
#38554=DIRECTION('ref_axis',(0.,1.,0.));
#38555=DIRECTION('center_axis',(0.707106781186546,0.191469263158417,0.680690473905413));
#38556=DIRECTION('ref_axis',(-0.707106781186549,0.191469263158416,0.68069047390541));
#38557=DIRECTION('',(-1.,0.,0.));
#38558=DIRECTION('center_axis',(-0.707106781186545,0.131414580971466,0.694787886990049));
#38559=DIRECTION('ref_axis',(0.70710678118655,0.131414580971465,0.694787886990044));
#38560=DIRECTION('center_axis',(-1.,0.,0.));
#38561=DIRECTION('ref_axis',(0.,1.,0.));
#38562=DIRECTION('center_axis',(-0.707106781186548,0.00876944775867127,
-0.707052400311326));
#38563=DIRECTION('ref_axis',(0.707106781186547,0.00876944775867126,-0.707052400311326));
#38564=DIRECTION('',(1.,0.,0.));
#38565=DIRECTION('center_axis',(0.707106781186549,0.00876944775867125,-0.707052400311324));
#38566=DIRECTION('ref_axis',(-0.707106781186546,0.00876944775867128,-0.707052400311328));
#38567=DIRECTION('center_axis',(1.,0.,0.));
#38568=DIRECTION('ref_axis',(0.,1.,0.));
#38569=DIRECTION('center_axis',(0.707106781186546,0.131414580971466,0.694787886990048));
#38570=DIRECTION('ref_axis',(-0.707106781186549,0.131414580971466,0.694787886990046));
#38571=DIRECTION('',(-1.,0.,0.));
#38572=DIRECTION('center_axis',(-0.707106781186548,0.0703597544730292,0.703597544730292));
#38573=DIRECTION('ref_axis',(0.707106781186547,0.0703597544730293,0.703597544730292));
#38574=DIRECTION('center_axis',(-1.,0.,0.));
#38575=DIRECTION('ref_axis',(0.,1.,0.));
#38576=DIRECTION('center_axis',(-0.707106781186547,0.070359754473029,-0.703597544730292));
#38577=DIRECTION('ref_axis',(0.707106781186548,0.0703597544730289,-0.703597544730292));
#38578=DIRECTION('',(1.,0.,0.));
#38579=DIRECTION('center_axis',(0.707106781186549,0.0703597544730288,-0.70359754473029));
#38580=DIRECTION('ref_axis',(-0.707106781186546,0.0703597544730291,-0.703597544730294));
#38581=DIRECTION('center_axis',(1.,0.,0.));
#38582=DIRECTION('ref_axis',(0.,1.,0.));
#38583=DIRECTION('center_axis',(0.707106781186548,0.0703597544730291,0.703597544730291));
#38584=DIRECTION('ref_axis',(-0.707106781186547,0.0703597544730294,0.703597544730293));
#38585=DIRECTION('',(-1.,0.,0.));
#38586=DIRECTION('center_axis',(-0.707106781186548,0.00876944775867152,
0.707052400311326));
#38587=DIRECTION('ref_axis',(0.707106781186547,0.00876944775867157,0.707052400311326));
#38588=DIRECTION('center_axis',(-1.,0.,0.));
#38589=DIRECTION('ref_axis',(0.,1.,0.));
#38590=DIRECTION('center_axis',(-0.707106781186548,0.131414580971466,-0.694787886990046));
#38591=DIRECTION('ref_axis',(0.707106781186547,0.131414580971466,-0.694787886990047));
#38592=DIRECTION('',(1.,0.,0.));
#38593=DIRECTION('center_axis',(0.707106781186548,0.131414580971466,-0.694787886990046));
#38594=DIRECTION('ref_axis',(-0.707106781186547,0.131414580971466,-0.694787886990047));
#38595=DIRECTION('center_axis',(1.,0.,0.));
#38596=DIRECTION('ref_axis',(0.,1.,0.));
#38597=DIRECTION('center_axis',(0.707106781186549,0.0087694477586715,0.707052400311324));
#38598=DIRECTION('ref_axis',(-0.707106781186546,0.00876944775867159,0.707052400311328));
#38599=DIRECTION('',(-1.,0.,0.));
#38600=DIRECTION('center_axis',(-0.707106781186545,-0.0528875997482672,
0.705126160196082));
#38601=DIRECTION('ref_axis',(-0.70710678118655,0.0528875997482668,-0.705126160196077));
#38602=DIRECTION('center_axis',(-1.,0.,0.));
#38603=DIRECTION('ref_axis',(0.,1.,0.));
#38604=DIRECTION('center_axis',(-0.707106781186544,0.191469263158417,-0.680690473905414));
#38605=DIRECTION('ref_axis',(0.707106781186551,0.191469263158415,-0.680690473905408));
#38606=DIRECTION('',(1.,0.,0.));
#38607=DIRECTION('center_axis',(0.707106781186546,0.191469263158416,-0.680690473905413));
#38608=DIRECTION('ref_axis',(-0.707106781186549,0.191469263158415,-0.68069047390541));
#38609=DIRECTION('center_axis',(1.,0.,0.));
#38610=DIRECTION('ref_axis',(0.,1.,0.));
#38611=DIRECTION('center_axis',(0.707106781186549,-0.0528875997482668,0.705126160196077));
#38612=DIRECTION('ref_axis',(0.707106781186546,0.0528875997482672,-0.705126160196081));
#38613=DIRECTION('',(-1.,0.,0.));
#38614=DIRECTION('center_axis',(-0.70710678118655,-0.114142140686715,0.697833484234922));
#38615=DIRECTION('ref_axis',(-0.707106781186545,0.114142140686716,-0.697833484234926));
#38616=DIRECTION('center_axis',(-1.,0.,0.));
#38617=DIRECTION('ref_axis',(0.,1.,0.));
#38618=DIRECTION('center_axis',(-0.707106781186544,0.25006674864043,-0.661412595302213));
#38619=DIRECTION('ref_axis',(0.707106781186551,0.250066748640427,-0.661412595302206));
#38620=DIRECTION('',(1.,0.,0.));
#38621=DIRECTION('center_axis',(0.707106781186545,0.250066748640429,-0.661412595302212));
#38622=DIRECTION('ref_axis',(-0.70710678118655,0.250066748640428,-0.661412595302208));
#38623=DIRECTION('center_axis',(1.,0.,0.));
#38624=DIRECTION('ref_axis',(0.,1.,0.));
#38625=DIRECTION('center_axis',(0.707106781186551,-0.114142140686715,0.697833484234921));
#38626=DIRECTION('ref_axis',(0.707106781186544,0.114142140686716,-0.697833484234928));
#38627=DIRECTION('',(-1.,0.,0.));
#38628=DIRECTION('center_axis',(-0.707106781186545,-0.17452799101363,0.685229874095366));
#38629=DIRECTION('ref_axis',(-0.70710678118655,0.174527991013628,-0.68522987409536));
#38630=DIRECTION('center_axis',(-1.,0.,0.));
#38631=DIRECTION('ref_axis',(0.,1.,0.));
#38632=DIRECTION('center_axis',(-0.707106781186547,0.306761075170857,-0.637100967476915));
#38633=DIRECTION('ref_axis',(0.707106781186548,0.306761075170856,-0.637100967476914));
#38634=DIRECTION('',(1.,0.,0.));
#38635=DIRECTION('center_axis',(0.707106781186549,0.306761075170856,-0.637100967476913));
#38636=DIRECTION('ref_axis',(-0.707106781186546,0.306761075170857,-0.637100967476915));
#38637=DIRECTION('center_axis',(1.,0.,0.));
#38638=DIRECTION('ref_axis',(0.,1.,0.));
#38639=DIRECTION('center_axis',(0.70710678118654,-0.174527991013631,0.68522987409537));
#38640=DIRECTION('ref_axis',(0.707106781186555,0.174527991013627,-0.685229874095356));
#38641=DIRECTION('',(-1.,0.,0.));
#38642=DIRECTION('center_axis',(-0.70710678118655,-0.233585577946046,0.667411250860823));
#38643=DIRECTION('ref_axis',(-0.707106781186545,0.233585577946047,-0.667411250860828));
#38644=DIRECTION('center_axis',(-1.,0.,0.));
#38645=DIRECTION('ref_axis',(0.,1.,0.));
#38646=DIRECTION('center_axis',(-0.70710678118654,0.361120764691836,-0.607940616597043));
#38647=DIRECTION('ref_axis',(0.707106781186555,0.361120764691829,-0.607940616597031));
#38648=DIRECTION('',(1.,0.,0.));
#38649=DIRECTION('center_axis',(0.707106781186542,0.361120764691835,-0.607940616597042));
#38650=DIRECTION('ref_axis',(-0.707106781186553,0.36112076469183,-0.607940616597033));
#38651=DIRECTION('center_axis',(1.,0.,0.));
#38652=DIRECTION('ref_axis',(0.,1.,0.));
#38653=DIRECTION('center_axis',(0.707106781186551,-0.233585577946045,0.667411250860822));
#38654=DIRECTION('ref_axis',(0.707106781186544,0.233585577946048,-0.667411250860829));
#38655=DIRECTION('',(-1.,0.,0.));
#38656=DIRECTION('center_axis',(-0.707106781186555,-0.290865437587464,0.644513225013298));
#38657=DIRECTION('ref_axis',(-0.70710678118654,0.29086543758747,-0.644513225013312));
#38658=DIRECTION('center_axis',(-1.,0.,0.));
#38659=DIRECTION('ref_axis',(0.,1.,0.));
#38660=DIRECTION('center_axis',(-0.707106781186546,0.412732107142826,-0.574153470540278));
#38661=DIRECTION('ref_axis',(0.707106781186549,0.412732107142824,-0.574153470540275));
#38662=DIRECTION('',(1.,0.,0.));
#38663=DIRECTION('center_axis',(0.707106781186547,0.412732107142825,-0.574153470540276));
#38664=DIRECTION('ref_axis',(-0.707106781186548,0.412732107142825,-0.574153470540276));
#38665=DIRECTION('center_axis',(1.,0.,0.));
#38666=DIRECTION('ref_axis',(0.,1.,0.));
#38667=DIRECTION('center_axis',(0.707106781186557,-0.290865437587463,0.644513225013297));
#38668=DIRECTION('ref_axis',(0.707106781186538,0.290865437587471,-0.644513225013314));
#38669=DIRECTION('',(-1.,0.,0.));
#38670=DIRECTION('center_axis',(-0.707106781186539,-0.345931635619497,0.616710064355716));
#38671=DIRECTION('ref_axis',(-0.707106781186556,0.345931635619489,-0.616710064355701));
#38672=DIRECTION('center_axis',(-1.,0.,0.));
#38673=DIRECTION('ref_axis',(0.,1.,0.));
#38674=DIRECTION('center_axis',(-0.707106781186546,0.461202309044001,-0.535996669889361));
#38675=DIRECTION('ref_axis',(0.707106781186549,0.461202309043999,-0.535996669889358));
#38676=DIRECTION('',(1.,0.,0.));
#38677=DIRECTION('center_axis',(0.707106781186547,0.461202309044,-0.53599666988936));
#38678=DIRECTION('ref_axis',(-0.707106781186548,0.461202309044,-0.535996669889359));
#38679=DIRECTION('center_axis',(1.,0.,0.));
#38680=DIRECTION('ref_axis',(0.,1.,0.));
#38681=DIRECTION('center_axis',(0.707106781186546,-0.345931635619494,0.61671006435571));
#38682=DIRECTION('ref_axis',(0.707106781186549,0.345931635619493,-0.616710064355707));
#38683=DIRECTION('',(-1.,0.,0.));
#38684=DIRECTION('center_axis',(-0.70710678118654,-0.398365085025227,0.584213367728653));
#38685=DIRECTION('ref_axis',(-0.707106781186555,0.398365085025218,-0.584213367728641));
#38686=DIRECTION('center_axis',(-1.,0.,0.));
#38687=DIRECTION('ref_axis',(0.,1.,0.));
#38688=DIRECTION('center_axis',(-0.707106781186549,0.506162482891781,-0.493760610936946));
#38689=DIRECTION('ref_axis',(0.707106781186546,0.506162482891783,-0.493760610936948));
#38690=DIRECTION('',(1.,0.,0.));
#38691=DIRECTION('center_axis',(0.707106781186551,0.50616248289178,-0.493760610936944));
#38692=DIRECTION('ref_axis',(-0.707106781186544,0.506162482891784,-0.493760610936949));
#38693=DIRECTION('center_axis',(1.,0.,0.));
#38694=DIRECTION('ref_axis',(0.,1.,0.));
#38695=DIRECTION('center_axis',(0.707106781186542,-0.398365085025226,0.584213367728652));
#38696=DIRECTION('ref_axis',(0.707106781186554,0.398365085025219,-0.584213367728642));
#38697=DIRECTION('',(-1.,0.,0.));
#38698=DIRECTION('center_axis',(-0.70710678118655,-0.447766735594494,0.547270454615492));
#38699=DIRECTION('ref_axis',(-0.707106781186545,0.447766735594496,-0.547270454615496));
#38700=DIRECTION('center_axis',(-1.,0.,0.));
#38701=DIRECTION('ref_axis',(0.,1.,0.));
#38702=DIRECTION('center_axis',(-0.70710678118655,0.547270454615492,-0.447766735594494));
#38703=DIRECTION('ref_axis',(0.707106781186545,0.547270454615496,-0.447766735594497));
#38704=DIRECTION('',(1.,0.,0.));
#38705=DIRECTION('center_axis',(0.707106781186551,0.547270454615491,-0.447766735594493));
#38706=DIRECTION('ref_axis',(-0.707106781186544,0.547270454615497,-0.447766735594498));
#38707=DIRECTION('center_axis',(1.,0.,0.));
#38708=DIRECTION('ref_axis',(0.,1.,0.));
#38709=DIRECTION('center_axis',(0.707106781186551,-0.447766735594493,0.547270454615491));
#38710=DIRECTION('ref_axis',(0.707106781186544,0.447766735594498,-0.547270454615497));
#38711=DIRECTION('',(-1.,0.,0.));
#38712=DIRECTION('center_axis',(-0.707106781186558,-0.493760610936939,0.506162482891775));
#38713=DIRECTION('ref_axis',(-0.707106781186537,0.493760610936954,-0.50616248289179));
#38714=DIRECTION('center_axis',(-1.,0.,0.));
#38715=DIRECTION('ref_axis',(0.,1.,0.));
#38716=DIRECTION('center_axis',(-0.707106781186557,0.584213367728639,-0.398365085025217));
#38717=DIRECTION('ref_axis',(0.707106781186538,0.584213367728655,-0.398365085025228));
#38718=DIRECTION('',(1.,0.,0.));
#38719=DIRECTION('center_axis',(0.707106781186542,0.584213367728652,-0.398365085025226));
#38720=DIRECTION('ref_axis',(-0.707106781186553,0.584213367728642,-0.39836508502522));
#38721=DIRECTION('center_axis',(1.,0.,0.));
#38722=DIRECTION('ref_axis',(0.,1.,0.));
#38723=DIRECTION('center_axis',(0.70710678118656,-0.493760610936938,0.506162482891773));
#38724=DIRECTION('ref_axis',(0.707106781186535,0.493760610936955,-0.506162482891791));
#38725=DIRECTION('',(-1.,0.,0.));
#38726=DIRECTION('center_axis',(-0.707106781186541,-0.535996669889364,0.461202309044004));
#38727=DIRECTION('ref_axis',(-0.707106781186554,0.535996669889354,-0.461202309043996));
#38728=DIRECTION('center_axis',(-1.,0.,0.));
#38729=DIRECTION('ref_axis',(0.,1.,0.));
#38730=DIRECTION('center_axis',(-0.70710678118655,0.616710064355706,-0.345931635619492));
#38731=DIRECTION('ref_axis',(0.707106781186545,0.616710064355711,-0.345931635619495));
#38732=DIRECTION('',(1.,0.,0.));
#38733=DIRECTION('center_axis',(0.707106781186552,0.616710064355705,-0.345931635619491));
#38734=DIRECTION('ref_axis',(-0.707106781186543,0.616710064355712,-0.345931635619496));
#38735=DIRECTION('center_axis',(1.,0.,0.));
#38736=DIRECTION('ref_axis',(0.,1.,0.));
#38737=DIRECTION('center_axis',(0.707106781186552,-0.535996669889356,0.461202309043997));
#38738=DIRECTION('ref_axis',(0.707106781186543,0.535996669889363,-0.461202309044003));
#38739=DIRECTION('',(-1.,0.,0.));
#38740=DIRECTION('center_axis',(-0.707106781186536,-0.574153470540286,0.412732107142832));
#38741=DIRECTION('ref_axis',(-0.707106781186559,0.574153470540266,-0.412732107142818));
#38742=DIRECTION('center_axis',(-1.,0.,0.));
#38743=DIRECTION('ref_axis',(0.,1.,0.));
#38744=DIRECTION('center_axis',(-0.707106781186549,0.644513225013303,-0.290865437587467));
#38745=DIRECTION('ref_axis',(0.707106781186546,0.644513225013307,-0.290865437587468));
#38746=DIRECTION('',(1.,0.,0.));
#38747=DIRECTION('center_axis',(0.707106781186551,0.644513225013302,-0.290865437587466));
#38748=DIRECTION('ref_axis',(-0.707106781186544,0.644513225013308,-0.290865437587469));
#38749=DIRECTION('center_axis',(1.,0.,0.));
#38750=DIRECTION('ref_axis',(0.,1.,0.));
#38751=DIRECTION('center_axis',(0.707106781186547,-0.574153470540276,0.412732107142825));
#38752=DIRECTION('ref_axis',(0.707106781186548,0.574153470540276,-0.412732107142825));
#38753=DIRECTION('',(-1.,0.,0.));
#38754=DIRECTION('center_axis',(-0.707106781186546,-0.607940616597038,0.361120764691834));
#38755=DIRECTION('ref_axis',(-0.707106781186549,0.607940616597036,-0.361120764691833));
#38756=DIRECTION('center_axis',(-1.,0.,0.));
#38757=DIRECTION('ref_axis',(0.,1.,0.));
#38758=DIRECTION('center_axis',(-0.70710678118655,0.667411250860823,-0.233585577946047));
#38759=DIRECTION('ref_axis',(0.707106781186545,0.667411250860827,-0.233585577946048));
#38760=DIRECTION('',(1.,0.,0.));
#38761=DIRECTION('center_axis',(0.707106781186551,0.667411250860821,-0.233585577946046));
#38762=DIRECTION('ref_axis',(-0.707106781186544,0.667411250860829,-0.233585577946049));
#38763=DIRECTION('center_axis',(1.,0.,0.));
#38764=DIRECTION('ref_axis',(0.,1.,0.));
#38765=DIRECTION('center_axis',(0.707106781186547,-0.607940616597037,0.361120764691833));
#38766=DIRECTION('ref_axis',(0.707106781186548,0.607940616597037,-0.361120764691833));
#38767=DIRECTION('',(-1.,0.,0.));
#38768=DIRECTION('center_axis',(-0.707106781186541,-0.637100967476919,0.30676107517086));
#38769=DIRECTION('ref_axis',(-0.707106781186554,0.637100967476908,-0.306761075170855));
#38770=DIRECTION('center_axis',(-1.,0.,0.));
#38771=DIRECTION('ref_axis',(0.,1.,0.));
#38772=DIRECTION('center_axis',(-0.707106781186539,0.685229874095371,-0.174527991013632));
#38773=DIRECTION('ref_axis',(0.707106781186556,0.685229874095354,-0.174527991013628));
#38774=DIRECTION('',(1.,0.,0.));
#38775=DIRECTION('center_axis',(0.707106781186549,0.685229874095361,-0.174527991013629));
#38776=DIRECTION('ref_axis',(-0.707106781186546,0.685229874095364,-0.17452799101363));
#38777=DIRECTION('center_axis',(1.,0.,0.));
#38778=DIRECTION('ref_axis',(0.,1.,0.));
#38779=DIRECTION('center_axis',(0.707106781186543,-0.637100967476918,0.306761075170859));
#38780=DIRECTION('ref_axis',(0.707106781186552,0.63710096747691,-0.306761075170855));
#38781=DIRECTION('',(-1.,0.,0.));
#38782=DIRECTION('center_axis',(-0.707106781186544,-0.661412595302213,0.25006674864043));
#38783=DIRECTION('ref_axis',(-0.707106781186551,0.661412595302206,-0.250066748640427));
#38784=DIRECTION('center_axis',(-1.,0.,0.));
#38785=DIRECTION('ref_axis',(0.,1.,0.));
#38786=DIRECTION('center_axis',(-0.707106781186546,0.697833484234925,-0.114142140686716));
#38787=DIRECTION('ref_axis',(0.707106781186548,0.697833484234923,-0.114142140686715));
#38788=DIRECTION('',(1.,0.,0.));
#38789=DIRECTION('center_axis',(0.707106781186548,0.697833484234924,-0.114142140686716));
#38790=DIRECTION('ref_axis',(-0.707106781186547,0.697833484234925,-0.114142140686716));
#38791=DIRECTION('center_axis',(1.,0.,0.));
#38792=DIRECTION('ref_axis',(0.,1.,0.));
#38793=DIRECTION('center_axis',(0.707106781186545,-0.661412595302212,0.25006674864043));
#38794=DIRECTION('ref_axis',(0.70710678118655,0.661412595302208,-0.250066748640428));
#38795=DIRECTION('',(-1.,0.,0.));
#38796=DIRECTION('center_axis',(-0.707106781186541,-0.680690473905417,0.191469263158418));
#38797=DIRECTION('ref_axis',(-0.707106781186554,0.680690473905405,-0.191469263158414));
#38798=DIRECTION('center_axis',(-1.,0.,0.));
#38799=DIRECTION('ref_axis',(0.,1.,0.));
#38800=DIRECTION('center_axis',(-0.707106781186545,0.705126160196082,-0.0528875997482675));
#38801=DIRECTION('ref_axis',(0.70710678118655,0.705126160196077,-0.0528875997482671));
#38802=DIRECTION('',(1.,0.,0.));
#38803=DIRECTION('center_axis',(0.707106781186546,0.705126160196081,-0.0528875997482674));
#38804=DIRECTION('ref_axis',(-0.707106781186549,0.705126160196078,-0.0528875997482672));
#38805=DIRECTION('center_axis',(1.,0.,0.));
#38806=DIRECTION('ref_axis',(0.,1.,0.));
#38807=DIRECTION('center_axis',(0.707106781186546,-0.680690473905413,0.191469263158417));
#38808=DIRECTION('ref_axis',(0.707106781186549,0.680690473905409,-0.191469263158416));
#38809=DIRECTION('',(-1.,0.,0.));
#38810=DIRECTION('center_axis',(-0.707106781186545,-0.694787886990049,0.131414580971466));
#38811=DIRECTION('ref_axis',(-0.70710678118655,0.694787886990044,-0.131414580971465));
#38812=DIRECTION('center_axis',(-1.,0.,0.));
#38813=DIRECTION('ref_axis',(0.,1.,0.));
#38814=DIRECTION('center_axis',(-0.707106781186548,0.707052400311326,0.00876944775867122));
#38815=DIRECTION('ref_axis',(0.707106781186547,0.707052400311326,0.00876944775867122));
#38816=DIRECTION('',(1.,0.,0.));
#38817=DIRECTION('center_axis',(0.707106781186549,0.707052400311324,0.00876944775867119));
#38818=DIRECTION('ref_axis',(-0.707106781186546,0.707052400311328,0.00876944775867124));
#38819=DIRECTION('center_axis',(1.,0.,0.));
#38820=DIRECTION('ref_axis',(0.,1.,0.));
#38821=DIRECTION('center_axis',(0.707106781186546,-0.694787886990048,0.131414580971466));
#38822=DIRECTION('ref_axis',(0.707106781186549,0.694787886990046,-0.131414580971466));
#38823=DIRECTION('center_axis',(-1.,0.,0.));
#38824=DIRECTION('ref_axis',(0.,0.,-1.));
#38825=DIRECTION('center_axis',(-1.,0.,0.));
#38826=DIRECTION('ref_axis',(0.,0.,-1.));
#38827=DIRECTION('center_axis',(1.,0.,0.));
#38828=DIRECTION('ref_axis',(0.,0.,-1.));
#38829=DIRECTION('center_axis',(-1.,0.,0.));
#38830=DIRECTION('ref_axis',(0.,-0.951056516295153,0.309016994374948));
#38831=DIRECTION('center_axis',(-1.,0.,0.));
#38832=DIRECTION('ref_axis',(0.,0.,1.));
#38833=DIRECTION('center_axis',(1.,0.,0.));
#38834=DIRECTION('ref_axis',(0.,0.,1.));
#38835=DIRECTION('center_axis',(-1.,0.,0.));
#38836=DIRECTION('ref_axis',(0.,0.,1.));
#38837=DIRECTION('center_axis',(-1.,0.,0.));
#38838=DIRECTION('ref_axis',(0.,0.,1.));
#38839=DIRECTION('center_axis',(1.,0.,0.));
#38840=DIRECTION('ref_axis',(0.,0.,1.));
#38841=DIRECTION('center_axis',(-1.,0.,0.));
#38842=DIRECTION('ref_axis',(0.,0.,1.));
#38843=DIRECTION('center_axis',(-1.,0.,0.));
#38844=DIRECTION('ref_axis',(0.,0.,1.));
#38845=DIRECTION('center_axis',(1.,0.,0.));
#38846=DIRECTION('ref_axis',(0.,0.,1.));
#38847=DIRECTION('center_axis',(-1.,0.,0.));
#38848=DIRECTION('ref_axis',(0.,0.,1.));
#38849=DIRECTION('center_axis',(-1.,0.,0.));
#38850=DIRECTION('ref_axis',(0.,0.,1.));
#38851=DIRECTION('center_axis',(1.,0.,0.));
#38852=DIRECTION('ref_axis',(0.,0.,1.));
#38853=DIRECTION('center_axis',(-1.,0.,0.));
#38854=DIRECTION('ref_axis',(0.,0.951056516295154,0.309016994374947));
#38855=DIRECTION('center_axis',(-1.,0.,0.));
#38856=DIRECTION('ref_axis',(0.,0.,1.));
#38857=DIRECTION('center_axis',(1.,0.,0.));
#38858=DIRECTION('ref_axis',(0.,0.,1.));
#38859=DIRECTION('center_axis',(-1.,0.,0.));
#38860=DIRECTION('ref_axis',(0.,0.,-1.));
#38861=DIRECTION('center_axis',(1.,0.,0.));
#38862=DIRECTION('ref_axis',(0.,0.,-1.));
#38863=DIRECTION('center_axis',(-1.,0.,0.));
#38864=DIRECTION('ref_axis',(0.,0.,-1.));
#38865=DIRECTION('center_axis',(-1.,0.,0.));
#38866=DIRECTION('ref_axis',(0.,0.,-1.));
#38867=DIRECTION('center_axis',(1.,0.,0.));
#38868=DIRECTION('ref_axis',(0.,0.,-1.));
#38869=DIRECTION('center_axis',(-1.,0.,0.));
#38870=DIRECTION('ref_axis',(0.,0.,-1.));
#38871=DIRECTION('center_axis',(-1.,0.,0.));
#38872=DIRECTION('ref_axis',(0.,0.,-1.));
#38873=DIRECTION('center_axis',(1.,0.,0.));
#38874=DIRECTION('ref_axis',(0.,0.,-1.));
#38875=DIRECTION('center_axis',(-1.,0.,0.));
#38876=DIRECTION('ref_axis',(0.,0.,-1.));
#38877=DIRECTION('center_axis',(-1.,0.,0.));
#38878=DIRECTION('ref_axis',(0.,0.,-1.));
#38879=DIRECTION('center_axis',(1.,0.,0.));
#38880=DIRECTION('ref_axis',(0.,0.,-1.));
#38881=DIRECTION('center_axis',(-1.,0.,0.));
#38882=DIRECTION('ref_axis',(0.,0.,-1.));
#38883=DIRECTION('center_axis',(1.,0.,0.));
#38884=DIRECTION('ref_axis',(0.,0.951056516295154,0.309016994374947));
#38885=DIRECTION('',(1.,0.,0.));
#38886=DIRECTION('center_axis',(-1.,0.,0.));
#38887=DIRECTION('ref_axis',(0.,0.,-1.));
#38888=DIRECTION('',(1.,0.,0.));
#38889=DIRECTION('center_axis',(1.,0.,0.));
#38890=DIRECTION('ref_axis',(0.,0.,-1.));
#38891=DIRECTION('',(1.,0.,0.));
#38892=DIRECTION('center_axis',(-1.,0.,0.));
#38893=DIRECTION('ref_axis',(0.,0.,-1.));
#38894=DIRECTION('center_axis',(1.,0.,0.));
#38895=DIRECTION('ref_axis',(0.,0.,-1.));
#38896=DIRECTION('',(1.,0.,0.));
#38897=DIRECTION('center_axis',(-1.,0.,0.));
#38898=DIRECTION('ref_axis',(0.,0.,-1.));
#38899=DIRECTION('center_axis',(1.,0.,0.));
#38900=DIRECTION('ref_axis',(0.,0.,-1.));
#38901=DIRECTION('',(1.,0.,0.));
#38902=DIRECTION('center_axis',(-1.,0.,0.));
#38903=DIRECTION('ref_axis',(0.,0.,-1.));
#38904=DIRECTION('center_axis',(1.,0.,0.));
#38905=DIRECTION('ref_axis',(0.,0.,-1.));
#38906=DIRECTION('',(1.,0.,0.));
#38907=DIRECTION('center_axis',(-1.,0.,0.));
#38908=DIRECTION('ref_axis',(0.,0.,-1.));
#38909=DIRECTION('center_axis',(1.,0.,0.));
#38910=DIRECTION('ref_axis',(0.,0.,-1.));
#38911=DIRECTION('',(1.,0.,0.));
#38912=DIRECTION('center_axis',(-1.,0.,0.));
#38913=DIRECTION('ref_axis',(0.,0.,-1.));
#38914=DIRECTION('center_axis',(1.,0.,0.));
#38915=DIRECTION('ref_axis',(0.,0.,-1.));
#38916=DIRECTION('center_axis',(-1.,0.,0.));
#38917=DIRECTION('ref_axis',(0.,0.,-1.));
#38918=DIRECTION('center_axis',(-1.,0.,0.));
#38919=DIRECTION('ref_axis',(0.,0.,-1.));
#38920=DIRECTION('center_axis',(-1.,0.,0.));
#38921=DIRECTION('ref_axis',(0.,0.,-1.));
#38922=DIRECTION('center_axis',(-1.,0.,0.));
#38923=DIRECTION('ref_axis',(0.,0.,-1.));
#38924=DIRECTION('center_axis',(-1.,0.,0.));
#38925=DIRECTION('ref_axis',(0.,0.,-1.));
#38926=DIRECTION('center_axis',(0.707106781186548,0.703597544730291,0.070359754473029));
#38927=DIRECTION('ref_axis',(0.099014754297667,0.,-0.995085965347403));
#38928=DIRECTION('',(0.595596683047421,-0.539007590193132,-0.595596683047431));
#38929=DIRECTION('',(0.,0.0995037190209988,-0.995037190209989));
#38930=DIRECTION('',(0.,-0.0995037190209988,0.995037190209989));
#38931=DIRECTION('',(0.557191914001244,-0.615690134680804,0.557191914001238));
#38932=DIRECTION('center_axis',(1.,0.,0.));
#38933=DIRECTION('ref_axis',(0.,0.,-1.));
#38934=DIRECTION('',(0.,1.,0.));
#38935=DIRECTION('',(0.,0.0995037190209988,0.995037190209989));
#38936=DIRECTION('center_axis',(0.707106781186554,0.,0.707106781186541));
#38937=DIRECTION('ref_axis',(0.707106781186541,0.,-0.707106781186554));
#38938=DIRECTION('',(0.557191914001233,0.61569013468081,-0.557191914001243));
#38939=DIRECTION('',(0.,-1.,0.));
#38940=DIRECTION('',(0.705516335778299,-0.0670328270320415,-0.705516335778311));
#38941=DIRECTION('center_axis',(0.,0.671005320760942,0.741452533551882));
#38942=DIRECTION('ref_axis',(1.,0.,0.));
#38943=DIRECTION('',(-1.,0.,0.));
#38944=DIRECTION('',(0.,-0.741452533551882,0.671005320760942));
#38945=DIRECTION('',(1.,0.,0.));
#38946=DIRECTION('center_axis',(0.56100663158041,-0.555465791309817,0.613782790576081));
#38947=DIRECTION('ref_axis',(0.738128342492238,0.,-0.674660321947023));
#38948=DIRECTION('',(0.,0.74145253355187,0.671005320760956));
#38949=DIRECTION('',(-0.705516335778304,-0.708685007986273,0.00350134337820634));
#38950=DIRECTION('center_axis',(-0.561006631580427,0.555465791309797,0.613782790576083));
#38951=DIRECTION('ref_axis',(0.738128342492228,0.,0.674660321947034));
#38952=DIRECTION('',(0.705516335778308,0.708685007986269,0.00350134337825648));
#38953=DIRECTION('',(-0.705516335778288,0.067032827032046,-0.705516335778322));
#38954=DIRECTION('center_axis',(-0.707106781186547,0.703597544730292,0.0703597544730291));
#38955=DIRECTION('ref_axis',(0.0990147542976674,0.,0.995085965347403));
#38956=DIRECTION('',(0.,-0.0995037190209988,0.995037190209989));
#38957=DIRECTION('',(0.,0.0995037190209988,-0.995037190209989));
#38958=DIRECTION('center_axis',(-0.561006631580422,-0.555465791309811,0.613782790576075));
#38959=DIRECTION('ref_axis',(0.738128342492227,0.,0.674660321947036));
#38960=DIRECTION('',(0.705516335778288,0.0670328270320413,0.705516335778322));
#38961=DIRECTION('',(-0.705516335778306,0.708685007986271,-0.0035013433782314));
#38962=DIRECTION('',(0.,-0.74145253355187,-0.671005320760956));
#38963=DIRECTION('center_axis',(-0.707106781186548,-0.703597544730292,0.0703597544730291));
#38964=DIRECTION('ref_axis',(0.0990147542976672,0.,0.995085965347403));
#38965=DIRECTION('',(0.,0.0995037190209988,0.995037190209989));
#38966=DIRECTION('',(0.,-0.0995037190209988,-0.995037190209989));
#38967=DIRECTION('center_axis',(0.,-0.671005320760956,0.74145253355187));
#38968=DIRECTION('ref_axis',(1.,0.,0.));
#38969=DIRECTION('',(-1.,0.,0.));
#38970=DIRECTION('',(1.,0.,0.));
#38971=DIRECTION('center_axis',(-0.707106781186565,0.,0.70710678118653));
#38972=DIRECTION('ref_axis',(0.70710678118653,0.,0.707106781186565));
#38973=DIRECTION('',(0.,1.,0.));
#38974=DIRECTION('',(0.,-1.,0.));
#38975=DIRECTION('center_axis',(0.707106781186548,-0.703597544730291,0.070359754473029));
#38976=DIRECTION('ref_axis',(0.099014754297667,0.,-0.995085965347403));
#38977=DIRECTION('',(0.,-0.0995037190209988,-0.995037190209989));
#38978=DIRECTION('center_axis',(0.,0.995037190209989,0.0995037190209988));
#38979=DIRECTION('ref_axis',(0.,-0.0995037190209988,0.995037190209989));
#38980=DIRECTION('center_axis',(0.,0.,1.));
#38981=DIRECTION('ref_axis',(0.,-1.,0.));
#38982=DIRECTION('center_axis',(0.56100663158041,0.499857381275776,0.659859195364379));
#38983=DIRECTION('ref_axis',(0.761867344215962,0.,-0.647733085319344));
#38984=DIRECTION('',(0.705516335778303,-0.705683085390289,-0.0652539879547519));
#38985=DIRECTION('',(0.,0.797113049929627,-0.603830096659556));
#38986=DIRECTION('',(-0.705516335778303,-0.128267547152789,0.696989337291012));
#38987=DIRECTION('center_axis',(0.56100663158041,-0.60684677127256,0.56303512813933));
#38988=DIRECTION('ref_axis',(0.708381704532383,0.,-0.705829554980376));
#38989=DIRECTION('',(0.7055163357783,-0.00528794662205797,-0.708673928947921));
#38990=DIRECTION('',(0.,0.680149115692518,0.733073789207257));
#38991=DIRECTION('',(-0.705516335778302,-0.706293409755775,-0.0582779485356024));
#38992=DIRECTION('center_axis',(-0.561006631580394,0.499857381275784,0.659859195364387));
#38993=DIRECTION('ref_axis',(0.761867344215974,0.,0.64773308531933));
#38994=DIRECTION('',(0.,-0.797113049929627,0.603830096659556));
#38995=DIRECTION('',(0.705516335778304,0.70568308539029,0.0652539879547266));
#38996=DIRECTION('',(-0.705516335778317,0.128267547152785,-0.696989337290998));
#38997=DIRECTION('center_axis',(-0.707106781186548,0.694787886990046,0.131414580971466));
#38998=DIRECTION('ref_axis',(0.182719541232954,0.,0.983165077314903));
#38999=DIRECTION('',(0.,-0.185848282703424,0.982578452753869));
#39000=DIRECTION('',(0.,0.185848282703424,-0.982578452753869));
#39001=DIRECTION('center_axis',(-0.561006631580395,-0.606846771272568,0.563035128139337));
#39002=DIRECTION('ref_axis',(0.708381704532398,0.,0.705829554980361));
#39003=DIRECTION('',(0.705516335778314,0.00528794662205805,0.708673928947907));
#39004=DIRECTION('',(-0.705516335778303,0.706293409755772,0.0582779485356272));
#39005=DIRECTION('',(0.,-0.680149115692518,-0.733073789207257));
#39006=DIRECTION('center_axis',(-0.707106781186548,-0.707052400311326,0.00876944775867132));
#39007=DIRECTION('ref_axis',(0.0124009183210273,0.,0.999923105656027));
#39008=DIRECTION('',(0.,0.0124018719548353,0.999923093828728));
#39009=DIRECTION('',(0.,-0.0124018719548353,-0.999923093828728));
#39010=DIRECTION('center_axis',(0.,-0.733073789207257,0.680149115692518));
#39011=DIRECTION('ref_axis',(1.,0.,0.));
#39012=DIRECTION('',(-1.,0.,0.));
#39013=DIRECTION('',(1.,0.,0.));
#39014=DIRECTION('center_axis',(-0.707106781186531,-0.0616284167162208,
0.704416026402775));
#39015=DIRECTION('ref_axis',(0.705757556807969,0.,0.708453436019931));
#39016=DIRECTION('',(0.,0.996194698091746,0.0871557427476582));
#39017=DIRECTION('',(0.,-0.996194698091746,-0.0871557427476582));
#39018=DIRECTION('center_axis',(0.,0.603830096659556,0.797113049929627));
#39019=DIRECTION('ref_axis',(1.,0.,0.));
#39020=DIRECTION('',(-1.,0.,0.));
#39021=DIRECTION('',(1.,0.,0.));
#39022=DIRECTION('center_axis',(0.707106781186549,-0.707052400311325,0.00876944775867131));
#39023=DIRECTION('ref_axis',(0.0124009183210273,0.,-0.999923105656027));
#39024=DIRECTION('',(0.,0.0124018719548353,0.999923093828728));
#39025=DIRECTION('',(0.,-0.0124018719548353,-0.999923093828728));
#39026=DIRECTION('center_axis',(0.707106781186545,-0.0616284167162196,0.704416026402761));
#39027=DIRECTION('ref_axis',(0.705757556807954,0.,-0.708453436019945));
#39028=DIRECTION('',(0.,0.996194698091746,0.0871557427476582));
#39029=DIRECTION('',(0.,-0.996194698091746,-0.0871557427476582));
#39030=DIRECTION('center_axis',(0.707106781186549,0.694787886990045,0.131414580971465));
#39031=DIRECTION('ref_axis',(0.182719541232953,0.,-0.983165077314903));
#39032=DIRECTION('',(0.,-0.185848282703424,0.982578452753869));
#39033=DIRECTION('',(0.,0.185848282703424,-0.982578452753869));
#39034=DIRECTION('center_axis',(1.,0.,0.));
#39035=DIRECTION('ref_axis',(0.,0.0871557427476582,-0.996194698091746));
#39036=DIRECTION('center_axis',(0.,0.98257845275387,0.185848282703424));
#39037=DIRECTION('ref_axis',(0.,-0.185848282703424,0.982578452753869));
#39038=DIRECTION('center_axis',(0.,-0.0871557427476582,0.996194698091746));
#39039=DIRECTION('ref_axis',(0.,-0.996194698091746,-0.0871557427476582));
#39040=DIRECTION('center_axis',(0.5610066315804,-0.65360928088182,0.508002428407545));
#39041=DIRECTION('ref_axis',(0.671222048820197,0.,-0.741256339721703));
#39042=DIRECTION('',(0.70551633577831,0.0564971782546651,-0.706438085609211));
#39043=DIRECTION('',(0.,0.613669352377492,0.789563123475628));
#39044=DIRECTION('',(-0.705516335778305,-0.698526492205411,-0.11961371007187));
#39045=DIRECTION('center_axis',(0.,-0.789563123475628,0.613669352377492));
#39046=DIRECTION('ref_axis',(1.,0.,0.));
#39047=DIRECTION('',(0.557191914001251,-0.509581057609725,-0.655640386718952));
#39048=DIRECTION('',(1.,0.,0.));
#39049=DIRECTION('',(-1.,0.,0.));
#39050=DIRECTION('',(-0.557191914001243,-0.509581057609728,-0.655640386718956));
#39051=DIRECTION('center_axis',(0.70710678118655,-0.705126160196078,-0.0528875997482671));
#39052=DIRECTION('ref_axis',(-0.0745860273602096,0.,-0.997214582987344));
#39053=DIRECTION('',(0.,-0.0747943608453594,0.997198978933359));
#39054=DIRECTION('',(0.,0.0747943608453594,-0.997198978933359));
#39055=DIRECTION('center_axis',(0.561006631580396,0.440444754748108,0.700913673242075));
#39056=DIRECTION('ref_axis',(0.780718990354275,0.,-0.624882275392894));
#39057=DIRECTION('',(0.705516335778308,-0.697310488411385,-0.1265100102815));
#39058=DIRECTION('',(0.,0.846707054687385,-0.532059360920014));
#39059=DIRECTION('',(-0.705516335778308,-0.188526073789645,0.683157829093256));
#39060=DIRECTION('center_axis',(0.,0.532059360920014,0.846707054687385));
#39061=DIRECTION('ref_axis',(1.,0.,0.));
#39062=DIRECTION('',(0.557191914001251,-0.703091778563843,0.441813446929307));
#39063=DIRECTION('',(1.,0.,0.));
#39064=DIRECTION('',(-1.,0.,0.));
#39065=DIRECTION('',(-0.557191914001251,-0.703091778563842,0.441813446929307));
#39066=DIRECTION('center_axis',(0.707106781186543,-0.122787803968974,0.696364240320023));
#39067=DIRECTION('ref_axis',(0.701673843159868,0.,-0.712498293208665));
#39068=DIRECTION('',(0.,0.984807753012208,0.17364817766693));
#39069=DIRECTION('',(0.,-0.984807753012208,-0.17364817766693));
#39070=DIRECTION('center_axis',(0.707106781186543,0.680690473905416,0.191469263158417));
#39071=DIRECTION('ref_axis',(0.261366100937226,0.,-0.965239742903737));
#39072=DIRECTION('',(0.,-0.270778428736215,0.962641699975202));
#39073=DIRECTION('',(0.,0.270778428736215,-0.962641699975202));
#39074=DIRECTION('center_axis',(-0.707106781186545,-0.705126160196082,-0.0528875997482674));
#39075=DIRECTION('ref_axis',(-0.0745860273602106,0.,0.997214582987344));
#39076=DIRECTION('',(-0.595596683047423,0.634243132390279,-0.49295054534778));
#39077=DIRECTION('',(0.,0.0747943608453594,-0.997198978933359));
#39078=DIRECTION('',(0.,-0.0747943608453594,0.997198978933359));
#39079=DIRECTION('center_axis',(0.,-0.17364817766693,0.984807753012208));
#39080=DIRECTION('ref_axis',(0.,-0.984807753012208,-0.17364817766693));
#39081=DIRECTION('',(0.,0.984807753012208,0.17364817766693));
#39082=DIRECTION('center_axis',(-0.707106781186541,-0.122787803968974,0.696364240320025));
#39083=DIRECTION('ref_axis',(0.701673843159869,0.,0.712498293208664));
#39084=DIRECTION('',(0.595596683047431,0.42739457511896,0.680145916919143));
#39085=DIRECTION('',(0.,-0.984807753012208,-0.17364817766693));
#39086=DIRECTION('center_axis',(-0.707106781186538,0.68069047390542,0.191469263158419));
#39087=DIRECTION('ref_axis',(0.261366100937229,0.,0.965239742903736));
#39088=DIRECTION('',(0.,0.270778428736215,-0.962641699975202));
#39089=DIRECTION('',(0.,-0.270778428736215,0.962641699975202));
#39090=DIRECTION('center_axis',(0.,0.962641699975202,0.270778428736215));
#39091=DIRECTION('ref_axis',(0.,-0.270778428736215,0.962641699975202));
#39092=DIRECTION('center_axis',(0.,-0.997198978933359,-0.0747943608453594));
#39093=DIRECTION('ref_axis',(0.,0.0747943608453594,-0.997198978933359));
#39094=DIRECTION('center_axis',(0.561006631580395,0.37768007768897,0.736633774843153));
#39095=DIRECTION('ref_axis',(0.795555689966288,0.,-0.605880470193802));
#39096=DIRECTION('',(0.705516335778309,-0.683630937568086,-0.186803215041197));
#39097=DIRECTION('',(0.,0.889857107503286,-0.456239332177625));
#39098=DIRECTION('',(-0.705516335778301,-0.247349803169823,0.664127077314131));
#39099=DIRECTION('center_axis',(0.561006631580428,-0.695397429203483,0.449103523455304));
#39100=DIRECTION('ref_axis',(0.624948053917873,0.,-0.780666337114816));
#39101=DIRECTION('',(0.705516335778292,0.117852325490946,-0.698825821880065));
#39102=DIRECTION('',(0.,0.542519194747178,0.84004340562311));
#39103=DIRECTION('',(-0.705516335778305,-0.685443366267552,-0.18003913904971));
#39104=DIRECTION('center_axis',(-0.561006631580391,0.377680077688971,0.736633774843155));
#39105=DIRECTION('ref_axis',(0.795555689966291,0.,0.605880470193798));
#39106=DIRECTION('',(0.,-0.889857107503286,0.456239332177625));
#39107=DIRECTION('',(0.705516335778314,0.683630937568081,0.186803215041198));
#39108=DIRECTION('',(-0.705516335778302,0.247349803169829,-0.664127077314128));
#39109=DIRECTION('center_axis',(-0.707106781186541,0.661412595302216,0.250066748640431));
#39110=DIRECTION('ref_axis',(0.333412439312666,0.,0.942781069661232));
#39111=DIRECTION('',(0.,-0.353647787425838,0.935378662600772));
#39112=DIRECTION('',(0.,0.353647787425838,-0.935378662600772));
#39113=DIRECTION('center_axis',(-0.561006631580427,-0.695397429203484,0.449103523455304));
#39114=DIRECTION('ref_axis',(0.624948053917874,0.,0.780666337114815));
#39115=DIRECTION('',(0.705516335778294,-0.117852325490946,0.698825821880063));
#39116=DIRECTION('',(-0.705516335778306,0.68544336626755,0.180039139049709));
#39117=DIRECTION('',(0.,-0.542519194747178,-0.84004340562311));
#39118=DIRECTION('center_axis',(-0.70710678118655,-0.697833484234922,-0.114142140686715));
#39119=DIRECTION('ref_axis',(-0.159358523666363,0.,0.987220776186805));
#39120=DIRECTION('',(0.,-0.161421363397451,0.986885577683101));
#39121=DIRECTION('',(0.,0.161421363397451,-0.986885577683101));
#39122=DIRECTION('center_axis',(0.,-0.84004340562311,0.542519194747178));
#39123=DIRECTION('ref_axis',(1.,0.,0.));
#39124=DIRECTION('',(-1.,0.,0.));
#39125=DIRECTION('',(1.,0.,0.));
#39126=DIRECTION('center_axis',(-0.707106781186552,-0.183012701892218,0.683012701892215));
#39127=DIRECTION('ref_axis',(0.694746590606862,0.,0.719254596676408));
#39128=DIRECTION('',(0.,0.965925826289068,0.258819045102521));
#39129=DIRECTION('',(0.,-0.965925826289068,-0.258819045102521));
#39130=DIRECTION('center_axis',(0.,0.456239332177625,0.889857107503286));
#39131=DIRECTION('ref_axis',(1.,0.,0.));
#39132=DIRECTION('',(-1.,0.,0.));
#39133=DIRECTION('',(1.,0.,0.));
#39134=DIRECTION('center_axis',(0.707106781186551,-0.697833484234921,-0.114142140686715));
#39135=DIRECTION('ref_axis',(-0.159358523666362,0.,-0.987220776186805));
#39136=DIRECTION('',(0.,-0.161421363397451,0.986885577683101));
#39137=DIRECTION('',(0.,0.161421363397451,-0.986885577683101));
#39138=DIRECTION('center_axis',(0.707106781186553,-0.183012701892218,0.683012701892214));
#39139=DIRECTION('ref_axis',(0.69474659060686,0.,-0.719254596676409));
#39140=DIRECTION('',(0.,0.965925826289068,0.258819045102521));
#39141=DIRECTION('',(0.,-0.965925826289068,-0.258819045102521));
#39142=DIRECTION('center_axis',(0.707106781186545,0.661412595302212,0.25006674864043));
#39143=DIRECTION('ref_axis',(0.333412439312663,0.,-0.942781069661234));
#39144=DIRECTION('',(0.,-0.353647787425838,0.935378662600772));
#39145=DIRECTION('',(0.,0.353647787425838,-0.935378662600772));
#39146=DIRECTION('center_axis',(1.,0.,0.));
#39147=DIRECTION('ref_axis',(0.,0.258819045102521,-0.965925826289068));
#39148=DIRECTION('center_axis',(0.,0.935378662600772,0.353647787425838));
#39149=DIRECTION('ref_axis',(0.,-0.353647787425838,0.935378662600772));
#39150=DIRECTION('center_axis',(0.,-0.258819045102521,0.965925826289068));
#39151=DIRECTION('ref_axis',(0.,-0.965925826289068,-0.258819045102521));
#39152=DIRECTION('center_axis',(0.56100663158041,0.312041027189168,0.76674764862602));
#39153=DIRECTION('ref_axis',(0.807044487383574,0.,-0.590490639539514));
#39154=DIRECTION('',(0.70551633577831,-0.664748542502243,-0.245674734539575));
#39155=DIRECTION('',(0.,0.926234810420662,-0.376947046632547));
#39156=DIRECTION('',(-0.705516335778298,-0.304291051193938,0.640041917465765));
#39157=DIRECTION('center_axis',(0.561006631580392,-0.73189318319651,0.386786669513444));
#39158=DIRECTION('ref_axis',(0.567619122871716,0.,-0.823291279773048));
#39159=DIRECTION('',(0.705516335778307,0.178310545369053,-0.685895071683813));
#39160=DIRECTION('',(0.,0.467240138462762,0.884130450221741));
#39161=DIRECTION('',(-0.705516335778315,-0.667143602430337,-0.239094361468882));
#39162=DIRECTION('center_axis',(-0.561006631580397,0.312041027189172,0.766747648626028));
#39163=DIRECTION('ref_axis',(0.807044487383583,0.,0.590490639539502));
#39164=DIRECTION('',(0.,-0.926234810420662,0.376947046632547));
#39165=DIRECTION('',(0.705516335778304,0.66474854250226,0.245674734539547));
#39166=DIRECTION('',(-0.705516335778316,0.304291051193919,-0.640041917465754));
#39167=DIRECTION('center_axis',(-0.707106781186553,0.637100967476909,0.306761075170854));
#39168=DIRECTION('ref_axis',(0.397987666358438,0.,0.917390765937049));
#39169=DIRECTION('',(0.,-0.433825672914778,0.900996828806872));
#39170=DIRECTION('',(0.,0.433825672914778,-0.900996828806872));
#39171=DIRECTION('center_axis',(-0.56100663158039,-0.731893183196511,0.386786669513445));
#39172=DIRECTION('ref_axis',(0.567619122871719,0.,0.823291279773046));
#39173=DIRECTION('',(0.705516335778319,-0.178310545369067,0.685895071683797));
#39174=DIRECTION('',(-0.705516335778307,0.667143602430338,0.239094361468903));
#39175=DIRECTION('',(0.,-0.467240138462762,-0.884130450221741));
#39176=DIRECTION('center_axis',(-0.707106781186539,-0.685229874095371,-0.174527991013631));
#39177=DIRECTION('ref_axis',(-0.239628661022763,0.,0.97086461714105));
#39178=DIRECTION('',(0.,-0.246819851905204,0.96906138128887));
#39179=DIRECTION('',(0.,0.246819851905204,-0.96906138128887));
#39180=DIRECTION('center_axis',(0.,-0.884130450221741,0.467240138462762));
#39181=DIRECTION('ref_axis',(0.,-0.467240138462762,-0.884130450221741));
#39182=DIRECTION('',(-1.,0.,0.));
#39183=DIRECTION('',(1.,0.,0.));
#39184=DIRECTION('center_axis',(-0.707106781186536,-0.241844762647979,0.664463024388686));
#39185=DIRECTION('ref_axis',(0.684791078771748,0.,0.728739444818671));
#39186=DIRECTION('',(0.,0.939692620785908,0.342020143325669));
#39187=DIRECTION('',(0.,-0.939692620785908,-0.342020143325669));
#39188=DIRECTION('center_axis',(0.,0.376947046632547,0.926234810420662));
#39189=DIRECTION('ref_axis',(1.,0.,0.));
#39190=DIRECTION('',(-1.,0.,0.));
#39191=DIRECTION('',(1.,0.,0.));
#39192=DIRECTION('center_axis',(0.707106781186534,-0.685229874095376,-0.174527991013633));
#39193=DIRECTION('ref_axis',(-0.239628661022766,0.,-0.970864617141049));
#39194=DIRECTION('',(0.,-0.246819851905204,0.96906138128887));
#39195=DIRECTION('',(0.,0.246819851905204,-0.96906138128887));
#39196=DIRECTION('center_axis',(0.707106781186551,-0.241844762647974,0.664463024388671));
#39197=DIRECTION('ref_axis',(0.684791078771732,0.,-0.728739444818686));
#39198=DIRECTION('',(0.,0.939692620785908,0.342020143325669));
#39199=DIRECTION('',(0.,-0.939692620785908,-0.342020143325669));
#39200=DIRECTION('center_axis',(0.707106781186549,0.637100967476913,0.306761075170856));
#39201=DIRECTION('ref_axis',(0.397987666358442,0.,-0.917390765937047));
#39202=DIRECTION('',(0.,-0.433825672914778,0.900996828806872));
#39203=DIRECTION('',(0.,0.433825672914778,-0.900996828806872));
#39204=DIRECTION('center_axis',(1.,0.,0.));
#39205=DIRECTION('ref_axis',(0.,0.342020143325669,-0.939692620785908));
#39206=DIRECTION('center_axis',(0.,0.900996828806872,0.433825672914778));
#39207=DIRECTION('ref_axis',(0.,-0.433825672914778,0.900996828806872));
#39208=DIRECTION('center_axis',(0.,-0.342020143325669,0.939692620785908));
#39209=DIRECTION('ref_axis',(0.,-0.939692620785908,-0.342020143325669));
#39210=DIRECTION('center_axis',(0.707106781186553,0.607940616597033,0.36112076469183));
#39211=DIRECTION('ref_axis',(0.454822071931215,0.,-0.890582327965358));
#39212=DIRECTION('',(0.59559668304742,-0.236796741375872,-0.76758836261155));
#39213=DIRECTION('',(0.,0.510701883081733,-0.859757865108992));
#39214=DIRECTION('',(0.,-0.510701883081733,0.859757865108992));
#39215=DIRECTION('',(0.557191914001231,-0.793484241614037,0.244785476043498));
#39216=DIRECTION('center_axis',(1.,0.,0.));
#39217=DIRECTION('ref_axis',(0.,0.422618261740699,-0.90630778703665));
#39218=DIRECTION('',(0.,0.90630778703665,0.422618261740699));
#39219=DIRECTION('',(0.,-0.330339892306057,0.943862042647771));
#39220=DIRECTION('center_axis',(0.707106781186551,-0.298836238730118,0.640856382055785));
#39221=DIRECTION('ref_axis',(0.671542934237814,0.,-0.740965645273293));
#39222=DIRECTION('',(0.557191914001249,0.793484241614025,-0.244785476043494));
#39223=DIRECTION('',(0.,-0.90630778703665,-0.422618261740699));
#39224=DIRECTION('',(0.705516335778313,0.237411714330102,-0.66774424583727));
#39225=DIRECTION('center_axis',(0.,0.294785966455752,0.955563307154868));
#39226=DIRECTION('ref_axis',(1.,0.,0.));
#39227=DIRECTION('',(-1.,0.,0.));
#39228=DIRECTION('',(0.,-0.955563307154868,0.294785966455752));
#39229=DIRECTION('',(1.,0.,0.));
#39230=DIRECTION('center_axis',(0.561006631580425,-0.762818788136162,0.321526135468429));
#39231=DIRECTION('ref_axis',(0.497247150959866,0.,-0.867608938901793));
#39232=DIRECTION('',(0.,0.388405102597383,0.921488728241597));
#39233=DIRECTION('',(-0.705516335778293,-0.643766472946365,-0.296329931428075));
#39234=DIRECTION('center_axis',(-0.5610066315804,0.244027156056943,0.791026109827971));
#39235=DIRECTION('ref_axis',(0.815685591418257,0.,0.578495476173019));
#39236=DIRECTION('',(0.705516335778303,0.640807009641843,0.302676520965595));
#39237=DIRECTION('',(-0.705516335778314,0.358916460582501,-0.611085652157594));
#39238=DIRECTION('center_axis',(-0.707106781186546,0.607940616597039,0.361120764691834));
#39239=DIRECTION('ref_axis',(0.454822071931222,0.,0.890582327965354));
#39240=DIRECTION('',(0.,-0.510701883081733,0.859757865108992));
#39241=DIRECTION('',(0.,0.510701883081733,-0.859757865108992));
#39242=DIRECTION('center_axis',(-0.561006631580432,-0.762818788136158,0.321526135468427));
#39243=DIRECTION('ref_axis',(0.497247150959859,0.,0.867608938901797));
#39244=DIRECTION('',(0.705516335778298,-0.237411714330121,0.667744245837279));
#39245=DIRECTION('',(-0.705516335778289,0.643766472946371,0.296329931428072));
#39246=DIRECTION('',(0.,-0.388405102597383,-0.921488728241597));
#39247=DIRECTION('center_axis',(-0.707106781186562,-0.667411250860812,-0.233585577946042));
#39248=DIRECTION('ref_axis',(-0.31366848359403,0.,0.949532559947168));
#39249=DIRECTION('',(0.,-0.330339892306057,0.943862042647771));
#39250=DIRECTION('',(0.,0.330339892306057,-0.943862042647771));
#39251=DIRECTION('center_axis',(0.,-0.921488728241597,0.388405102597383));
#39252=DIRECTION('ref_axis',(0.,-0.388405102597383,-0.921488728241597));
#39253=DIRECTION('',(-1.,0.,0.));
#39254=DIRECTION('',(1.,0.,0.));
#39255=DIRECTION('center_axis',(-0.70710678118655,-0.298836238730119,0.640856382055787));
#39256=DIRECTION('ref_axis',(0.671542934237816,0.,0.740965645273291));
#39257=DIRECTION('',(0.,0.90630778703665,0.422618261740699));
#39258=DIRECTION('',(0.,-0.90630778703665,-0.422618261740699));
#39259=DIRECTION('center_axis',(0.707106781186557,-0.667411250860816,-0.233585577946044));
#39260=DIRECTION('ref_axis',(-0.313668483594033,0.,-0.949532559947167));
#39261=DIRECTION('',(0.,0.330339892306057,-0.943862042647771));
#39262=DIRECTION('center_axis',(0.,0.859757865108992,0.510701883081733));
#39263=DIRECTION('ref_axis',(0.,-0.510701883081733,0.859757865108992));
#39264=DIRECTION('center_axis',(0.,-0.422618261740699,0.90630778703665));
#39265=DIRECTION('ref_axis',(0.,-0.90630778703665,-0.422618261740699));
#39266=DIRECTION('center_axis',(0.561006631580408,0.174156090919479,0.809284384699502));
#39267=DIRECTION('ref_axis',(0.821843752318935,0.,-0.569712951208179));
#39268=DIRECTION('',(0.705516335778312,-0.611988548508171,-0.357374756306047));
#39269=DIRECTION('',(0.,0.977619390136733,-0.210381387077569));
#39270=DIRECTION('',(-0.705516335778306,-0.410810298986386,0.577478656052905));
#39271=DIRECTION('center_axis',(0.561006631580416,-0.787938881495562,0.253818593389686));
#39272=DIRECTION('ref_axis',(0.412208150462307,0.,-0.911089699586404));
#39273=DIRECTION('',(0.705516335778306,0.29470603679192,-0.644511483084942));
#39274=DIRECTION('',(0.,0.306614069375781,0.951833920629446));
#39275=DIRECTION('',(-0.705516335778295,-0.6154898918864,-0.351310251680243));
#39276=DIRECTION('center_axis',(-0.561006631580406,0.174156090919479,0.809284384699503));
#39277=DIRECTION('ref_axis',(0.821843752318936,0.,0.569712951208178));
#39278=DIRECTION('',(0.,-0.977619390136733,0.210381387077569));
#39279=DIRECTION('',(0.705516335778313,0.61198854850817,0.357374756306046));
#39280=DIRECTION('',(-0.705516335778307,0.410810298986385,-0.577478656052904));
#39281=DIRECTION('center_axis',(-0.707106781186541,0.574153470540282,0.412732107142829));
#39282=DIRECTION('ref_axis',(0.504101701135477,0.,0.863644298836227));
#39283=DIRECTION('',(0.,-0.583691343548208,0.81197562492164));
#39284=DIRECTION('',(0.,0.583691343548208,-0.81197562492164));
#39285=DIRECTION('center_axis',(-0.561006631580414,-0.787938881495563,0.253818593389686));
#39286=DIRECTION('ref_axis',(0.412208150462309,0.,0.911089699586403));
#39287=DIRECTION('',(0.705516335778305,-0.294706036791931,0.644511483084939));
#39288=DIRECTION('',(-0.705516335778296,0.615489891886399,0.351310251680242));
#39289=DIRECTION('',(0.,-0.306614069375781,-0.951833920629446));
#39290=DIRECTION('center_axis',(-0.707106781186555,-0.644513225013298,-0.290865437587464));
#39291=DIRECTION('ref_axis',(-0.380418570543382,0.,0.924814419862564));
#39292=DIRECTION('',(0.,-0.411345846661781,0.911479343942639));
#39293=DIRECTION('',(0.,0.411345846661781,-0.911479343942639));
#39294=DIRECTION('center_axis',(0.,-0.951833920629447,0.306614069375781));
#39295=DIRECTION('ref_axis',(0.,-0.306614069375781,-0.951833920629446));
#39296=DIRECTION('',(-1.,0.,0.));
#39297=DIRECTION('',(1.,0.,0.));
#39298=DIRECTION('center_axis',(-0.707106781186547,-0.353553390593274,0.612372435695795));
#39299=DIRECTION('ref_axis',(0.654653670707978,0.,0.755928946018454));
#39300=DIRECTION('',(0.,0.866025403784439,0.5));
#39301=DIRECTION('',(0.,-0.866025403784439,-0.5));
#39302=DIRECTION('center_axis',(0.,0.210381387077569,0.977619390136733));
#39303=DIRECTION('ref_axis',(1.,0.,0.));
#39304=DIRECTION('',(-1.,0.,0.));
#39305=DIRECTION('',(1.,0.,0.));
#39306=DIRECTION('center_axis',(0.707106781186557,-0.644513225013297,-0.290865437587463));
#39307=DIRECTION('ref_axis',(-0.38041857054338,0.,-0.924814419862564));
#39308=DIRECTION('',(0.,-0.411345846661781,0.911479343942639));
#39309=DIRECTION('',(0.,0.411345846661781,-0.911479343942639));
#39310=DIRECTION('center_axis',(0.707106781186549,-0.353553390593273,0.612372435695794));
#39311=DIRECTION('ref_axis',(0.654653670707976,0.,-0.755928946018455));
#39312=DIRECTION('',(0.,0.866025403784439,0.5));
#39313=DIRECTION('',(0.,-0.866025403784439,-0.5));
#39314=DIRECTION('center_axis',(0.707106781186542,0.57415347054028,0.412732107142828));
#39315=DIRECTION('ref_axis',(0.504101701135476,0.,-0.863644298836228));
#39316=DIRECTION('',(0.,-0.583691343548208,0.81197562492164));
#39317=DIRECTION('',(0.,0.583691343548208,-0.81197562492164));
#39318=DIRECTION('center_axis',(1.,0.,0.));
#39319=DIRECTION('ref_axis',(0.,0.5,-0.866025403784439));
#39320=DIRECTION('center_axis',(0.,0.81197562492164,0.583691343548208));
#39321=DIRECTION('ref_axis',(0.,-0.583691343548208,0.81197562492164));
#39322=DIRECTION('center_axis',(0.,-0.5,0.866025403784439));
#39323=DIRECTION('ref_axis',(0.,-0.866025403784439,-0.5));
#39324=DIRECTION('center_axis',(0.561006631580412,-0.807062284196263,0.184179338555415));
#39325=DIRECTION('ref_axis',(0.311921838389587,0.,-0.950107765853779));
#39326=DIRECTION('',(0.705516335778304,0.349757468365403,-0.616373598779652));
#39327=DIRECTION('',(0.,0.222489517947625,0.97493508214826));
#39328=DIRECTION('',(-0.705516335778314,-0.582529061106241,-0.403616888790129));
#39329=DIRECTION('center_axis',(0.,-0.97493508214826,0.222489517947625));
#39330=DIRECTION('ref_axis',(0.,-0.222489517947625,-0.97493508214826));
#39331=DIRECTION('',(0.557191914001254,-0.184751680075895,-0.809570248762115));
#39332=DIRECTION('',(1.,0.,0.));
#39333=DIRECTION('',(-1.,0.,0.));
#39334=DIRECTION('',(-0.557191914001257,-0.184751680075895,-0.809570248762113));
#39335=DIRECTION('center_axis',(0.707106781186546,-0.61671006435571,-0.345931635619494));
#39336=DIRECTION('ref_axis',(-0.439451044888514,0.,-0.898266541259549));
#39337=DIRECTION('',(0.,-0.489221210746995,0.872159737063827));
#39338=DIRECTION('',(0.,0.489221210746995,-0.872159737063827));
#39339=DIRECTION('center_axis',(0.561006631580408,0.1029595927718,0.8213835167442));
#39340=DIRECTION('ref_axis',(0.82577204978196,0.,-0.564004008672722));
#39341=DIRECTION('',(0.705516335778304,-0.578512484991598,-0.409353153962201));
#39342=DIRECTION('',(0.,0.992235199256928,-0.124375678311979));
#39343=DIRECTION('',(-0.705516335778303,-0.459577622960939,0.539476698684503));
#39344=DIRECTION('center_axis',(0.,0.124375678311979,0.992235199256928));
#39345=DIRECTION('ref_axis',(1.,0.,0.));
#39346=DIRECTION('',(0.55719191400126,-0.823935984868783,0.103279542068703));
#39347=DIRECTION('',(1.,0.,0.));
#39348=DIRECTION('',(-1.,0.,0.));
#39349=DIRECTION('',(-0.557191914001244,-0.823935984868793,0.103279542068704));
#39350=DIRECTION('center_axis',(0.707106781186547,-0.405579787672639,0.579227965339569));
#39351=DIRECTION('ref_axis',(0.633687274224642,0.,-0.773589321594955));
#39352=DIRECTION('',(0.,0.819152044288992,0.573576436351046));
#39353=DIRECTION('',(0.,-0.819152044288992,-0.573576436351046));
#39354=DIRECTION('center_axis',(0.707106781186547,0.53599666988936,0.461202309044));
#39355=DIRECTION('ref_axis',(0.546305769586287,0.,-0.837585820150231));
#39356=DIRECTION('',(0.,-0.652238560447812,0.758013759944347));
#39357=DIRECTION('',(0.,0.652238560447812,-0.758013759944347));
#39358=DIRECTION('center_axis',(-0.707106781186539,-0.616710064355716,-0.345931635619497));
#39359=DIRECTION('ref_axis',(-0.439451044888521,0.,0.898266541259546));
#39360=DIRECTION('',(-0.595596683047429,0.783149392358831,-0.178722187740901));
#39361=DIRECTION('',(0.,0.489221210746995,-0.872159737063827));
#39362=DIRECTION('',(0.,-0.489221210746995,0.872159737063827));
#39363=DIRECTION('center_axis',(0.,-0.573576436351046,0.819152044288992));
#39364=DIRECTION('ref_axis',(0.,-0.819152044288992,-0.573576436351046));
#39365=DIRECTION('',(0.,0.819152044288992,0.573576436351046));
#39366=DIRECTION('center_axis',(-0.707106781186532,-0.405579787672648,0.579227965339582));
#39367=DIRECTION('ref_axis',(0.633687274224659,0.,0.773589321594942));
#39368=DIRECTION('',(0.595596683047437,0.0999089464291446,0.797046293239175));
#39369=DIRECTION('',(0.,-0.819152044288992,-0.573576436351046));
#39370=DIRECTION('center_axis',(-0.707106781186546,0.535996669889361,0.461202309044001));
#39371=DIRECTION('ref_axis',(0.546305769586289,0.,0.83758582015023));
#39372=DIRECTION('',(0.,0.652238560447812,-0.758013759944347));
#39373=DIRECTION('',(0.,-0.652238560447812,0.758013759944347));
#39374=DIRECTION('center_axis',(0.,0.758013759944347,0.652238560447812));
#39375=DIRECTION('ref_axis',(0.,-0.652238560447812,0.758013759944347));
#39376=DIRECTION('center_axis',(0.,-0.872159737063827,-0.489221210746995));
#39377=DIRECTION('ref_axis',(0.,0.489221210746995,-0.872159737063827));
#39378=DIRECTION('center_axis',(0.56100663158041,0.0309795099544078,0.827231424261547));
#39379=DIRECTION('ref_axis',(0.827628669643383,0.,-0.561276032968025));
#39380=DIRECTION('',(0.705516335778304,-0.540633592148827,-0.458216126942529));
#39381=DIRECTION('',(0.,0.999299499382783,-0.037423395534326));
#39382=DIRECTION('',(-0.705516335778297,-0.50484728372422,0.497368997894162));
#39383=DIRECTION('center_axis',(0.561006631580422,-0.820043455596693,0.113138367744206));
#39384=DIRECTION('ref_axis',(0.197690230426216,0.,-0.980264542250728));
#39385=DIRECTION('',(0.70551633577829,0.402147034415294,-0.583544739211107));
#39386=DIRECTION('',(0.,0.136671686945037,0.990616399010029));
#39387=DIRECTION('',(-0.705516335778305,-0.545134832430407,-0.452851757665825));
#39388=DIRECTION('center_axis',(-0.561006631580388,0.0309795099544084,0.827231424261562));
#39389=DIRECTION('ref_axis',(0.827628669643398,0.,0.561276032968003));
#39390=DIRECTION('',(0.,-0.999299499382783,0.037423395534326));
#39391=DIRECTION('',(0.705516335778314,0.540633592148832,0.458216126942508));
#39392=DIRECTION('',(-0.705516335778307,0.504847283724225,-0.497368997894142));
#39393=DIRECTION('center_axis',(-0.70710678118654,0.493760610936952,0.506162482891787));
#39394=DIRECTION('ref_axis',(0.582064997116551,0.,0.813142262541868));
#39395=DIRECTION('',(0.,-0.715821848069997,0.698282952552655));
#39396=DIRECTION('',(0.,0.715821848069997,-0.698282952552655));
#39397=DIRECTION('center_axis',(-0.561006631580398,-0.820043455596709,0.113138367744208));
#39398=DIRECTION('ref_axis',(0.197690230426228,0.,0.980264542250726));
#39399=DIRECTION('',(0.70551633577832,-0.402147034415284,0.583544739211079));
#39400=DIRECTION('',(-0.705516335778308,0.545134832430382,0.45285175766585));
#39401=DIRECTION('',(0.,-0.136671686945037,-0.990616399010029));
#39402=DIRECTION('center_axis',(-0.70710678118654,-0.584213367728653,-0.398365085025227));
#39403=DIRECTION('ref_axis',(-0.490839120629142,0.,0.871250226777595));
#39404=DIRECTION('',(0.,-0.563373306018581,0.826202467961513));
#39405=DIRECTION('',(0.,0.563373306018581,-0.826202467961513));
#39406=DIRECTION('center_axis',(0.,-0.990616399010029,0.136671686945037));
#39407=DIRECTION('ref_axis',(0.,-0.136671686945037,-0.990616399010029));
#39408=DIRECTION('',(-1.,0.,0.));
#39409=DIRECTION('',(1.,0.,0.));
#39410=DIRECTION('center_axis',(-0.70710678118653,-0.454519477672055,0.541675220419715));
#39411=DIRECTION('ref_axis',(0.608120402411362,0.,0.793844806099431));
#39412=DIRECTION('',(0.,0.766044443118978,0.642787609686539));
#39413=DIRECTION('',(0.,-0.766044443118978,-0.642787609686539));
#39414=DIRECTION('center_axis',(0.,0.037423395534326,0.999299499382783));
#39415=DIRECTION('ref_axis',(1.,0.,0.));
#39416=DIRECTION('',(-1.,0.,0.));
#39417=DIRECTION('',(1.,0.,0.));
#39418=DIRECTION('center_axis',(0.707106781186542,-0.584213367728652,-0.398365085025226));
#39419=DIRECTION('ref_axis',(-0.490839120629141,0.,-0.871250226777596));
#39420=DIRECTION('',(0.,-0.563373306018581,0.826202467961513));
#39421=DIRECTION('',(0.,0.563373306018581,-0.826202467961513));
#39422=DIRECTION('center_axis',(0.707106781186559,-0.454519477672036,0.541675220419693));
#39423=DIRECTION('ref_axis',(0.60812040241133,0.,-0.793844806099455));
#39424=DIRECTION('',(0.,0.766044443118978,0.642787609686539));
#39425=DIRECTION('',(0.,-0.766044443118978,-0.642787609686539));
#39426=DIRECTION('center_axis',(0.707106781186551,0.493760610936944,0.50616248289178));
#39427=DIRECTION('ref_axis',(0.58206499711654,0.,-0.813142262541876));
#39428=DIRECTION('',(0.,-0.715821848069997,0.698282952552655));
#39429=DIRECTION('',(0.,0.715821848069997,-0.698282952552655));
#39430=DIRECTION('center_axis',(1.,0.,0.));
#39431=DIRECTION('ref_axis',(0.,0.642787609686539,-0.766044443118978));
#39432=DIRECTION('center_axis',(0.,0.698282952552655,0.715821848069998));
#39433=DIRECTION('ref_axis',(0.,-0.715821848069997,0.698282952552655));
#39434=DIRECTION('center_axis',(0.,-0.642787609686539,0.766044443118978));
#39435=DIRECTION('ref_axis',(0.,-0.766044443118978,-0.642787609686539));
#39436=DIRECTION('center_axis',(0.561006631580394,-0.041236345639636,0.826783601144283));
#39437=DIRECTION('ref_axis',(0.827487445286316,0.,-0.561484218739517));
#39438=DIRECTION('',(0.705516335778304,-0.498640151226356,-0.503591798518316));
#39439=DIRECTION('',(0.,0.998758526924799,0.049813701880158));
#39440=DIRECTION('',(-0.705516335778303,-0.546274751823203,0.451476018710246));
#39441=DIRECTION('center_axis',(0.561006631580414,-0.826783601144269,0.0412363456396373));
#39442=DIRECTION('ref_axis',(0.0733064378127061,0.,-0.997309463594531));
#39443=DIRECTION('',(0.705516335778305,0.451476018710272,-0.546274751823179));
#39444=DIRECTION('',(0.,0.0498137018801604,0.998758526924799));
#39445=DIRECTION('',(-0.705516335778304,-0.503591798518341,-0.49864015122633));
#39446=DIRECTION('center_axis',(-0.561006631580412,-0.0412363456396354,
0.826783601144271));
#39447=DIRECTION('ref_axis',(0.827487445286305,0.,0.561484218739534));
#39448=DIRECTION('',(0.,-0.998758526924799,-0.049813701880158));
#39449=DIRECTION('',(0.705516335778288,0.498640151226367,0.503591798518327));
#39450=DIRECTION('',(-0.705516335778307,0.546274751823178,-0.451476018710271));
#39451=DIRECTION('center_axis',(-0.70710678118655,0.447766735594494,0.547270454615492));
#39452=DIRECTION('ref_axis',(0.61205637248212,0.,0.790814135498366));
#39453=DIRECTION('',(0.,-0.773957299203321,0.633237790257263));
#39454=DIRECTION('',(0.,0.773957299203321,-0.633237790257263));
#39455=DIRECTION('center_axis',(-0.561006631580413,-0.82678360114427,0.0412363456396374));
#39456=DIRECTION('ref_axis',(0.0733064378127065,0.,0.997309463594531));
#39457=DIRECTION('',(0.705516335778307,-0.451476018710271,0.546274751823178));
#39458=DIRECTION('',(-0.705516335778306,0.50359179851834,0.498640151226329));
#39459=DIRECTION('',(0.,-0.0498137018801604,-0.998758526924799));
#39460=DIRECTION('center_axis',(-0.70710678118655,-0.547270454615492,-0.447766735594494));
#39461=DIRECTION('ref_axis',(-0.534994468449985,0.,0.844855560867015));
#39462=DIRECTION('',(0.,-0.633237790257263,0.773957299203321));
#39463=DIRECTION('',(0.,0.633237790257263,-0.773957299203321));
#39464=DIRECTION('center_axis',(0.,-0.998758526924799,0.0498137018801604));
#39465=DIRECTION('ref_axis',(0.,-0.0498137018801604,-0.998758526924799));
#39466=DIRECTION('',(-1.,0.,0.));
#39467=DIRECTION('',(1.,0.,0.));
#39468=DIRECTION('center_axis',(-0.707106781186547,-0.500000000000001,0.500000000000001));
#39469=DIRECTION('ref_axis',(0.577350269189627,0.,0.816496580927725));
#39470=DIRECTION('',(0.,0.707106781186548,0.707106781186548));
#39471=DIRECTION('',(0.,-0.707106781186547,-0.707106781186547));
#39472=DIRECTION('center_axis',(0.,-0.049813701880158,0.998758526924799));
#39473=DIRECTION('ref_axis',(1.,0.,0.));
#39474=DIRECTION('',(-1.,0.,0.));
#39475=DIRECTION('',(1.,0.,0.));
#39476=DIRECTION('center_axis',(0.707106781186552,-0.547270454615491,-0.447766735594493));
#39477=DIRECTION('ref_axis',(-0.534994468449983,0.,-0.844855560867016));
#39478=DIRECTION('',(0.,-0.633237790257263,0.773957299203321));
#39479=DIRECTION('',(0.,0.633237790257263,-0.773957299203321));
#39480=DIRECTION('center_axis',(0.707106781186548,-0.5,0.5));
#39481=DIRECTION('ref_axis',(0.577350269189625,0.,-0.816496580927726));
#39482=DIRECTION('',(0.,0.707106781186548,0.707106781186548));
#39483=DIRECTION('',(0.,-0.707106781186548,-0.707106781186548));
#39484=DIRECTION('center_axis',(0.707106781186552,0.447766735594493,0.547270454615491));
#39485=DIRECTION('ref_axis',(0.612056372482119,0.,-0.790814135498367));
#39486=DIRECTION('',(0.,-0.773957299203321,0.633237790257263));
#39487=DIRECTION('',(0.,0.773957299203321,-0.633237790257263));
#39488=DIRECTION('center_axis',(1.,0.,0.));
#39489=DIRECTION('ref_axis',(0.,0.707106781186548,-0.707106781186548));
#39490=DIRECTION('center_axis',(0.,0.633237790257263,0.773957299203321));
#39491=DIRECTION('ref_axis',(0.,-0.773957299203321,0.633237790257263));
#39492=DIRECTION('center_axis',(0.,-0.707106781186548,0.707106781186548));
#39493=DIRECTION('ref_axis',(0.,-0.707106781186548,-0.707106781186548));
#39494=DIRECTION('center_axis',(0.707106781186549,0.398365085025222,0.584213367728646));
#39495=DIRECTION('ref_axis',(0.636934375125929,0.,-0.770918025332747));
#39496=DIRECTION('',(0.595596683047418,0.109786128885441,-0.795745937499692));
#39497=DIRECTION('',(0.,0.826202467961513,-0.563373306018581));
#39498=DIRECTION('',(0.,-0.826202467961513,0.563373306018581));
#39499=DIRECTION('',(0.557191914001254,-0.822591759450525,-0.1134899478179));
#39500=DIRECTION('center_axis',(1.,0.,0.));
#39501=DIRECTION('ref_axis',(0.,0.766044443118978,-0.642787609686539));
#39502=DIRECTION('',(0.,0.642787609686539,0.766044443118978));
#39503=DIRECTION('',(0.,-0.698282952552655,0.715821848069998));
#39504=DIRECTION('center_axis',(0.707106781186559,-0.541675220419693,0.454519477672036));
#39505=DIRECTION('ref_axis',(0.540716203060924,0.,-0.8412050806714));
#39506=DIRECTION('',(0.557191914001221,0.822591759450547,0.113489947817903));
#39507=DIRECTION('',(0.,-0.642787609686539,-0.766044443118978));
#39508=DIRECTION('',(0.705516335778297,0.497368997894187,-0.504847283724195));
#39509=DIRECTION('center_axis',(0.,-0.136671686945054,0.990616399010027));
#39510=DIRECTION('ref_axis',(1.,0.,0.));
#39511=DIRECTION('',(-1.,0.,0.));
#39512=DIRECTION('',(0.,-0.990616399010027,-0.136671686945054));
#39513=DIRECTION('',(1.,0.,0.));
#39514=DIRECTION('center_axis',(0.56100663158042,-0.827231424261539,-0.0309795099544281));
#39515=DIRECTION('ref_axis',(-0.055137286528771,0.,-0.998478782766186));
#39516=DIRECTION('',(0.,-0.0374233955343508,0.999299499382783));
#39517=DIRECTION('',(-0.705516335778304,-0.458216126942529,-0.540633592148827));
#39518=DIRECTION('center_axis',(-0.561006631580388,-0.113138367744223,0.820043455596714));
#39519=DIRECTION('ref_axis',(0.825342782028785,0.,0.56463199710341));
#39520=DIRECTION('',(0.7055163357783,0.45285175766587,0.545134832430375));
#39521=DIRECTION('',(-0.705516335778316,0.583544739211101,-0.402147034415257));
#39522=DIRECTION('center_axis',(-0.707106781186547,0.398365085025223,0.584213367728647));
#39523=DIRECTION('ref_axis',(0.636934375125931,0.,0.770918025332746));
#39524=DIRECTION('',(0.,-0.826202467961513,0.563373306018581));
#39525=DIRECTION('',(0.,0.826202467961513,-0.563373306018581));
#39526=DIRECTION('center_axis',(-0.56100663158042,-0.827231424261539,-0.0309795099544281));
#39527=DIRECTION('ref_axis',(-0.055137286528771,0.,0.998478782766186));
#39528=DIRECTION('',(0.705516335778325,-0.49736899789418,0.504847283724163));
#39529=DIRECTION('',(-0.705516335778286,0.458216126942515,0.540633592148861));
#39530=DIRECTION('',(0.,0.0374233955343508,-0.999299499382783));
#39531=DIRECTION('center_axis',(-0.707106781186558,-0.506162482891774,-0.493760610936939));
#39532=DIRECTION('ref_axis',(-0.572517134274658,0.,0.819892755768663));
#39533=DIRECTION('',(0.,-0.698282952552655,0.715821848069998));
#39534=DIRECTION('',(0.,0.698282952552655,-0.715821848069998));
#39535=DIRECTION('center_axis',(0.,-0.999299499382783,-0.0374233955343508));
#39536=DIRECTION('ref_axis',(0.,0.0374233955343508,-0.999299499382783));
#39537=DIRECTION('',(-1.,0.,0.));
#39538=DIRECTION('',(1.,0.,0.));
#39539=DIRECTION('center_axis',(-0.70710678118653,-0.541675220419715,0.454519477672055));
#39540=DIRECTION('ref_axis',(0.540716203060955,0.,0.84120508067138));
#39541=DIRECTION('',(0.,0.642787609686539,0.766044443118978));
#39542=DIRECTION('',(0.,-0.642787609686539,-0.766044443118978));
#39543=DIRECTION('center_axis',(0.707106781186551,-0.50616248289178,-0.493760610936944));
#39544=DIRECTION('ref_axis',(-0.572517134274666,0.,-0.819892755768658));
#39545=DIRECTION('',(0.,0.698282952552655,-0.715821848069998));
#39546=DIRECTION('center_axis',(0.,0.563373306018581,0.826202467961513));
#39547=DIRECTION('ref_axis',(0.,-0.826202467961513,0.563373306018581));
#39548=DIRECTION('center_axis',(0.,-0.766044443118978,0.642787609686539));
#39549=DIRECTION('ref_axis',(0.,-0.642787609686539,-0.766044443118978));
#39550=DIRECTION('center_axis',(0.56100663158041,-0.184179338555411,0.807062284196266));
#39551=DIRECTION('ref_axis',(0.821109284001917,0.,-0.570771008133611));
#39552=DIRECTION('',(0.705516335778307,-0.40361688879015,-0.582529061106235));
#39553=DIRECTION('',(0.,0.974935082148261,0.22248951794762));
#39554=DIRECTION('',(-0.705516335778304,-0.616373598779652,0.349757468365403));
#39555=DIRECTION('center_axis',(0.561006631580401,-0.821383516744203,-0.102959592771817));
#39556=DIRECTION('ref_axis',(-0.180511696561755,0.,-0.983572837874449));
#39557=DIRECTION('',(0.705516335778307,0.539476698684506,-0.459577622960929));
#39558=DIRECTION('',(0.,-0.124375678312,0.992235199256925));
#39559=DIRECTION('',(-0.705516335778296,-0.409353153962171,-0.578512484991629));
#39560=DIRECTION('center_axis',(-0.561006631580408,-0.184179338555411,0.807062284196267));
#39561=DIRECTION('ref_axis',(0.821109284001918,0.,0.570771008133609));
#39562=DIRECTION('',(0.,-0.974935082148261,-0.22248951794762));
#39563=DIRECTION('',(0.705516335778308,0.403616888790149,0.582529061106233));
#39564=DIRECTION('',(-0.705516335778306,0.616373598779651,-0.349757468365402));
#39565=DIRECTION('center_axis',(-0.707106781186545,0.345931635619495,0.616710064355711));
#39566=DIRECTION('ref_axis',(0.657291420225582,0.,0.753636509796226));
#39567=DIRECTION('',(0.,-0.872159737063827,0.489221210746995));
#39568=DIRECTION('',(0.,0.872159737063827,-0.489221210746995));
#39569=DIRECTION('center_axis',(-0.561006631580399,-0.821383516744204,-0.102959592771817));
#39570=DIRECTION('ref_axis',(-0.180511696561756,0.,0.983572837874449));
#39571=DIRECTION('',(0.705516335778309,-0.539476698684505,0.459577622960928));
#39572=DIRECTION('',(-0.705516335778298,0.40935315396217,0.578512484991627));
#39573=DIRECTION('',(0.,0.124375678312,-0.992235199256925));
#39574=DIRECTION('center_axis',(-0.707106781186551,-0.461202309043998,-0.535996669889357));
#39575=DIRECTION('ref_axis',(-0.604079438549189,0.,0.796924106751764));
#39576=DIRECTION('',(0.,-0.758013759944347,0.652238560447812));
#39577=DIRECTION('',(0.,0.758013759944347,-0.652238560447812));
#39578=DIRECTION('center_axis',(0.,-0.992235199256925,-0.124375678312));
#39579=DIRECTION('ref_axis',(0.,0.124375678312,-0.992235199256925));
#39580=DIRECTION('',(-1.,0.,0.));
#39581=DIRECTION('',(1.,0.,0.));
#39582=DIRECTION('center_axis',(-0.707106781186546,-0.579227965339571,0.40557978767264));
#39583=DIRECTION('ref_axis',(0.497542812164525,0.,0.867439421552546));
#39584=DIRECTION('',(0.,0.573576436351046,0.819152044288992));
#39585=DIRECTION('',(0.,-0.573576436351046,-0.819152044288992));
#39586=DIRECTION('center_axis',(0.,-0.22248951794762,0.974935082148261));
#39587=DIRECTION('ref_axis',(1.,0.,0.));
#39588=DIRECTION('',(-1.,0.,0.));
#39589=DIRECTION('',(1.,0.,0.));
#39590=DIRECTION('center_axis',(0.707106781186552,-0.461202309043997,-0.535996669889356));
#39591=DIRECTION('ref_axis',(-0.604079438549187,0.,-0.796924106751765));
#39592=DIRECTION('',(0.,-0.758013759944347,0.652238560447812));
#39593=DIRECTION('',(0.,0.758013759944347,-0.652238560447812));
#39594=DIRECTION('center_axis',(0.707106781186547,-0.579227965339569,0.405579787672639));
#39595=DIRECTION('ref_axis',(0.497542812164523,0.,-0.867439421552547));
#39596=DIRECTION('',(0.,0.573576436351046,0.819152044288992));
#39597=DIRECTION('',(0.,-0.573576436351046,-0.819152044288992));
#39598=DIRECTION('center_axis',(0.707106781186546,0.345931635619494,0.61671006435571));
#39599=DIRECTION('ref_axis',(0.657291420225581,0.,-0.753636509796227));
#39600=DIRECTION('',(0.,-0.872159737063827,0.489221210746995));
#39601=DIRECTION('',(0.,0.872159737063827,-0.489221210746995));
#39602=DIRECTION('center_axis',(1.,0.,0.));
#39603=DIRECTION('ref_axis',(0.,0.819152044288992,-0.573576436351046));
#39604=DIRECTION('center_axis',(0.,0.489221210746995,0.872159737063827));
#39605=DIRECTION('ref_axis',(0.,-0.872159737063827,0.489221210746995));
#39606=DIRECTION('center_axis',(0.,-0.819152044288992,0.573576436351046));
#39607=DIRECTION('ref_axis',(0.,-0.573576436351046,-0.819152044288992));
#39608=DIRECTION('center_axis',(0.56100663158041,-0.809284384699501,-0.174156090919474));
#39609=DIRECTION('ref_axis',(-0.296477762129624,0.,-0.955039756535093));
#39610=DIRECTION('',(0.705516335778306,0.577478656052905,-0.410810298986386));
#39611=DIRECTION('',(0.,-0.210381387077564,0.977619390136734));
#39612=DIRECTION('',(-0.705516335778301,-0.357374756306042,-0.611988548508187));
#39613=DIRECTION('center_axis',(0.,-0.977619390136734,-0.210381387077564));
#39614=DIRECTION('ref_axis',(0.,0.210381387077564,-0.977619390136734));
#39615=DIRECTION('',(0.557191914001251,0.174697284967946,-0.811799254493653));
#39616=DIRECTION('',(1.,0.,0.));
#39617=DIRECTION('',(-1.,0.,0.));
#39618=DIRECTION('',(-0.55719191400123,0.174697284967949,-0.811799254493666));
#39619=DIRECTION('center_axis',(0.707106781186555,-0.412732107142821,-0.57415347054027));
#39620=DIRECTION('ref_axis',(-0.630347388214425,0.,-0.776313190774994));
#39621=DIRECTION('',(0.,-0.81197562492164,0.583691343548209));
#39622=DIRECTION('',(0.,0.81197562492164,-0.583691343548209));
#39623=DIRECTION('center_axis',(0.561006631580402,-0.253818593389698,0.787938881495568));
#39624=DIRECTION('ref_axis',(0.814616058663784,0.,-0.580000583592019));
#39625=DIRECTION('',(0.7055163357783,-0.351310251680245,-0.615489891886393));
#39626=DIRECTION('',(0.,0.951833920629443,0.306614069375792));
#39627=DIRECTION('',(-0.705516335778309,-0.644511483084945,0.294706036791908));
#39628=DIRECTION('center_axis',(0.,-0.306614069375792,0.951833920629443));
#39629=DIRECTION('ref_axis',(1.,0.,0.));
#39630=DIRECTION('',(0.557191914001229,-0.790387419648759,-0.254607340492422));
#39631=DIRECTION('',(1.,0.,0.));
#39632=DIRECTION('',(-1.,0.,0.));
#39633=DIRECTION('',(-0.557191914001243,-0.79038741964875,-0.254607340492419));
#39634=DIRECTION('center_axis',(0.707106781186546,-0.612372435695796,0.353553390593275));
#39635=DIRECTION('ref_axis',(0.44721359549996,0.,-0.894427190999915));
#39636=DIRECTION('',(0.,0.5,0.866025403784439));
#39637=DIRECTION('',(0.,-0.5,-0.866025403784439));
#39638=DIRECTION('center_axis',(0.707106781186551,0.290865437587466,0.644513225013302));
#39639=DIRECTION('ref_axis',(0.673638686438954,0.,-0.739060836557317));
#39640=DIRECTION('',(0.,-0.911479343942638,0.411345846661781));
#39641=DIRECTION('',(0.,0.911479343942638,-0.411345846661781));
#39642=DIRECTION('center_axis',(-0.707106781186541,-0.412732107142829,-0.574153470540282));
#39643=DIRECTION('ref_axis',(-0.63034738821444,0.,0.776313190774982));
#39644=DIRECTION('',(-0.595596683047425,0.78530565302539,0.168995924416156));
#39645=DIRECTION('',(0.,0.81197562492164,-0.583691343548209));
#39646=DIRECTION('',(0.,-0.81197562492164,0.583691343548209));
#39647=DIRECTION('center_axis',(0.,-0.866025403784439,0.5));
#39648=DIRECTION('ref_axis',(0.,-0.5,-0.866025403784439));
#39649=DIRECTION('',(0.,0.5,0.866025403784439));
#39650=DIRECTION('center_axis',(-0.707106781186558,-0.612372435695785,0.353553390593269));
#39651=DIRECTION('ref_axis',(0.447213595499947,0.,0.894427190999921));
#39652=DIRECTION('',(0.595596683047419,-0.246298062832259,0.764592607463602));
#39653=DIRECTION('',(0.,-0.5,-0.866025403784438));
#39654=DIRECTION('center_axis',(-0.707106781186549,0.290865437587466,0.644513225013304));
#39655=DIRECTION('ref_axis',(0.673638686438956,0.,0.739060836557315));
#39656=DIRECTION('',(0.,0.911479343942638,-0.411345846661781));
#39657=DIRECTION('',(0.,-0.911479343942638,0.411345846661781));
#39658=DIRECTION('center_axis',(0.,0.411345846661781,0.911479343942639));
#39659=DIRECTION('ref_axis',(0.,-0.911479343942638,0.411345846661781));
#39660=DIRECTION('center_axis',(0.,-0.583691343548209,-0.81197562492164));
#39661=DIRECTION('ref_axis',(0.,0.81197562492164,-0.583691343548209));
#39662=DIRECTION('center_axis',(0.561006631580424,-0.321526135468413,0.762818788136169));
#39663=DIRECTION('ref_axis',(0.805595332751381,0.,-0.592466167683179));
#39664=DIRECTION('',(0.705516335778305,-0.29632993142808,-0.64376647294635));
#39665=DIRECTION('',(0.,0.921488728241605,0.388405102597364));
#39666=DIRECTION('',(-0.705516335778301,-0.667744245837284,0.237411714330098));
#39667=DIRECTION('center_axis',(0.561006631580402,-0.79102610982797,-0.244027156056943));
#39668=DIRECTION('ref_axis',(-0.398879012810071,0.,-0.917003562228448));
#39669=DIRECTION('',(0.705516335778309,0.611085652157592,-0.358916460582513));
#39670=DIRECTION('',(0.,-0.294785966455749,0.955563307154869));
#39671=DIRECTION('',(-0.705516335778301,-0.302676520965596,-0.640807009641845));
#39672=DIRECTION('center_axis',(-0.56100663158041,-0.321526135468408,0.762818788136182));
#39673=DIRECTION('ref_axis',(0.805595332751393,0.,0.592466167683162));
#39674=DIRECTION('',(0.,-0.921488728241605,-0.388405102597364));
#39675=DIRECTION('',(0.705516335778301,0.296329931428102,0.643766472946344));
#39676=DIRECTION('',(-0.705516335778315,0.667744245837269,-0.237411714330102));
#39677=DIRECTION('center_axis',(-0.70710678118655,0.233585577946046,0.667411250860823));
#39678=DIRECTION('ref_axis',(0.686399640790371,0.,0.727224541062009));
#39679=DIRECTION('',(0.,-0.943862042647771,0.330339892306057));
#39680=DIRECTION('',(0.,0.943862042647771,-0.330339892306057));
#39681=DIRECTION('center_axis',(-0.5610066315804,-0.791026109827971,-0.244027156056943));
#39682=DIRECTION('ref_axis',(-0.398879012810073,0.,0.917003562228447));
#39683=DIRECTION('',(0.705516335778317,-0.611085652157596,0.35891646058249));
#39684=DIRECTION('',(-0.705516335778303,0.302676520965595,0.640807009641843));
#39685=DIRECTION('',(0.,0.294785966455749,-0.955563307154869));
#39686=DIRECTION('center_axis',(-0.707106781186551,-0.361120764691831,-0.607940616597034));
#39687=DIRECTION('ref_axis',(-0.651933718094179,0.,0.758275957163288));
#39688=DIRECTION('',(0.,-0.859757865108992,0.510701883081733));
#39689=DIRECTION('',(0.,0.859757865108992,-0.510701883081733));
#39690=DIRECTION('center_axis',(0.,-0.955563307154869,-0.294785966455749));
#39691=DIRECTION('ref_axis',(0.,0.294785966455749,-0.955563307154869));
#39692=DIRECTION('',(-1.,0.,0.));
#39693=DIRECTION('',(1.,0.,0.));
#39694=DIRECTION('center_axis',(-0.707106781186538,-0.640856382055797,0.298836238730124));
#39695=DIRECTION('ref_axis',(0.389281620635034,0.,0.921118787038763));
#39696=DIRECTION('',(0.,0.422618261740699,0.90630778703665));
#39697=DIRECTION('',(0.,-0.422618261740699,-0.90630778703665));
#39698=DIRECTION('center_axis',(0.,-0.388405102597364,0.921488728241605));
#39699=DIRECTION('ref_axis',(1.,0.,0.));
#39700=DIRECTION('',(-1.,0.,0.));
#39701=DIRECTION('',(1.,0.,0.));
#39702=DIRECTION('center_axis',(0.707106781186553,-0.36112076469183,-0.607940616597033));
#39703=DIRECTION('ref_axis',(-0.651933718094177,0.,-0.758275957163289));
#39704=DIRECTION('',(0.,-0.859757865108992,0.510701883081733));
#39705=DIRECTION('',(0.,0.859757865108992,-0.510701883081733));
#39706=DIRECTION('center_axis',(0.707106781186554,-0.640856382055783,0.298836238730117));
#39707=DIRECTION('ref_axis',(0.389281620635019,0.,-0.921118787038769));
#39708=DIRECTION('',(0.,0.422618261740699,0.90630778703665));
#39709=DIRECTION('',(0.,-0.422618261740699,-0.90630778703665));
#39710=DIRECTION('center_axis',(0.707106781186551,0.233585577946046,0.667411250860822));
#39711=DIRECTION('ref_axis',(0.68639964079037,0.,-0.72722454106201));
#39712=DIRECTION('',(0.,-0.943862042647771,0.330339892306057));
#39713=DIRECTION('',(0.,0.943862042647771,-0.330339892306057));
#39714=DIRECTION('center_axis',(1.,0.,0.));
#39715=DIRECTION('ref_axis',(0.,0.90630778703665,-0.422618261740699));
#39716=DIRECTION('center_axis',(0.,0.330339892306057,0.943862042647771));
#39717=DIRECTION('ref_axis',(0.,-0.943862042647771,0.330339892306057));
#39718=DIRECTION('center_axis',(0.,-0.90630778703665,0.422618261740699));
#39719=DIRECTION('ref_axis',(0.,-0.422618261740699,-0.90630778703665));
#39720=DIRECTION('center_axis',(0.561006631580401,-0.386786669513441,0.731893183196504));
#39721=DIRECTION('ref_axis',(0.793664727118314,0.,-0.60835540675514));
#39722=DIRECTION('',(0.70551633577831,-0.23909436146888,-0.667143602430344));
#39723=DIRECTION('',(0.,0.884130450221741,0.467240138462762));
#39724=DIRECTION('',(-0.705516335778305,-0.685895071683811,0.178310545369065));
#39725=DIRECTION('center_axis',(0.561006631580418,-0.766747648626013,-0.312041027189173));
#39726=DIRECTION('ref_axis',(-0.486084108127403,0.,-0.873912032086747));
#39727=DIRECTION('',(0.705516335778306,0.640041917465772,-0.304291051193904));
#39728=DIRECTION('',(0.,-0.376947046632555,0.926234810420659));
#39729=DIRECTION('',(-0.705516335778304,-0.245674734539573,-0.66474854250225));
#39730=DIRECTION('center_axis',(-0.561006631580399,-0.386786669513442,0.731893183196506));
#39731=DIRECTION('ref_axis',(0.793664727118316,0.,0.608355406755138));
#39732=DIRECTION('',(0.,-0.884130450221741,-0.467240138462762));
#39733=DIRECTION('',(0.705516335778311,0.239094361468879,0.667143602430342));
#39734=DIRECTION('',(-0.705516335778307,0.68589507168381,-0.178310545369064));
#39735=DIRECTION('center_axis',(-0.707106781186539,0.174527991013632,0.685229874095371));
#39736=DIRECTION('ref_axis',(0.695910561235553,0.,0.718128463967846));
#39737=DIRECTION('',(0.,-0.96906138128887,0.246819851905204));
#39738=DIRECTION('',(0.,0.96906138128887,-0.246819851905204));
#39739=DIRECTION('center_axis',(-0.561006631580416,-0.766747648626014,-0.312041027189174));
#39740=DIRECTION('ref_axis',(-0.486084108127405,0.,0.873912032086746));
#39741=DIRECTION('',(0.705516335778307,-0.640041917465771,0.304291051193903));
#39742=DIRECTION('',(-0.705516335778305,0.245674734539572,0.664748542502249));
#39743=DIRECTION('',(0.,0.376947046632555,-0.926234810420659));
#39744=DIRECTION('center_axis',(-0.707106781186547,-0.306761075170857,-0.637100967476915));
#39745=DIRECTION('ref_axis',(-0.669373784875801,0.,0.742925794491647));
#39746=DIRECTION('',(0.,-0.900996828806872,0.433825672914778));
#39747=DIRECTION('',(0.,0.900996828806872,-0.433825672914778));
#39748=DIRECTION('center_axis',(0.,-0.926234810420659,-0.376947046632555));
#39749=DIRECTION('ref_axis',(0.,0.376947046632555,-0.926234810420659));
#39750=DIRECTION('',(-1.,0.,0.));
#39751=DIRECTION('',(1.,0.,0.));
#39752=DIRECTION('center_axis',(-0.70710678118655,-0.664463024388673,0.241844762647975));
#39753=DIRECTION('ref_axis',(0.323615577118183,0.,0.946188648339466));
#39754=DIRECTION('',(0.,0.342020143325669,0.939692620785908));
#39755=DIRECTION('',(0.,-0.342020143325669,-0.939692620785908));
#39756=DIRECTION('center_axis',(0.,-0.467240138462762,0.884130450221741));
#39757=DIRECTION('ref_axis',(1.,0.,0.));
#39758=DIRECTION('',(-1.,0.,0.));
#39759=DIRECTION('',(1.,0.,0.));
#39760=DIRECTION('center_axis',(0.707106781186549,-0.306761075170856,-0.637100967476913));
#39761=DIRECTION('ref_axis',(-0.669373784875799,0.,-0.742925794491649));
#39762=DIRECTION('',(0.,-0.900996828806872,0.433825672914778));
#39763=DIRECTION('',(0.,0.900996828806872,-0.433825672914778));
#39764=DIRECTION('center_axis',(0.707106781186551,-0.664463024388671,0.241844762647974));
#39765=DIRECTION('ref_axis',(0.323615577118182,0.,-0.946188648339466));
#39766=DIRECTION('',(0.,0.342020143325669,0.939692620785908));
#39767=DIRECTION('',(0.,-0.342020143325669,-0.939692620785908));
#39768=DIRECTION('center_axis',(0.70710678118654,0.174527991013631,0.68522987409537));
#39769=DIRECTION('ref_axis',(0.695910561235551,0.,-0.718128463967847));
#39770=DIRECTION('',(0.,-0.96906138128887,0.246819851905204));
#39771=DIRECTION('',(0.,0.96906138128887,-0.246819851905204));
#39772=DIRECTION('center_axis',(1.,0.,0.));
#39773=DIRECTION('ref_axis',(0.,0.939692620785908,-0.342020143325669));
#39774=DIRECTION('center_axis',(0.,0.246819851905204,0.96906138128887));
#39775=DIRECTION('ref_axis',(0.,-0.96906138128887,0.246819851905204));
#39776=DIRECTION('center_axis',(0.,-0.939692620785908,0.342020143325669));
#39777=DIRECTION('ref_axis',(0.,-0.342020143325669,-0.939692620785908));
#39778=DIRECTION('center_axis',(0.707106781186548,0.114142140686716,0.697833484234924));
#39779=DIRECTION('ref_axis',(0.702424227635742,0.,-0.711758529580314));
#39780=DIRECTION('',(0.595596683047422,0.43579678841082,-0.674793116705946));
#39781=DIRECTION('',(0.,0.986885577683101,-0.161421363397451));
#39782=DIRECTION('',(0.,-0.986885577683101,0.161421363397451));
#39783=DIRECTION('',(0.557191914001245,-0.697558392670361,-0.450499122958937));
#39784=DIRECTION('center_axis',(1.,0.,0.));
#39785=DIRECTION('ref_axis',(0.,0.965925826289068,-0.258819045102521));
#39786=DIRECTION('',(0.,0.258819045102521,0.965925826289068));
#39787=DIRECTION('',(0.,-0.935378662600772,0.353647787425838));
#39788=DIRECTION('center_axis',(0.707106781186552,-0.683012701892215,0.183012701892218));
#39789=DIRECTION('ref_axis',(0.250562807085728,0.,-0.968100345886376));
#39790=DIRECTION('',(0.557191914001229,0.69755839267037,0.450499122958943));
#39791=DIRECTION('',(0.,-0.258819045102521,-0.965925826289068));
#39792=DIRECTION('',(0.705516335778306,0.664127077314135,-0.2473498031698));
#39793=DIRECTION('center_axis',(0.,-0.542519194747167,0.840043405623117));
#39794=DIRECTION('ref_axis',(1.,0.,0.));
#39795=DIRECTION('',(-1.,0.,0.));
#39796=DIRECTION('',(0.,-0.840043405623117,-0.542519194747167));
#39797=DIRECTION('',(1.,0.,0.));
#39798=DIRECTION('center_axis',(0.561006631580396,-0.736633774843142,-0.37768007768899));
#39799=DIRECTION('ref_axis',(-0.558457227212258,0.,-0.829533317820566));
#39800=DIRECTION('',(0.,-0.456239332177649,0.889857107503274));
#39801=DIRECTION('',(-0.705516335778303,-0.186803215041171,-0.683630937568099));
#39802=DIRECTION('center_axis',(-0.561006631580404,-0.4491035234553,0.695397429203505));
#39803=DIRECTION('ref_axis',(0.778302413620333,0.,0.627889602520032));
#39804=DIRECTION('',(0.705516335778306,0.180039139049759,0.685443366267538));
#39805=DIRECTION('',(-0.705516335778306,0.69882582188005,-0.117852325490948));
#39806=DIRECTION('center_axis',(-0.707106781186546,0.114142140686716,0.697833484234925));
#39807=DIRECTION('ref_axis',(0.702424227635744,0.,0.711758529580313));
#39808=DIRECTION('',(0.,-0.986885577683101,0.161421363397451));
#39809=DIRECTION('',(0.,0.986885577683101,-0.161421363397451));
#39810=DIRECTION('center_axis',(-0.561006631580394,-0.736633774843143,-0.37768007768899));
#39811=DIRECTION('ref_axis',(-0.55845722721226,0.,0.829533317820565));
#39812=DIRECTION('',(0.705516335778307,-0.664127077314133,0.247349803169799));
#39813=DIRECTION('',(-0.705516335778305,0.18680321504117,0.683630937568098));
#39814=DIRECTION('',(0.,0.456239332177649,-0.889857107503274));
#39815=DIRECTION('center_axis',(-0.707106781186544,-0.25006674864043,-0.661412595302213));
#39816=DIRECTION('ref_axis',(-0.683116152038589,0.,0.730309744439982));
#39817=DIRECTION('',(0.,-0.935378662600772,0.353647787425838));
#39818=DIRECTION('',(0.,0.935378662600772,-0.353647787425838));
#39819=DIRECTION('center_axis',(0.,-0.889857107503274,-0.456239332177649));
#39820=DIRECTION('ref_axis',(0.,0.456239332177649,-0.889857107503274));
#39821=DIRECTION('',(-1.,0.,0.));
#39822=DIRECTION('',(1.,0.,0.));
#39823=DIRECTION('center_axis',(-0.707106781186551,-0.683012701892216,0.183012701892218));
#39824=DIRECTION('ref_axis',(0.250562807085729,0.,0.968100345886375));
#39825=DIRECTION('',(0.,0.258819045102521,0.965925826289068));
#39826=DIRECTION('',(0.,-0.258819045102521,-0.965925826289068));
#39827=DIRECTION('center_axis',(0.707106781186545,-0.25006674864043,-0.661412595302212));
#39828=DIRECTION('ref_axis',(-0.683116152038587,0.,-0.730309744439983));
#39829=DIRECTION('',(0.,0.935378662600772,-0.353647787425838));
#39830=DIRECTION('center_axis',(0.,0.161421363397451,0.986885577683101));
#39831=DIRECTION('ref_axis',(0.,-0.986885577683101,0.161421363397451));
#39832=DIRECTION('center_axis',(0.,-0.965925826289068,0.258819045102521));
#39833=DIRECTION('ref_axis',(0.,-0.258819045102521,-0.965925826289068));
#39834=DIRECTION('center_axis',(0.561006631580396,-0.508002428407528,0.653609280881837));
#39835=DIRECTION('ref_axis',(0.758814655754537,0.,-0.651306623804889));
#39836=DIRECTION('',(0.705516335778306,-0.119613710071895,-0.698526492205406));
#39837=DIRECTION('',(0.,0.789563123475645,0.613669352377469));
#39838=DIRECTION('',(-0.70551633577831,-0.706438085609211,0.0564971782546713));
#39839=DIRECTION('center_axis',(0.56100663158039,-0.700913673242072,-0.44044475474812));
#39840=DIRECTION('ref_axis',(-0.617521420133027,0.,-0.786554064052109));
#39841=DIRECTION('',(0.70551633577831,0.683157829093258,-0.188526073789633));
#39842=DIRECTION('',(0.,-0.532059360920026,0.846707054687377));
#39843=DIRECTION('',(-0.705516335778307,-0.126510010281474,-0.697310488411391));
#39844=DIRECTION('center_axis',(-0.561006631580394,-0.508002428407529,0.653609280881838));
#39845=DIRECTION('ref_axis',(0.758814655754539,0.,0.651306623804887));
#39846=DIRECTION('',(0.,-0.789563123475645,-0.613669352377469));
#39847=DIRECTION('',(0.705516335778308,0.119613710071895,0.698526492205404));
#39848=DIRECTION('',(-0.705516335778312,0.70643808560921,-0.0564971782546712));
#39849=DIRECTION('center_axis',(-0.707106781186545,0.0528875997482675,0.705126160196082));
#39850=DIRECTION('ref_axis',(0.706114387365564,0.,0.708097784176278));
#39851=DIRECTION('',(0.,-0.997198978933359,0.0747943608453595));
#39852=DIRECTION('',(0.,0.997198978933359,-0.0747943608453595));
#39853=DIRECTION('center_axis',(-0.561006631580388,-0.700913673242073,-0.44044475474812));
#39854=DIRECTION('ref_axis',(-0.617521420133029,0.,0.786554064052108));
#39855=DIRECTION('',(0.705516335778312,-0.683157829093257,0.188526073789632));
#39856=DIRECTION('',(-0.705516335778309,0.126510010281474,0.697310488411389));
#39857=DIRECTION('',(0.,0.532059360920026,-0.846707054687377));
#39858=DIRECTION('center_axis',(-0.707106781186544,-0.191469263158417,-0.680690473905414));
#39859=DIRECTION('ref_axis',(-0.693521587324702,0.,0.720435845800739));
#39860=DIRECTION('',(0.,-0.962641699975202,0.270778428736215));
#39861=DIRECTION('',(0.,0.962641699975202,-0.270778428736215));
#39862=DIRECTION('center_axis',(0.,-0.846707054687377,-0.532059360920026));
#39863=DIRECTION('ref_axis',(-1.,0.,0.));
#39864=DIRECTION('',(-1.,0.,0.));
#39865=DIRECTION('',(1.,0.,0.));
#39866=DIRECTION('center_axis',(-0.707106781186541,-0.696364240320026,0.122787803968974));
#39867=DIRECTION('ref_axis',(0.171087869746039,0.,0.985255774317391));
#39868=DIRECTION('',(0.,0.17364817766693,0.984807753012208));
#39869=DIRECTION('',(0.,-0.17364817766693,-0.984807753012208));
#39870=DIRECTION('center_axis',(0.,-0.61366935237747,0.789563123475645));
#39871=DIRECTION('ref_axis',(1.,0.,0.));
#39872=DIRECTION('',(-1.,0.,0.));
#39873=DIRECTION('',(1.,0.,0.));
#39874=DIRECTION('center_axis',(0.707106781186546,-0.191469263158417,-0.680690473905413));
#39875=DIRECTION('ref_axis',(-0.6935215873247,0.,-0.72043584580074));
#39876=DIRECTION('',(0.,-0.962641699975202,0.270778428736215));
#39877=DIRECTION('',(0.,0.962641699975202,-0.270778428736215));
#39878=DIRECTION('center_axis',(0.707106781186543,-0.696364240320024,0.122787803968974));
#39879=DIRECTION('ref_axis',(0.171087869746038,0.,-0.985255774317391));
#39880=DIRECTION('',(0.,0.17364817766693,0.984807753012208));
#39881=DIRECTION('',(0.,-0.17364817766693,-0.984807753012208));
#39882=DIRECTION('center_axis',(0.707106781186546,0.0528875997482674,0.705126160196081));
#39883=DIRECTION('ref_axis',(0.706114387365562,0.,-0.708097784176279));
#39884=DIRECTION('',(0.,-0.997198978933359,0.0747943608453595));
#39885=DIRECTION('',(0.,0.997198978933359,-0.0747943608453595));
#39886=DIRECTION('center_axis',(1.,0.,0.));
#39887=DIRECTION('ref_axis',(0.,0.984807753012208,-0.17364817766693));
#39888=DIRECTION('center_axis',(0.,0.0747943608453595,0.997198978933359));
#39889=DIRECTION('ref_axis',(0.,-0.997198978933359,0.0747943608453595));
#39890=DIRECTION('center_axis',(0.,-0.984807753012208,0.17364817766693));
#39891=DIRECTION('ref_axis',(0.,-0.17364817766693,-0.984807753012208));
#39892=DIRECTION('center_axis',(0.561006631580394,-0.659859195364386,-0.499857381275785));
#39893=DIRECTION('ref_axis',(-0.665244232298936,0.,-0.746625817523744));
#39894=DIRECTION('',(0.705516335778315,0.696989337290999,-0.128267547152788));
#39895=DIRECTION('',(0.,-0.603830096659559,0.797113049929624));
#39896=DIRECTION('',(-0.705516335778306,-0.0652539879547271,-0.705683085390288));
#39897=DIRECTION('center_axis',(0.,-0.797113049929624,-0.603830096659559));
#39898=DIRECTION('ref_axis',(-1.,0.,0.));
#39899=DIRECTION('',(0.557191914001245,0.501410699557118,-0.661909722954173));
#39900=DIRECTION('',(1.,0.,0.));
#39901=DIRECTION('',(-1.,0.,0.));
#39902=DIRECTION('',(-0.557191914001234,0.501410699557122,-0.66190972295418));
#39903=DIRECTION('center_axis',(0.707106781186545,-0.131414580971466,-0.694787886990049));
#39904=DIRECTION('ref_axis',(-0.700866150214856,0.,-0.713292814686232));
#39905=DIRECTION('',(0.,-0.982578452753869,0.185848282703424));
#39906=DIRECTION('',(0.,0.982578452753869,-0.185848282703424));
#39907=DIRECTION('center_axis',(0.561006631580395,-0.563035128139337,0.606846771272568));
#39908=DIRECTION('ref_axis',(0.734296425103064,0.,-0.678828962317357));
#39909=DIRECTION('',(0.705516335778303,-0.0582779485356275,-0.706293409755772));
#39910=DIRECTION('',(0.,0.733073789207257,0.680149115692518));
#39911=DIRECTION('',(-0.705516335778312,-0.708673928947909,-0.00528794662206119));
#39912=DIRECTION('center_axis',(0.,-0.680149115692518,0.733073789207257));
#39913=DIRECTION('ref_axis',(1.,0.,0.));
#39914=DIRECTION('',(0.557191914001236,-0.608732561538147,-0.564784772718639));
#39915=DIRECTION('',(1.,0.,0.));
#39916=DIRECTION('',(-1.,0.,0.));
#39917=DIRECTION('',(-0.55719191400124,-0.608732561538145,-0.564784772718638));
#39918=DIRECTION('center_axis',(0.707106781186545,-0.704416026402761,0.0616284167162197));
#39919=DIRECTION('ref_axis',(0.0868265938642484,0.,-0.996223440096615));
#39920=DIRECTION('',(0.,0.0871557427476584,0.996194698091746));
#39921=DIRECTION('',(0.,-0.0871557427476584,-0.996194698091746));
#39922=DIRECTION('center_axis',(0.707106781186549,-0.00876944775867117,
0.707052400311324));
#39923=DIRECTION('ref_axis',(0.70707958918054,0.,-0.707133972146918));
#39924=DIRECTION('',(0.,-0.999923093828728,-0.0124018719548351));
#39925=DIRECTION('',(0.,0.999923093828728,0.0124018719548351));
#39926=DIRECTION('center_axis',(-0.707106781186545,-0.131414580971466,-0.694787886990049));
#39927=DIRECTION('ref_axis',(-0.700866150214856,0.,0.713292814686232));
#39928=DIRECTION('',(-0.59559668304743,0.640307864722775,0.485046832292573));
#39929=DIRECTION('',(0.,0.982578452753869,-0.185848282703424));
#39930=DIRECTION('',(0.,-0.982578452753869,0.185848282703424));
#39931=DIRECTION('center_axis',(0.,-0.996194698091746,0.0871557427476584));
#39932=DIRECTION('ref_axis',(0.,-0.0871557427476584,-0.996194698091746));
#39933=DIRECTION('',(0.,0.0871557427476584,0.996194698091746));
#39934=DIRECTION('center_axis',(-0.707106781186556,-0.70441602640275,0.0616284167162188));
#39935=DIRECTION('ref_axis',(0.0868265938642457,0.,0.996223440096615));
#39936=DIRECTION('',(0.595596683047425,-0.546352650982967,0.588866174870648));
#39937=DIRECTION('',(0.,-0.0871557427476584,-0.996194698091746));
#39938=DIRECTION('center_axis',(-0.707106781186548,-0.00876944775867119,
0.707052400311326));
#39939=DIRECTION('ref_axis',(0.707079589180542,0.,0.707133972146916));
#39940=DIRECTION('',(0.,0.999923093828728,0.0124018719548351));
#39941=DIRECTION('',(0.,-0.999923093828728,-0.0124018719548351));
#39942=DIRECTION('center_axis',(0.,-0.0124018719548351,0.999923093828728));
#39943=DIRECTION('ref_axis',(0.,-0.999923093828728,-0.0124018719548351));
#39944=DIRECTION('center_axis',(0.,-0.185848282703424,-0.982578452753869));
#39945=DIRECTION('ref_axis',(0.,0.982578452753869,-0.185848282703424));
#39946=DIRECTION('center_axis',(0.561006631580415,-0.613782790576089,0.555465791309803));
#39947=DIRECTION('ref_axis',(0.703588880269149,0.,-0.710607266752603));
#39948=DIRECTION('',(0.705516335778305,0.00350134337823142,-0.708685007986272));
#39949=DIRECTION('',(0.,0.671005320760942,0.741452533551882));
#39950=DIRECTION('',(-0.705516335778299,-0.705516335778311,-0.067032827032045));
#39951=DIRECTION('center_axis',(0.561006631580416,-0.613782790576088,-0.555465791309803));
#39952=DIRECTION('ref_axis',(-0.703588880269148,0.,-0.710607266752604));
#39953=DIRECTION('',(0.705516335778299,0.705516335778311,-0.0670328270320441));
#39954=DIRECTION('',(0.,-0.671005320760943,0.741452533551882));
#39955=DIRECTION('',(-0.705516335778305,-0.00350134337823142,-0.708685007986272));
#39956=DIRECTION('center_axis',(-0.561006631580427,-0.613782790576083,0.555465791309797));
#39957=DIRECTION('ref_axis',(0.703588880269137,0.,0.710607266752615));
#39958=DIRECTION('',(0.,-0.671005320760942,-0.741452533551882));
#39959=DIRECTION('',(0.705516335778308,-0.00350134337825648,0.708685007986269));
#39960=DIRECTION('',(-0.705516335778288,0.705516335778322,0.0670328270320461));
#39961=DIRECTION('center_axis',(-0.707106781186547,-0.0703597544730291,
0.703597544730292));
#39962=DIRECTION('ref_axis',(0.705345615858599,0.,0.708863570928182));
#39963=DIRECTION('',(0.,-0.995037190209989,-0.0995037190209987));
#39964=DIRECTION('',(0.,0.995037190209989,0.0995037190209987));
#39965=DIRECTION('center_axis',(-0.561006631580428,-0.613782790576082,-0.555465791309797));
#39966=DIRECTION('ref_axis',(-0.703588880269137,0.,0.710607266752615));
#39967=DIRECTION('',(0.705516335778288,-0.705516335778322,0.0670328270320439));
#39968=DIRECTION('',(-0.705516335778307,0.00350134337825647,0.708685007986269));
#39969=DIRECTION('',(0.,0.671005320760943,-0.741452533551882));
#39970=DIRECTION('center_axis',(-0.707106781186548,-0.0703597544730291,
-0.703597544730292));
#39971=DIRECTION('ref_axis',(-0.705345615858598,0.,0.708863570928183));
#39972=DIRECTION('',(0.,-0.995037190209989,0.0995037190209988));
#39973=DIRECTION('',(0.,0.995037190209989,-0.0995037190209988));
#39974=DIRECTION('center_axis',(0.,-0.741452533551882,-0.671005320760943));
#39975=DIRECTION('ref_axis',(-1.,0.,0.));
#39976=DIRECTION('',(-1.,0.,0.));
#39977=DIRECTION('',(1.,0.,0.));
#39978=DIRECTION('center_axis',(-0.707106781186565,-0.70710678118653,4.32978028117736E-17));
#39979=DIRECTION('ref_axis',(6.12323399573647E-17,0.,1.));
#39980=DIRECTION('',(0.,6.12323399573677E-17,1.));
#39981=DIRECTION('',(0.,-6.12323399573677E-17,-1.));
#39982=DIRECTION('center_axis',(0.,-0.741452533551882,0.671005320760942));
#39983=DIRECTION('ref_axis',(1.,0.,0.));
#39984=DIRECTION('',(-1.,0.,0.));
#39985=DIRECTION('',(1.,0.,0.));
#39986=DIRECTION('center_axis',(0.707106781186548,-0.070359754473029,-0.703597544730291));
#39987=DIRECTION('ref_axis',(-0.705345615858597,0.,-0.708863570928184));
#39988=DIRECTION('',(0.,-0.995037190209989,0.0995037190209988));
#39989=DIRECTION('',(0.,0.995037190209989,-0.0995037190209988));
#39990=DIRECTION('center_axis',(0.707106781186554,-0.707106781186541,4.32978028117743E-17));
#39991=DIRECTION('ref_axis',(6.12323399573666E-17,0.,-1.));
#39992=DIRECTION('',(0.,6.12323399573677E-17,1.));
#39993=DIRECTION('',(0.,-6.12323399573677E-17,-1.));
#39994=DIRECTION('center_axis',(0.707106781186548,-0.070359754473029,0.703597544730291));
#39995=DIRECTION('ref_axis',(0.705345615858597,0.,-0.708863570928184));
#39996=DIRECTION('',(0.,-0.995037190209989,-0.0995037190209987));
#39997=DIRECTION('',(0.,0.995037190209989,0.0995037190209987));
#39998=DIRECTION('center_axis',(1.,0.,0.));
#39999=DIRECTION('ref_axis',(0.,1.,-6.12323399573677E-17));
#40000=DIRECTION('center_axis',(0.,-0.0995037190209987,0.995037190209989));
#40001=DIRECTION('ref_axis',(0.,-0.995037190209989,-0.0995037190209987));
#40002=DIRECTION('center_axis',(0.,-1.,6.12323399573677E-17));
#40003=DIRECTION('ref_axis',(0.,-6.12323399573677E-17,-1.));
#40004=DIRECTION('center_axis',(0.56100663158041,-0.65985919536438,0.499857381275775));
#40005=DIRECTION('ref_axis',(0.665244232298917,0.,-0.746625817523761));
#40006=DIRECTION('',(0.705516335778303,0.0652539879547519,-0.705683085390289));
#40007=DIRECTION('',(0.,0.603830096659555,0.797113049929628));
#40008=DIRECTION('',(-0.705516335778303,-0.696989337291012,-0.128267547152789));
#40009=DIRECTION('center_axis',(0.56100663158041,-0.56303512813933,-0.60684677127256));
#40010=DIRECTION('ref_axis',(-0.734296425103051,0.,-0.678828962317372));
#40011=DIRECTION('',(0.7055163357783,0.708673928947921,-0.00528794662205797));
#40012=DIRECTION('',(0.,-0.733073789207257,0.680149115692518));
#40013=DIRECTION('',(-0.705516335778302,0.0582779485356024,-0.706293409755775));
#40014=DIRECTION('center_axis',(-0.561006631580394,-0.659859195364389,0.499857381275781));
#40015=DIRECTION('ref_axis',(0.665244232298933,0.,0.746625817523747));
#40016=DIRECTION('',(0.,-0.603830096659555,-0.797113049929628));
#40017=DIRECTION('',(0.705516335778303,-0.0652539879547265,0.705683085390291));
#40018=DIRECTION('',(-0.705516335778317,0.696989337290998,0.128267547152788));
#40019=DIRECTION('center_axis',(-0.707106781186548,-0.131414580971466,0.694787886990046));
#40020=DIRECTION('ref_axis',(0.700866150214853,0.,0.713292814686235));
#40021=DIRECTION('',(0.,-0.98257845275387,-0.185848282703424));
#40022=DIRECTION('',(0.,0.98257845275387,0.185848282703424));
#40023=DIRECTION('center_axis',(-0.561006631580395,-0.563035128139337,-0.606846771272568));
#40024=DIRECTION('ref_axis',(-0.734296425103064,0.,0.678828962317357));
#40025=DIRECTION('',(0.705516335778314,-0.708673928947907,0.00528794662205805));
#40026=DIRECTION('',(-0.705516335778303,-0.0582779485356272,0.706293409755772));
#40027=DIRECTION('',(0.,0.733073789207257,-0.680149115692518));
#40028=DIRECTION('center_axis',(-0.707106781186548,-0.00876944775867143,
-0.707052400311326));
#40029=DIRECTION('ref_axis',(-0.707079589180542,0.,0.707133972146916));
#40030=DIRECTION('',(0.,-0.999923093828728,0.0124018719548355));
#40031=DIRECTION('',(0.,0.999923093828728,-0.0124018719548355));
#40032=DIRECTION('center_axis',(0.,-0.680149115692518,-0.733073789207257));
#40033=DIRECTION('ref_axis',(-1.,0.,0.));
#40034=DIRECTION('',(-1.,0.,0.));
#40035=DIRECTION('',(1.,0.,0.));
#40036=DIRECTION('center_axis',(-0.707106781186531,-0.704416026402775,-0.0616284167162207));
#40037=DIRECTION('ref_axis',(-0.0868265938642515,0.,0.996223440096614));
#40038=DIRECTION('',(0.,-0.087155742747658,0.996194698091746));
#40039=DIRECTION('',(0.,0.087155742747658,-0.996194698091746));
#40040=DIRECTION('center_axis',(0.,-0.797113049929628,0.603830096659555));
#40041=DIRECTION('ref_axis',(1.,0.,0.));
#40042=DIRECTION('',(-1.,0.,0.));
#40043=DIRECTION('',(1.,0.,0.));
#40044=DIRECTION('center_axis',(0.707106781186549,-0.00876944775867141,
-0.707052400311324));
#40045=DIRECTION('ref_axis',(-0.70707958918054,0.,-0.707133972146918));
#40046=DIRECTION('',(0.,-0.999923093828728,0.0124018719548355));
#40047=DIRECTION('',(0.,0.999923093828728,-0.0124018719548355));
#40048=DIRECTION('center_axis',(0.707106781186545,-0.704416026402761,-0.0616284167162195));
#40049=DIRECTION('ref_axis',(-0.0868265938642481,0.,-0.996223440096615));
#40050=DIRECTION('',(0.,-0.087155742747658,0.996194698091746));
#40051=DIRECTION('',(0.,0.087155742747658,-0.996194698091746));
#40052=DIRECTION('center_axis',(0.707106781186549,-0.131414580971465,0.694787886990045));
#40053=DIRECTION('ref_axis',(0.700866150214851,0.,-0.713292814686237));
#40054=DIRECTION('',(0.,-0.98257845275387,-0.185848282703424));
#40055=DIRECTION('',(0.,0.98257845275387,0.185848282703424));
#40056=DIRECTION('center_axis',(1.,0.,0.));
#40057=DIRECTION('ref_axis',(0.,0.996194698091746,0.087155742747658));
#40058=DIRECTION('center_axis',(0.,-0.185848282703424,0.98257845275387));
#40059=DIRECTION('ref_axis',(0.,-0.98257845275387,-0.185848282703424));
#40060=DIRECTION('center_axis',(0.,-0.996194698091746,-0.087155742747658));
#40061=DIRECTION('ref_axis',(0.,0.087155742747658,-0.996194698091746));
#40062=DIRECTION('center_axis',(0.707106781186546,-0.191469263158417,0.680690473905413));
#40063=DIRECTION('ref_axis',(0.6935215873247,0.,-0.72043584580074));
#40064=DIRECTION('',(0.595596683047428,0.680145916919136,-0.427394575118975));
#40065=DIRECTION('',(0.,0.962641699975202,0.270778428736215));
#40066=DIRECTION('',(0.,-0.962641699975202,-0.270778428736215));
#40067=DIRECTION('',(0.557191914001241,-0.441813446929312,-0.703091778563846));
#40068=DIRECTION('center_axis',(1.,0.,0.));
#40069=DIRECTION('ref_axis',(0.,0.984807753012208,0.17364817766693));
#40070=DIRECTION('',(0.,-0.17364817766693,0.984807753012208));
#40071=DIRECTION('',(0.,-0.997198978933359,-0.0747943608453594));
#40072=DIRECTION('center_axis',(0.707106781186543,-0.696364240320023,-0.122787803968974));
#40073=DIRECTION('ref_axis',(-0.171087869746038,0.,-0.985255774317392));
#40074=DIRECTION('',(0.557191914001248,0.44181344692931,0.703091778563843));
#40075=DIRECTION('',(0.,0.17364817766693,-0.984807753012208));
#40076=DIRECTION('',(0.70551633577831,0.706438085609211,0.0564971782546651));
#40077=DIRECTION('center_axis',(0.,-0.846707054687383,0.532059360920017));
#40078=DIRECTION('ref_axis',(1.,0.,0.));
#40079=DIRECTION('',(-1.,0.,0.));
#40080=DIRECTION('',(0.,-0.532059360920017,-0.846707054687383));
#40081=DIRECTION('',(1.,0.,0.));
#40082=DIRECTION('center_axis',(0.5610066315804,-0.508002428407545,-0.65360928088182));
#40083=DIRECTION('ref_axis',(-0.758814655754527,0.,-0.651306623804901));
#40084=DIRECTION('',(0.,-0.789563123475628,0.613669352377492));
#40085=DIRECTION('',(-0.705516335778305,0.11961371007187,-0.698526492205411));
#40086=DIRECTION('center_axis',(-0.561006631580394,-0.700913673242075,0.440444754748109));
#40087=DIRECTION('ref_axis',(0.617521420133015,0.,0.786554064052119));
#40088=DIRECTION('',(0.705516335778313,-0.1265100102815,0.697310488411381));
#40089=DIRECTION('',(-0.70551633577831,0.683157829093255,0.188526073789644));
#40090=DIRECTION('center_axis',(-0.707106781186538,-0.191469263158419,0.68069047390542));
#40091=DIRECTION('ref_axis',(0.693521587324708,0.,0.720435845800733));
#40092=DIRECTION('',(0.,-0.962641699975202,-0.270778428736215));
#40093=DIRECTION('',(0.,0.962641699975202,0.270778428736215));
#40094=DIRECTION('center_axis',(-0.561006631580398,-0.508002428407546,-0.653609280881821));
#40095=DIRECTION('ref_axis',(-0.758814655754528,0.,0.651306623804899));
#40096=DIRECTION('',(0.705516335778312,-0.70643808560921,-0.056497178254665));
#40097=DIRECTION('',(-0.705516335778307,-0.119613710071869,0.69852649220541));
#40098=DIRECTION('',(0.,0.789563123475628,-0.613669352377492));
#40099=DIRECTION('center_axis',(-0.707106781186548,0.0528875997482672,-0.705126160196079));
#40100=DIRECTION('ref_axis',(-0.706114387365561,0.,0.708097784176281));
#40101=DIRECTION('',(0.,-0.997198978933359,-0.0747943608453594));
#40102=DIRECTION('',(0.,0.997198978933359,0.0747943608453594));
#40103=DIRECTION('center_axis',(0.,-0.613669352377492,-0.789563123475628));
#40104=DIRECTION('ref_axis',(-1.,0.,0.));
#40105=DIRECTION('',(-1.,0.,0.));
#40106=DIRECTION('',(1.,0.,0.));
#40107=DIRECTION('center_axis',(-0.707106781186541,-0.696364240320025,-0.122787803968974));
#40108=DIRECTION('ref_axis',(-0.171087869746038,0.,0.985255774317391));
#40109=DIRECTION('',(0.,-0.17364817766693,0.984807753012208));
#40110=DIRECTION('',(0.,0.17364817766693,-0.984807753012208));
#40111=DIRECTION('center_axis',(0.707106781186549,0.0528875997482671,-0.705126160196077));
#40112=DIRECTION('ref_axis',(-0.706114387365559,0.,-0.708097784176282));
#40113=DIRECTION('',(0.,0.997198978933359,0.0747943608453594));
#40114=DIRECTION('center_axis',(0.,-0.270778428736215,0.962641699975202));
#40115=DIRECTION('ref_axis',(0.,-0.962641699975202,-0.270778428736215));
#40116=DIRECTION('center_axis',(0.,-0.984807753012208,-0.17364817766693));
#40117=DIRECTION('ref_axis',(0.,0.17364817766693,-0.984807753012208));
#40118=DIRECTION('center_axis',(0.561006631580395,-0.736633774843153,0.37768007768897));
#40119=DIRECTION('ref_axis',(0.558457227212238,0.,-0.829533317820579));
#40120=DIRECTION('',(0.705516335778309,0.186803215041197,-0.683630937568086));
#40121=DIRECTION('',(0.,0.456239332177625,0.889857107503286));
#40122=DIRECTION('',(-0.705516335778301,-0.664127077314131,-0.247349803169823));
#40123=DIRECTION('center_axis',(0.56100663158042,-0.449103523455307,-0.695397429203488));
#40124=DIRECTION('ref_axis',(-0.778302413620316,0.,-0.627889602520053));
#40125=DIRECTION('',(0.705516335778293,0.698825821880065,0.11785232549094));
#40126=DIRECTION('',(0.,-0.84004340562311,0.542519194747178));
#40127=DIRECTION('',(-0.705516335778311,0.180039139049711,-0.685443366267545));
#40128=DIRECTION('center_axis',(-0.561006631580394,-0.736633774843153,0.37768007768897));
#40129=DIRECTION('ref_axis',(0.55845722721224,0.,0.829533317820578));
#40130=DIRECTION('',(0.,-0.456239332177625,-0.889857107503286));
#40131=DIRECTION('',(0.705516335778311,-0.186803215041197,0.683630937568085));
#40132=DIRECTION('',(-0.705516335778303,0.664127077314129,0.247349803169823));
#40133=DIRECTION('center_axis',(-0.707106781186544,-0.25006674864043,0.661412595302213));
#40134=DIRECTION('ref_axis',(0.683116152038589,0.,0.730309744439982));
#40135=DIRECTION('',(0.,-0.935378662600772,-0.353647787425838));
#40136=DIRECTION('',(0.,0.935378662600772,0.353647787425838));
#40137=DIRECTION('center_axis',(-0.561006631580427,-0.449103523455304,-0.695397429203484));
#40138=DIRECTION('ref_axis',(-0.778302413620311,0.,0.627889602520059));
#40139=DIRECTION('',(0.705516335778293,-0.698825821880063,-0.117852325490952));
#40140=DIRECTION('',(-0.705516335778306,-0.180039139049709,0.68544336626755));
#40141=DIRECTION('',(0.,0.84004340562311,-0.542519194747178));
#40142=DIRECTION('center_axis',(-0.70710678118655,0.114142140686715,-0.697833484234922));
#40143=DIRECTION('ref_axis',(-0.702424227635741,0.,0.711758529580316));
#40144=DIRECTION('',(0.,-0.986885577683101,-0.161421363397451));
#40145=DIRECTION('',(0.,0.986885577683101,0.161421363397451));
#40146=DIRECTION('center_axis',(0.,-0.542519194747178,-0.84004340562311));
#40147=DIRECTION('ref_axis',(-1.,0.,0.));
#40148=DIRECTION('',(-1.,0.,0.));
#40149=DIRECTION('',(1.,0.,0.));
#40150=DIRECTION('center_axis',(-0.707106781186552,-0.683012701892215,-0.183012701892218));
#40151=DIRECTION('ref_axis',(-0.250562807085729,0.,0.968100345886376));
#40152=DIRECTION('',(0.,-0.258819045102521,0.965925826289068));
#40153=DIRECTION('',(0.,0.258819045102521,-0.965925826289068));
#40154=DIRECTION('center_axis',(0.,-0.889857107503286,0.456239332177625));
#40155=DIRECTION('ref_axis',(0.,-0.456239332177625,-0.889857107503286));
#40156=DIRECTION('',(-1.,0.,0.));
#40157=DIRECTION('',(1.,0.,0.));
#40158=DIRECTION('center_axis',(0.707106781186545,0.114142140686716,-0.697833484234927));
#40159=DIRECTION('ref_axis',(-0.702424227635745,0.,-0.711758529580311));
#40160=DIRECTION('',(0.,-0.986885577683101,-0.161421363397451));
#40161=DIRECTION('',(0.,0.986885577683101,0.161421363397451));
#40162=DIRECTION('center_axis',(0.707106781186553,-0.683012701892214,-0.183012701892218));
#40163=DIRECTION('ref_axis',(-0.250562807085728,0.,-0.968100345886376));
#40164=DIRECTION('',(0.,-0.258819045102521,0.965925826289068));
#40165=DIRECTION('',(0.,0.258819045102521,-0.965925826289068));
#40166=DIRECTION('center_axis',(0.707106781186545,-0.25006674864043,0.661412595302212));
#40167=DIRECTION('ref_axis',(0.683116152038587,0.,-0.730309744439983));
#40168=DIRECTION('',(0.,-0.935378662600772,-0.353647787425838));
#40169=DIRECTION('',(0.,0.935378662600772,0.353647787425838));
#40170=DIRECTION('center_axis',(1.,0.,0.));
#40171=DIRECTION('ref_axis',(0.,0.965925826289068,0.258819045102521));
#40172=DIRECTION('center_axis',(0.,-0.353647787425838,0.935378662600772));
#40173=DIRECTION('ref_axis',(0.,-0.935378662600772,-0.353647787425838));
#40174=DIRECTION('center_axis',(0.,-0.965925826289068,-0.258819045102521));
#40175=DIRECTION('ref_axis',(0.,0.258819045102521,-0.965925826289068));
#40176=DIRECTION('center_axis',(0.561006631580392,-0.386786669513444,-0.73189318319651));
#40177=DIRECTION('ref_axis',(-0.793664727118321,0.,-0.608355406755131));
#40178=DIRECTION('',(0.705516335778307,0.685895071683813,0.178310545369053));
#40179=DIRECTION('',(0.,-0.884130450221741,0.467240138462762));
#40180=DIRECTION('',(-0.705516335778315,0.239094361468882,-0.667143602430337));
#40181=DIRECTION('center_axis',(0.,-0.467240138462762,-0.884130450221741));
#40182=DIRECTION('ref_axis',(-1.,0.,0.));
#40183=DIRECTION('',(0.557191914001248,0.734167558056273,-0.387988617963614));
#40184=DIRECTION('',(1.,0.,0.));
#40185=DIRECTION('',(-1.,0.,0.));
#40186=DIRECTION('',(-0.55719191400126,0.734167558056266,-0.38798861796361));
#40187=DIRECTION('center_axis',(0.707106781186534,0.174527991013633,-0.685229874095376));
#40188=DIRECTION('ref_axis',(-0.695910561235558,0.,-0.718128463967841));
#40189=DIRECTION('',(0.,-0.96906138128887,-0.246819851905204));
#40190=DIRECTION('',(0.,0.96906138128887,0.246819851905204));
#40191=DIRECTION('center_axis',(0.56100663158041,-0.76674764862602,0.312041027189168));
#40192=DIRECTION('ref_axis',(0.486084108127403,0.,-0.873912032086747));
#40193=DIRECTION('',(0.70551633577831,0.245674734539575,-0.664748542502243));
#40194=DIRECTION('',(0.,0.376947046632547,0.926234810420662));
#40195=DIRECTION('',(-0.705516335778298,-0.640041917465765,-0.304291051193938));
#40196=DIRECTION('center_axis',(0.,-0.926234810420662,0.376947046632547));
#40197=DIRECTION('ref_axis',(0.,-0.376947046632547,-0.926234810420662));
#40198=DIRECTION('',(0.557191914001255,-0.313010701840811,-0.769130334536833));
#40199=DIRECTION('',(1.,0.,0.));
#40200=DIRECTION('',(-1.,0.,0.));
#40201=DIRECTION('',(-0.557191914001238,-0.313010701840815,-0.769130334536844));
#40202=DIRECTION('center_axis',(0.707106781186551,-0.664463024388671,-0.241844762647974));
#40203=DIRECTION('ref_axis',(-0.323615577118182,0.,-0.946188648339466));
#40204=DIRECTION('',(0.,-0.342020143325669,0.939692620785908));
#40205=DIRECTION('',(0.,0.342020143325669,-0.939692620785908));
#40206=DIRECTION('center_axis',(0.707106781186549,-0.306761075170856,0.637100967476913));
#40207=DIRECTION('ref_axis',(0.669373784875799,0.,-0.742925794491649));
#40208=DIRECTION('',(0.,-0.900996828806872,-0.433825672914778));
#40209=DIRECTION('',(0.,0.900996828806872,0.433825672914778));
#40210=DIRECTION('center_axis',(-0.707106781186539,0.174527991013631,-0.685229874095371));
#40211=DIRECTION('ref_axis',(-0.695910561235553,0.,0.718128463967846));
#40212=DIRECTION('',(-0.595596683047436,0.375326354772729,0.710207517952259));
#40213=DIRECTION('',(0.,0.96906138128887,0.246819851905204));
#40214=DIRECTION('',(0.,-0.96906138128887,-0.246819851905204));
#40215=DIRECTION('center_axis',(0.,-0.939692620785908,-0.342020143325669));
#40216=DIRECTION('ref_axis',(0.,0.342020143325669,-0.939692620785908));
#40217=DIRECTION('',(0.,-0.342020143325669,0.939692620785908));
#40218=DIRECTION('center_axis',(-0.707106781186536,-0.664463024388686,-0.241844762647979));
#40219=DIRECTION('ref_axis',(-0.323615577118194,0.,0.946188648339462));
#40220=DIRECTION('',(0.595596683047426,-0.744029261275698,0.302795392151933));
#40221=DIRECTION('',(0.,0.342020143325669,-0.939692620785908));
#40222=DIRECTION('center_axis',(-0.707106781186553,-0.306761075170854,0.637100967476909));
#40223=DIRECTION('ref_axis',(0.669373784875795,0.,0.742925794491652));
#40224=DIRECTION('',(0.,0.900996828806872,0.433825672914778));
#40225=DIRECTION('',(0.,-0.900996828806872,-0.433825672914778));
#40226=DIRECTION('center_axis',(0.,-0.433825672914778,0.900996828806872));
#40227=DIRECTION('ref_axis',(0.,-0.900996828806872,-0.433825672914778));
#40228=DIRECTION('center_axis',(0.,0.246819851905204,-0.96906138128887));
#40229=DIRECTION('ref_axis',(0.,0.96906138128887,0.246819851905204));
#40230=DIRECTION('center_axis',(0.561006631580396,-0.791026109827976,0.244027156056938));
#40231=DIRECTION('ref_axis',(0.398879012810069,0.,-0.917003562228449));
#40232=DIRECTION('',(0.705516335778307,0.302676520965598,-0.640807009641837));
#40233=DIRECTION('',(0.,0.294785966455742,0.955563307154871));
#40234=DIRECTION('',(-0.705516335778303,-0.611085652157587,-0.358916460582535));
#40235=DIRECTION('center_axis',(0.561006631580424,-0.321526135468413,-0.76281878813617));
#40236=DIRECTION('ref_axis',(-0.805595332751381,0.,-0.592466167683178));
#40237=DIRECTION('',(0.705516335778303,0.667744245837286,0.237411714330086));
#40238=DIRECTION('',(0.,-0.921488728241605,0.388405102597364));
#40239=DIRECTION('',(-0.705516335778299,0.296329931428078,-0.643766472946357));
#40240=DIRECTION('center_axis',(-0.561006631580408,-0.791026109827968,0.244027156056936));
#40241=DIRECTION('ref_axis',(0.398879012810058,0.,0.917003562228454));
#40242=DIRECTION('',(0.,-0.294785966455742,-0.955563307154871));
#40243=DIRECTION('',(0.705516335778314,-0.302676520965625,0.640807009641816));
#40244=DIRECTION('',(-0.705516335778287,0.611085652157596,0.35891646058255));
#40245=DIRECTION('center_axis',(-0.70710678118654,-0.361120764691837,0.607940616597043));
#40246=DIRECTION('ref_axis',(0.65193371809419,0.,0.758275957163278));
#40247=DIRECTION('',(0.,-0.859757865108992,-0.510701883081733));
#40248=DIRECTION('',(0.,0.859757865108992,0.510701883081733));
#40249=DIRECTION('center_axis',(-0.561006631580422,-0.321526135468414,-0.762818788136171));
#40250=DIRECTION('ref_axis',(-0.805595332751382,0.,0.592466167683177));
#40251=DIRECTION('',(0.705516335778289,-0.667744245837295,-0.237411714330105));
#40252=DIRECTION('',(-0.705516335778301,-0.296329931428077,0.643766472946356));
#40253=DIRECTION('',(0.,0.921488728241605,-0.388405102597364));
#40254=DIRECTION('center_axis',(-0.70710678118655,0.233585577946046,-0.667411250860823));
#40255=DIRECTION('ref_axis',(-0.686399640790371,0.,0.727224541062009));
#40256=DIRECTION('',(0.,-0.943862042647771,-0.330339892306057));
#40257=DIRECTION('',(0.,0.943862042647771,0.330339892306057));
#40258=DIRECTION('center_axis',(0.,-0.388405102597364,-0.921488728241605));
#40259=DIRECTION('ref_axis',(-1.,0.,0.));
#40260=DIRECTION('',(-1.,0.,0.));
#40261=DIRECTION('',(1.,0.,0.));
#40262=DIRECTION('center_axis',(-0.707106781186564,-0.640856382055774,-0.298836238730113));
#40263=DIRECTION('ref_axis',(-0.38928162063501,0.,0.921118787038773));
#40264=DIRECTION('',(0.,-0.422618261740699,0.90630778703665));
#40265=DIRECTION('',(0.,0.422618261740699,-0.90630778703665));
#40266=DIRECTION('center_axis',(0.,-0.955563307154871,0.294785966455742));
#40267=DIRECTION('ref_axis',(0.,-0.294785966455742,-0.955563307154871));
#40268=DIRECTION('',(-1.,0.,0.));
#40269=DIRECTION('',(1.,0.,0.));
#40270=DIRECTION('center_axis',(0.707106781186551,0.233585577946046,-0.667411250860822));
#40271=DIRECTION('ref_axis',(-0.686399640790369,0.,-0.72722454106201));
#40272=DIRECTION('',(0.,-0.943862042647771,-0.330339892306057));
#40273=DIRECTION('',(0.,0.943862042647771,0.330339892306057));
#40274=DIRECTION('center_axis',(0.707106781186551,-0.640856382055785,-0.298836238730118));
#40275=DIRECTION('ref_axis',(-0.389281620635021,0.,-0.921118787038768));
#40276=DIRECTION('',(0.,-0.422618261740699,0.90630778703665));
#40277=DIRECTION('',(0.,0.422618261740699,-0.90630778703665));
#40278=DIRECTION('center_axis',(0.707106781186547,-0.361120764691833,0.607940616597037));
#40279=DIRECTION('ref_axis',(0.651933718094183,0.,-0.758275957163284));
#40280=DIRECTION('',(0.,-0.859757865108992,-0.510701883081733));
#40281=DIRECTION('',(0.,0.859757865108992,0.510701883081733));
#40282=DIRECTION('center_axis',(1.,0.,0.));
#40283=DIRECTION('ref_axis',(0.,0.90630778703665,0.422618261740699));
#40284=DIRECTION('center_axis',(0.,-0.510701883081733,0.859757865108992));
#40285=DIRECTION('ref_axis',(0.,-0.859757865108992,-0.510701883081733));
#40286=DIRECTION('center_axis',(0.,-0.90630778703665,-0.422618261740699));
#40287=DIRECTION('ref_axis',(0.,0.422618261740699,-0.90630778703665));
#40288=DIRECTION('center_axis',(0.561006631580406,-0.809284384699504,0.174156090919475));
#40289=DIRECTION('ref_axis',(0.296477762129627,0.,-0.955039756535092));
#40290=DIRECTION('',(0.705516335778312,0.357374756306047,-0.611988548508171));
#40291=DIRECTION('',(0.,0.210381387077564,0.977619390136734));
#40292=DIRECTION('',(-0.705516335778298,-0.577478656052899,-0.410810298986407));
#40293=DIRECTION('center_axis',(0.561006631580407,-0.253818593389688,-0.787938881495568));
#40294=DIRECTION('ref_axis',(-0.814616058663781,0.,-0.580000583592023));
#40295=DIRECTION('',(0.705516335778306,0.644511483084942,0.29470603679192));
#40296=DIRECTION('',(0.,-0.951833920629446,0.306614069375781));
#40297=DIRECTION('',(-0.7055163357783,0.351310251680245,-0.615489891886393));
#40298=DIRECTION('center_axis',(-0.561006631580389,-0.809284384699515,0.174156090919477));
#40299=DIRECTION('ref_axis',(0.296477762129639,0.,0.955039756535089));
#40300=DIRECTION('',(0.,-0.210381387077564,-0.977619390136734));
#40301=DIRECTION('',(0.705516335778309,-0.357374756306019,0.611988548508191));
#40302=DIRECTION('',(-0.705516335778317,0.577478656052887,0.410810298986391));
#40303=DIRECTION('center_axis',(-0.707106781186541,-0.412732107142829,0.574153470540282));
#40304=DIRECTION('ref_axis',(0.63034738821444,0.,0.776313190774982));
#40305=DIRECTION('',(0.,-0.81197562492164,-0.583691343548208));
#40306=DIRECTION('',(0.,0.81197562492164,0.583691343548208));
#40307=DIRECTION('center_axis',(-0.561006631580389,-0.253818593389691,-0.787938881495579));
#40308=DIRECTION('ref_axis',(-0.814616058663794,0.,0.580000583592005));
#40309=DIRECTION('',(0.705516335778322,-0.644511483084929,-0.294706036791912));
#40310=DIRECTION('',(-0.705516335778301,-0.351310251680269,0.615489891886378));
#40311=DIRECTION('',(0.,0.951833920629446,-0.306614069375781));
#40312=DIRECTION('center_axis',(-0.707106781186549,0.290865437587466,-0.644513225013304));
#40313=DIRECTION('ref_axis',(-0.673638686438956,0.,0.739060836557315));
#40314=DIRECTION('',(0.,-0.911479343942639,-0.411345846661781));
#40315=DIRECTION('',(0.,0.911479343942639,0.411345846661781));
#40316=DIRECTION('center_axis',(0.,-0.306614069375781,-0.951833920629447));
#40317=DIRECTION('ref_axis',(-1.,0.,0.));
#40318=DIRECTION('',(-1.,0.,0.));
#40319=DIRECTION('',(1.,0.,0.));
#40320=DIRECTION('center_axis',(-0.707106781186533,-0.612372435695807,-0.353553390593281));
#40321=DIRECTION('ref_axis',(-0.447213595499973,0.,0.894427190999908));
#40322=DIRECTION('',(0.,-0.5,0.866025403784439));
#40323=DIRECTION('',(0.,0.5,-0.866025403784439));
#40324=DIRECTION('center_axis',(0.,-0.977619390136734,0.210381387077564));
#40325=DIRECTION('ref_axis',(0.,-0.210381387077564,-0.977619390136734));
#40326=DIRECTION('',(-1.,0.,0.));
#40327=DIRECTION('',(1.,0.,0.));
#40328=DIRECTION('center_axis',(0.707106781186551,0.290865437587465,-0.644513225013302));
#40329=DIRECTION('ref_axis',(-0.673638686438954,0.,-0.739060836557317));
#40330=DIRECTION('',(0.,-0.911479343942639,-0.411345846661781));
#40331=DIRECTION('',(0.,0.911479343942639,0.411345846661781));
#40332=DIRECTION('center_axis',(0.707106781186549,-0.612372435695794,-0.353553390593273));
#40333=DIRECTION('ref_axis',(-0.447213595499957,0.,-0.894427190999916));
#40334=DIRECTION('',(0.,-0.5,0.866025403784439));
#40335=DIRECTION('',(0.,0.5,-0.866025403784439));
#40336=DIRECTION('center_axis',(0.707106781186542,-0.412732107142828,0.57415347054028));
#40337=DIRECTION('ref_axis',(0.630347388214439,0.,-0.776313190774983));
#40338=DIRECTION('',(0.,-0.81197562492164,-0.583691343548208));
#40339=DIRECTION('',(0.,0.81197562492164,0.583691343548208));
#40340=DIRECTION('center_axis',(1.,0.,0.));
#40341=DIRECTION('ref_axis',(0.,0.866025403784439,0.5));
#40342=DIRECTION('center_axis',(0.,-0.583691343548208,0.81197562492164));
#40343=DIRECTION('ref_axis',(0.,-0.81197562492164,-0.583691343548208));
#40344=DIRECTION('center_axis',(0.,-0.866025403784439,-0.5));
#40345=DIRECTION('ref_axis',(0.,0.5,-0.866025403784439));
#40346=DIRECTION('center_axis',(0.707106781186547,-0.461202309044,0.53599666988936));
#40347=DIRECTION('ref_axis',(0.604079438549193,0.,-0.796924106751761));
#40348=DIRECTION('',(0.595596683047425,0.797046293239184,-0.099908946429145));
#40349=DIRECTION('',(0.,0.758013759944347,0.652238560447812));
#40350=DIRECTION('',(0.,-0.758013759944347,-0.652238560447812));
#40351=DIRECTION('',(0.557191914001244,-0.103279542068703,-0.823935984868794));
#40352=DIRECTION('center_axis',(1.,0.,0.));
#40353=DIRECTION('ref_axis',(0.,0.819152044288992,0.573576436351046));
#40354=DIRECTION('',(0.,-0.573576436351046,0.819152044288992));
#40355=DIRECTION('',(0.,-0.872159737063827,-0.489221210746995));
#40356=DIRECTION('center_axis',(0.707106781186547,-0.57922796533957,-0.405579787672639));
#40357=DIRECTION('ref_axis',(-0.497542812164523,0.,-0.867439421552547));
#40358=DIRECTION('',(0.55719191400124,0.103279542068703,0.823935984868796));
#40359=DIRECTION('',(0.,0.573576436351046,-0.819152044288992));
#40360=DIRECTION('',(0.705516335778315,0.616373598779637,0.349757468365408));
#40361=DIRECTION('center_axis',(0.,-0.992235199256928,0.124375678311978));
#40362=DIRECTION('ref_axis',(0.,-0.124375678311978,-0.992235199256928));
#40363=DIRECTION('',(-1.,0.,0.));
#40364=DIRECTION('',(0.,-0.124375678311978,-0.992235199256928));
#40365=DIRECTION('',(1.,0.,0.));
#40366=DIRECTION('center_axis',(0.561006631580405,-0.184179338555412,-0.807062284196269));
#40367=DIRECTION('ref_axis',(-0.821109284001921,0.,-0.570771008133607));
#40368=DIRECTION('',(0.,-0.974935082148261,0.22248951794762));
#40369=DIRECTION('',(-0.7055163357783,0.403616888790171,-0.582529061106229));
#40370=DIRECTION('center_axis',(-0.561006631580388,-0.821383516744214,0.102959592771799));
#40371=DIRECTION('ref_axis',(0.180511696561728,0.,0.983572837874454));
#40372=DIRECTION('',(0.705516335778303,-0.409353153962173,0.578512484991619));
#40373=DIRECTION('',(-0.705516335778314,0.539476698684484,0.459577622960944));
#40374=DIRECTION('center_axis',(-0.707106781186546,-0.461202309044001,0.535996669889361));
#40375=DIRECTION('ref_axis',(0.604079438549194,0.,0.79692410675176));
#40376=DIRECTION('',(0.,-0.758013759944347,-0.652238560447812));
#40377=DIRECTION('',(0.,0.758013759944347,0.652238560447812));
#40378=DIRECTION('center_axis',(-0.561006631580403,-0.184179338555412,-0.80706228419627));
#40379=DIRECTION('ref_axis',(-0.821109284001922,0.,0.570771008133605));
#40380=DIRECTION('',(0.705516335778317,-0.616373598779635,-0.349757468365407));
#40381=DIRECTION('',(-0.705516335778301,-0.40361688879017,0.582529061106227));
#40382=DIRECTION('',(0.,0.974935082148261,-0.22248951794762));
#40383=DIRECTION('center_axis',(-0.707106781186545,0.345931635619494,-0.616710064355711));
#40384=DIRECTION('ref_axis',(-0.657291420225582,0.,0.753636509796226));
#40385=DIRECTION('',(0.,-0.872159737063827,-0.489221210746995));
#40386=DIRECTION('',(0.,0.872159737063827,0.489221210746995));
#40387=DIRECTION('center_axis',(0.,-0.22248951794762,-0.974935082148261));
#40388=DIRECTION('ref_axis',(-1.,0.,0.));
#40389=DIRECTION('',(-1.,0.,0.));
#40390=DIRECTION('',(1.,0.,0.));
#40391=DIRECTION('center_axis',(-0.707106781186546,-0.579227965339571,-0.40557978767264));
#40392=DIRECTION('ref_axis',(-0.497542812164525,0.,0.867439421552546));
#40393=DIRECTION('',(0.,-0.573576436351046,0.819152044288992));
#40394=DIRECTION('',(0.,0.573576436351046,-0.819152044288992));
#40395=DIRECTION('center_axis',(0.707106781186546,0.345931635619494,-0.61671006435571));
#40396=DIRECTION('ref_axis',(-0.657291420225581,0.,-0.753636509796227));
#40397=DIRECTION('',(0.,0.872159737063827,0.489221210746995));
#40398=DIRECTION('center_axis',(0.,-0.652238560447812,0.758013759944347));
#40399=DIRECTION('ref_axis',(0.,-0.758013759944347,-0.652238560447812));
#40400=DIRECTION('center_axis',(0.,-0.819152044288992,-0.573576436351046));
#40401=DIRECTION('ref_axis',(0.,0.573576436351046,-0.819152044288992));
#40402=DIRECTION('center_axis',(0.56100663158041,-0.827231424261547,0.0309795099544078));
#40403=DIRECTION('ref_axis',(0.055137286528736,0.,-0.998478782766188));
#40404=DIRECTION('',(0.705516335778304,0.458216126942529,-0.540633592148827));
#40405=DIRECTION('',(0.,0.037423395534326,0.999299499382783));
#40406=DIRECTION('',(-0.705516335778297,-0.497368997894162,-0.50484728372422));
#40407=DIRECTION('center_axis',(0.561006631580388,-0.113138367744187,-0.820043455596719));
#40408=DIRECTION('ref_axis',(-0.825342782028786,0.,-0.564631997103409));
#40409=DIRECTION('',(0.705516335778318,0.58354473921108,0.402147034415285));
#40410=DIRECTION('',(0.,-0.990616399010033,0.136671686945011));
#40411=DIRECTION('',(-0.705516335778308,0.452851757665877,-0.545134832430359));
#40412=DIRECTION('center_axis',(-0.561006631580408,-0.827231424261548,0.0309795099544079));
#40413=DIRECTION('ref_axis',(0.0551372865287363,0.,0.998478782766188));
#40414=DIRECTION('',(0.,-0.037423395534326,-0.999299499382783));
#40415=DIRECTION('',(0.705516335778305,-0.458216126942528,0.540633592148826));
#40416=DIRECTION('',(-0.705516335778298,0.497368997894161,0.504847283724219));
#40417=DIRECTION('center_axis',(-0.707106781186549,-0.506162482891781,0.493760610936946));
#40418=DIRECTION('ref_axis',(0.572517134274668,0.,0.819892755768657));
#40419=DIRECTION('',(0.,-0.698282952552655,-0.715821848069998));
#40420=DIRECTION('',(0.,0.698282952552655,0.715821848069998));
#40421=DIRECTION('center_axis',(-0.561006631580386,-0.113138367744187,-0.82004345559672));
#40422=DIRECTION('ref_axis',(-0.825342782028787,0.,0.564631997103407));
#40423=DIRECTION('',(0.705516335778319,-0.583544739211079,-0.402147034415284));
#40424=DIRECTION('',(-0.70551633577831,-0.452851757665876,0.545134832430358));
#40425=DIRECTION('',(0.,0.990616399010033,-0.136671686945011));
#40426=DIRECTION('center_axis',(-0.70710678118654,0.398365085025227,-0.584213367728653));
#40427=DIRECTION('ref_axis',(-0.636934375125939,0.,0.770918025332739));
#40428=DIRECTION('',(0.,-0.826202467961513,-0.563373306018581));
#40429=DIRECTION('',(0.,0.826202467961513,0.563373306018581));
#40430=DIRECTION('center_axis',(0.,-0.136671686945011,-0.990616399010033));
#40431=DIRECTION('ref_axis',(-1.,0.,0.));
#40432=DIRECTION('',(-1.,0.,0.));
#40433=DIRECTION('',(1.,0.,0.));
#40434=DIRECTION('center_axis',(-0.707106781186548,-0.541675220419702,-0.454519477672043));
#40435=DIRECTION('ref_axis',(-0.540716203060936,0.,0.841205080671393));
#40436=DIRECTION('',(0.,-0.642787609686539,0.766044443118978));
#40437=DIRECTION('',(0.,0.642787609686539,-0.766044443118978));
#40438=DIRECTION('center_axis',(0.,-0.999299499382783,0.037423395534326));
#40439=DIRECTION('ref_axis',(0.,-0.037423395534326,-0.999299499382783));
#40440=DIRECTION('',(-1.,0.,0.));
#40441=DIRECTION('',(1.,0.,0.));
#40442=DIRECTION('center_axis',(0.707106781186542,0.398365085025226,-0.584213367728652));
#40443=DIRECTION('ref_axis',(-0.636934375125937,0.,-0.770918025332741));
#40444=DIRECTION('',(0.,-0.826202467961513,-0.563373306018581));
#40445=DIRECTION('',(0.,0.826202467961513,0.563373306018581));
#40446=DIRECTION('center_axis',(0.70710678118655,-0.5416752204197,-0.454519477672042));
#40447=DIRECTION('ref_axis',(-0.540716203060935,0.,-0.841205080671394));
#40448=DIRECTION('',(0.,-0.642787609686539,0.766044443118978));
#40449=DIRECTION('',(0.,0.642787609686539,-0.766044443118978));
#40450=DIRECTION('center_axis',(0.707106781186551,-0.50616248289178,0.493760610936944));
#40451=DIRECTION('ref_axis',(0.572517134274666,0.,-0.819892755768658));
#40452=DIRECTION('',(0.,-0.698282952552655,-0.715821848069998));
#40453=DIRECTION('',(0.,0.698282952552655,0.715821848069998));
#40454=DIRECTION('center_axis',(1.,0.,0.));
#40455=DIRECTION('ref_axis',(0.,0.766044443118978,0.642787609686539));
#40456=DIRECTION('center_axis',(0.,-0.715821848069998,0.698282952552655));
#40457=DIRECTION('ref_axis',(0.,-0.698282952552655,-0.715821848069998));
#40458=DIRECTION('center_axis',(0.,-0.766044443118978,-0.642787609686539));
#40459=DIRECTION('ref_axis',(0.,0.642787609686539,-0.766044443118978));
#40460=DIRECTION('center_axis',(0.561006631580414,-0.0412363456396373,-0.826783601144269));
#40461=DIRECTION('ref_axis',(-0.827487445286302,0.,-0.561484218739537));
#40462=DIRECTION('',(0.705516335778305,0.546274751823179,0.451476018710272));
#40463=DIRECTION('',(0.,-0.998758526924799,0.0498137018801604));
#40464=DIRECTION('',(-0.705516335778304,0.49864015122633,-0.503591798518341));
#40465=DIRECTION('center_axis',(0.,-0.0498137018801604,-0.998758526924799));
#40466=DIRECTION('ref_axis',(-1.,0.,0.));
#40467=DIRECTION('',(0.55719191400124,0.829352850155045,-0.041364488529864));
#40468=DIRECTION('',(1.,0.,0.));
#40469=DIRECTION('',(-1.,0.,0.));
#40470=DIRECTION('',(-0.557191914001243,0.829352850155043,-0.0413644885298639));
#40471=DIRECTION('center_axis',(0.707106781186551,0.447766735594493,-0.547270454615491));
#40472=DIRECTION('ref_axis',(-0.612056372482119,0.,-0.790814135498367));
#40473=DIRECTION('',(0.,-0.773957299203321,-0.633237790257263));
#40474=DIRECTION('',(0.,0.773957299203321,0.633237790257263));
#40475=DIRECTION('center_axis',(0.561006631580404,-0.826783601144275,-0.0412363456396555));
#40476=DIRECTION('ref_axis',(-0.0733064378127395,0.,-0.997309463594529));
#40477=DIRECTION('',(0.705516335778296,0.503591798518335,-0.498640151226349));
#40478=DIRECTION('',(0.,-0.0498137018801819,0.998758526924798));
#40479=DIRECTION('',(-0.705516335778303,-0.451476018710246,-0.546274751823203));
#40480=DIRECTION('center_axis',(0.,-0.998758526924798,-0.0498137018801819));
#40481=DIRECTION('ref_axis',(0.,0.0498137018801819,-0.998758526924798));
#40482=DIRECTION('',(0.557191914001234,0.0413644885298821,-0.829352850155049));
#40483=DIRECTION('',(1.,0.,0.));
#40484=DIRECTION('',(-1.,0.,0.));
#40485=DIRECTION('',(-0.557191914001249,0.0413644885298816,-0.829352850155038));
#40486=DIRECTION('center_axis',(0.707106781186548,-0.5,-0.5));
#40487=DIRECTION('ref_axis',(-0.577350269189625,0.,-0.816496580927727));
#40488=DIRECTION('',(0.,-0.707106781186547,0.707106781186548));
#40489=DIRECTION('',(0.,0.707106781186547,-0.707106781186548));
#40490=DIRECTION('center_axis',(0.707106781186552,-0.547270454615491,0.447766735594493));
#40491=DIRECTION('ref_axis',(0.534994468449983,0.,-0.844855560867016));
#40492=DIRECTION('',(0.,-0.633237790257263,-0.773957299203321));
#40493=DIRECTION('',(0.,0.633237790257263,0.773957299203321));
#40494=DIRECTION('center_axis',(-0.70710678118655,0.447766735594494,-0.547270454615492));
#40495=DIRECTION('ref_axis',(-0.61205637248212,0.,0.790814135498366));
#40496=DIRECTION('',(-0.595596683047422,0.0400145312984556,0.802286375571637));
#40497=DIRECTION('',(0.,0.773957299203321,0.633237790257263));
#40498=DIRECTION('',(0.,-0.773957299203321,-0.633237790257263));
#40499=DIRECTION('center_axis',(0.,-0.707106781186548,-0.707106781186547));
#40500=DIRECTION('ref_axis',(0.,0.707106781186547,-0.707106781186548));
#40501=DIRECTION('',(0.,-0.707106781186547,0.707106781186548));
#40502=DIRECTION('center_axis',(-0.707106781186547,-0.500000000000001,-0.500000000000001));
#40503=DIRECTION('ref_axis',(-0.577350269189627,0.,0.816496580927725));
#40504=DIRECTION('',(0.595596683047432,-0.802286375571628,-0.0400145312984774));
#40505=DIRECTION('',(0.,0.707106781186547,-0.707106781186548));
#40506=DIRECTION('center_axis',(-0.70710678118655,-0.547270454615492,0.447766735594494));
#40507=DIRECTION('ref_axis',(0.534994468449985,0.,0.844855560867015));
#40508=DIRECTION('',(0.,0.633237790257263,0.773957299203321));
#40509=DIRECTION('',(0.,-0.633237790257263,-0.773957299203321));
#40510=DIRECTION('center_axis',(0.,-0.773957299203321,0.633237790257263));
#40511=DIRECTION('ref_axis',(0.,-0.633237790257263,-0.773957299203321));
#40512=DIRECTION('center_axis',(0.,0.633237790257263,-0.773957299203321));
#40513=DIRECTION('ref_axis',(0.,0.773957299203321,0.633237790257263));
#40514=DIRECTION('center_axis',(0.561006631580392,-0.820043455596711,-0.113138367744223));
#40515=DIRECTION('ref_axis',(-0.197690230426254,0.,-0.98026454225072));
#40516=DIRECTION('',(0.705516335778306,0.545134832430383,-0.452851757665851));
#40517=DIRECTION('',(0.,-0.136671686945054,0.990616399010027));
#40518=DIRECTION('',(-0.705516335778304,-0.402147034415252,-0.583544739211119));
#40519=DIRECTION('center_axis',(0.5610066315804,0.0309795099544278,-0.827231424261552));
#40520=DIRECTION('ref_axis',(-0.827628669643389,0.,-0.561276032968016));
#40521=DIRECTION('',(0.705516335778306,0.504847283724201,0.497368997894168));
#40522=DIRECTION('',(0.,-0.999299499382783,-0.0374233955343499));
#40523=DIRECTION('',(-0.705516335778302,0.540633592148851,-0.458216126942503));
#40524=DIRECTION('center_axis',(-0.56100663158039,-0.820043455596712,-0.113138367744223));
#40525=DIRECTION('ref_axis',(-0.197690230426255,0.,0.98026454225072));
#40526=DIRECTION('',(0.,0.136671686945054,-0.990616399010027));
#40527=DIRECTION('',(0.705516335778308,-0.545134832430382,0.45285175766585));
#40528=DIRECTION('',(-0.705516335778306,0.402147034415251,0.583544739211118));
#40529=DIRECTION('center_axis',(-0.707106781186547,-0.584213367728647,0.398365085025223));
#40530=DIRECTION('ref_axis',(0.490839120629135,0.,0.871250226777599));
#40531=DIRECTION('',(0.,-0.563373306018581,-0.826202467961513));
#40532=DIRECTION('',(0.,0.563373306018581,0.826202467961513));
#40533=DIRECTION('center_axis',(-0.561006631580419,0.0309795099544274,-0.82723142426154));
#40534=DIRECTION('ref_axis',(-0.827628669643377,0.,0.561276032968035));
#40535=DIRECTION('',(0.705516335778298,-0.504847283724194,-0.497368997894186));
#40536=DIRECTION('',(-0.705516335778296,-0.540633592148843,0.458216126942521));
#40537=DIRECTION('',(0.,0.999299499382783,0.0374233955343499));
#40538=DIRECTION('center_axis',(-0.707106781186558,0.493760610936939,-0.506162482891774));
#40539=DIRECTION('ref_axis',(-0.582064997116532,0.,0.813142262541882));
#40540=DIRECTION('',(0.,-0.715821848069998,-0.698282952552655));
#40541=DIRECTION('',(0.,0.715821848069998,0.698282952552655));
#40542=DIRECTION('center_axis',(0.,0.0374233955343499,-0.999299499382783));
#40543=DIRECTION('ref_axis',(-1.,0.,0.));
#40544=DIRECTION('',(-1.,0.,0.));
#40545=DIRECTION('',(1.,0.,0.));
#40546=DIRECTION('center_axis',(-0.707106781186558,-0.454519477672037,-0.541675220419694));
#40547=DIRECTION('ref_axis',(-0.608120402411332,0.,0.793844806099454));
#40548=DIRECTION('',(0.,-0.766044443118978,0.642787609686539));
#40549=DIRECTION('',(0.,0.766044443118978,-0.642787609686539));
#40550=DIRECTION('center_axis',(0.,-0.990616399010027,-0.136671686945054));
#40551=DIRECTION('ref_axis',(0.,0.136671686945054,-0.990616399010027));
#40552=DIRECTION('',(-1.,0.,0.));
#40553=DIRECTION('',(1.,0.,0.));
#40554=DIRECTION('center_axis',(0.70710678118656,0.493760610936938,-0.506162482891773));
#40555=DIRECTION('ref_axis',(-0.58206499711653,0.,-0.813142262541884));
#40556=DIRECTION('',(0.,-0.715821848069998,-0.698282952552655));
#40557=DIRECTION('',(0.,0.715821848069998,0.698282952552655));
#40558=DIRECTION('center_axis',(0.70710678118655,-0.454519477672042,-0.5416752204197));
#40559=DIRECTION('ref_axis',(-0.608120402411341,0.,-0.793844806099447));
#40560=DIRECTION('',(0.,-0.766044443118978,0.642787609686539));
#40561=DIRECTION('',(0.,0.766044443118978,-0.642787609686539));
#40562=DIRECTION('center_axis',(0.707106781186549,-0.584213367728646,0.398365085025222));
#40563=DIRECTION('ref_axis',(0.490839120629133,0.,-0.8712502267776));
#40564=DIRECTION('',(0.,-0.563373306018581,-0.826202467961513));
#40565=DIRECTION('',(0.,0.563373306018581,0.826202467961513));
#40566=DIRECTION('center_axis',(1.,0.,0.));
#40567=DIRECTION('ref_axis',(0.,0.642787609686539,0.766044443118978));
#40568=DIRECTION('center_axis',(0.,-0.826202467961513,0.563373306018581));
#40569=DIRECTION('ref_axis',(0.,-0.563373306018581,-0.826202467961513));
#40570=DIRECTION('center_axis',(0.,-0.642787609686539,-0.766044443118978));
#40571=DIRECTION('ref_axis',(0.,0.766044443118978,-0.642787609686539));
#40572=DIRECTION('center_axis',(0.56100663158041,-0.807062284196261,-0.18417933855543));
#40573=DIRECTION('ref_axis',(-0.311921838389611,0.,-0.950107765853772));
#40574=DIRECTION('',(0.705516335778302,0.582529061106243,-0.403616888790147));
#40575=DIRECTION('',(0.,-0.222489517947642,0.974935082148255));
#40576=DIRECTION('',(-0.705516335778307,-0.349757468365392,-0.616373598779655));
#40577=DIRECTION('center_axis',(0.56100663158042,0.102959592771817,-0.82138351674419));
#40578=DIRECTION('ref_axis',(-0.825772049781951,0.,-0.564004008672735));
#40579=DIRECTION('',(0.705516335778302,0.459577622960913,0.539476698684527));
#40580=DIRECTION('',(0.,-0.992235199256925,-0.124375678312001));
#40581=DIRECTION('',(-0.705516335778294,0.578512484991614,-0.409353153962195));
#40582=DIRECTION('center_axis',(-0.561006631580408,-0.807062284196262,-0.18417933855543));
#40583=DIRECTION('ref_axis',(-0.311921838389613,0.,0.950107765853771));
#40584=DIRECTION('',(0.,0.222489517947642,-0.974935082148255));
#40585=DIRECTION('',(0.705516335778303,-0.582529061106242,0.403616888790146));
#40586=DIRECTION('',(-0.705516335778309,0.349757468365391,0.616373598779654));
#40587=DIRECTION('center_axis',(-0.707106781186545,-0.616710064355711,0.345931635619495));
#40588=DIRECTION('ref_axis',(0.439451044888515,0.,0.898266541259548));
#40589=DIRECTION('',(0.,-0.489221210746995,-0.872159737063827));
#40590=DIRECTION('',(0.,0.489221210746995,0.872159737063827));
#40591=DIRECTION('center_axis',(-0.561006631580396,0.102959592771819,-0.821383516744206));
#40592=DIRECTION('ref_axis',(-0.825772049781968,0.,0.564004008672711));
#40593=DIRECTION('',(0.705516335778305,-0.459577622960938,-0.539476698684502));
#40594=DIRECTION('',(-0.705516335778313,-0.578512484991602,0.409353153962179));
#40595=DIRECTION('',(0.,0.992235199256925,0.124375678312001));
#40596=DIRECTION('center_axis',(-0.707106781186541,0.535996669889364,-0.461202309044004));
#40597=DIRECTION('ref_axis',(-0.546305769586294,0.,0.837585820150226));
#40598=DIRECTION('',(0.,-0.652238560447812,-0.758013759944346));
#40599=DIRECTION('',(0.,0.652238560447812,0.758013759944346));
#40600=DIRECTION('center_axis',(0.,0.124375678312001,-0.992235199256925));
#40601=DIRECTION('ref_axis',(-1.,0.,0.));
#40602=DIRECTION('',(-1.,0.,0.));
#40603=DIRECTION('',(1.,0.,0.));
#40604=DIRECTION('center_axis',(-0.707106781186546,-0.40557978767264,-0.579227965339571));
#40605=DIRECTION('ref_axis',(-0.633687274224644,0.,0.773589321594954));
#40606=DIRECTION('',(0.,-0.819152044288992,0.573576436351046));
#40607=DIRECTION('',(0.,0.819152044288992,-0.573576436351046));
#40608=DIRECTION('center_axis',(0.,-0.974935082148256,-0.222489517947642));
#40609=DIRECTION('ref_axis',(0.,0.222489517947642,-0.974935082148255));
#40610=DIRECTION('',(-1.,0.,0.));
#40611=DIRECTION('',(1.,0.,0.));
#40612=DIRECTION('center_axis',(0.707106781186552,0.535996669889356,-0.461202309043997));
#40613=DIRECTION('ref_axis',(-0.546305769586282,0.,-0.837585820150234));
#40614=DIRECTION('',(0.,-0.652238560447812,-0.758013759944346));
#40615=DIRECTION('',(0.,0.652238560447812,0.758013759944346));
#40616=DIRECTION('center_axis',(0.707106781186547,-0.405579787672639,-0.579227965339569));
#40617=DIRECTION('ref_axis',(-0.633687274224642,0.,-0.773589321594955));
#40618=DIRECTION('',(0.,-0.819152044288992,0.573576436351046));
#40619=DIRECTION('',(0.,0.819152044288992,-0.573576436351046));
#40620=DIRECTION('center_axis',(0.707106781186546,-0.61671006435571,0.345931635619494));
#40621=DIRECTION('ref_axis',(0.439451044888514,0.,-0.898266541259549));
#40622=DIRECTION('',(0.,-0.489221210746995,-0.872159737063827));
#40623=DIRECTION('',(0.,0.489221210746995,0.872159737063827));
#40624=DIRECTION('center_axis',(1.,0.,0.));
#40625=DIRECTION('ref_axis',(0.,0.573576436351046,0.819152044288992));
#40626=DIRECTION('center_axis',(0.,-0.872159737063827,0.489221210746995));
#40627=DIRECTION('ref_axis',(0.,-0.489221210746995,-0.872159737063827));
#40628=DIRECTION('center_axis',(0.,-0.573576436351046,-0.819152044288992));
#40629=DIRECTION('ref_axis',(0.,0.819152044288992,-0.573576436351046));
#40630=DIRECTION('center_axis',(0.707106781186551,-0.644513225013302,0.290865437587466));
#40631=DIRECTION('ref_axis',(0.380418570543385,0.,-0.924814419862562));
#40632=DIRECTION('',(0.595596683047424,0.764592607463602,0.246298062832244));
#40633=DIRECTION('',(0.,0.411345846661781,0.911479343942639));
#40634=DIRECTION('',(0.,-0.411345846661781,-0.911479343942639));
#40635=DIRECTION('',(0.557191914001241,0.25460734049242,-0.790387419648751));
#40636=DIRECTION('center_axis',(1.,0.,0.));
#40637=DIRECTION('ref_axis',(0.,0.5,0.866025403784439));
#40638=DIRECTION('',(0.,-0.866025403784439,0.5));
#40639=DIRECTION('',(0.,-0.583691343548208,-0.81197562492164));
#40640=DIRECTION('center_axis',(0.707106781186545,-0.353553390593275,-0.612372435695796));
#40641=DIRECTION('ref_axis',(-0.654653670707979,0.,-0.755928946018453));
#40642=DIRECTION('',(0.557191914001241,-0.25460734049242,0.790387419648751));
#40643=DIRECTION('',(0.,0.866025403784439,-0.5));
#40644=DIRECTION('',(0.705516335778306,0.410810298986386,0.577478656052905));
#40645=DIRECTION('center_axis',(0.,-0.951833920629443,-0.306614069375792));
#40646=DIRECTION('ref_axis',(0.,0.306614069375792,-0.951833920629443));
#40647=DIRECTION('',(-1.,0.,0.));
#40648=DIRECTION('',(0.,0.306614069375792,-0.951833920629443));
#40649=DIRECTION('',(1.,0.,0.));
#40650=DIRECTION('center_axis',(0.561006631580401,0.174156090919492,-0.809284384699503));
#40651=DIRECTION('ref_axis',(-0.821843752318938,0.,-0.569712951208174));
#40652=DIRECTION('',(0.,-0.97761939013673,-0.210381387077584));
#40653=DIRECTION('',(-0.705516335778302,0.6119885485082,-0.357374756306017));
#40654=DIRECTION('center_axis',(-0.561006631580415,-0.787938881495563,-0.253818593389686));
#40655=DIRECTION('ref_axis',(-0.412208150462309,0.,0.911089699586403));
#40656=DIRECTION('',(0.705516335778296,-0.615489891886399,0.351310251680242));
#40657=DIRECTION('',(-0.705516335778305,0.294706036791931,0.644511483084939));
#40658=DIRECTION('center_axis',(-0.707106781186555,-0.644513225013298,0.290865437587464));
#40659=DIRECTION('ref_axis',(0.380418570543382,0.,0.924814419862564));
#40660=DIRECTION('',(0.,-0.411345846661781,-0.911479343942639));
#40661=DIRECTION('',(0.,0.411345846661781,0.911479343942639));
#40662=DIRECTION('center_axis',(-0.5610066315804,0.174156090919493,-0.809284384699504));
#40663=DIRECTION('ref_axis',(-0.82184375231894,0.,0.569712951208172));
#40664=DIRECTION('',(0.705516335778307,-0.410810298986385,-0.577478656052904));
#40665=DIRECTION('',(-0.705516335778303,-0.611988548508199,0.357374756306016));
#40666=DIRECTION('',(0.,0.97761939013673,0.210381387077584));
#40667=DIRECTION('center_axis',(-0.707106781186546,0.574153470540278,-0.412732107142826));
#40668=DIRECTION('ref_axis',(-0.504101701135472,0.,0.86364429883623));
#40669=DIRECTION('',(0.,-0.583691343548208,-0.81197562492164));
#40670=DIRECTION('',(0.,0.583691343548208,0.81197562492164));
#40671=DIRECTION('center_axis',(0.,0.210381387077584,-0.97761939013673));
#40672=DIRECTION('ref_axis',(-1.,0.,0.));
#40673=DIRECTION('',(-1.,0.,0.));
#40674=DIRECTION('',(1.,0.,0.));
#40675=DIRECTION('center_axis',(-0.707106781186544,-0.353553390593276,-0.612372435695798));
#40676=DIRECTION('ref_axis',(-0.654653670707981,0.,0.755928946018451));
#40677=DIRECTION('',(0.,-0.866025403784439,0.5));
#40678=DIRECTION('',(0.,0.866025403784439,-0.5));
#40679=DIRECTION('center_axis',(0.707106781186547,0.574153470540276,-0.412732107142825));
#40680=DIRECTION('ref_axis',(-0.50410170113547,0.,-0.863644298836231));
#40681=DIRECTION('',(0.,0.583691343548208,0.81197562492164));
#40682=DIRECTION('center_axis',(0.,-0.911479343942639,0.411345846661781));
#40683=DIRECTION('ref_axis',(0.,-0.411345846661781,-0.911479343942639));
#40684=DIRECTION('center_axis',(0.,-0.5,-0.866025403784439));
#40685=DIRECTION('ref_axis',(0.,0.866025403784439,-0.5));
#40686=DIRECTION('center_axis',(0.561006631580433,-0.762818788136164,-0.321526135468411));
#40687=DIRECTION('ref_axis',(-0.49724715095984,0.,-0.867608938901808));
#40688=DIRECTION('',(0.705516335778299,0.643766472946357,-0.296329931428078));
#40689=DIRECTION('',(0.,-0.388405102597364,0.921488728241605));
#40690=DIRECTION('',(-0.705516335778299,-0.23741171433011,-0.667744245837282));
#40691=DIRECTION('center_axis',(0.561006631580399,0.244027156056944,-0.791026109827972));
#40692=DIRECTION('ref_axis',(-0.815685591418258,0.,-0.578495476173018));
#40693=DIRECTION('',(0.705516335778309,0.358916460582513,0.611085652157592));
#40694=DIRECTION('',(0.,-0.955563307154869,-0.294785966455749));
#40695=DIRECTION('',(-0.705516335778307,0.640807009641837,-0.302676520965598));
#40696=DIRECTION('center_axis',(-0.56100663158041,-0.762818788136182,-0.321526135468408));
#40697=DIRECTION('ref_axis',(-0.497247150959853,0.,0.867608938901801));
#40698=DIRECTION('',(0.,0.388405102597364,-0.921488728241605));
#40699=DIRECTION('',(0.705516335778301,-0.643766472946344,0.296329931428102));
#40700=DIRECTION('',(-0.705516335778315,0.237411714330102,0.667744245837269));
#40701=DIRECTION('center_axis',(-0.707106781186556,-0.667411250860817,0.233585577946044));
#40702=DIRECTION('ref_axis',(0.313668483594035,0.,0.949532559947166));
#40703=DIRECTION('',(0.,-0.330339892306057,-0.943862042647771));
#40704=DIRECTION('',(0.,0.330339892306057,0.943862042647771));
#40705=DIRECTION('center_axis',(-0.561006631580381,0.244027156056947,-0.791026109827984));
#40706=DIRECTION('ref_axis',(-0.815685591418271,0.,0.578495476173));
#40707=DIRECTION('',(0.705516335778325,-0.358916460582507,-0.611085652157578));
#40708=DIRECTION('',(-0.705516335778308,-0.640807009641848,0.302676520965572));
#40709=DIRECTION('',(0.,0.955563307154869,0.294785966455749));
#40710=DIRECTION('center_axis',(-0.707106781186546,0.607940616597039,-0.361120764691834));
#40711=DIRECTION('ref_axis',(-0.454822071931222,0.,0.890582327965354));
#40712=DIRECTION('',(0.,-0.510701883081733,-0.859757865108992));
#40713=DIRECTION('',(0.,0.510701883081733,0.859757865108992));
#40714=DIRECTION('center_axis',(0.,0.294785966455749,-0.955563307154869));
#40715=DIRECTION('ref_axis',(-1.,0.,0.));
#40716=DIRECTION('',(-1.,0.,0.));
#40717=DIRECTION('',(1.,0.,0.));
#40718=DIRECTION('center_axis',(-0.707106781186538,-0.298836238730124,-0.640856382055797));
#40719=DIRECTION('ref_axis',(-0.671542934237828,0.,0.74096564527328));
#40720=DIRECTION('',(0.,-0.90630778703665,0.422618261740699));
#40721=DIRECTION('',(0.,0.90630778703665,-0.422618261740699));
#40722=DIRECTION('center_axis',(0.,-0.921488728241605,-0.388405102597364));
#40723=DIRECTION('ref_axis',(0.,0.388405102597364,-0.921488728241605));
#40724=DIRECTION('',(-1.,0.,0.));
#40725=DIRECTION('',(1.,0.,0.));
#40726=DIRECTION('center_axis',(0.707106781186547,0.607940616597037,-0.361120764691833));
#40727=DIRECTION('ref_axis',(-0.454822071931221,0.,-0.890582327965355));
#40728=DIRECTION('',(0.,-0.510701883081733,-0.859757865108992));
#40729=DIRECTION('',(0.,0.510701883081733,0.859757865108992));
#40730=DIRECTION('center_axis',(0.707106781186554,-0.298836238730117,-0.640856382055783));
#40731=DIRECTION('ref_axis',(-0.671542934237811,0.,-0.740965645273295));
#40732=DIRECTION('',(0.,-0.90630778703665,0.422618261740699));
#40733=DIRECTION('',(0.,0.90630778703665,-0.422618261740699));
#40734=DIRECTION('center_axis',(0.707106781186557,-0.667411250860816,0.233585577946044));
#40735=DIRECTION('ref_axis',(0.313668483594033,0.,-0.949532559947167));
#40736=DIRECTION('',(0.,-0.330339892306057,-0.943862042647771));
#40737=DIRECTION('',(0.,0.330339892306057,0.943862042647771));
#40738=DIRECTION('center_axis',(1.,0.,0.));
#40739=DIRECTION('ref_axis',(0.,0.422618261740699,0.90630778703665));
#40740=DIRECTION('center_axis',(0.,-0.943862042647771,0.330339892306057));
#40741=DIRECTION('ref_axis',(0.,-0.330339892306057,-0.943862042647771));
#40742=DIRECTION('center_axis',(0.,-0.422618261740699,-0.90630778703665));
#40743=DIRECTION('ref_axis',(0.,0.90630778703665,-0.422618261740699));
#40744=DIRECTION('center_axis',(0.561006631580418,0.312041027189173,-0.766747648626013));
#40745=DIRECTION('ref_axis',(-0.807044487383567,0.,-0.590490639539523));
#40746=DIRECTION('',(0.705516335778306,0.304291051193903,0.640041917465772));
#40747=DIRECTION('',(0.,-0.926234810420659,-0.376947046632555));
#40748=DIRECTION('',(-0.705516335778304,0.66474854250225,-0.245674734539573));
#40749=DIRECTION('center_axis',(0.,0.376947046632555,-0.926234810420659));
#40750=DIRECTION('ref_axis',(-1.,0.,0.));
#40751=DIRECTION('',(0.557191914001246,0.769130334536836,0.31301070184082));
#40752=DIRECTION('',(1.,0.,0.));
#40753=DIRECTION('',(-1.,0.,0.));
#40754=DIRECTION('',(-0.557191914001243,0.769130334536838,0.313010701840821));
#40755=DIRECTION('center_axis',(0.707106781186549,0.637100967476913,-0.306761075170856));
#40756=DIRECTION('ref_axis',(-0.397987666358442,0.,-0.917390765937047));
#40757=DIRECTION('',(0.,-0.433825672914778,-0.900996828806872));
#40758=DIRECTION('',(0.,0.433825672914778,0.900996828806872));
#40759=DIRECTION('center_axis',(0.561006631580401,-0.731893183196504,-0.386786669513441));
#40760=DIRECTION('ref_axis',(-0.567619122871708,0.,-0.823291279773054));
#40761=DIRECTION('',(0.70551633577831,0.667143602430344,-0.23909436146888));
#40762=DIRECTION('',(0.,-0.467240138462762,0.884130450221741));
#40763=DIRECTION('',(-0.705516335778305,-0.178310545369065,-0.685895071683811));
#40764=DIRECTION('center_axis',(0.,-0.884130450221741,-0.467240138462762));
#40765=DIRECTION('ref_axis',(0.,0.467240138462762,-0.884130450221741));
#40766=DIRECTION('',(0.557191914001245,0.387988617963615,-0.734167558056275));
#40767=DIRECTION('',(1.,0.,0.));
#40768=DIRECTION('',(-1.,0.,0.));
#40769=DIRECTION('',(-0.557191914001248,0.387988617963614,-0.734167558056273));
#40770=DIRECTION('center_axis',(0.707106781186551,-0.241844762647974,-0.664463024388671));
#40771=DIRECTION('ref_axis',(-0.684791078771732,0.,-0.728739444818686));
#40772=DIRECTION('',(0.,-0.939692620785908,0.342020143325669));
#40773=DIRECTION('',(0.,0.939692620785908,-0.342020143325669));
#40774=DIRECTION('center_axis',(0.70710678118654,-0.68522987409537,0.174527991013631));
#40775=DIRECTION('ref_axis',(0.239628661022762,0.,-0.97086461714105));
#40776=DIRECTION('',(0.,-0.246819851905204,-0.96906138128887));
#40777=DIRECTION('',(0.,0.246819851905204,0.96906138128887));
#40778=DIRECTION('center_axis',(-0.707106781186541,0.63710096747692,-0.30676107517086));
#40779=DIRECTION('ref_axis',(-0.397987666358449,0.,0.917390765937044));
#40780=DIRECTION('',(-0.595596683047422,-0.3027953921519,0.744029261275715));
#40781=DIRECTION('',(0.,0.433825672914778,0.900996828806872));
#40782=DIRECTION('',(0.,-0.433825672914778,-0.900996828806872));
#40783=DIRECTION('center_axis',(0.,-0.342020143325669,-0.939692620785908));
#40784=DIRECTION('ref_axis',(0.,0.939692620785908,-0.342020143325669));
#40785=DIRECTION('',(0.,-0.939692620785908,0.342020143325669));
#40786=DIRECTION('center_axis',(-0.70710678118655,-0.241844762647975,-0.664463024388673));
#40787=DIRECTION('ref_axis',(-0.684791078771734,0.,0.728739444818685));
#40788=DIRECTION('',(0.595596683047427,-0.710207517952258,-0.375326354772744));
#40789=DIRECTION('',(0.,0.939692620785908,-0.342020143325669));
#40790=DIRECTION('center_axis',(-0.707106781186539,-0.685229874095371,0.174527991013632));
#40791=DIRECTION('ref_axis',(0.239628661022763,0.,0.97086461714105));
#40792=DIRECTION('',(0.,0.246819851905204,0.96906138128887));
#40793=DIRECTION('',(0.,-0.246819851905204,-0.96906138128887));
#40794=DIRECTION('center_axis',(0.,-0.96906138128887,0.246819851905204));
#40795=DIRECTION('ref_axis',(0.,-0.246819851905204,-0.96906138128887));
#40796=DIRECTION('center_axis',(0.,0.900996828806872,-0.433825672914778));
#40797=DIRECTION('ref_axis',(0.,0.433825672914778,0.900996828806872));
#40798=DIRECTION('center_axis',(0.561006631580406,-0.695397429203504,-0.449103523455299));
#40799=DIRECTION('ref_axis',(-0.624948053917885,0.,-0.780666337114806));
#40800=DIRECTION('',(0.705516335778305,0.685443366267539,-0.18003913904976));
#40801=DIRECTION('',(0.,-0.542519194747163,0.84004340562312));
#40802=DIRECTION('',(-0.705516335778305,-0.117852325490949,-0.698825821880052));
#40803=DIRECTION('center_axis',(0.561006631580393,0.37768007768899,-0.736633774843144));
#40804=DIRECTION('ref_axis',(-0.795555689966286,0.,-0.605880470193806));
#40805=DIRECTION('',(0.705516335778306,0.2473498031698,0.664127077314135));
#40806=DIRECTION('',(0.,-0.889857107503274,-0.456239332177649));
#40807=DIRECTION('',(-0.705516335778306,0.683630937568096,-0.186803215041171));
#40808=DIRECTION('center_axis',(-0.561006631580404,-0.695397429203505,-0.4491035234553));
#40809=DIRECTION('ref_axis',(-0.624948053917886,0.,0.780666337114805));
#40810=DIRECTION('',(0.,0.542519194747163,-0.84004340562312));
#40811=DIRECTION('',(0.705516335778306,-0.685443366267538,0.180039139049759));
#40812=DIRECTION('',(-0.705516335778306,0.117852325490948,0.69882582188005));
#40813=DIRECTION('center_axis',(-0.707106781186546,-0.697833484234925,0.114142140686716));
#40814=DIRECTION('ref_axis',(0.159358523666365,0.,0.987220776186805));
#40815=DIRECTION('',(0.,-0.161421363397452,-0.986885577683101));
#40816=DIRECTION('',(0.,0.161421363397452,0.986885577683101));
#40817=DIRECTION('center_axis',(-0.561006631580394,0.37768007768899,-0.736633774843143));
#40818=DIRECTION('ref_axis',(-0.795555689966285,0.,0.605880470193806));
#40819=DIRECTION('',(0.705516335778308,-0.247349803169793,-0.664127077314134));
#40820=DIRECTION('',(-0.705516335778305,-0.683630937568098,0.18680321504117));
#40821=DIRECTION('',(0.,0.889857107503274,0.456239332177649));
#40822=DIRECTION('center_axis',(-0.707106781186547,0.66141259530221,-0.250066748640429));
#40823=DIRECTION('ref_axis',(-0.333412439312661,0.,0.942781069661234));
#40824=DIRECTION('',(0.,-0.353647787425838,-0.935378662600772));
#40825=DIRECTION('',(0.,0.353647787425838,0.935378662600772));
#40826=DIRECTION('center_axis',(0.,0.456239332177649,-0.889857107503274));
#40827=DIRECTION('ref_axis',(-1.,0.,0.));
#40828=DIRECTION('',(-1.,0.,0.));
#40829=DIRECTION('',(1.,0.,0.));
#40830=DIRECTION('center_axis',(-0.707106781186551,-0.183012701892219,-0.683012701892216));
#40831=DIRECTION('ref_axis',(-0.694746590606862,0.,0.719254596676407));
#40832=DIRECTION('',(0.,-0.965925826289068,0.258819045102521));
#40833=DIRECTION('',(0.,0.965925826289068,-0.258819045102521));
#40834=DIRECTION('center_axis',(0.,-0.84004340562312,-0.542519194747163));
#40835=DIRECTION('ref_axis',(-1.,0.,0.));
#40836=DIRECTION('',(-1.,0.,0.));
#40837=DIRECTION('',(1.,0.,0.));
#40838=DIRECTION('center_axis',(0.707106781186545,0.661412595302212,-0.25006674864043));
#40839=DIRECTION('ref_axis',(-0.333412439312663,0.,-0.942781069661234));
#40840=DIRECTION('',(0.,-0.353647787425838,-0.935378662600772));
#40841=DIRECTION('',(0.,0.353647787425838,0.935378662600772));
#40842=DIRECTION('center_axis',(0.707106781186552,-0.183012701892218,-0.683012701892215));
#40843=DIRECTION('ref_axis',(-0.694746590606861,0.,-0.719254596676409));
#40844=DIRECTION('',(0.,-0.965925826289068,0.258819045102521));
#40845=DIRECTION('',(0.,0.965925826289068,-0.258819045102521));
#40846=DIRECTION('center_axis',(0.707106781186548,-0.697833484234924,0.114142140686716));
#40847=DIRECTION('ref_axis',(0.159358523666364,0.,-0.987220776186805));
#40848=DIRECTION('',(0.,-0.161421363397452,-0.986885577683101));
#40849=DIRECTION('',(0.,0.161421363397452,0.986885577683101));
#40850=DIRECTION('center_axis',(1.,0.,0.));
#40851=DIRECTION('ref_axis',(0.,0.258819045102521,0.965925826289068));
#40852=DIRECTION('center_axis',(0.,-0.986885577683101,0.161421363397451));
#40853=DIRECTION('ref_axis',(0.,-0.161421363397452,-0.986885577683101));
#40854=DIRECTION('center_axis',(0.,-0.258819045102521,-0.965925826289068));
#40855=DIRECTION('ref_axis',(0.,0.965925826289068,-0.258819045102521));
#40856=DIRECTION('center_axis',(0.5610066315804,-0.65360928088183,-0.508002428407533));
#40857=DIRECTION('ref_axis',(-0.671222048820188,0.,-0.741256339721711));
#40858=DIRECTION('',(0.7055163357783,0.698526492205412,-0.119613710071894));
#40859=DIRECTION('',(0.,-0.613669352377477,0.78956312347564));
#40860=DIRECTION('',(-0.70551633577831,-0.0564971782546714,-0.706438085609211));
#40861=DIRECTION('center_axis',(0.561006631580382,0.440444754748134,-0.700913673242068));
#40862=DIRECTION('ref_axis',(-0.78071899035428,0.,-0.624882275392889));
#40863=DIRECTION('',(0.705516335778309,0.188526073789639,0.683157829093257));
#40864=DIRECTION('',(0.,-0.846707054687368,-0.532059360920041));
#40865=DIRECTION('',(-0.705516335778306,0.697310488411396,-0.126510010281449));
#40866=DIRECTION('center_axis',(-0.561006631580414,-0.653609280881823,-0.508002428407526));
#40867=DIRECTION('ref_axis',(-0.671222048820174,0.,0.741256339721724));
#40868=DIRECTION('',(0.,0.613669352377477,-0.78956312347564));
#40869=DIRECTION('',(0.705516335778301,-0.698526492205416,0.119613710071868));
#40870=DIRECTION('',(-0.705516335778299,0.0564971782546765,0.706438085609222));
#40871=DIRECTION('center_axis',(-0.707106781186551,-0.705126160196076,0.0528875997482672));
#40872=DIRECTION('ref_axis',(0.0745860273602096,0.,0.997214582987344));
#40873=DIRECTION('',(0.,-0.0747943608453598,-0.997198978933359));
#40874=DIRECTION('',(0.,0.0747943608453598,0.997198978933359));
#40875=DIRECTION('center_axis',(-0.561006631580395,0.44044475474813,-0.700913673242061));
#40876=DIRECTION('ref_axis',(-0.78071899035427,0.,0.624882275392901));
#40877=DIRECTION('',(0.705516335778298,-0.188526073789641,-0.683157829093268));
#40878=DIRECTION('',(-0.705516335778309,-0.697310488411389,0.126510010281474));
#40879=DIRECTION('',(0.,0.846707054687368,0.532059360920041));
#40880=DIRECTION('center_axis',(-0.707106781186541,0.680690473905417,-0.191469263158418));
#40881=DIRECTION('ref_axis',(-0.261366100937227,0.,0.965239742903736));
#40882=DIRECTION('',(0.,-0.270778428736216,-0.962641699975202));
#40883=DIRECTION('',(0.,0.270778428736216,0.962641699975202));
#40884=DIRECTION('center_axis',(0.,0.532059360920041,-0.846707054687368));
#40885=DIRECTION('ref_axis',(-1.,0.,0.));
#40886=DIRECTION('',(-1.,0.,0.));
#40887=DIRECTION('',(1.,0.,0.));
#40888=DIRECTION('center_axis',(-0.707106781186554,-0.122787803968972,-0.696364240320013));
#40889=DIRECTION('ref_axis',(-0.701673843159857,0.,0.712498293208676));
#40890=DIRECTION('',(0.,-0.984807753012208,0.173648177666931));
#40891=DIRECTION('',(0.,0.984807753012208,-0.173648177666931));
#40892=DIRECTION('center_axis',(0.,-0.78956312347564,-0.613669352377477));
#40893=DIRECTION('ref_axis',(-1.,0.,0.));
#40894=DIRECTION('',(-1.,0.,0.));
#40895=DIRECTION('',(1.,0.,0.));
#40896=DIRECTION('center_axis',(0.707106781186543,0.680690473905416,-0.191469263158418));
#40897=DIRECTION('ref_axis',(-0.261366100937226,0.,-0.965239742903737));
#40898=DIRECTION('',(0.,-0.270778428736216,-0.962641699975202));
#40899=DIRECTION('',(0.,0.270778428736216,0.962641699975202));
#40900=DIRECTION('center_axis',(0.707106781186542,-0.122787803968974,-0.696364240320024));
#40901=DIRECTION('ref_axis',(-0.701673843159868,0.,-0.712498293208665));
#40902=DIRECTION('',(0.,-0.984807753012208,0.173648177666931));
#40903=DIRECTION('',(0.,0.984807753012208,-0.173648177666931));
#40904=DIRECTION('center_axis',(0.707106781186553,-0.705126160196074,0.0528875997482671));
#40905=DIRECTION('ref_axis',(0.0745860273602093,0.,-0.997214582987344));
#40906=DIRECTION('',(0.,-0.0747943608453598,-0.997198978933359));
#40907=DIRECTION('',(0.,0.0747943608453598,0.997198978933359));
#40908=DIRECTION('center_axis',(1.,0.,0.));
#40909=DIRECTION('ref_axis',(0.,0.173648177666931,0.984807753012208));
#40910=DIRECTION('center_axis',(0.,-0.997198978933359,0.0747943608453598));
#40911=DIRECTION('ref_axis',(0.,-0.0747943608453598,-0.997198978933359));
#40912=DIRECTION('center_axis',(0.,-0.173648177666931,-0.984807753012208));
#40913=DIRECTION('ref_axis',(0.,0.984807753012208,-0.173648177666931));
#40914=DIRECTION('center_axis',(0.707106781186549,-0.707052400311325,-0.00876944775867129));
#40915=DIRECTION('ref_axis',(-0.0124009183210272,0.,-0.999923105656027));
#40916=DIRECTION('',(0.595596683047425,0.588866174870653,0.546352650982962));
#40917=DIRECTION('',(0.,-0.0124018719548353,0.999923093828728));
#40918=DIRECTION('',(0.,0.0124018719548353,-0.999923093828728));
#40919=DIRECTION('',(0.557191914001238,0.564784772718638,-0.608732561538146));
#40920=DIRECTION('center_axis',(1.,0.,0.));
#40921=DIRECTION('ref_axis',(0.,0.0871557427476582,0.996194698091746));
#40922=DIRECTION('',(0.,-0.996194698091746,0.0871557427476582));
#40923=DIRECTION('',(0.,-0.185848282703424,-0.982578452753869));
#40924=DIRECTION('center_axis',(0.707106781186545,-0.0616284167162196,-0.704416026402761));
#40925=DIRECTION('ref_axis',(-0.705757556807954,0.,-0.708453436019945));
#40926=DIRECTION('',(0.557191914001255,-0.564784772718631,0.608732561538138));
#40927=DIRECTION('',(0.,0.996194698091746,-0.0871557427476582));
#40928=DIRECTION('',(0.705516335778315,0.128267547152788,0.696989337290999));
#40929=DIRECTION('center_axis',(0.,-0.733073789207257,-0.680149115692518));
#40930=DIRECTION('ref_axis',(-1.,0.,0.));
#40931=DIRECTION('',(-1.,0.,0.));
#40932=DIRECTION('',(0.,0.680149115692518,-0.733073789207257));
#40933=DIRECTION('',(1.,0.,0.));
#40934=DIRECTION('center_axis',(0.561006631580394,0.499857381275784,-0.659859195364387));
#40935=DIRECTION('ref_axis',(-0.761867344215974,0.,-0.64773308531933));
#40936=DIRECTION('',(0.,-0.797113049929625,-0.603830096659557));
#40937=DIRECTION('',(-0.705516335778304,0.70568308539029,-0.0652539879547269));
#40938=DIRECTION('center_axis',(-0.561006631580409,-0.606846771272559,-0.563035128139331));
#40939=DIRECTION('ref_axis',(-0.708381704532385,0.,0.705829554980374));
#40940=DIRECTION('',(0.705516335778303,-0.706293409755775,0.0582779485356021));
#40941=DIRECTION('',(-0.705516335778301,-0.00528794662205795,0.70867392894792));
#40942=DIRECTION('center_axis',(-0.707106781186549,-0.707052400311325,-0.00876944775867129));
#40943=DIRECTION('ref_axis',(-0.0124009183210272,0.,0.999923105656027));
#40944=DIRECTION('',(0.,0.0124018719548353,-0.999923093828728));
#40945=DIRECTION('',(0.,-0.0124018719548353,0.999923093828728));
#40946=DIRECTION('center_axis',(-0.561006631580407,0.499857381275778,-0.65985919536438));
#40947=DIRECTION('ref_axis',(-0.761867344215964,0.,0.647733085319342));
#40948=DIRECTION('',(0.705516335778305,-0.128267547152786,-0.696989337291011));
#40949=DIRECTION('',(-0.705516335778306,-0.705683085390286,0.0652539879547519));
#40950=DIRECTION('',(0.,0.797113049929625,0.603830096659557));
#40951=DIRECTION('center_axis',(-0.707106781186546,0.694787886990048,-0.131414580971466));
#40952=DIRECTION('ref_axis',(-0.182719541232955,0.,0.983165077314903));
#40953=DIRECTION('',(0.,-0.185848282703424,-0.982578452753869));
#40954=DIRECTION('',(0.,0.185848282703424,0.982578452753869));
#40955=DIRECTION('center_axis',(0.,0.603830096659558,-0.797113049929625));
#40956=DIRECTION('ref_axis',(-1.,0.,0.));
#40957=DIRECTION('',(-1.,0.,0.));
#40958=DIRECTION('',(1.,0.,0.));
#40959=DIRECTION('center_axis',(-0.707106781186556,-0.0616284167162186,
-0.70441602640275));
#40960=DIRECTION('ref_axis',(-0.705757556807943,0.,0.708453436019956));
#40961=DIRECTION('',(0.,-0.996194698091746,0.0871557427476582));
#40962=DIRECTION('',(0.,0.996194698091746,-0.0871557427476582));
#40963=DIRECTION('center_axis',(0.707106781186546,0.694787886990048,-0.131414580971466));
#40964=DIRECTION('ref_axis',(-0.182719541232955,0.,-0.983165077314903));
#40965=DIRECTION('',(0.,0.185848282703424,0.982578452753869));
#40966=DIRECTION('center_axis',(0.,-0.999923093828728,-0.0124018719548353));
#40967=DIRECTION('ref_axis',(0.,0.0124018719548353,-0.999923093828728));
#40968=DIRECTION('center_axis',(0.,-0.0871557427476582,-0.996194698091746));
#40969=DIRECTION('ref_axis',(0.,0.996194698091746,-0.0871557427476582));
#40970=DIRECTION('center_axis',(0.561006631580416,-0.555465791309803,-0.613782790576088));
#40971=DIRECTION('ref_axis',(-0.738128342492238,0.,-0.674660321947023));
#40972=DIRECTION('',(0.705516335778304,0.708685007986272,0.00350134337823141));
#40973=DIRECTION('',(0.,-0.741452533551882,0.671005320760942));
#40974=DIRECTION('',(-0.705516335778299,0.0670328270320436,-0.705516335778311));
#40975=DIRECTION('center_axis',(0.561006631580416,0.555465791309803,-0.613782790576088));
#40976=DIRECTION('ref_axis',(-0.738128342492238,0.,-0.674660321947023));
#40977=DIRECTION('',(0.705516335778299,0.0670328270320439,0.705516335778311));
#40978=DIRECTION('',(0.,-0.741452533551882,-0.671005320760943));
#40979=DIRECTION('',(-0.705516335778305,0.708685007986272,-0.00350134337823141));
#40980=DIRECTION('center_axis',(-0.561006631580428,-0.555465791309797,-0.613782790576082));
#40981=DIRECTION('ref_axis',(-0.738128342492228,0.,0.674660321947035));
#40982=DIRECTION('',(0.,0.741452533551882,-0.671005320760942));
#40983=DIRECTION('',(0.705516335778307,-0.708685007986269,-0.00350134337825647));
#40984=DIRECTION('',(-0.705516335778288,-0.0670328270320448,0.705516335778322));
#40985=DIRECTION('center_axis',(-0.707106781186548,-0.703597544730292,-0.070359754473029));
#40986=DIRECTION('ref_axis',(-0.0990147542976672,0.,0.995085965347403));
#40987=DIRECTION('',(0.,0.0995037190209987,-0.995037190209989));
#40988=DIRECTION('',(0.,-0.0995037190209987,0.995037190209989));
#40989=DIRECTION('center_axis',(-0.561006631580428,0.555465791309797,-0.613782790576082));
#40990=DIRECTION('ref_axis',(-0.738128342492227,0.,0.674660321947035));
#40991=DIRECTION('',(0.705516335778288,-0.0670328270320442,-0.705516335778322));
#40992=DIRECTION('',(-0.705516335778307,-0.708685007986269,0.00350134337825648));
#40993=DIRECTION('',(0.,0.741452533551882,0.671005320760943));
#40994=DIRECTION('center_axis',(-0.707106781186548,0.703597544730292,-0.0703597544730292));
#40995=DIRECTION('ref_axis',(-0.0990147542976674,0.,0.995085965347403));
#40996=DIRECTION('',(0.,-0.0995037190209989,-0.995037190209989));
#40997=DIRECTION('',(0.,0.0995037190209989,0.995037190209989));
#40998=DIRECTION('center_axis',(0.,0.671005320760943,-0.741452533551882));
#40999=DIRECTION('ref_axis',(-1.,0.,0.));
#41000=DIRECTION('',(-1.,0.,0.));
#41001=DIRECTION('',(1.,0.,0.));
#41002=DIRECTION('center_axis',(-0.707106781186565,-8.65956056235472E-17,
-0.70710678118653));
#41003=DIRECTION('ref_axis',(-0.70710678118653,0.,0.707106781186565));
#41004=DIRECTION('',(0.,-1.,1.22464679914735E-16));
#41005=DIRECTION('',(0.,1.,-1.22464679914735E-16));
#41006=DIRECTION('center_axis',(0.,-0.671005320760942,-0.741452533551882));
#41007=DIRECTION('ref_axis',(-1.,0.,0.));
#41008=DIRECTION('',(-1.,0.,0.));
#41009=DIRECTION('',(1.,0.,0.));
#41010=DIRECTION('center_axis',(0.707106781186548,0.703597544730291,-0.0703597544730291));
#41011=DIRECTION('ref_axis',(-0.0990147542976671,0.,-0.995085965347403));
#41012=DIRECTION('',(0.,-0.0995037190209989,-0.995037190209989));
#41013=DIRECTION('',(0.,0.0995037190209989,0.995037190209989));
#41014=DIRECTION('center_axis',(0.707106781186554,-8.65956056235486E-17,
-0.707106781186541));
#41015=DIRECTION('ref_axis',(-0.707106781186541,0.,-0.707106781186554));
#41016=DIRECTION('',(0.,-1.,1.22464679914735E-16));
#41017=DIRECTION('',(0.,1.,-1.22464679914735E-16));
#41018=DIRECTION('center_axis',(0.707106781186549,-0.70359754473029,-0.0703597544730288));
#41019=DIRECTION('ref_axis',(-0.0990147542976667,0.,-0.995085965347403));
#41020=DIRECTION('',(0.,0.0995037190209987,-0.995037190209989));
#41021=DIRECTION('',(0.,-0.0995037190209987,0.995037190209989));
#41022=DIRECTION('center_axis',(1.,0.,0.));
#41023=DIRECTION('ref_axis',(0.,1.22464679914735E-16,1.));
#41024=DIRECTION('center_axis',(0.,-0.995037190209989,-0.0995037190209987));
#41025=DIRECTION('ref_axis',(0.,0.0995037190209987,-0.995037190209989));
#41026=DIRECTION('center_axis',(0.,-1.22464679914735E-16,-1.));
#41027=DIRECTION('ref_axis',(0.,1.,-1.22464679914735E-16));
#41028=DIRECTION('center_axis',(0.561006631580408,0.606846771272561,-0.56303512813933));
#41029=DIRECTION('ref_axis',(-0.708381704532385,0.,-0.705829554980374));
#41030=DIRECTION('',(0.7055163357783,0.00528794662205797,0.708673928947921));
#41031=DIRECTION('',(0.,-0.680149115692518,-0.733073789207257));
#41032=DIRECTION('',(-0.705516335778304,0.706293409755774,0.0582779485356025));
#41033=DIRECTION('center_axis',(0.,0.733073789207257,-0.680149115692518));
#41034=DIRECTION('ref_axis',(-1.,0.,0.));
#41035=DIRECTION('',(0.55719191400124,0.564784772718638,0.608732561538145));
#41036=DIRECTION('',(1.,0.,0.));
#41037=DIRECTION('',(-1.,0.,0.));
#41038=DIRECTION('',(-0.557191914001263,0.564784772718627,0.608732561538133));
#41039=DIRECTION('center_axis',(0.707106781186549,0.707052400311325,-0.00876944775867146));
#41040=DIRECTION('ref_axis',(-0.0124009183210275,0.,-0.999923105656027));
#41041=DIRECTION('',(0.,-0.0124018719548356,-0.999923093828728));
#41042=DIRECTION('',(0.,0.0124018719548356,0.999923093828728));
#41043=DIRECTION('center_axis',(0.561006631580409,-0.499857381275773,-0.659859195364382));
#41044=DIRECTION('ref_axis',(-0.761867344215964,0.,-0.647733085319342));
#41045=DIRECTION('',(0.705516335778303,0.705683085390289,0.0652539879547519));
#41046=DIRECTION('',(0.,-0.79711304992963,0.603830096659552));
#41047=DIRECTION('',(-0.705516335778302,0.128267547152795,-0.696989337291011));
#41048=DIRECTION('center_axis',(0.,-0.603830096659552,-0.79711304992963));
#41049=DIRECTION('ref_axis',(-1.,0.,0.));
#41050=DIRECTION('',(0.557191914001257,0.661909722954172,-0.501410699557107));
#41051=DIRECTION('',(1.,0.,0.));
#41052=DIRECTION('',(-1.,0.,0.));
#41053=DIRECTION('',(-0.557191914001246,0.661909722954178,-0.501410699557111));
#41054=DIRECTION('center_axis',(0.707106781186545,0.0616284167162194,-0.704416026402761));
#41055=DIRECTION('ref_axis',(-0.705757556807954,0.,-0.708453436019945));
#41056=DIRECTION('',(0.,-0.996194698091746,-0.0871557427476579));
#41057=DIRECTION('',(0.,0.996194698091746,0.0871557427476579));
#41058=DIRECTION('center_axis',(0.707106781186549,-0.694787886990045,-0.131414580971465));
#41059=DIRECTION('ref_axis',(-0.182719541232953,0.,-0.983165077314903));
#41060=DIRECTION('',(0.,0.185848282703424,-0.98257845275387));
#41061=DIRECTION('',(0.,-0.185848282703424,0.98257845275387));
#41062=DIRECTION('center_axis',(-0.707106781186548,0.707052400311326,-0.00876944775867148));
#41063=DIRECTION('ref_axis',(-0.0124009183210275,0.,0.999923105656027));
#41064=DIRECTION('',(-0.595596683047425,-0.58886617487065,0.546352650982966));
#41065=DIRECTION('',(0.,0.0124018719548356,0.999923093828728));
#41066=DIRECTION('',(0.,-0.0124018719548356,-0.999923093828728));
#41067=DIRECTION('center_axis',(0.,0.0871557427476579,-0.996194698091746));
#41068=DIRECTION('ref_axis',(0.,0.996194698091746,0.0871557427476579));
#41069=DIRECTION('',(0.,-0.996194698091746,-0.0871557427476579));
#41070=DIRECTION('center_axis',(-0.707106781186531,0.0616284167162207,-0.704416026402775));
#41071=DIRECTION('ref_axis',(-0.705757556807969,0.,0.708453436019931));
#41072=DIRECTION('',(0.59559668304743,-0.485046832292573,-0.640307864722775));
#41073=DIRECTION('',(0.,0.996194698091746,0.0871557427476579));
#41074=DIRECTION('center_axis',(-0.707106781186548,-0.694787886990046,-0.131414580971466));
#41075=DIRECTION('ref_axis',(-0.182719541232954,0.,0.983165077314903));
#41076=DIRECTION('',(0.,-0.185848282703424,0.98257845275387));
#41077=DIRECTION('',(0.,0.185848282703424,-0.98257845275387));
#41078=DIRECTION('center_axis',(0.,-0.98257845275387,-0.185848282703424));
#41079=DIRECTION('ref_axis',(0.,0.185848282703424,-0.98257845275387));
#41080=DIRECTION('center_axis',(0.,0.999923093828728,-0.0124018719548356));
#41081=DIRECTION('ref_axis',(0.,0.0124018719548356,0.999923093828728));
#41082=DIRECTION('center_axis',(0.561006631580393,-0.440444754748104,-0.700913673242079));
#41083=DIRECTION('ref_axis',(-0.780718990354279,0.,-0.62488227539289));
#41084=DIRECTION('',(0.705516335778308,0.697310488411385,0.1265100102815));
#41085=DIRECTION('',(0.,-0.846707054687388,0.532059360920009));
#41086=DIRECTION('',(-0.705516335778307,0.188526073789657,-0.683157829093255));
#41087=DIRECTION('center_axis',(0.561006631580402,0.653609280881817,-0.508002428407548));
#41088=DIRECTION('ref_axis',(-0.671222048820198,0.,-0.741256339721703));
#41089=DIRECTION('',(0.70551633577831,-0.0564971782546651,0.706438085609211));
#41090=DIRECTION('',(0.,-0.613669352377496,-0.789563123475625));
#41091=DIRECTION('',(-0.705516335778302,0.698526492205414,0.119613710071869));
#41092=DIRECTION('center_axis',(-0.56100663158039,-0.440444754748103,-0.700913673242082));
#41093=DIRECTION('ref_axis',(-0.780718990354282,0.,0.624882275392886));
#41094=DIRECTION('',(0.,0.846707054687388,-0.532059360920009));
#41095=DIRECTION('',(0.705516335778313,-0.697310488411381,-0.1265100102815));
#41096=DIRECTION('',(-0.705516335778307,-0.188526073789662,0.683157829093252));
#41097=DIRECTION('center_axis',(-0.707106781186538,-0.68069047390542,-0.191469263158418));
#41098=DIRECTION('ref_axis',(-0.261366100937229,0.,0.965239742903736));
#41099=DIRECTION('',(0.,0.270778428736215,-0.962641699975202));
#41100=DIRECTION('',(0.,-0.270778428736215,0.962641699975202));
#41101=DIRECTION('center_axis',(-0.561006631580396,0.65360928088182,-0.50800242840755));
#41102=DIRECTION('ref_axis',(-0.671222048820203,0.,0.741256339721698));
#41103=DIRECTION('',(0.705516335778312,0.0564971782546587,-0.70643808560921));
#41104=DIRECTION('',(-0.705516335778307,-0.69852649220541,-0.119613710071869));
#41105=DIRECTION('',(0.,0.613669352377496,0.789563123475625));
#41106=DIRECTION('center_axis',(-0.707106781186545,0.705126160196082,0.0528875997482672));
#41107=DIRECTION('ref_axis',(0.0745860273602103,0.,0.997214582987344));
#41108=DIRECTION('',(0.,0.0747943608453591,-0.997198978933359));
#41109=DIRECTION('',(0.,-0.0747943608453591,0.997198978933359));
#41110=DIRECTION('center_axis',(0.,0.789563123475625,-0.613669352377496));
#41111=DIRECTION('ref_axis',(-1.,0.,0.));
#41112=DIRECTION('',(-1.,0.,0.));
#41113=DIRECTION('',(1.,0.,0.));
#41114=DIRECTION('center_axis',(-0.707106781186541,0.122787803968974,-0.696364240320025));
#41115=DIRECTION('ref_axis',(-0.701673843159869,0.,0.712498293208664));
#41116=DIRECTION('',(0.,-0.984807753012208,-0.17364817766693));
#41117=DIRECTION('',(0.,0.984807753012208,0.17364817766693));
#41118=DIRECTION('center_axis',(0.,-0.532059360920009,-0.846707054687388));
#41119=DIRECTION('ref_axis',(-1.,0.,0.));
#41120=DIRECTION('',(-1.,0.,0.));
#41121=DIRECTION('',(1.,0.,0.));
#41122=DIRECTION('center_axis',(0.70710678118655,0.705126160196078,0.0528875997482669));
#41123=DIRECTION('ref_axis',(0.0745860273602093,0.,-0.997214582987344));
#41124=DIRECTION('',(0.,0.0747943608453591,-0.997198978933359));
#41125=DIRECTION('',(0.,-0.0747943608453591,0.997198978933359));
#41126=DIRECTION('center_axis',(0.707106781186543,0.122787803968973,-0.696364240320023));
#41127=DIRECTION('ref_axis',(-0.701673843159868,0.,-0.712498293208665));
#41128=DIRECTION('',(0.,-0.984807753012208,-0.17364817766693));
#41129=DIRECTION('',(0.,0.984807753012208,0.17364817766693));
#41130=DIRECTION('center_axis',(0.707106781186543,-0.680690473905416,-0.191469263158417));
#41131=DIRECTION('ref_axis',(-0.261366100937225,0.,-0.965239742903737));
#41132=DIRECTION('',(0.,0.270778428736215,-0.962641699975202));
#41133=DIRECTION('',(0.,-0.270778428736215,0.962641699975202));
#41134=DIRECTION('center_axis',(1.,0.,0.));
#41135=DIRECTION('ref_axis',(0.,-0.17364817766693,0.984807753012208));
#41136=DIRECTION('center_axis',(0.,-0.962641699975202,-0.270778428736215));
#41137=DIRECTION('ref_axis',(0.,0.270778428736215,-0.962641699975202));
#41138=DIRECTION('center_axis',(0.,0.17364817766693,-0.984807753012208));
#41139=DIRECTION('ref_axis',(0.,0.984807753012208,0.17364817766693));
#41140=DIRECTION('center_axis',(0.561006631580395,-0.37768007768897,-0.736633774843153));
#41141=DIRECTION('ref_axis',(-0.795555689966288,0.,-0.605880470193802));
#41142=DIRECTION('',(0.705516335778309,0.683630937568086,0.186803215041197));
#41143=DIRECTION('',(0.,-0.889857107503286,0.456239332177625));
#41144=DIRECTION('',(-0.705516335778301,0.247349803169823,-0.664127077314131));
#41145=DIRECTION('center_axis',(0.56100663158043,0.695397429203484,-0.449103523455299));
#41146=DIRECTION('ref_axis',(-0.624948053917868,0.,-0.78066633711482));
#41147=DIRECTION('',(0.705516335778292,-0.117852325490953,0.698825821880064));
#41148=DIRECTION('',(0.,-0.542519194747174,-0.840043405623113));
#41149=DIRECTION('',(-0.705516335778305,0.685443366267552,0.18003913904971));
#41150=DIRECTION('center_axis',(-0.561006631580394,-0.37768007768897,-0.736633774843153));
#41151=DIRECTION('ref_axis',(-0.795555689966289,0.,0.605880470193801));
#41152=DIRECTION('',(0.,0.889857107503286,-0.456239332177625));
#41153=DIRECTION('',(0.705516335778311,-0.683630937568085,-0.186803215041197));
#41154=DIRECTION('',(-0.705516335778303,-0.247349803169823,0.664127077314129));
#41155=DIRECTION('center_axis',(-0.707106781186544,-0.661412595302213,-0.25006674864043));
#41156=DIRECTION('ref_axis',(-0.333412439312664,0.,0.942781069661233));
#41157=DIRECTION('',(0.,0.353647787425838,-0.935378662600772));
#41158=DIRECTION('',(0.,-0.353647787425838,0.935378662600772));
#41159=DIRECTION('center_axis',(-0.561006631580425,0.695397429203487,-0.449103523455301));
#41160=DIRECTION('ref_axis',(-0.624948053917874,0.,0.780666337114815));
#41161=DIRECTION('',(0.705516335778293,0.117852325490952,-0.698825821880063));
#41162=DIRECTION('',(-0.70551633577831,-0.685443366267547,-0.18003913904971));
#41163=DIRECTION('',(0.,0.542519194747174,0.840043405623113));
#41164=DIRECTION('center_axis',(-0.707106781186546,0.697833484234925,0.114142140686716));
#41165=DIRECTION('ref_axis',(0.159358523666365,0.,0.987220776186805));
#41166=DIRECTION('',(0.,0.161421363397451,-0.986885577683101));
#41167=DIRECTION('',(0.,-0.161421363397451,0.986885577683101));
#41168=DIRECTION('center_axis',(0.,0.840043405623113,-0.542519194747174));
#41169=DIRECTION('ref_axis',(-1.,0.,0.));
#41170=DIRECTION('',(-1.,0.,0.));
#41171=DIRECTION('',(1.,0.,0.));
#41172=DIRECTION('center_axis',(-0.707106781186552,0.183012701892218,-0.683012701892215));
#41173=DIRECTION('ref_axis',(-0.694746590606862,0.,0.719254596676408));
#41174=DIRECTION('',(0.,-0.965925826289068,-0.258819045102521));
#41175=DIRECTION('',(0.,0.965925826289068,0.258819045102521));
#41176=DIRECTION('center_axis',(0.,-0.456239332177625,-0.889857107503286));
#41177=DIRECTION('ref_axis',(-1.,0.,0.));
#41178=DIRECTION('',(-1.,0.,0.));
#41179=DIRECTION('',(1.,0.,0.));
#41180=DIRECTION('center_axis',(0.707106781186551,0.697833484234921,0.114142140686715));
#41181=DIRECTION('ref_axis',(0.159358523666362,0.,-0.987220776186805));
#41182=DIRECTION('',(0.,0.161421363397451,-0.986885577683101));
#41183=DIRECTION('',(0.,-0.161421363397451,0.986885577683101));
#41184=DIRECTION('center_axis',(0.707106781186553,0.183012701892218,-0.683012701892214));
#41185=DIRECTION('ref_axis',(-0.69474659060686,0.,-0.719254596676409));
#41186=DIRECTION('',(0.,-0.965925826289068,-0.258819045102521));
#41187=DIRECTION('',(0.,0.965925826289068,0.258819045102521));
#41188=DIRECTION('center_axis',(0.707106781186545,-0.661412595302212,-0.25006674864043));
#41189=DIRECTION('ref_axis',(-0.333412439312663,0.,-0.942781069661234));
#41190=DIRECTION('',(0.,0.353647787425838,-0.935378662600772));
#41191=DIRECTION('',(0.,-0.353647787425838,0.935378662600772));
#41192=DIRECTION('center_axis',(1.,0.,0.));
#41193=DIRECTION('ref_axis',(0.,-0.258819045102521,0.965925826289068));
#41194=DIRECTION('center_axis',(0.,-0.935378662600772,-0.353647787425838));
#41195=DIRECTION('ref_axis',(0.,0.353647787425838,-0.935378662600772));
#41196=DIRECTION('center_axis',(0.,0.258819045102521,-0.965925826289068));
#41197=DIRECTION('ref_axis',(0.,0.965925826289068,0.258819045102521));
#41198=DIRECTION('center_axis',(0.707106781186549,-0.637100967476913,-0.306761075170856));
#41199=DIRECTION('ref_axis',(-0.397987666358442,0.,-0.917390765937047));
#41200=DIRECTION('',(0.595596683047422,0.302795392151909,0.744029261275711));
#41201=DIRECTION('',(0.,-0.433825672914778,0.900996828806872));
#41202=DIRECTION('',(0.,0.433825672914778,-0.900996828806872));
#41203=DIRECTION('',(0.557191914001242,0.769130334536841,-0.313010701840814));
#41204=DIRECTION('center_axis',(1.,0.,0.));
#41205=DIRECTION('ref_axis',(0.,-0.342020143325669,0.939692620785909));
#41206=DIRECTION('',(0.,-0.939692620785909,-0.342020143325669));
#41207=DIRECTION('',(0.,0.246819851905204,-0.96906138128887));
#41208=DIRECTION('center_axis',(0.707106781186551,0.241844762647974,-0.664463024388671));
#41209=DIRECTION('ref_axis',(-0.684791078771732,0.,-0.728739444818686));
#41210=DIRECTION('',(0.557191914001232,-0.769130334536847,0.313010701840817));
#41211=DIRECTION('',(0.,0.939692620785909,0.342020143325669));
#41212=DIRECTION('',(0.705516335778307,-0.178310545369053,0.685895071683813));
#41213=DIRECTION('center_axis',(0.,-0.376947046632547,-0.926234810420662));
#41214=DIRECTION('ref_axis',(-1.,0.,0.));
#41215=DIRECTION('',(-1.,0.,0.));
#41216=DIRECTION('',(0.,0.926234810420662,-0.376947046632547));
#41217=DIRECTION('',(1.,0.,0.));
#41218=DIRECTION('center_axis',(0.561006631580392,0.73189318319651,-0.386786669513444));
#41219=DIRECTION('ref_axis',(-0.567619122871716,0.,-0.823291279773048));
#41220=DIRECTION('',(0.,-0.467240138462762,-0.884130450221741));
#41221=DIRECTION('',(-0.705516335778315,0.667143602430337,0.239094361468882));
#41222=DIRECTION('center_axis',(-0.561006631580397,-0.312041027189172,-0.766747648626028));
#41223=DIRECTION('ref_axis',(-0.807044487383583,0.,0.590490639539502));
#41224=DIRECTION('',(0.705516335778304,-0.66474854250226,-0.245674734539547));
#41225=DIRECTION('',(-0.705516335778316,-0.304291051193919,0.640041917465754));
#41226=DIRECTION('center_axis',(-0.707106781186553,-0.637100967476909,-0.306761075170854));
#41227=DIRECTION('ref_axis',(-0.397987666358438,0.,0.917390765937049));
#41228=DIRECTION('',(0.,0.433825672914778,-0.900996828806872));
#41229=DIRECTION('',(0.,-0.433825672914778,0.900996828806872));
#41230=DIRECTION('center_axis',(-0.561006631580381,0.731893183196516,-0.386786669513448));
#41231=DIRECTION('ref_axis',(-0.567619122871728,0.,0.82329127977304));
#41232=DIRECTION('',(0.70551633577832,0.178310545369055,-0.685895071683798));
#41233=DIRECTION('',(-0.705516335778313,-0.667143602430331,-0.239094361468905));
#41234=DIRECTION('',(0.,0.467240138462762,0.884130450221741));
#41235=DIRECTION('center_axis',(-0.707106781186533,0.685229874095377,0.174527991013633));
#41236=DIRECTION('ref_axis',(0.239628661022767,0.,0.970864617141049));
#41237=DIRECTION('',(0.,0.246819851905204,-0.96906138128887));
#41238=DIRECTION('',(0.,-0.246819851905204,0.96906138128887));
#41239=DIRECTION('center_axis',(0.,0.884130450221741,-0.467240138462762));
#41240=DIRECTION('ref_axis',(0.,0.467240138462762,0.884130450221741));
#41241=DIRECTION('',(-1.,0.,0.));
#41242=DIRECTION('',(1.,0.,0.));
#41243=DIRECTION('center_axis',(-0.707106781186536,0.241844762647979,-0.664463024388686));
#41244=DIRECTION('ref_axis',(-0.684791078771748,0.,0.728739444818671));
#41245=DIRECTION('',(0.,-0.939692620785909,-0.342020143325669));
#41246=DIRECTION('',(0.,0.939692620785909,0.342020143325669));
#41247=DIRECTION('center_axis',(0.707106781186534,0.685229874095376,0.174527991013633));
#41248=DIRECTION('ref_axis',(0.239628661022766,0.,-0.970864617141049));
#41249=DIRECTION('',(0.,-0.246819851905204,0.96906138128887));
#41250=DIRECTION('center_axis',(0.,-0.900996828806872,-0.433825672914778));
#41251=DIRECTION('ref_axis',(0.,0.433825672914778,-0.900996828806872));
#41252=DIRECTION('center_axis',(0.,0.342020143325669,-0.939692620785908));
#41253=DIRECTION('ref_axis',(0.,0.939692620785909,0.342020143325669));
#41254=DIRECTION('center_axis',(0.561006631580397,-0.244027156056947,-0.791026109827972));
#41255=DIRECTION('ref_axis',(-0.815685591418259,0.,-0.578495476173017));
#41256=DIRECTION('',(0.705516335778307,0.640807009641837,0.302676520965598));
#41257=DIRECTION('',(0.,-0.955563307154868,0.294785966455752));
#41258=DIRECTION('',(-0.705516335778309,0.358916460582513,-0.611085652157592));
#41259=DIRECTION('center_axis',(0.561006631580416,0.762818788136174,-0.321526135468415));
#41260=DIRECTION('ref_axis',(-0.497247150959857,0.,-0.867608938901799));
#41261=DIRECTION('',(0.705516335778299,-0.23741171433011,0.667744245837282));
#41262=DIRECTION('',(0.,-0.388405102597364,-0.921488728241605));
#41263=DIRECTION('',(-0.705516335778294,0.643766472946353,0.2963299314281));
#41264=DIRECTION('center_axis',(-0.561006631580414,-0.244027156056941,-0.791026109827963));
#41265=DIRECTION('ref_axis',(-0.815685591418248,0.,0.578495476173032));
#41266=DIRECTION('',(0.,0.955563307154868,-0.294785966455752));
#41267=DIRECTION('',(0.705516335778309,-0.640807009641824,-0.302676520965623));
#41268=DIRECTION('',(-0.705516335778296,-0.358916460582518,0.611085652157604));
#41269=DIRECTION('center_axis',(-0.707106781186546,-0.607940616597039,-0.361120764691834));
#41270=DIRECTION('ref_axis',(-0.454822071931222,0.,0.890582327965354));
#41271=DIRECTION('',(0.,0.510701883081733,-0.859757865108992));
#41272=DIRECTION('',(0.,-0.510701883081733,0.859757865108992));
#41273=DIRECTION('center_axis',(-0.561006631580431,0.762818788136165,-0.321526135468411));
#41274=DIRECTION('ref_axis',(-0.497247150959842,0.,0.867608938901807));
#41275=DIRECTION('',(0.705516335778287,0.237411714330117,-0.667744245837293));
#41276=DIRECTION('',(-0.705516335778295,-0.643766472946363,-0.296329931428075));
#41277=DIRECTION('',(0.,0.388405102597364,0.921488728241605));
#41278=DIRECTION('center_axis',(-0.707106781186556,0.667411250860817,0.233585577946044));
#41279=DIRECTION('ref_axis',(0.313668483594034,0.,0.949532559947166));
#41280=DIRECTION('',(0.,0.330339892306057,-0.943862042647771));
#41281=DIRECTION('',(0.,-0.330339892306057,0.943862042647771));
#41282=DIRECTION('center_axis',(0.,0.921488728241605,-0.388405102597364));
#41283=DIRECTION('ref_axis',(0.,0.388405102597364,0.921488728241605));
#41284=DIRECTION('',(-1.,0.,0.));
#41285=DIRECTION('',(1.,0.,0.));
#41286=DIRECTION('center_axis',(-0.707106781186564,0.298836238730113,-0.640856382055774));
#41287=DIRECTION('ref_axis',(-0.671542934237801,0.,0.740965645273304));
#41288=DIRECTION('',(0.,-0.90630778703665,-0.422618261740699));
#41289=DIRECTION('',(0.,0.90630778703665,0.422618261740699));
#41290=DIRECTION('center_axis',(0.,-0.294785966455752,-0.955563307154868));
#41291=DIRECTION('ref_axis',(-1.,0.,0.));
#41292=DIRECTION('',(-1.,0.,0.));
#41293=DIRECTION('',(1.,0.,0.));
#41294=DIRECTION('center_axis',(0.707106781186557,0.667411250860816,0.233585577946044));
#41295=DIRECTION('ref_axis',(0.313668483594033,0.,-0.949532559947167));
#41296=DIRECTION('',(0.,0.330339892306057,-0.943862042647771));
#41297=DIRECTION('',(0.,-0.330339892306057,0.943862042647771));
#41298=DIRECTION('center_axis',(0.707106781186551,0.298836238730118,-0.640856382055785));
#41299=DIRECTION('ref_axis',(-0.671542934237814,0.,-0.740965645273293));
#41300=DIRECTION('',(0.,-0.90630778703665,-0.422618261740699));
#41301=DIRECTION('',(0.,0.90630778703665,0.422618261740699));
#41302=DIRECTION('center_axis',(0.707106781186547,-0.607940616597037,-0.361120764691833));
#41303=DIRECTION('ref_axis',(-0.454822071931221,0.,-0.890582327965355));
#41304=DIRECTION('',(0.,0.510701883081733,-0.859757865108992));
#41305=DIRECTION('',(0.,-0.510701883081733,0.859757865108992));
#41306=DIRECTION('center_axis',(1.,0.,0.));
#41307=DIRECTION('ref_axis',(0.,-0.422618261740699,0.90630778703665));
#41308=DIRECTION('center_axis',(0.,-0.859757865108992,-0.510701883081733));
#41309=DIRECTION('ref_axis',(0.,0.510701883081733,-0.859757865108992));
#41310=DIRECTION('center_axis',(0.,0.422618261740699,-0.90630778703665));
#41311=DIRECTION('ref_axis',(0.,0.90630778703665,0.422618261740699));
#41312=DIRECTION('center_axis',(0.561006631580407,0.787938881495568,-0.253818593389688));
#41313=DIRECTION('ref_axis',(-0.412208150462316,0.,-0.9110896995864));
#41314=DIRECTION('',(0.705516335778306,-0.29470603679192,0.644511483084942));
#41315=DIRECTION('',(0.,-0.306614069375781,-0.951833920629446));
#41316=DIRECTION('',(-0.7055163357783,0.615489891886393,0.351310251680245));
#41317=DIRECTION('center_axis',(0.,0.951833920629447,-0.306614069375781));
#41318=DIRECTION('ref_axis',(0.,0.306614069375781,0.951833920629446));
#41319=DIRECTION('',(0.557191914001238,0.254607340492412,0.790387419648756));
#41320=DIRECTION('',(1.,0.,0.));
#41321=DIRECTION('',(-1.,0.,0.));
#41322=DIRECTION('',(-0.557191914001261,0.254607340492407,0.790387419648741));
#41323=DIRECTION('center_axis',(0.707106781186551,0.644513225013302,0.290865437587465));
#41324=DIRECTION('ref_axis',(0.380418570543385,0.,-0.924814419862562));
#41325=DIRECTION('',(0.,0.41134584666178,-0.911479343942639));
#41326=DIRECTION('',(0.,-0.41134584666178,0.911479343942639));
#41327=DIRECTION('center_axis',(0.561006631580406,-0.174156090919475,-0.809284384699504));
#41328=DIRECTION('ref_axis',(-0.821843752318937,0.,-0.569712951208177));
#41329=DIRECTION('',(0.705516335778312,0.611988548508171,0.357374756306047));
#41330=DIRECTION('',(0.,-0.977619390136734,0.210381387077564));
#41331=DIRECTION('',(-0.705516335778298,0.410810298986407,-0.577478656052899));
#41332=DIRECTION('center_axis',(0.,-0.210381387077564,-0.977619390136734));
#41333=DIRECTION('ref_axis',(-1.,0.,0.));
#41334=DIRECTION('',(0.557191914001257,0.811799254493649,-0.174697284967946));
#41335=DIRECTION('',(1.,0.,0.));
#41336=DIRECTION('',(-1.,0.,0.));
#41337=DIRECTION('',(-0.557191914001251,0.811799254493653,-0.174697284967946));
#41338=DIRECTION('center_axis',(0.707106781186549,0.353553390593273,-0.612372435695794));
#41339=DIRECTION('ref_axis',(-0.654653670707976,0.,-0.755928946018455));
#41340=DIRECTION('',(0.,-0.866025403784439,-0.5));
#41341=DIRECTION('',(0.,0.866025403784439,0.5));
#41342=DIRECTION('center_axis',(0.707106781186542,-0.574153470540281,-0.412732107142828));
#41343=DIRECTION('ref_axis',(-0.504101701135475,0.,-0.863644298836228));
#41344=DIRECTION('',(0.,0.583691343548208,-0.81197562492164));
#41345=DIRECTION('',(0.,-0.583691343548208,0.81197562492164));
#41346=DIRECTION('center_axis',(-0.707106781186549,0.644513225013304,0.290865437587466));
#41347=DIRECTION('ref_axis',(0.380418570543387,0.,0.924814419862562));
#41348=DIRECTION('',(-0.595596683047435,-0.764592607463601,0.246298062832224));
#41349=DIRECTION('',(0.,-0.41134584666178,0.911479343942639));
#41350=DIRECTION('',(0.,0.41134584666178,-0.911479343942639));
#41351=DIRECTION('center_axis',(0.,0.5,-0.866025403784439));
#41352=DIRECTION('ref_axis',(0.,0.866025403784439,0.5));
#41353=DIRECTION('',(0.,-0.866025403784439,-0.5));
#41354=DIRECTION('center_axis',(-0.707106781186533,0.353553390593281,-0.612372435695807));
#41355=DIRECTION('ref_axis',(-0.654653670707993,0.,0.755928946018441));
#41356=DIRECTION('',(0.595596683047433,-0.168995924416179,-0.785305653025379));
#41357=DIRECTION('',(0.,0.866025403784439,0.5));
#41358=DIRECTION('center_axis',(-0.707106781186541,-0.574153470540282,-0.412732107142829));
#41359=DIRECTION('ref_axis',(-0.504101701135477,0.,0.863644298836227));
#41360=DIRECTION('',(0.,-0.583691343548208,0.81197562492164));
#41361=DIRECTION('',(0.,0.583691343548208,-0.81197562492164));
#41362=DIRECTION('center_axis',(0.,-0.81197562492164,-0.583691343548208));
#41363=DIRECTION('ref_axis',(0.,0.583691343548208,-0.81197562492164));
#41364=DIRECTION('center_axis',(0.,0.911479343942639,0.41134584666178));
#41365=DIRECTION('ref_axis',(0.,-0.41134584666178,0.911479343942639));
#41366=DIRECTION('center_axis',(0.561006631580388,-0.1029595927718,-0.821383516744214));
#41367=DIRECTION('ref_axis',(-0.825772049781974,0.,-0.564004008672702));
#41368=DIRECTION('',(0.705516335778307,0.578512484991612,0.409353153962177));
#41369=DIRECTION('',(0.,-0.992235199256928,0.124375678311978));
#41370=DIRECTION('',(-0.705516335778309,0.459577622960955,-0.539476698684482));
#41371=DIRECTION('center_axis',(0.561006631580405,0.807062284196269,-0.184179338555412));
#41372=DIRECTION('ref_axis',(-0.311921838389586,0.,-0.95010776585378));
#41373=DIRECTION('',(0.705516335778315,-0.349757468365408,0.616373598779637));
#41374=DIRECTION('',(0.,-0.22248951794762,-0.974935082148261));
#41375=DIRECTION('',(-0.7055163357783,0.582529061106229,0.403616888790171));
#41376=DIRECTION('center_axis',(-0.561006631580387,-0.102959592771799,-0.821383516744215));
#41377=DIRECTION('ref_axis',(-0.825772049781975,0.,0.5640040086727));
#41378=DIRECTION('',(0.,0.992235199256928,-0.124375678311978));
#41379=DIRECTION('',(0.705516335778308,-0.578512484991611,-0.409353153962176));
#41380=DIRECTION('',(-0.70551633577831,-0.459577622960954,0.539476698684481));
#41381=DIRECTION('center_axis',(-0.707106781186546,-0.535996669889361,-0.461202309044001));
#41382=DIRECTION('ref_axis',(-0.546305769586289,0.,0.83758582015023));
#41383=DIRECTION('',(0.,0.652238560447812,-0.758013759944347));
#41384=DIRECTION('',(0.,-0.652238560447812,0.758013759944347));
#41385=DIRECTION('center_axis',(-0.561006631580403,0.80706228419627,-0.184179338555412));
#41386=DIRECTION('ref_axis',(-0.311921838389587,0.,0.95010776585378));
#41387=DIRECTION('',(0.705516335778317,0.349757468365407,-0.616373598779635));
#41388=DIRECTION('',(-0.705516335778301,-0.582529061106227,-0.40361688879017));
#41389=DIRECTION('',(0.,0.22248951794762,0.974935082148261));
#41390=DIRECTION('center_axis',(-0.707106781186545,0.616710064355711,0.345931635619494));
#41391=DIRECTION('ref_axis',(0.439451044888515,0.,0.898266541259549));
#41392=DIRECTION('',(0.,0.489221210746995,-0.872159737063827));
#41393=DIRECTION('',(0.,-0.489221210746995,0.872159737063827));
#41394=DIRECTION('center_axis',(0.,0.974935082148261,-0.22248951794762));
#41395=DIRECTION('ref_axis',(0.,0.22248951794762,0.974935082148261));
#41396=DIRECTION('',(-1.,0.,0.));
#41397=DIRECTION('',(1.,0.,0.));
#41398=DIRECTION('center_axis',(-0.707106781186546,0.40557978767264,-0.579227965339571));
#41399=DIRECTION('ref_axis',(-0.633687274224644,0.,0.773589321594954));
#41400=DIRECTION('',(0.,-0.819152044288992,-0.573576436351046));
#41401=DIRECTION('',(0.,0.819152044288992,0.573576436351046));
#41402=DIRECTION('center_axis',(0.,-0.124375678311978,-0.992235199256928));
#41403=DIRECTION('ref_axis',(-1.,0.,0.));
#41404=DIRECTION('',(-1.,0.,0.));
#41405=DIRECTION('',(1.,0.,0.));
#41406=DIRECTION('center_axis',(0.707106781186546,0.61671006435571,0.345931635619494));
#41407=DIRECTION('ref_axis',(0.439451044888513,0.,-0.898266541259549));
#41408=DIRECTION('',(0.,0.489221210746995,-0.872159737063827));
#41409=DIRECTION('',(0.,-0.489221210746995,0.872159737063827));
#41410=DIRECTION('center_axis',(0.707106781186547,0.405579787672639,-0.57922796533957));
#41411=DIRECTION('ref_axis',(-0.633687274224642,0.,-0.773589321594955));
#41412=DIRECTION('',(0.,-0.819152044288992,-0.573576436351046));
#41413=DIRECTION('',(0.,0.819152044288992,0.573576436351046));
#41414=DIRECTION('center_axis',(0.707106781186547,-0.53599666988936,-0.461202309044));
#41415=DIRECTION('ref_axis',(-0.546305769586287,0.,-0.837585820150231));
#41416=DIRECTION('',(0.,0.652238560447812,-0.758013759944347));
#41417=DIRECTION('',(0.,-0.652238560447812,0.758013759944347));
#41418=DIRECTION('center_axis',(1.,0.,0.));
#41419=DIRECTION('ref_axis',(0.,-0.573576436351046,0.819152044288992));
#41420=DIRECTION('center_axis',(0.,-0.758013759944347,-0.652238560447812));
#41421=DIRECTION('ref_axis',(0.,0.652238560447812,-0.758013759944347));
#41422=DIRECTION('center_axis',(0.,0.573576436351046,-0.819152044288992));
#41423=DIRECTION('ref_axis',(0.,0.819152044288992,0.573576436351046));
#41424=DIRECTION('center_axis',(0.56100663158041,-0.0309795099544078,-0.827231424261547));
#41425=DIRECTION('ref_axis',(-0.827628669643383,0.,-0.561276032968025));
#41426=DIRECTION('',(0.705516335778304,0.540633592148827,0.458216126942529));
#41427=DIRECTION('',(0.,-0.999299499382783,0.037423395534326));
#41428=DIRECTION('',(-0.705516335778297,0.50484728372422,-0.497368997894162));
#41429=DIRECTION('center_axis',(0.561006631580422,0.820043455596693,-0.113138367744206));
#41430=DIRECTION('ref_axis',(-0.197690230426216,0.,-0.980264542250728));
#41431=DIRECTION('',(0.70551633577829,-0.402147034415294,0.583544739211107));
#41432=DIRECTION('',(0.,-0.136671686945037,-0.990616399010029));
#41433=DIRECTION('',(-0.705516335778305,0.545134832430407,0.452851757665825));
#41434=DIRECTION('center_axis',(-0.561006631580388,-0.0309795099544084,
-0.827231424261562));
#41435=DIRECTION('ref_axis',(-0.827628669643398,0.,0.561276032968003));
#41436=DIRECTION('',(0.,0.999299499382783,-0.037423395534326));
#41437=DIRECTION('',(0.705516335778314,-0.540633592148832,-0.458216126942508));
#41438=DIRECTION('',(-0.705516335778307,-0.504847283724225,0.497368997894142));
#41439=DIRECTION('center_axis',(-0.70710678118654,-0.493760610936952,-0.506162482891787));
#41440=DIRECTION('ref_axis',(-0.582064997116551,0.,0.813142262541868));
#41441=DIRECTION('',(0.,0.715821848069997,-0.698282952552655));
#41442=DIRECTION('',(0.,-0.715821848069997,0.698282952552655));
#41443=DIRECTION('center_axis',(-0.561006631580398,0.820043455596709,-0.113138367744208));
#41444=DIRECTION('ref_axis',(-0.197690230426228,0.,0.980264542250726));
#41445=DIRECTION('',(0.70551633577832,0.402147034415284,-0.583544739211079));
#41446=DIRECTION('',(-0.705516335778308,-0.545134832430382,-0.45285175766585));
#41447=DIRECTION('',(0.,0.136671686945037,0.990616399010029));
#41448=DIRECTION('center_axis',(-0.70710678118654,0.584213367728653,0.398365085025227));
#41449=DIRECTION('ref_axis',(0.490839120629142,0.,0.871250226777595));
#41450=DIRECTION('',(0.,0.563373306018581,-0.826202467961513));
#41451=DIRECTION('',(0.,-0.563373306018581,0.826202467961513));
#41452=DIRECTION('center_axis',(0.,0.990616399010029,-0.136671686945037));
#41453=DIRECTION('ref_axis',(0.,0.136671686945037,0.990616399010029));
#41454=DIRECTION('',(-1.,0.,0.));
#41455=DIRECTION('',(1.,0.,0.));
#41456=DIRECTION('center_axis',(-0.70710678118653,0.454519477672055,-0.541675220419715));
#41457=DIRECTION('ref_axis',(-0.608120402411362,0.,0.793844806099431));
#41458=DIRECTION('',(0.,-0.766044443118978,-0.642787609686539));
#41459=DIRECTION('',(0.,0.766044443118978,0.642787609686539));
#41460=DIRECTION('center_axis',(0.,-0.037423395534326,-0.999299499382783));
#41461=DIRECTION('ref_axis',(-1.,0.,0.));
#41462=DIRECTION('',(-1.,0.,0.));
#41463=DIRECTION('',(1.,0.,0.));
#41464=DIRECTION('center_axis',(0.707106781186542,0.584213367728652,0.398365085025226));
#41465=DIRECTION('ref_axis',(0.490839120629141,0.,-0.871250226777596));
#41466=DIRECTION('',(0.,0.563373306018581,-0.826202467961513));
#41467=DIRECTION('',(0.,-0.563373306018581,0.826202467961513));
#41468=DIRECTION('center_axis',(0.707106781186559,0.454519477672036,-0.541675220419693));
#41469=DIRECTION('ref_axis',(-0.60812040241133,0.,-0.793844806099455));
#41470=DIRECTION('',(0.,-0.766044443118978,-0.642787609686539));
#41471=DIRECTION('',(0.,0.766044443118978,0.642787609686539));
#41472=DIRECTION('center_axis',(0.707106781186551,-0.493760610936944,-0.50616248289178));
#41473=DIRECTION('ref_axis',(-0.58206499711654,0.,-0.813142262541876));
#41474=DIRECTION('',(0.,0.715821848069997,-0.698282952552655));
#41475=DIRECTION('',(0.,-0.715821848069997,0.698282952552655));
#41476=DIRECTION('center_axis',(1.,0.,0.));
#41477=DIRECTION('ref_axis',(0.,-0.642787609686539,0.766044443118978));
#41478=DIRECTION('center_axis',(0.,-0.698282952552655,-0.715821848069998));
#41479=DIRECTION('ref_axis',(0.,0.715821848069997,-0.698282952552655));
#41480=DIRECTION('center_axis',(0.,0.642787609686539,-0.766044443118978));
#41481=DIRECTION('ref_axis',(0.,0.766044443118978,0.642787609686539));
#41482=DIRECTION('center_axis',(0.707106781186551,-0.447766735594493,-0.547270454615491));
#41483=DIRECTION('ref_axis',(-0.612056372482119,0.,-0.790814135498367));
#41484=DIRECTION('',(0.595596683047422,-0.0400145312984589,0.802286375571637));
#41485=DIRECTION('',(0.,-0.773957299203321,0.633237790257263));
#41486=DIRECTION('',(0.,0.773957299203321,-0.633237790257263));
#41487=DIRECTION('',(0.557191914001248,0.829352850155039,0.0413644885298826));
#41488=DIRECTION('center_axis',(1.,0.,0.));
#41489=DIRECTION('ref_axis',(0.,-0.707106781186547,0.707106781186548));
#41490=DIRECTION('',(0.,-0.707106781186548,-0.707106781186547));
#41491=DIRECTION('',(0.,0.633237790257263,-0.773957299203321));
#41492=DIRECTION('center_axis',(0.707106781186548,0.5,-0.5));
#41493=DIRECTION('ref_axis',(-0.577350269189625,0.,-0.816496580927726));
#41494=DIRECTION('',(0.55719191400122,-0.829352850155059,-0.0413644885298627));
#41495=DIRECTION('',(0.,0.707106781186548,0.707106781186547));
#41496=DIRECTION('',(0.705516335778303,-0.451476018710246,0.546274751823203));
#41497=DIRECTION('center_axis',(0.,0.0498137018801831,-0.998758526924798));
#41498=DIRECTION('ref_axis',(-1.,0.,0.));
#41499=DIRECTION('',(-1.,0.,0.));
#41500=DIRECTION('',(0.,0.998758526924798,0.0498137018801831));
#41501=DIRECTION('',(1.,0.,0.));
#41502=DIRECTION('center_axis',(0.561006631580394,0.826783601144283,-0.041236345639636));
#41503=DIRECTION('ref_axis',(-0.0733064378127065,0.,-0.997309463594531));
#41504=DIRECTION('',(0.,-0.049813701880158,-0.998758526924799));
#41505=DIRECTION('',(-0.705516335778304,0.503591798518316,0.498640151226356));
#41506=DIRECTION('center_axis',(-0.561006631580403,0.0412363456396555,-0.826783601144276));
#41507=DIRECTION('ref_axis',(-0.82748744528631,0.,0.561484218739526));
#41508=DIRECTION('',(0.705516335778297,-0.498640151226348,-0.503591798518334));
#41509=DIRECTION('',(-0.705516335778305,-0.546274751823202,0.451476018710245));
#41510=DIRECTION('center_axis',(-0.70710678118655,-0.447766735594494,-0.547270454615492));
#41511=DIRECTION('ref_axis',(-0.61205637248212,0.,0.790814135498366));
#41512=DIRECTION('',(0.,0.773957299203321,-0.633237790257263));
#41513=DIRECTION('',(0.,-0.773957299203321,0.633237790257263));
#41514=DIRECTION('center_axis',(-0.561006631580412,0.826783601144271,-0.0412363456396355));
#41515=DIRECTION('ref_axis',(-0.0733064378127032,0.,0.997309463594532));
#41516=DIRECTION('',(0.705516335778307,0.451476018710271,-0.546274751823178));
#41517=DIRECTION('',(-0.705516335778288,-0.503591798518327,-0.498640151226367));
#41518=DIRECTION('',(0.,0.049813701880158,0.998758526924799));
#41519=DIRECTION('center_axis',(-0.707106781186558,0.547270454615486,0.447766735594489));
#41520=DIRECTION('ref_axis',(0.534994468449976,0.,0.84485556086702));
#41521=DIRECTION('',(0.,0.633237790257263,-0.773957299203321));
#41522=DIRECTION('',(0.,-0.633237790257263,0.773957299203321));
#41523=DIRECTION('center_axis',(0.,0.998758526924799,-0.049813701880158));
#41524=DIRECTION('ref_axis',(0.,0.049813701880158,0.998758526924799));
#41525=DIRECTION('',(-1.,0.,0.));
#41526=DIRECTION('',(1.,0.,0.));
#41527=DIRECTION('center_axis',(-0.707106781186547,0.500000000000001,-0.500000000000001));
#41528=DIRECTION('ref_axis',(-0.577350269189627,0.,0.816496580927725));
#41529=DIRECTION('',(0.,-0.707106781186548,-0.707106781186547));
#41530=DIRECTION('',(0.,0.707106781186548,0.707106781186547));
#41531=DIRECTION('center_axis',(0.707106781186551,0.547270454615491,0.447766735594493));
#41532=DIRECTION('ref_axis',(0.534994468449983,0.,-0.844855560867016));
#41533=DIRECTION('',(0.,-0.633237790257263,0.773957299203321));
#41534=DIRECTION('center_axis',(0.,-0.633237790257263,-0.773957299203321));
#41535=DIRECTION('ref_axis',(0.,0.773957299203321,-0.633237790257263));
#41536=DIRECTION('center_axis',(0.,0.707106781186547,-0.707106781186548));
#41537=DIRECTION('ref_axis',(0.,0.707106781186548,0.707106781186547));
#41538=DIRECTION('center_axis',(0.561006631580392,0.113138367744223,-0.820043455596711));
#41539=DIRECTION('ref_axis',(-0.825342782028782,0.,-0.564631997103415));
#41540=DIRECTION('',(0.705516335778306,0.452851757665851,0.545134832430383));
#41541=DIRECTION('',(0.,-0.990616399010027,-0.136671686945054));
#41542=DIRECTION('',(-0.705516335778304,0.583544739211119,-0.402147034415252));
#41543=DIRECTION('center_axis',(0.5610066315804,0.827231424261552,0.0309795099544278));
#41544=DIRECTION('ref_axis',(0.0551372865287725,0.,-0.998478782766186));
#41545=DIRECTION('',(0.705516335778306,-0.497368997894168,0.504847283724201));
#41546=DIRECTION('',(0.,0.0374233955343499,-0.999299499382783));
#41547=DIRECTION('',(-0.705516335778302,0.458216126942503,0.540633592148851));
#41548=DIRECTION('center_axis',(-0.56100663158039,0.113138367744223,-0.820043455596712));
#41549=DIRECTION('ref_axis',(-0.825342782028783,0.,0.564631997103413));
#41550=DIRECTION('',(0.,0.990616399010027,0.136671686945054));
#41551=DIRECTION('',(0.705516335778308,-0.45285175766585,-0.545134832430382));
#41552=DIRECTION('',(-0.705516335778306,-0.583544739211118,0.402147034415251));
#41553=DIRECTION('center_axis',(-0.707106781186547,-0.398365085025223,-0.584213367728647));
#41554=DIRECTION('ref_axis',(-0.636934375125931,0.,0.770918025332746));
#41555=DIRECTION('',(0.,0.826202467961513,-0.563373306018581));
#41556=DIRECTION('',(0.,-0.826202467961513,0.563373306018581));
#41557=DIRECTION('center_axis',(-0.561006631580419,0.82723142426154,0.0309795099544274));
#41558=DIRECTION('ref_axis',(0.0551372865287699,0.,0.998478782766186));
#41559=DIRECTION('',(0.705516335778298,0.497368997894186,-0.504847283724194));
#41560=DIRECTION('',(-0.705516335778296,-0.458216126942521,-0.540633592148843));
#41561=DIRECTION('',(0.,-0.0374233955343499,0.999299499382783));
#41562=DIRECTION('center_axis',(-0.707106781186558,0.506162482891774,0.493760610936939));
#41563=DIRECTION('ref_axis',(0.572517134274658,0.,0.819892755768663));
#41564=DIRECTION('',(0.,0.698282952552655,-0.715821848069998));
#41565=DIRECTION('',(0.,-0.698282952552655,0.715821848069998));
#41566=DIRECTION('center_axis',(0.,0.999299499382783,0.0374233955343499));
#41567=DIRECTION('ref_axis',(0.,-0.0374233955343499,0.999299499382783));
#41568=DIRECTION('',(-1.,0.,0.));
#41569=DIRECTION('',(1.,0.,0.));
#41570=DIRECTION('center_axis',(-0.707106781186558,0.541675220419694,-0.454519477672037));
#41571=DIRECTION('ref_axis',(-0.540716203060926,0.,0.841205080671399));
#41572=DIRECTION('',(0.,-0.642787609686539,-0.766044443118978));
#41573=DIRECTION('',(0.,0.642787609686539,0.766044443118978));
#41574=DIRECTION('center_axis',(0.,0.136671686945054,-0.990616399010027));
#41575=DIRECTION('ref_axis',(-1.,0.,0.));
#41576=DIRECTION('',(-1.,0.,0.));
#41577=DIRECTION('',(1.,0.,0.));
#41578=DIRECTION('center_axis',(0.70710678118656,0.506162482891773,0.493760610936938));
#41579=DIRECTION('ref_axis',(0.572517134274656,0.,-0.819892755768665));
#41580=DIRECTION('',(0.,0.698282952552655,-0.715821848069998));
#41581=DIRECTION('',(0.,-0.698282952552655,0.715821848069998));
#41582=DIRECTION('center_axis',(0.70710678118655,0.5416752204197,-0.454519477672042));
#41583=DIRECTION('ref_axis',(-0.540716203060935,0.,-0.841205080671394));
#41584=DIRECTION('',(0.,-0.642787609686539,-0.766044443118978));
#41585=DIRECTION('',(0.,0.642787609686539,0.766044443118978));
#41586=DIRECTION('center_axis',(0.707106781186549,-0.398365085025222,-0.584213367728646));
#41587=DIRECTION('ref_axis',(-0.636934375125929,0.,-0.770918025332747));
#41588=DIRECTION('',(0.,0.826202467961513,-0.563373306018581));
#41589=DIRECTION('',(0.,-0.826202467961513,0.563373306018581));
#41590=DIRECTION('center_axis',(1.,0.,0.));
#41591=DIRECTION('ref_axis',(0.,-0.766044443118978,0.642787609686539));
#41592=DIRECTION('center_axis',(0.,-0.563373306018581,-0.826202467961513));
#41593=DIRECTION('ref_axis',(0.,0.826202467961513,-0.563373306018581));
#41594=DIRECTION('center_axis',(0.,0.766044443118978,-0.642787609686539));
#41595=DIRECTION('ref_axis',(0.,0.642787609686539,0.766044443118978));
#41596=DIRECTION('center_axis',(0.56100663158042,0.82138351674419,0.102959592771817));
#41597=DIRECTION('ref_axis',(0.180511696561749,0.,-0.98357283787445));
#41598=DIRECTION('',(0.705516335778302,-0.539476698684527,0.459577622960913));
#41599=DIRECTION('',(0.,0.124375678312001,-0.992235199256925));
#41600=DIRECTION('',(-0.705516335778294,0.409353153962195,0.578512484991614));
#41601=DIRECTION('center_axis',(0.,0.992235199256925,0.124375678312001));
#41602=DIRECTION('ref_axis',(0.,-0.124375678312001,0.992235199256925));
#41603=DIRECTION('',(0.55719191400124,-0.103279542068723,0.823935984868794));
#41604=DIRECTION('',(1.,0.,0.));
#41605=DIRECTION('',(-1.,0.,0.));
#41606=DIRECTION('',(-0.557191914001254,-0.103279542068721,0.823935984868785));
#41607=DIRECTION('center_axis',(0.707106781186552,0.461202309043997,0.535996669889356));
#41608=DIRECTION('ref_axis',(0.604079438549187,0.,-0.796924106751765));
#41609=DIRECTION('',(0.,0.758013759944346,-0.652238560447812));
#41610=DIRECTION('',(0.,-0.758013759944346,0.652238560447812));
#41611=DIRECTION('center_axis',(0.56100663158041,0.18417933855543,-0.807062284196261));
#41612=DIRECTION('ref_axis',(-0.821109284001916,0.,-0.570771008133613));
#41613=DIRECTION('',(0.705516335778302,0.403616888790147,0.582529061106243));
#41614=DIRECTION('',(0.,-0.974935082148255,-0.222489517947642));
#41615=DIRECTION('',(-0.705516335778307,0.616373598779655,-0.349757468365392));
#41616=DIRECTION('center_axis',(0.,0.222489517947642,-0.974935082148256));
#41617=DIRECTION('ref_axis',(-1.,0.,0.));
#41618=DIRECTION('',(0.557191914001234,0.809570248762125,0.184751680075913));
#41619=DIRECTION('',(1.,0.,0.));
#41620=DIRECTION('',(-1.,0.,0.));
#41621=DIRECTION('',(-0.557191914001256,0.809570248762111,0.184751680075909));
#41622=DIRECTION('center_axis',(0.707106781186547,0.579227965339569,-0.405579787672639));
#41623=DIRECTION('ref_axis',(-0.497542812164523,0.,-0.867439421552547));
#41624=DIRECTION('',(0.,-0.573576436351046,-0.819152044288992));
#41625=DIRECTION('',(0.,0.573576436351046,0.819152044288992));
#41626=DIRECTION('center_axis',(0.707106781186546,-0.345931635619494,-0.61671006435571));
#41627=DIRECTION('ref_axis',(-0.657291420225581,0.,-0.753636509796227));
#41628=DIRECTION('',(0.,0.872159737063827,-0.489221210746995));
#41629=DIRECTION('',(0.,-0.872159737063827,0.489221210746995));
#41630=DIRECTION('center_axis',(-0.707106781186541,0.461202309044004,0.535996669889364));
#41631=DIRECTION('ref_axis',(0.604079438549199,0.,0.796924106751756));
#41632=DIRECTION('',(-0.595596683047437,-0.797046293239175,-0.0999089464291446));
#41633=DIRECTION('',(0.,-0.758013759944346,0.652238560447812));
#41634=DIRECTION('',(0.,0.758013759944346,-0.652238560447812));
#41635=DIRECTION('center_axis',(0.,0.819152044288992,-0.573576436351046));
#41636=DIRECTION('ref_axis',(0.,0.573576436351046,0.819152044288992));
#41637=DIRECTION('',(0.,-0.573576436351046,-0.819152044288992));
#41638=DIRECTION('center_axis',(-0.707106781186546,0.579227965339571,-0.40557978767264));
#41639=DIRECTION('ref_axis',(-0.497542812164525,0.,0.867439421552546));
#41640=DIRECTION('',(0.595596683047429,0.178722187740901,-0.783149392358831));
#41641=DIRECTION('',(0.,0.573576436351046,0.819152044288992));
#41642=DIRECTION('center_axis',(-0.707106781186545,-0.345931635619495,-0.616710064355711));
#41643=DIRECTION('ref_axis',(-0.657291420225582,0.,0.753636509796226));
#41644=DIRECTION('',(0.,-0.872159737063827,0.489221210746995));
#41645=DIRECTION('',(0.,0.872159737063827,-0.489221210746995));
#41646=DIRECTION('center_axis',(0.,-0.489221210746995,-0.872159737063827));
#41647=DIRECTION('ref_axis',(0.,0.872159737063827,-0.489221210746995));
#41648=DIRECTION('center_axis',(0.,0.652238560447812,0.758013759944346));
#41649=DIRECTION('ref_axis',(0.,-0.758013759944346,0.652238560447812));
#41650=DIRECTION('center_axis',(0.561006631580402,0.253818593389698,-0.787938881495568));
#41651=DIRECTION('ref_axis',(-0.814616058663784,0.,-0.580000583592019));
#41652=DIRECTION('',(0.7055163357783,0.351310251680245,0.615489891886393));
#41653=DIRECTION('',(0.,-0.951833920629443,-0.306614069375792));
#41654=DIRECTION('',(-0.705516335778309,0.644511483084945,-0.294706036791908));
#41655=DIRECTION('center_axis',(0.561006631580397,0.809284384699514,0.174156090919455));
#41656=DIRECTION('ref_axis',(0.2964777621296,0.,-0.955039756535101));
#41657=DIRECTION('',(0.705516335778309,-0.577478656052882,0.410810298986413));
#41658=DIRECTION('',(0.,0.210381387077539,-0.97761939013674));
#41659=DIRECTION('',(-0.705516335778306,0.357374756306044,0.611988548508179));
#41660=DIRECTION('center_axis',(-0.561006631580411,0.253818593389687,-0.787938881495565));
#41661=DIRECTION('ref_axis',(-0.814616058663778,0.,0.580000583592027));
#41662=DIRECTION('',(0.,0.951833920629443,0.306614069375792));
#41663=DIRECTION('',(0.705516335778308,-0.351310251680223,-0.615489891886397));
#41664=DIRECTION('',(-0.705516335778296,-0.644511483084956,0.294706036791914));
#41665=DIRECTION('center_axis',(-0.707106781186549,-0.290865437587467,-0.644513225013303));
#41666=DIRECTION('ref_axis',(-0.673638686438956,0.,0.739060836557315));
#41667=DIRECTION('',(0.,0.911479343942638,-0.411345846661781));
#41668=DIRECTION('',(0.,-0.911479343942638,0.411345846661781));
#41669=DIRECTION('center_axis',(-0.561006631580409,0.809284384699507,0.174156090919453));
#41670=DIRECTION('ref_axis',(0.296477762129592,0.,0.955039756535103));
#41671=DIRECTION('',(0.705516335778289,0.577478656052889,-0.410810298986437));
#41672=DIRECTION('',(-0.705516335778318,-0.357374756306074,-0.611988548508149));
#41673=DIRECTION('',(0.,-0.210381387077539,0.97761939013674));
#41674=DIRECTION('center_axis',(-0.707106781186536,0.412732107142832,0.574153470540286));
#41675=DIRECTION('ref_axis',(0.630347388214446,0.,0.776313190774978));
#41676=DIRECTION('',(0.,0.811975624921639,-0.583691343548209));
#41677=DIRECTION('',(0.,-0.811975624921639,0.583691343548209));
#41678=DIRECTION('center_axis',(0.,0.97761939013674,0.210381387077539));
#41679=DIRECTION('ref_axis',(0.,-0.210381387077539,0.97761939013674));
#41680=DIRECTION('',(-1.,0.,0.));
#41681=DIRECTION('',(1.,0.,0.));
#41682=DIRECTION('center_axis',(-0.707106781186558,0.612372435695785,-0.353553390593269));
#41683=DIRECTION('ref_axis',(-0.447213595499948,0.,0.894427190999921));
#41684=DIRECTION('',(0.,-0.5,-0.866025403784438));
#41685=DIRECTION('',(0.,0.5,0.866025403784438));
#41686=DIRECTION('center_axis',(0.,0.306614069375792,-0.951833920629443));
#41687=DIRECTION('ref_axis',(-1.,0.,0.));
#41688=DIRECTION('',(-1.,0.,0.));
#41689=DIRECTION('',(1.,0.,0.));
#41690=DIRECTION('center_axis',(0.707106781186547,0.412732107142825,0.574153470540276));
#41691=DIRECTION('ref_axis',(0.630347388214433,0.,-0.776313190774988));
#41692=DIRECTION('',(0.,0.811975624921639,-0.583691343548209));
#41693=DIRECTION('',(0.,-0.811975624921639,0.583691343548209));
#41694=DIRECTION('center_axis',(0.707106781186545,0.612372435695796,-0.353553390593275));
#41695=DIRECTION('ref_axis',(-0.44721359549996,0.,-0.894427190999915));
#41696=DIRECTION('',(0.,-0.5,-0.866025403784438));
#41697=DIRECTION('',(0.,0.5,0.866025403784438));
#41698=DIRECTION('center_axis',(0.707106781186551,-0.290865437587466,-0.644513225013302));
#41699=DIRECTION('ref_axis',(-0.673638686438954,0.,-0.739060836557317));
#41700=DIRECTION('',(0.,0.911479343942638,-0.411345846661781));
#41701=DIRECTION('',(0.,-0.911479343942638,0.411345846661781));
#41702=DIRECTION('center_axis',(1.,0.,0.));
#41703=DIRECTION('ref_axis',(0.,-0.866025403784438,0.5));
#41704=DIRECTION('center_axis',(0.,-0.411345846661781,-0.911479343942638));
#41705=DIRECTION('ref_axis',(0.,0.911479343942638,-0.411345846661781));
#41706=DIRECTION('center_axis',(0.,0.866025403784438,-0.5));
#41707=DIRECTION('ref_axis',(0.,0.5,0.866025403784438));
#41708=DIRECTION('center_axis',(0.561006631580419,0.321526135468423,-0.762818788136169));
#41709=DIRECTION('ref_axis',(-0.805595332751383,0.,-0.592466167683176));
#41710=DIRECTION('',(0.705516335778299,0.296329931428078,0.643766472946357));
#41711=DIRECTION('',(0.,-0.921488728241601,-0.388405102597375));
#41712=DIRECTION('',(-0.705516335778303,0.667744245837286,-0.237411714330086));
#41713=DIRECTION('center_axis',(0.561006631580396,0.791026109827976,0.244027156056938));
#41714=DIRECTION('ref_axis',(0.398879012810069,0.,-0.917003562228449));
#41715=DIRECTION('',(0.705516335778303,-0.611085652157587,0.358916460582535));
#41716=DIRECTION('',(0.,0.294785966455742,-0.955563307154871));
#41717=DIRECTION('',(-0.705516335778307,0.302676520965598,0.640807009641837));
#41718=DIRECTION('center_axis',(-0.561006631580408,0.321526135468426,-0.762818788136176));
#41719=DIRECTION('ref_axis',(-0.805595332751391,0.,0.592466167683165));
#41720=DIRECTION('',(0.,0.921488728241601,0.388405102597375));
#41721=DIRECTION('',(0.705516335778306,-0.296329931428079,-0.643766472946349));
#41722=DIRECTION('',(-0.705516335778307,-0.667744245837287,0.237411714330074));
#41723=DIRECTION('center_axis',(-0.70710678118655,-0.233585577946047,-0.667411250860823));
#41724=DIRECTION('ref_axis',(-0.686399640790371,0.,0.727224541062009));
#41725=DIRECTION('',(0.,0.943862042647771,-0.330339892306058));
#41726=DIRECTION('',(0.,-0.943862042647771,0.330339892306058));
#41727=DIRECTION('center_axis',(-0.561006631580394,0.791026109827977,0.244027156056939));
#41728=DIRECTION('ref_axis',(0.39887901281007,0.,0.917003562228448));
#41729=DIRECTION('',(0.705516335778304,0.611085652157585,-0.358916460582534));
#41730=DIRECTION('',(-0.705516335778308,-0.302676520965597,-0.640807009641836));
#41731=DIRECTION('',(0.,-0.294785966455742,0.955563307154871));
#41732=DIRECTION('center_axis',(-0.707106781186546,0.361120764691834,0.607940616597038));
#41733=DIRECTION('ref_axis',(0.651933718094184,0.,0.758275957163283));
#41734=DIRECTION('',(0.,0.859757865108992,-0.510701883081734));
#41735=DIRECTION('',(0.,-0.859757865108992,0.510701883081734));
#41736=DIRECTION('center_axis',(0.,0.955563307154871,0.294785966455742));
#41737=DIRECTION('ref_axis',(0.,-0.294785966455742,0.955563307154871));
#41738=DIRECTION('',(-1.,0.,0.));
#41739=DIRECTION('',(1.,0.,0.));
#41740=DIRECTION('center_axis',(-0.707106781186552,0.640856382055784,-0.298836238730118));
#41741=DIRECTION('ref_axis',(-0.389281620635021,0.,0.921118787038768));
#41742=DIRECTION('',(0.,-0.4226182617407,-0.90630778703665));
#41743=DIRECTION('',(0.,0.4226182617407,0.90630778703665));
#41744=DIRECTION('center_axis',(0.,0.388405102597375,-0.921488728241601));
#41745=DIRECTION('ref_axis',(-1.,0.,0.));
#41746=DIRECTION('',(-1.,0.,0.));
#41747=DIRECTION('',(1.,0.,0.));
#41748=DIRECTION('center_axis',(0.707106781186547,0.361120764691833,0.607940616597037));
#41749=DIRECTION('ref_axis',(0.651933718094183,0.,-0.758275957163284));
#41750=DIRECTION('',(0.,0.859757865108992,-0.510701883081734));
#41751=DIRECTION('',(0.,-0.859757865108992,0.510701883081734));
#41752=DIRECTION('center_axis',(0.707106781186554,0.640856382055783,-0.298836238730118));
#41753=DIRECTION('ref_axis',(-0.389281620635019,0.,-0.921118787038769));
#41754=DIRECTION('',(0.,-0.4226182617407,-0.90630778703665));
#41755=DIRECTION('',(0.,0.4226182617407,0.90630778703665));
#41756=DIRECTION('center_axis',(0.707106781186551,-0.233585577946046,-0.667411250860821));
#41757=DIRECTION('ref_axis',(-0.686399640790369,0.,-0.727224541062011));
#41758=DIRECTION('',(0.,0.943862042647771,-0.330339892306058));
#41759=DIRECTION('',(0.,-0.943862042647771,0.330339892306058));
#41760=DIRECTION('center_axis',(1.,0.,0.));
#41761=DIRECTION('ref_axis',(0.,-0.90630778703665,0.4226182617407));
#41762=DIRECTION('center_axis',(0.,-0.330339892306058,-0.943862042647771));
#41763=DIRECTION('ref_axis',(0.,0.943862042647771,-0.330339892306058));
#41764=DIRECTION('center_axis',(0.,0.90630778703665,-0.4226182617407));
#41765=DIRECTION('ref_axis',(0.,0.4226182617407,0.90630778703665));
#41766=DIRECTION('center_axis',(0.707106781186546,-0.17452799101363,-0.685229874095364));
#41767=DIRECTION('ref_axis',(-0.695910561235545,0.,-0.718128463967853));
#41768=DIRECTION('',(0.595596683047423,-0.375326354772754,0.710207517952256));
#41769=DIRECTION('',(0.,-0.96906138128887,0.246819851905205));
#41770=DIRECTION('',(0.,0.96906138128887,-0.246819851905205));
#41771=DIRECTION('',(0.55719191400124,0.734167558056277,0.387988617963616));
#41772=DIRECTION('center_axis',(1.,0.,0.));
#41773=DIRECTION('ref_axis',(0.,-0.939692620785908,0.342020143325669));
#41774=DIRECTION('',(0.,-0.342020143325669,-0.939692620785908));
#41775=DIRECTION('',(0.,0.900996828806872,-0.433825672914779));
#41776=DIRECTION('center_axis',(0.707106781186551,0.664463024388671,-0.241844762647975));
#41777=DIRECTION('ref_axis',(-0.323615577118182,0.,-0.946188648339466));
#41778=DIRECTION('',(0.557191914001246,-0.734167558056274,-0.387988617963615));
#41779=DIRECTION('',(0.,0.342020143325669,0.939692620785908));
#41780=DIRECTION('',(0.705516335778303,-0.64004191746577,0.304291051193915));
#41781=DIRECTION('center_axis',(0.,0.467240138462762,-0.884130450221741));
#41782=DIRECTION('ref_axis',(-1.,0.,0.));
#41783=DIRECTION('',(-1.,0.,0.));
#41784=DIRECTION('',(0.,0.884130450221741,0.467240138462762));
#41785=DIRECTION('',(1.,0.,0.));
#41786=DIRECTION('center_axis',(0.561006631580418,0.766747648626013,0.312041027189173));
#41787=DIRECTION('ref_axis',(0.486084108127403,0.,-0.873912032086747));
#41788=DIRECTION('',(0.,0.376947046632555,-0.926234810420659));
#41789=DIRECTION('',(-0.705516335778304,0.245674734539573,0.66474854250225));
#41790=DIRECTION('center_axis',(-0.561006631580399,0.386786669513442,-0.731893183196506));
#41791=DIRECTION('ref_axis',(-0.793664727118316,0.,0.608355406755138));
#41792=DIRECTION('',(0.705516335778311,-0.239094361468879,-0.667143602430342));
#41793=DIRECTION('',(-0.705516335778307,-0.68589507168381,0.178310545369064));
#41794=DIRECTION('center_axis',(-0.707106781186545,-0.17452799101363,-0.685229874095365));
#41795=DIRECTION('ref_axis',(-0.695910561235547,0.,0.718128463967852));
#41796=DIRECTION('',(0.,0.96906138128887,-0.246819851905205));
#41797=DIRECTION('',(0.,-0.96906138128887,0.246819851905205));
#41798=DIRECTION('center_axis',(-0.561006631580416,0.766747648626014,0.312041027189174));
#41799=DIRECTION('ref_axis',(0.486084108127405,0.,0.873912032086746));
#41800=DIRECTION('',(0.705516335778304,0.640041917465768,-0.304291051193914));
#41801=DIRECTION('',(-0.705516335778305,-0.245674734539572,-0.664748542502249));
#41802=DIRECTION('',(0.,-0.376947046632555,0.926234810420659));
#41803=DIRECTION('center_axis',(-0.707106781186547,0.306761075170857,0.637100967476914));
#41804=DIRECTION('ref_axis',(0.669373784875801,0.,0.742925794491647));
#41805=DIRECTION('',(0.,0.900996828806872,-0.433825672914779));
#41806=DIRECTION('',(0.,-0.900996828806872,0.433825672914779));
#41807=DIRECTION('center_axis',(0.,0.926234810420659,0.376947046632555));
#41808=DIRECTION('ref_axis',(0.,-0.376947046632555,0.926234810420659));
#41809=DIRECTION('',(-1.,0.,0.));
#41810=DIRECTION('',(1.,0.,0.));
#41811=DIRECTION('center_axis',(-0.707106781186549,0.664463024388673,-0.241844762647975));
#41812=DIRECTION('ref_axis',(-0.323615577118184,0.,0.946188648339466));
#41813=DIRECTION('',(0.,-0.342020143325669,-0.939692620785908));
#41814=DIRECTION('',(0.,0.342020143325669,0.939692620785908));
#41815=DIRECTION('center_axis',(0.707106781186549,0.306761075170857,0.637100967476913));
#41816=DIRECTION('ref_axis',(0.669373784875799,0.,-0.742925794491649));
#41817=DIRECTION('',(0.,-0.900996828806872,0.433825672914779));
#41818=DIRECTION('center_axis',(0.,-0.246819851905205,-0.96906138128887));
#41819=DIRECTION('ref_axis',(0.,0.96906138128887,-0.246819851905205));
#41820=DIRECTION('center_axis',(0.,0.939692620785908,-0.342020143325669));
#41821=DIRECTION('ref_axis',(0.,0.342020143325669,0.939692620785908));
#41822=DIRECTION('center_axis',(0.561006631580399,0.449103523455305,-0.695397429203505));
#41823=DIRECTION('ref_axis',(-0.778302413620336,0.,-0.627889602520029));
#41824=DIRECTION('',(0.705516335778308,0.18003913904976,0.685443366267536));
#41825=DIRECTION('',(0.,-0.840043405623117,-0.542519194747167));
#41826=DIRECTION('',(-0.705516335778306,0.698825821880053,-0.117852325490936));
#41827=DIRECTION('center_axis',(0.561006631580396,0.736633774843142,0.37768007768899));
#41828=DIRECTION('ref_axis',(0.558457227212258,0.,-0.829533317820566));
#41829=DIRECTION('',(0.705516335778306,-0.664127077314135,0.2473498031698));
#41830=DIRECTION('',(0.,0.456239332177649,-0.889857107503274));
#41831=DIRECTION('',(-0.705516335778303,0.186803215041171,0.683630937568099));
#41832=DIRECTION('center_axis',(-0.561006631580406,0.449103523455303,-0.695397429203502));
#41833=DIRECTION('ref_axis',(-0.77830241362033,0.,0.627889602520036));
#41834=DIRECTION('',(0.,0.840043405623117,0.542519194747167));
#41835=DIRECTION('',(0.705516335778303,-0.180039139049758,-0.685443366267541));
#41836=DIRECTION('',(-0.705516335778306,-0.69882582188005,0.117852325490948));
#41837=DIRECTION('center_axis',(-0.70710678118655,-0.114142140686715,-0.697833484234922));
#41838=DIRECTION('ref_axis',(-0.702424227635741,0.,0.711758529580316));
#41839=DIRECTION('',(0.,0.986885577683101,-0.161421363397451));
#41840=DIRECTION('',(0.,-0.986885577683101,0.161421363397451));
#41841=DIRECTION('center_axis',(-0.561006631580396,0.736633774843142,0.377680077688989));
#41842=DIRECTION('ref_axis',(0.558457227212258,0.,0.829533317820566));
#41843=DIRECTION('',(0.705516335778308,0.664127077314134,-0.247349803169793));
#41844=DIRECTION('',(-0.705516335778302,-0.186803215041169,-0.683630937568101));
#41845=DIRECTION('',(0.,-0.456239332177649,0.889857107503274));
#41846=DIRECTION('center_axis',(-0.707106781186547,0.250066748640429,0.661412595302211));
#41847=DIRECTION('ref_axis',(0.683116152038586,0.,0.730309744439985));
#41848=DIRECTION('',(0.,0.935378662600772,-0.353647787425838));
#41849=DIRECTION('',(0.,-0.935378662600772,0.353647787425838));
#41850=DIRECTION('center_axis',(0.,0.889857107503274,0.456239332177649));
#41851=DIRECTION('ref_axis',(0.,-0.456239332177649,0.889857107503274));
#41852=DIRECTION('',(-1.,0.,0.));
#41853=DIRECTION('',(1.,0.,0.));
#41854=DIRECTION('center_axis',(-0.707106781186551,0.683012701892216,-0.183012701892218));
#41855=DIRECTION('ref_axis',(-0.250562807085729,0.,0.968100345886375));
#41856=DIRECTION('',(0.,-0.258819045102521,-0.965925826289068));
#41857=DIRECTION('',(0.,0.258819045102521,0.965925826289068));
#41858=DIRECTION('center_axis',(0.,0.542519194747167,-0.840043405623117));
#41859=DIRECTION('ref_axis',(-1.,0.,0.));
#41860=DIRECTION('',(-1.,0.,0.));
#41861=DIRECTION('',(1.,0.,0.));
#41862=DIRECTION('center_axis',(0.707106781186545,0.25006674864043,0.661412595302212));
#41863=DIRECTION('ref_axis',(0.683116152038587,0.,-0.730309744439983));
#41864=DIRECTION('',(0.,0.935378662600772,-0.353647787425838));
#41865=DIRECTION('',(0.,-0.935378662600772,0.353647787425838));
#41866=DIRECTION('center_axis',(0.707106781186552,0.683012701892215,-0.183012701892218));
#41867=DIRECTION('ref_axis',(-0.250562807085728,0.,-0.968100345886376));
#41868=DIRECTION('',(0.,-0.258819045102521,-0.965925826289068));
#41869=DIRECTION('',(0.,0.258819045102521,0.965925826289068));
#41870=DIRECTION('center_axis',(0.707106781186545,-0.114142140686716,-0.697833484234927));
#41871=DIRECTION('ref_axis',(-0.702424227635745,0.,-0.711758529580311));
#41872=DIRECTION('',(0.,0.986885577683101,-0.161421363397451));
#41873=DIRECTION('',(0.,-0.986885577683101,0.161421363397451));
#41874=DIRECTION('center_axis',(1.,0.,0.));
#41875=DIRECTION('ref_axis',(0.,-0.965925826289068,0.258819045102521));
#41876=DIRECTION('center_axis',(0.,-0.161421363397451,-0.986885577683101));
#41877=DIRECTION('ref_axis',(0.,0.986885577683101,-0.161421363397451));
#41878=DIRECTION('center_axis',(0.,0.965925826289068,-0.258819045102521));
#41879=DIRECTION('ref_axis',(0.,0.258819045102521,0.965925826289068));
#41880=DIRECTION('center_axis',(0.56100663158039,0.700913673242072,0.44044475474812));
#41881=DIRECTION('ref_axis',(0.617521420133027,0.,-0.786554064052109));
#41882=DIRECTION('',(0.70551633577831,-0.683157829093258,0.188526073789633));
#41883=DIRECTION('',(0.,0.532059360920026,-0.846707054687377));
#41884=DIRECTION('',(-0.705516335778307,0.126510010281474,0.697310488411391));
#41885=DIRECTION('center_axis',(0.,0.846707054687377,0.532059360920026));
#41886=DIRECTION('ref_axis',(1.,0.,0.));
#41887=DIRECTION('',(0.557191914001242,-0.44181344692932,0.703091778563841));
#41888=DIRECTION('',(1.,0.,0.));
#41889=DIRECTION('',(-1.,0.,0.));
#41890=DIRECTION('',(-0.557191914001257,-0.441813446929314,0.703091778563833));
#41891=DIRECTION('center_axis',(0.707106781186546,0.191469263158417,0.680690473905413));
#41892=DIRECTION('ref_axis',(0.6935215873247,0.,-0.72043584580074));
#41893=DIRECTION('',(0.,0.962641699975202,-0.270778428736215));
#41894=DIRECTION('',(0.,-0.962641699975202,0.270778428736215));
#41895=DIRECTION('center_axis',(0.561006631580394,0.508002428407532,-0.653609280881836));
#41896=DIRECTION('ref_axis',(-0.758814655754538,0.,-0.651306623804888));
#41897=DIRECTION('',(0.705516335778306,0.119613710071895,0.698526492205406));
#41898=DIRECTION('',(0.,-0.789563123475643,-0.613669352377473));
#41899=DIRECTION('',(-0.70551633577831,0.706438085609211,-0.0564971782546651));
#41900=DIRECTION('center_axis',(0.,0.613669352377473,-0.789563123475643));
#41901=DIRECTION('ref_axis',(-1.,0.,0.));
#41902=DIRECTION('',(0.557191914001254,0.655640386718963,0.509581057609707));
#41903=DIRECTION('',(1.,0.,0.));
#41904=DIRECTION('',(-1.,0.,0.));
#41905=DIRECTION('',(-0.557191914001241,0.65564038671897,0.509581057609713));
#41906=DIRECTION('center_axis',(0.707106781186543,0.696364240320024,-0.122787803968974));
#41907=DIRECTION('ref_axis',(-0.171087869746038,0.,-0.985255774317392));
#41908=DIRECTION('',(0.,-0.17364817766693,-0.984807753012208));
#41909=DIRECTION('',(0.,0.17364817766693,0.984807753012208));
#41910=DIRECTION('center_axis',(0.707106781186546,-0.0528875997482673,-0.705126160196081));
#41911=DIRECTION('ref_axis',(-0.706114387365562,0.,-0.708097784176279));
#41912=DIRECTION('',(0.,0.997198978933359,-0.0747943608453594));
#41913=DIRECTION('',(0.,-0.997198978933359,0.0747943608453594));
#41914=DIRECTION('center_axis',(-0.707106781186541,0.191469263158418,0.680690473905417));
#41915=DIRECTION('ref_axis',(0.693521587324705,0.,0.720435845800736));
#41916=DIRECTION('',(-0.595596683047434,-0.680145916919126,-0.427394575118983));
#41917=DIRECTION('',(0.,-0.962641699975202,0.270778428736215));
#41918=DIRECTION('',(0.,0.962641699975202,-0.270778428736215));
#41919=DIRECTION('center_axis',(0.,0.984807753012208,-0.17364817766693));
#41920=DIRECTION('ref_axis',(0.,0.17364817766693,0.984807753012208));
#41921=DIRECTION('',(0.,-0.17364817766693,-0.984807753012208));
#41922=DIRECTION('center_axis',(-0.707106781186541,0.696364240320026,-0.122787803968974));
#41923=DIRECTION('ref_axis',(-0.171087869746039,0.,0.985255774317391));
#41924=DIRECTION('',(0.595596683047432,0.492950545347766,-0.634243132390283));
#41925=DIRECTION('',(0.,0.17364817766693,0.984807753012208));
#41926=DIRECTION('center_axis',(-0.707106781186545,-0.0528875997482674,
-0.705126160196082));
#41927=DIRECTION('ref_axis',(-0.706114387365564,0.,0.708097784176278));
#41928=DIRECTION('',(0.,-0.997198978933359,0.0747943608453594));
#41929=DIRECTION('',(0.,0.997198978933359,-0.0747943608453594));
#41930=DIRECTION('center_axis',(0.,-0.0747943608453594,-0.997198978933359));
#41931=DIRECTION('ref_axis',(0.,0.997198978933359,-0.0747943608453594));
#41932=DIRECTION('center_axis',(0.,0.270778428736215,0.962641699975202));
#41933=DIRECTION('ref_axis',(0.,-0.962641699975202,0.270778428736215));
#41934=DIRECTION('center_axis',(0.561006631580398,0.563035128139334,-0.606846771272567));
#41935=DIRECTION('ref_axis',(-0.734296425103062,0.,-0.678828962317359));
#41936=DIRECTION('',(0.705516335778301,0.0582779485356274,0.706293409755774));
#41937=DIRECTION('',(0.,-0.733073789207258,-0.680149115692517));
#41938=DIRECTION('',(-0.705516335778312,0.708673928947909,0.00528794662205492));
#41939=DIRECTION('center_axis',(0.561006631580394,0.659859195364387,0.499857381275784));
#41940=DIRECTION('ref_axis',(0.665244232298934,0.,-0.746625817523746));
#41941=DIRECTION('',(0.705516335778315,-0.696989337290999,0.128267547152788));
#41942=DIRECTION('',(0.,0.603830096659557,-0.797113049929625));
#41943=DIRECTION('',(-0.705516335778304,0.0652539879547269,0.70568308539029));
#41944=DIRECTION('center_axis',(-0.561006631580408,0.56303512813933,-0.606846771272562));
#41945=DIRECTION('ref_axis',(-0.734296425103054,0.,0.678828962317369));
#41946=DIRECTION('',(0.,0.733073789207258,0.680149115692517));
#41947=DIRECTION('',(0.705516335778306,-0.0582779485356024,-0.706293409755772));
#41948=DIRECTION('',(-0.705516335778301,-0.70867392894792,-0.00528794662205795));
#41949=DIRECTION('center_axis',(-0.707106781186548,0.00876944775867127,
-0.707052400311326));
#41950=DIRECTION('ref_axis',(-0.707079589180542,0.,0.707133972146916));
#41951=DIRECTION('',(0.,0.999923093828728,0.0124018719548352));
#41952=DIRECTION('',(0.,-0.999923093828728,-0.0124018719548352));
#41953=DIRECTION('center_axis',(-0.561006631580406,0.659859195364381,0.499857381275779));
#41954=DIRECTION('ref_axis',(0.665244232298923,0.,0.746625817523755));
#41955=DIRECTION('',(0.705516335778304,0.696989337291011,-0.128267547152789));
#41956=DIRECTION('',(-0.705516335778308,-0.065253987954752,-0.705683085390284));
#41957=DIRECTION('',(0.,-0.603830096659557,0.797113049929625));
#41958=DIRECTION('center_axis',(-0.707106781186545,0.131414580971466,0.694787886990049));
#41959=DIRECTION('ref_axis',(0.700866150214856,0.,0.713292814686232));
#41960=DIRECTION('',(0.,0.982578452753869,-0.185848282703424));
#41961=DIRECTION('',(0.,-0.982578452753869,0.185848282703424));
#41962=DIRECTION('center_axis',(0.,0.797113049929625,0.603830096659558));
#41963=DIRECTION('ref_axis',(1.,0.,0.));
#41964=DIRECTION('',(-1.,0.,0.));
#41965=DIRECTION('',(1.,0.,0.));
#41966=DIRECTION('center_axis',(-0.707106781186556,0.70441602640275,-0.0616284167162187));
#41967=DIRECTION('ref_axis',(-0.0868265938642456,0.,0.996223440096615));
#41968=DIRECTION('',(0.,-0.0871557427476582,-0.996194698091746));
#41969=DIRECTION('',(0.,0.0871557427476582,0.996194698091746));
#41970=DIRECTION('center_axis',(0.,0.680149115692517,-0.733073789207258));
#41971=DIRECTION('ref_axis',(-1.,0.,0.));
#41972=DIRECTION('',(-1.,0.,0.));
#41973=DIRECTION('',(1.,0.,0.));
#41974=DIRECTION('center_axis',(0.707106781186546,0.131414580971466,0.694787886990048));
#41975=DIRECTION('ref_axis',(0.700866150214854,0.,-0.713292814686234));
#41976=DIRECTION('',(0.,0.982578452753869,-0.185848282703424));
#41977=DIRECTION('',(0.,-0.982578452753869,0.185848282703424));
#41978=DIRECTION('center_axis',(0.707106781186545,0.704416026402761,-0.0616284167162196));
#41979=DIRECTION('ref_axis',(-0.0868265938642483,0.,-0.996223440096615));
#41980=DIRECTION('',(0.,-0.0871557427476582,-0.996194698091746));
#41981=DIRECTION('',(0.,0.0871557427476582,0.996194698091746));
#41982=DIRECTION('center_axis',(0.707106781186549,0.00876944775867125,-0.707052400311324));
#41983=DIRECTION('ref_axis',(-0.70707958918054,0.,-0.707133972146918));
#41984=DIRECTION('',(0.,0.999923093828728,0.0124018719548352));
#41985=DIRECTION('',(0.,-0.999923093828728,-0.0124018719548352));
#41986=DIRECTION('center_axis',(1.,0.,0.));
#41987=DIRECTION('ref_axis',(0.,-0.996194698091746,0.0871557427476582));
#41988=DIRECTION('center_axis',(0.,0.0124018719548352,-0.999923093828728));
#41989=DIRECTION('ref_axis',(0.,0.999923093828728,0.0124018719548352));
#41990=DIRECTION('center_axis',(0.,0.996194698091746,-0.0871557427476582));
#41991=DIRECTION('ref_axis',(0.,0.0871557427476582,0.996194698091746));
#41992=DIRECTION('center_axis',(0.561006631580416,0.613782790576088,-0.555465791309803));
#41993=DIRECTION('ref_axis',(-0.703588880269148,0.,-0.710607266752604));
#41994=DIRECTION('',(0.705516335778304,-0.00350134337823141,0.708685007986272));
#41995=DIRECTION('',(0.,-0.671005320760942,-0.741452533551882));
#41996=DIRECTION('',(-0.705516335778299,0.705516335778311,0.0670328270320439));
#41997=DIRECTION('center_axis',(0.561006631580416,0.613782790576088,0.555465791309803));
#41998=DIRECTION('ref_axis',(0.703588880269148,0.,-0.710607266752604));
#41999=DIRECTION('',(0.705516335778299,-0.705516335778311,0.0670328270320437));
#42000=DIRECTION('',(0.,0.671005320760943,-0.741452533551882));
#42001=DIRECTION('',(-0.705516335778305,0.00350134337823141,0.708685007986272));
#42002=DIRECTION('center_axis',(-0.561006631580414,0.613782790576089,-0.555465791309803));
#42003=DIRECTION('ref_axis',(-0.703588880269149,0.,0.710607266752603));
#42004=DIRECTION('',(0.,0.671005320760942,0.741452533551882));
#42005=DIRECTION('',(0.705516335778306,0.0035013433782314,-0.708685007986271));
#42006=DIRECTION('',(-0.7055163357783,-0.70551633577831,-0.067032827032044));
#42007=DIRECTION('center_axis',(-0.707106781186547,0.070359754473029,-0.703597544730292));
#42008=DIRECTION('ref_axis',(-0.705345615858598,0.,0.708863570928183));
#42009=DIRECTION('',(0.,0.995037190209989,0.0995037190209986));
#42010=DIRECTION('',(0.,-0.995037190209989,-0.0995037190209986));
#42011=DIRECTION('center_axis',(-0.561006631580415,0.613782790576088,0.555465791309804));
#42012=DIRECTION('ref_axis',(0.703588880269149,0.,0.710607266752603));
#42013=DIRECTION('',(0.7055163357783,0.70551633577831,-0.0670328270320424));
#42014=DIRECTION('',(-0.705516335778306,-0.0035013433782314,-0.708685007986271));
#42015=DIRECTION('',(0.,-0.671005320760943,0.741452533551882));
#42016=DIRECTION('center_axis',(-0.707106781186548,0.0703597544730292,0.703597544730292));
#42017=DIRECTION('ref_axis',(0.705345615858598,0.,0.708863570928183));
#42018=DIRECTION('',(0.,0.995037190209989,-0.099503719020999));
#42019=DIRECTION('',(0.,-0.995037190209989,0.099503719020999));
#42020=DIRECTION('center_axis',(0.,0.741452533551882,0.671005320760943));
#42021=DIRECTION('ref_axis',(1.,0.,0.));
#42022=DIRECTION('',(-1.,0.,0.));
#42023=DIRECTION('',(1.,0.,0.));
#42024=DIRECTION('center_axis',(-0.707106781186552,0.707106781186543,-1.29893408435323E-16));
#42025=DIRECTION('ref_axis',(-1.83697019872101E-16,0.,1.));
#42026=DIRECTION('',(0.,-1.83697019872103E-16,-1.));
#42027=DIRECTION('',(0.,1.83697019872103E-16,1.));
#42028=DIRECTION('center_axis',(0.,0.741452533551882,-0.671005320760942));
#42029=DIRECTION('ref_axis',(-1.,0.,0.));
#42030=DIRECTION('',(-1.,0.,0.));
#42031=DIRECTION('',(1.,0.,0.));
#42032=DIRECTION('center_axis',(0.707106781186548,0.0703597544730291,0.703597544730291));
#42033=DIRECTION('ref_axis',(0.705345615858597,0.,-0.708863570928184));
#42034=DIRECTION('',(0.,0.995037190209989,-0.099503719020999));
#42035=DIRECTION('',(0.,-0.995037190209989,0.099503719020999));
#42036=DIRECTION('center_axis',(0.707106781186554,0.707106781186541,-1.29893408435323E-16));
#42037=DIRECTION('ref_axis',(-1.836970198721E-16,0.,-1.));
#42038=DIRECTION('',(0.,-1.83697019872103E-16,-1.));
#42039=DIRECTION('',(0.,1.83697019872103E-16,1.));
#42040=DIRECTION('center_axis',(0.707106781186549,0.0703597544730288,-0.70359754473029));
#42041=DIRECTION('ref_axis',(-0.705345615858597,0.,-0.708863570928184));
#42042=DIRECTION('',(0.,0.995037190209989,0.0995037190209986));
#42043=DIRECTION('',(0.,-0.995037190209989,-0.0995037190209986));
#42044=DIRECTION('center_axis',(1.,0.,0.));
#42045=DIRECTION('ref_axis',(0.,-1.,1.83697019872103E-16));
#42046=DIRECTION('center_axis',(0.,0.0995037190209986,-0.995037190209989));
#42047=DIRECTION('ref_axis',(0.,0.995037190209989,0.0995037190209986));
#42048=DIRECTION('center_axis',(0.,1.,-1.83697019872103E-16));
#42049=DIRECTION('ref_axis',(0.,1.83697019872103E-16,1.));
#42050=DIRECTION('center_axis',(0.707106781186548,0.131414580971466,-0.694787886990046));
#42051=DIRECTION('ref_axis',(-0.700866150214853,0.,-0.713292814686235));
#42052=DIRECTION('',(0.595596683047426,-0.640307864722779,0.485046832292573));
#42053=DIRECTION('',(0.,-0.98257845275387,-0.185848282703424));
#42054=DIRECTION('',(0.,0.98257845275387,0.185848282703424));
#42055=DIRECTION('',(0.557191914001245,0.501410699557114,0.661909722954177));
#42056=DIRECTION('center_axis',(1.,0.,0.));
#42057=DIRECTION('ref_axis',(0.,-0.996194698091746,-0.0871557427476579));
#42058=DIRECTION('',(0.,0.0871557427476579,-0.996194698091746));
#42059=DIRECTION('',(0.,0.999923093828728,-0.0124018719548356));
#42060=DIRECTION('center_axis',(0.707106781186545,0.704416026402761,0.0616284167162194));
#42061=DIRECTION('ref_axis',(0.0868265938642479,0.,-0.996223440096615));
#42062=DIRECTION('',(0.557191914001243,-0.501410699557115,-0.661909722954177));
#42063=DIRECTION('',(0.,-0.0871557427476579,0.996194698091746));
#42064=DIRECTION('',(0.7055163357783,-0.708673928947921,0.00528794662205797));
#42065=DIRECTION('center_axis',(0.,0.797113049929628,-0.603830096659555));
#42066=DIRECTION('ref_axis',(-1.,0.,0.));
#42067=DIRECTION('',(-1.,0.,0.));
#42068=DIRECTION('',(0.,0.603830096659555,0.797113049929628));
#42069=DIRECTION('',(1.,0.,0.));
#42070=DIRECTION('center_axis',(0.561006631580408,0.56303512813933,0.606846771272561));
#42071=DIRECTION('ref_axis',(0.734296425103052,0.,-0.67882896231737));
#42072=DIRECTION('',(0.,0.733073789207257,-0.680149115692518));
#42073=DIRECTION('',(-0.705516335778304,-0.0582779485356025,0.706293409755774));
#42074=DIRECTION('center_axis',(-0.561006631580394,0.659859195364389,-0.499857381275781));
#42075=DIRECTION('ref_axis',(-0.665244232298933,0.,0.746625817523747));
#42076=DIRECTION('',(0.705516335778303,0.0652539879547265,-0.705683085390291));
#42077=DIRECTION('',(-0.705516335778317,-0.696989337290998,-0.128267547152788));
#42078=DIRECTION('center_axis',(-0.707106781186548,0.131414580971466,-0.694787886990046));
#42079=DIRECTION('ref_axis',(-0.700866150214853,0.,0.713292814686235));
#42080=DIRECTION('',(0.,0.98257845275387,0.185848282703424));
#42081=DIRECTION('',(0.,-0.98257845275387,-0.185848282703424));
#42082=DIRECTION('center_axis',(-0.561006631580393,0.563035128139338,0.606846771272568));
#42083=DIRECTION('ref_axis',(0.734296425103066,0.,0.678828962317356));
#42084=DIRECTION('',(0.705516335778314,0.708673928947907,-0.00528794662205805));
#42085=DIRECTION('',(-0.705516335778305,0.0582779485356274,-0.706293409755771));
#42086=DIRECTION('',(0.,-0.733073789207257,0.680149115692518));
#42087=DIRECTION('center_axis',(-0.707106781186548,0.00876944775867152,
0.707052400311326));
#42088=DIRECTION('ref_axis',(0.707079589180542,0.,0.707133972146916));
#42089=DIRECTION('',(0.,0.999923093828728,-0.0124018719548356));
#42090=DIRECTION('',(0.,-0.999923093828728,0.0124018719548356));
#42091=DIRECTION('center_axis',(0.,0.680149115692518,0.733073789207257));
#42092=DIRECTION('ref_axis',(1.,0.,0.));
#42093=DIRECTION('',(-1.,0.,0.));
#42094=DIRECTION('',(1.,0.,0.));
#42095=DIRECTION('center_axis',(-0.707106781186531,0.704416026402775,0.0616284167162206));
#42096=DIRECTION('ref_axis',(0.0868265938642514,0.,0.996223440096614));
#42097=DIRECTION('',(0.,0.0871557427476579,-0.996194698091746));
#42098=DIRECTION('',(0.,-0.0871557427476579,0.996194698091746));
#42099=DIRECTION('center_axis',(0.707106781186549,0.0087694477586715,0.707052400311324));
#42100=DIRECTION('ref_axis',(0.70707958918054,0.,-0.707133972146918));
#42101=DIRECTION('',(0.,-0.999923093828728,0.0124018719548356));
#42102=DIRECTION('center_axis',(0.,0.185848282703424,-0.98257845275387));
#42103=DIRECTION('ref_axis',(0.,0.98257845275387,0.185848282703424));
#42104=DIRECTION('center_axis',(0.,0.996194698091746,0.0871557427476579));
#42105=DIRECTION('ref_axis',(0.,-0.0871557427476579,0.996194698091746));
#42106=DIRECTION('center_axis',(0.561006631580397,0.700913673242075,-0.440444754748105));
#42107=DIRECTION('ref_axis',(-0.61752142013301,0.,-0.786554064052123));
#42108=DIRECTION('',(0.705516335778305,-0.126510010281499,0.697310488411388));
#42109=DIRECTION('',(0.,-0.532059360920012,-0.846707054687386));
#42110=DIRECTION('',(-0.705516335778308,0.683157829093256,0.188526073789645));
#42111=DIRECTION('center_axis',(0.561006631580402,0.508002428407548,0.653609280881817));
#42112=DIRECTION('ref_axis',(0.758814655754524,0.,-0.651306623804904));
#42113=DIRECTION('',(0.70551633577831,-0.706438085609211,-0.0564971782546651));
#42114=DIRECTION('',(0.,0.789563123475625,-0.613669352377496));
#42115=DIRECTION('',(-0.705516335778302,-0.119613710071869,0.698526492205414));
#42116=DIRECTION('center_axis',(-0.561006631580396,0.700913673242077,-0.440444754748103));
#42117=DIRECTION('ref_axis',(-0.617521420133008,0.,0.786554064052124));
#42118=DIRECTION('',(0.,0.532059360920012,0.846707054687386));
#42119=DIRECTION('',(0.705516335778306,0.126510010281499,-0.697310488411387));
#42120=DIRECTION('',(-0.70551633577831,-0.683157829093255,-0.188526073789644));
#42121=DIRECTION('center_axis',(-0.707106781186544,0.191469263158417,-0.680690473905414));
#42122=DIRECTION('ref_axis',(-0.693521587324702,0.,0.720435845800739));
#42123=DIRECTION('',(0.,0.962641699975202,0.270778428736215));
#42124=DIRECTION('',(0.,-0.962641699975202,-0.270778428736215));
#42125=DIRECTION('center_axis',(-0.561006631580396,0.50800242840755,0.65360928088182));
#42126=DIRECTION('ref_axis',(0.758814655754529,0.,0.651306623804899));
#42127=DIRECTION('',(0.705516335778312,0.70643808560921,0.0564971782546587));
#42128=DIRECTION('',(-0.705516335778307,0.119613710071869,-0.69852649220541));
#42129=DIRECTION('',(0.,-0.789563123475625,0.613669352377496));
#42130=DIRECTION('center_axis',(-0.707106781186545,-0.0528875997482672,
0.705126160196082));
#42131=DIRECTION('ref_axis',(0.706114387365564,0.,0.708097784176278));
#42132=DIRECTION('',(0.,0.997198978933359,0.0747943608453591));
#42133=DIRECTION('',(0.,-0.997198978933359,-0.0747943608453591));
#42134=DIRECTION('center_axis',(0.,0.613669352377496,0.789563123475625));
#42135=DIRECTION('ref_axis',(1.,0.,0.));
#42136=DIRECTION('',(-1.,0.,0.));
#42137=DIRECTION('',(1.,0.,0.));
#42138=DIRECTION('center_axis',(-0.707106781186541,0.696364240320025,0.122787803968974));
#42139=DIRECTION('ref_axis',(0.171087869746038,0.,0.985255774317391));
#42140=DIRECTION('',(0.,0.17364817766693,-0.984807753012208));
#42141=DIRECTION('',(0.,-0.17364817766693,0.984807753012208));
#42142=DIRECTION('center_axis',(0.,0.846707054687386,-0.532059360920012));
#42143=DIRECTION('ref_axis',(-1.,0.,0.));
#42144=DIRECTION('',(-1.,0.,0.));
#42145=DIRECTION('',(1.,0.,0.));
#42146=DIRECTION('center_axis',(0.707106781186549,-0.0528875997482668,0.705126160196077));
#42147=DIRECTION('ref_axis',(0.706114387365559,0.,-0.708097784176282));
#42148=DIRECTION('',(0.,0.997198978933359,0.0747943608453591));
#42149=DIRECTION('',(0.,-0.997198978933359,-0.0747943608453591));
#42150=DIRECTION('center_axis',(0.707106781186543,0.696364240320023,0.122787803968973));
#42151=DIRECTION('ref_axis',(0.171087869746037,0.,-0.985255774317392));
#42152=DIRECTION('',(0.,0.17364817766693,-0.984807753012208));
#42153=DIRECTION('',(0.,-0.17364817766693,0.984807753012208));
#42154=DIRECTION('center_axis',(0.707106781186546,0.191469263158416,-0.680690473905413));
#42155=DIRECTION('ref_axis',(-0.6935215873247,0.,-0.72043584580074));
#42156=DIRECTION('',(0.,0.962641699975202,0.270778428736215));
#42157=DIRECTION('',(0.,-0.962641699975202,-0.270778428736215));
#42158=DIRECTION('center_axis',(1.,0.,0.));
#42159=DIRECTION('ref_axis',(0.,-0.984807753012208,-0.17364817766693));
#42160=DIRECTION('center_axis',(0.,0.270778428736215,-0.962641699975202));
#42161=DIRECTION('ref_axis',(0.,0.962641699975202,0.270778428736215));
#42162=DIRECTION('center_axis',(0.,0.984807753012208,0.17364817766693));
#42163=DIRECTION('ref_axis',(0.,-0.17364817766693,0.984807753012208));
#42164=DIRECTION('center_axis',(0.561006631580423,0.449103523455315,0.69539742920348));
#42165=DIRECTION('ref_axis',(0.778302413620312,0.,-0.627889602520059));
#42166=DIRECTION('',(0.705516335778304,-0.698825821880051,-0.117852325490961));
#42167=DIRECTION('',(0.,0.840043405623103,-0.542519194747189));
#42168=DIRECTION('',(-0.705516335778305,-0.18003913904971,0.685443366267552));
#42169=DIRECTION('center_axis',(0.,0.542519194747189,0.840043405623103));
#42170=DIRECTION('ref_axis',(1.,0.,0.));
#42171=DIRECTION('',(0.557191914001254,-0.697558392670345,0.450499122958952));
#42172=DIRECTION('',(1.,0.,0.));
#42173=DIRECTION('',(-1.,0.,0.));
#42174=DIRECTION('',(-0.557191914001225,-0.697558392670361,0.450499122958962));
#42175=DIRECTION('center_axis',(0.707106781186551,-0.114142140686715,0.697833484234921));
#42176=DIRECTION('ref_axis',(0.702424227635739,0.,-0.711758529580317));
#42177=DIRECTION('',(0.,0.986885577683101,0.161421363397451));
#42178=DIRECTION('',(0.,-0.986885577683101,-0.161421363397451));
#42179=DIRECTION('center_axis',(0.561006631580397,0.736633774843151,-0.377680077688971));
#42180=DIRECTION('ref_axis',(-0.558457227212239,0.,-0.829533317820579));
#42181=DIRECTION('',(0.705516335778306,-0.186803215041196,0.68363093756809));
#42182=DIRECTION('',(0.,-0.456239332177628,-0.889857107503285));
#42183=DIRECTION('',(-0.705516335778302,0.664127077314132,0.247349803169817));
#42184=DIRECTION('center_axis',(0.,0.889857107503285,-0.456239332177628));
#42185=DIRECTION('ref_axis',(0.,0.456239332177628,0.889857107503285));
#42186=DIRECTION('',(0.557191914001234,0.378853727196106,0.738922881200238));
#42187=DIRECTION('',(1.,0.,0.));
#42188=DIRECTION('',(-1.,0.,0.));
#42189=DIRECTION('',(-0.557191914001251,0.3788537271961,0.738922881200227));
#42190=DIRECTION('center_axis',(0.707106781186553,0.683012701892214,0.183012701892218));
#42191=DIRECTION('ref_axis',(0.250562807085727,0.,-0.968100345886376));
#42192=DIRECTION('',(0.,0.25881904510252,-0.965925826289068));
#42193=DIRECTION('',(0.,-0.25881904510252,0.965925826289068));
#42194=DIRECTION('center_axis',(0.707106781186545,0.250066748640429,-0.661412595302212));
#42195=DIRECTION('ref_axis',(-0.683116152038588,0.,-0.730309744439983));
#42196=DIRECTION('',(0.,0.935378662600772,0.353647787425838));
#42197=DIRECTION('',(0.,-0.935378662600772,-0.353647787425838));
#42198=DIRECTION('center_axis',(-0.70710678118655,-0.114142140686715,0.697833484234922));
#42199=DIRECTION('ref_axis',(0.702424227635741,0.,0.711758529580316));
#42200=DIRECTION('',(-0.595596683047418,-0.435796788410821,-0.674793116705948));
#42201=DIRECTION('',(0.,-0.986885577683101,-0.161421363397451));
#42202=DIRECTION('',(0.,0.986885577683101,0.161421363397451));
#42203=DIRECTION('center_axis',(0.,0.965925826289068,0.25881904510252));
#42204=DIRECTION('ref_axis',(0.,-0.25881904510252,0.965925826289068));
#42205=DIRECTION('',(0.,0.25881904510252,-0.965925826289068));
#42206=DIRECTION('center_axis',(-0.707106781186552,0.683012701892215,0.183012701892218));
#42207=DIRECTION('ref_axis',(0.250562807085728,0.,0.968100345886376));
#42208=DIRECTION('',(0.595596683047428,0.714807648004415,-0.366489587160805));
#42209=DIRECTION('',(0.,-0.25881904510252,0.965925826289068));
#42210=DIRECTION('center_axis',(-0.707106781186544,0.25006674864043,-0.661412595302213));
#42211=DIRECTION('ref_axis',(-0.683116152038589,0.,0.730309744439982));
#42212=DIRECTION('',(0.,-0.935378662600772,-0.353647787425838));
#42213=DIRECTION('',(0.,0.935378662600772,0.353647787425838));
#42214=DIRECTION('center_axis',(0.,0.353647787425838,-0.935378662600772));
#42215=DIRECTION('ref_axis',(0.,0.935378662600772,0.353647787425838));
#42216=DIRECTION('center_axis',(0.,-0.161421363397451,0.986885577683101));
#42217=DIRECTION('ref_axis',(0.,-0.986885577683101,-0.161421363397451));
#42218=DIRECTION('center_axis',(0.561006631580414,0.766747648626018,-0.312041027189167));
#42219=DIRECTION('ref_axis',(-0.486084108127399,0.,-0.873912032086749));
#42220=DIRECTION('',(0.705516335778304,-0.245674734539573,0.66474854250225));
#42221=DIRECTION('',(0.,-0.376947046632547,-0.926234810420662));
#42222=DIRECTION('',(-0.7055163357783,0.640041917465767,0.304291051193926));
#42223=DIRECTION('center_axis',(0.561006631580401,0.386786669513441,0.731893183196505));
#42224=DIRECTION('ref_axis',(0.793664727118314,0.,-0.60835540675514));
#42225=DIRECTION('',(0.705516335778305,-0.685895071683811,-0.178310545369065));
#42226=DIRECTION('',(0.,0.884130450221741,-0.467240138462762));
#42227=DIRECTION('',(-0.70551633577831,-0.23909436146888,0.667143602430344));
#42228=DIRECTION('center_axis',(-0.561006631580397,0.766747648626028,-0.312041027189172));
#42229=DIRECTION('ref_axis',(-0.486084108127415,0.,0.87391203208674));
#42230=DIRECTION('',(0.,0.376947046632547,0.926234810420662));
#42231=DIRECTION('',(0.705516335778304,0.245674734539547,-0.66474854250226));
#42232=DIRECTION('',(-0.705516335778316,-0.640041917465754,-0.304291051193919));
#42233=DIRECTION('center_axis',(-0.707106781186547,0.306761075170857,-0.637100967476915));
#42234=DIRECTION('ref_axis',(-0.669373784875801,0.,0.742925794491647));
#42235=DIRECTION('',(0.,0.900996828806872,0.433825672914778));
#42236=DIRECTION('',(0.,-0.900996828806872,-0.433825672914778));
#42237=DIRECTION('center_axis',(-0.561006631580399,0.386786669513442,0.731893183196506));
#42238=DIRECTION('ref_axis',(0.793664727118316,0.,0.608355406755138));
#42239=DIRECTION('',(0.705516335778319,0.685895071683797,0.178310545369067));
#42240=DIRECTION('',(-0.705516335778301,0.239094361468901,-0.667143602430345));
#42241=DIRECTION('',(0.,-0.884130450221741,0.467240138462762));
#42242=DIRECTION('center_axis',(-0.707106781186545,-0.17452799101363,0.685229874095366));
#42243=DIRECTION('ref_axis',(0.695910561235547,0.,0.718128463967852));
#42244=DIRECTION('',(0.,0.96906138128887,0.246819851905204));
#42245=DIRECTION('',(0.,-0.96906138128887,-0.246819851905204));
#42246=DIRECTION('center_axis',(0.,0.467240138462762,0.884130450221741));
#42247=DIRECTION('ref_axis',(1.,0.,0.));
#42248=DIRECTION('',(-1.,0.,0.));
#42249=DIRECTION('',(1.,0.,0.));
#42250=DIRECTION('center_axis',(-0.707106781186536,0.664463024388686,0.241844762647979));
#42251=DIRECTION('ref_axis',(0.323615577118194,0.,0.946188648339462));
#42252=DIRECTION('',(0.,0.342020143325668,-0.939692620785909));
#42253=DIRECTION('',(0.,-0.342020143325668,0.939692620785909));
#42254=DIRECTION('center_axis',(0.,0.926234810420662,-0.376947046632547));
#42255=DIRECTION('ref_axis',(0.,0.376947046632547,0.926234810420662));
#42256=DIRECTION('',(-1.,0.,0.));
#42257=DIRECTION('',(1.,0.,0.));
#42258=DIRECTION('center_axis',(0.70710678118654,-0.174527991013631,0.68522987409537));
#42259=DIRECTION('ref_axis',(0.695910561235552,0.,-0.718128463967847));
#42260=DIRECTION('',(0.,0.96906138128887,0.246819851905204));
#42261=DIRECTION('',(0.,-0.96906138128887,-0.246819851905204));
#42262=DIRECTION('center_axis',(0.707106781186551,0.664463024388672,0.241844762647974));
#42263=DIRECTION('ref_axis',(0.323615577118181,0.,-0.946188648339466));
#42264=DIRECTION('',(0.,0.342020143325668,-0.939692620785909));
#42265=DIRECTION('',(0.,-0.342020143325668,0.939692620785909));
#42266=DIRECTION('center_axis',(0.707106781186549,0.306761075170856,-0.637100967476913));
#42267=DIRECTION('ref_axis',(-0.669373784875799,0.,-0.742925794491649));
#42268=DIRECTION('',(0.,0.900996828806872,0.433825672914778));
#42269=DIRECTION('',(0.,-0.900996828806872,-0.433825672914778));
#42270=DIRECTION('center_axis',(1.,0.,0.));
#42271=DIRECTION('ref_axis',(0.,-0.939692620785909,-0.342020143325668));
#42272=DIRECTION('center_axis',(0.,0.433825672914778,-0.900996828806872));
#42273=DIRECTION('ref_axis',(0.,0.900996828806872,0.433825672914778));
#42274=DIRECTION('center_axis',(0.,0.939692620785909,0.342020143325668));
#42275=DIRECTION('ref_axis',(0.,-0.342020143325668,0.939692620785909));
#42276=DIRECTION('center_axis',(0.561006631580415,0.791026109827961,-0.24402715605694));
#42277=DIRECTION('ref_axis',(-0.398879012810059,0.,-0.917003562228453));
#42278=DIRECTION('',(0.705516335778313,-0.302676520965626,0.640807009641818));
#42279=DIRECTION('',(0.,-0.294785966455749,-0.955563307154869));
#42280=DIRECTION('',(-0.705516335778295,0.611085652157605,0.358916460582518));
#42281=DIRECTION('center_axis',(0.561006631580423,0.321526135468429,0.762818788136163));
#42282=DIRECTION('ref_axis',(0.805595332751379,0.,-0.592466167683181));
#42283=DIRECTION('',(0.705516335778303,-0.667744245837286,-0.237411714330086));
#42284=DIRECTION('',(0.,0.921488728241597,-0.388405102597383));
#42285=DIRECTION('',(-0.705516335778304,-0.296329931428055,0.643766472946362));
#42286=DIRECTION('center_axis',(-0.561006631580412,0.791026109827963,-0.244027156056944));
#42287=DIRECTION('ref_axis',(-0.398879012810066,0.,0.91700356222845));
#42288=DIRECTION('',(0.,0.294785966455749,0.955563307154869));
#42289=DIRECTION('',(0.705516335778314,0.302676520965625,-0.640807009641816));
#42290=DIRECTION('',(-0.705516335778296,-0.611085652157604,-0.358916460582518));
#42291=DIRECTION('center_axis',(-0.70710678118654,0.361120764691836,-0.607940616597043));
#42292=DIRECTION('ref_axis',(-0.65193371809419,0.,0.758275957163278));
#42293=DIRECTION('',(0.,0.859757865108992,0.510701883081733));
#42294=DIRECTION('',(0.,-0.859757865108992,-0.510701883081733));
#42295=DIRECTION('center_axis',(-0.561006631580421,0.321526135468429,0.762818788136165));
#42296=DIRECTION('ref_axis',(0.80559533275138,0.,0.592466167683179));
#42297=DIRECTION('',(0.705516335778305,0.667744245837285,0.237411714330086));
#42298=DIRECTION('',(-0.705516335778306,0.296329931428054,-0.643766472946361));
#42299=DIRECTION('',(0.,-0.921488728241597,0.388405102597383));
#42300=DIRECTION('center_axis',(-0.70710678118655,-0.233585577946046,0.667411250860823));
#42301=DIRECTION('ref_axis',(0.686399640790371,0.,0.727224541062009));
#42302=DIRECTION('',(0.,0.943862042647771,0.330339892306057));
#42303=DIRECTION('',(0.,-0.943862042647771,-0.330339892306057));
#42304=DIRECTION('center_axis',(0.,0.388405102597383,0.921488728241597));
#42305=DIRECTION('ref_axis',(1.,0.,0.));
#42306=DIRECTION('',(-1.,0.,0.));
#42307=DIRECTION('',(1.,0.,0.));
#42308=DIRECTION('center_axis',(-0.707106781186552,0.640856382055784,0.298836238730117));
#42309=DIRECTION('ref_axis',(0.38928162063502,0.,0.921118787038769));
#42310=DIRECTION('',(0.,0.422618261740699,-0.90630778703665));
#42311=DIRECTION('',(0.,-0.422618261740699,0.90630778703665));
#42312=DIRECTION('center_axis',(0.,0.955563307154869,-0.294785966455749));
#42313=DIRECTION('ref_axis',(0.,0.294785966455749,0.955563307154869));
#42314=DIRECTION('',(-1.,0.,0.));
#42315=DIRECTION('',(1.,0.,0.));
#42316=DIRECTION('center_axis',(0.707106781186551,-0.233585577946045,0.667411250860822));
#42317=DIRECTION('ref_axis',(0.68639964079037,0.,-0.72722454106201));
#42318=DIRECTION('',(0.,0.943862042647771,0.330339892306057));
#42319=DIRECTION('',(0.,-0.943862042647771,-0.330339892306057));
#42320=DIRECTION('center_axis',(0.707106781186554,0.640856382055783,0.298836238730117));
#42321=DIRECTION('ref_axis',(0.389281620635018,0.,-0.921118787038769));
#42322=DIRECTION('',(0.,0.422618261740699,-0.90630778703665));
#42323=DIRECTION('',(0.,-0.422618261740699,0.90630778703665));
#42324=DIRECTION('center_axis',(0.707106781186542,0.361120764691835,-0.607940616597042));
#42325=DIRECTION('ref_axis',(-0.651933718094189,0.,-0.758275957163279));
#42326=DIRECTION('',(0.,0.859757865108992,0.510701883081733));
#42327=DIRECTION('',(0.,-0.859757865108992,-0.510701883081733));
#42328=DIRECTION('center_axis',(1.,0.,0.));
#42329=DIRECTION('ref_axis',(0.,-0.90630778703665,-0.422618261740699));
#42330=DIRECTION('center_axis',(0.,0.510701883081733,-0.859757865108992));
#42331=DIRECTION('ref_axis',(0.,0.859757865108992,0.510701883081733));
#42332=DIRECTION('center_axis',(0.,0.90630778703665,0.422618261740699));
#42333=DIRECTION('ref_axis',(0.,-0.422618261740699,0.90630778703665));
#42334=DIRECTION('center_axis',(0.707106781186547,0.412732107142825,-0.574153470540276));
#42335=DIRECTION('ref_axis',(-0.630347388214433,0.,-0.776313190774988));
#42336=DIRECTION('',(0.595596683047424,-0.785305653025387,0.168995924416173));
#42337=DIRECTION('',(0.,-0.81197562492164,-0.583691343548209));
#42338=DIRECTION('',(0.,0.81197562492164,0.583691343548209));
#42339=DIRECTION('',(0.557191914001233,0.17469728496797,0.81179925449366));
#42340=DIRECTION('center_axis',(1.,0.,0.));
#42341=DIRECTION('ref_axis',(0.,-0.866025403784439,-0.5));
#42342=DIRECTION('',(0.,0.5,-0.866025403784438));
#42343=DIRECTION('',(0.,0.911479343942638,0.411345846661781));
#42344=DIRECTION('center_axis',(0.707106781186549,0.612372435695794,0.353553390593273));
#42345=DIRECTION('ref_axis',(0.447213595499957,0.,-0.894427190999916));
#42346=DIRECTION('',(0.557191914001247,-0.174697284967968,-0.811799254493651));
#42347=DIRECTION('',(0.,-0.5,0.866025403784439));
#42348=DIRECTION('',(0.705516335778306,-0.644511483084942,-0.29470603679192));
#42349=DIRECTION('center_axis',(0.,0.977619390136729,-0.210381387077589));
#42350=DIRECTION('ref_axis',(0.,0.210381387077589,0.977619390136729));
#42351=DIRECTION('',(-1.,0.,0.));
#42352=DIRECTION('',(0.,0.210381387077589,0.977619390136729));
#42353=DIRECTION('',(1.,0.,0.));
#42354=DIRECTION('center_axis',(0.561006631580424,0.253818593389699,0.787938881495552));
#42355=DIRECTION('ref_axis',(0.814616058663767,0.,-0.580000583592042));
#42356=DIRECTION('',(0.,0.951833920629441,-0.306614069375799));
#42357=DIRECTION('',(-0.705516335778296,-0.351310251680218,0.615489891886414));
#42358=DIRECTION('center_axis',(-0.561006631580398,0.809284384699505,-0.174156090919495));
#42359=DIRECTION('ref_axis',(-0.296477762129661,0.,0.955039756535082));
#42360=DIRECTION('',(0.705516335778309,0.357374756306019,-0.611988548508191));
#42361=DIRECTION('',(-0.705516335778307,-0.577478656052904,-0.410810298986385));
#42362=DIRECTION('center_axis',(-0.707106781186546,0.412732107142826,-0.574153470540278));
#42363=DIRECTION('ref_axis',(-0.630347388214435,0.,0.776313190774987));
#42364=DIRECTION('',(0.,0.81197562492164,0.583691343548209));
#42365=DIRECTION('',(0.,-0.81197562492164,-0.583691343548209));
#42366=DIRECTION('center_axis',(-0.561006631580422,0.253818593389699,0.787938881495553));
#42367=DIRECTION('ref_axis',(0.814616058663768,0.,0.580000583592041));
#42368=DIRECTION('',(0.705516335778308,0.644511483084941,0.294706036791919));
#42369=DIRECTION('',(-0.705516335778297,0.351310251680217,-0.615489891886412));
#42370=DIRECTION('',(0.,-0.951833920629441,0.306614069375799));
#42371=DIRECTION('center_axis',(-0.707106781186555,-0.290865437587464,0.644513225013298));
#42372=DIRECTION('ref_axis',(0.67363868643895,0.,0.739060836557321));
#42373=DIRECTION('',(0.,0.911479343942638,0.411345846661781));
#42374=DIRECTION('',(0.,-0.911479343942638,-0.411345846661781));
#42375=DIRECTION('center_axis',(0.,0.306614069375799,0.951833920629441));
#42376=DIRECTION('ref_axis',(1.,0.,0.));
#42377=DIRECTION('',(-1.,0.,0.));
#42378=DIRECTION('',(1.,0.,0.));
#42379=DIRECTION('center_axis',(-0.707106781186547,0.612372435695795,0.353553390593274));
#42380=DIRECTION('ref_axis',(0.447213595499958,0.,0.894427190999916));
#42381=DIRECTION('',(0.,0.5,-0.866025403784439));
#42382=DIRECTION('',(0.,-0.5,0.866025403784439));
#42383=DIRECTION('center_axis',(0.707106781186557,-0.290865437587463,0.644513225013297));
#42384=DIRECTION('ref_axis',(0.673638686438948,0.,-0.739060836557322));
#42385=DIRECTION('',(0.,-0.911479343942638,-0.411345846661781));
#42386=DIRECTION('center_axis',(0.,0.583691343548209,-0.81197562492164));
#42387=DIRECTION('ref_axis',(0.,0.81197562492164,0.583691343548209));
#42388=DIRECTION('center_axis',(0.,0.866025403784439,0.5));
#42389=DIRECTION('ref_axis',(0.,-0.5,0.866025403784439));
#42390=DIRECTION('center_axis',(0.561006631580409,0.8213835167442,-0.1029595927718));
#42391=DIRECTION('ref_axis',(-0.180511696561723,0.,-0.983572837874455));
#42392=DIRECTION('',(0.705516335778304,-0.409353153962201,0.578512484991598));
#42393=DIRECTION('',(0.,-0.124375678311979,-0.992235199256928));
#42394=DIRECTION('',(-0.705516335778303,0.539476698684503,0.459577622960939));
#42395=DIRECTION('center_axis',(0.561006631580412,0.184179338555415,0.807062284196263));
#42396=DIRECTION('ref_axis',(0.821109284001915,0.,-0.570771008133614));
#42397=DIRECTION('',(0.705516335778304,-0.616373598779652,-0.349757468365403));
#42398=DIRECTION('',(0.,0.97493508214826,-0.222489517947625));
#42399=DIRECTION('',(-0.705516335778314,-0.403616888790129,0.582529061106241));
#42400=DIRECTION('center_axis',(-0.561006631580389,0.821383516744213,-0.1029595927718));
#42401=DIRECTION('ref_axis',(-0.18051169656173,0.,0.983572837874453));
#42402=DIRECTION('',(0.,0.124375678311979,0.992235199256928));
#42403=DIRECTION('',(0.705516335778303,0.409353153962173,-0.578512484991619));
#42404=DIRECTION('',(-0.705516335778318,-0.539476698684487,-0.459577622960934));
#42405=DIRECTION('center_axis',(-0.707106781186546,0.461202309044001,-0.535996669889361));
#42406=DIRECTION('ref_axis',(-0.604079438549194,0.,0.79692410675176));
#42407=DIRECTION('',(0.,0.758013759944347,0.652238560447812));
#42408=DIRECTION('',(0.,-0.758013759944347,-0.652238560447812));
#42409=DIRECTION('center_axis',(-0.561006631580396,0.184179338555417,0.807062284196274));
#42410=DIRECTION('ref_axis',(0.821109284001927,0.,0.570771008133598));
#42411=DIRECTION('',(0.70551633577832,0.616373598779638,0.349757468365396));
#42412=DIRECTION('',(-0.705516335778313,0.403616888790152,-0.582529061106225));
#42413=DIRECTION('',(0.,-0.97493508214826,0.222489517947625));
#42414=DIRECTION('center_axis',(-0.707106781186539,-0.345931635619497,0.616710064355716));
#42415=DIRECTION('ref_axis',(0.657291420225588,0.,0.753636509796221));
#42416=DIRECTION('',(0.,0.872159737063827,0.489221210746995));
#42417=DIRECTION('',(0.,-0.872159737063827,-0.489221210746995));
#42418=DIRECTION('center_axis',(0.,0.222489517947625,0.97493508214826));
#42419=DIRECTION('ref_axis',(1.,0.,0.));
#42420=DIRECTION('',(-1.,0.,0.));
#42421=DIRECTION('',(1.,0.,0.));
#42422=DIRECTION('center_axis',(-0.707106781186532,0.579227965339582,0.405579787672648));
#42423=DIRECTION('ref_axis',(0.49754281216454,0.,0.867439421552538));
#42424=DIRECTION('',(0.,0.573576436351046,-0.819152044288992));
#42425=DIRECTION('',(0.,-0.573576436351046,0.819152044288992));
#42426=DIRECTION('center_axis',(0.,0.992235199256928,-0.124375678311979));
#42427=DIRECTION('ref_axis',(0.,0.124375678311979,0.992235199256928));
#42428=DIRECTION('',(-1.,0.,0.));
#42429=DIRECTION('',(1.,0.,0.));
#42430=DIRECTION('center_axis',(0.707106781186546,-0.345931635619494,0.61671006435571));
#42431=DIRECTION('ref_axis',(0.657291420225581,0.,-0.753636509796227));
#42432=DIRECTION('',(0.,0.872159737063827,0.489221210746995));
#42433=DIRECTION('',(0.,-0.872159737063827,-0.489221210746995));
#42434=DIRECTION('center_axis',(0.707106781186547,0.579227965339569,0.405579787672639));
#42435=DIRECTION('ref_axis',(0.497542812164523,0.,-0.867439421552547));
#42436=DIRECTION('',(0.,0.573576436351046,-0.819152044288992));
#42437=DIRECTION('',(0.,-0.573576436351046,0.819152044288992));
#42438=DIRECTION('center_axis',(0.707106781186547,0.461202309044,-0.53599666988936));
#42439=DIRECTION('ref_axis',(-0.604079438549193,0.,-0.796924106751761));
#42440=DIRECTION('',(0.,0.758013759944347,0.652238560447812));
#42441=DIRECTION('',(0.,-0.758013759944347,-0.652238560447812));
#42442=DIRECTION('center_axis',(1.,0.,0.));
#42443=DIRECTION('ref_axis',(0.,-0.819152044288992,-0.573576436351046));
#42444=DIRECTION('center_axis',(0.,0.652238560447812,-0.758013759944347));
#42445=DIRECTION('ref_axis',(0.,0.758013759944347,0.652238560447812));
#42446=DIRECTION('center_axis',(0.,0.819152044288992,0.573576436351046));
#42447=DIRECTION('ref_axis',(0.,-0.573576436351046,0.819152044288992));
#42448=DIRECTION('center_axis',(0.561006631580388,0.113138367744187,0.820043455596719));
#42449=DIRECTION('ref_axis',(0.825342782028786,0.,-0.564631997103409));
#42450=DIRECTION('',(0.705516335778318,-0.58354473921108,-0.402147034415285));
#42451=DIRECTION('',(0.,0.990616399010033,-0.136671686945011));
#42452=DIRECTION('',(-0.705516335778308,-0.452851757665877,0.545134832430359));
#42453=DIRECTION('center_axis',(0.,0.136671686945011,0.990616399010033));
#42454=DIRECTION('ref_axis',(1.,0.,0.));
#42455=DIRECTION('',(0.557191914001244,-0.822591759450536,0.113489947817864));
#42456=DIRECTION('',(1.,0.,0.));
#42457=DIRECTION('',(-1.,0.,0.));
#42458=DIRECTION('',(-0.557191914001257,-0.822591759450527,0.113489947817863));
#42459=DIRECTION('center_axis',(0.707106781186542,-0.398365085025226,0.584213367728652));
#42460=DIRECTION('ref_axis',(0.636934375125937,0.,-0.770918025332741));
#42461=DIRECTION('',(0.,0.826202467961513,0.563373306018581));
#42462=DIRECTION('',(0.,-0.826202467961513,-0.563373306018581));
#42463=DIRECTION('center_axis',(0.561006631580411,0.827231424261544,-0.0309795099544489));
#42464=DIRECTION('ref_axis',(-0.0551372865288087,0.,-0.998478782766184));
#42465=DIRECTION('',(0.705516335778302,-0.458216126942503,0.540633592148851));
#42466=DIRECTION('',(0.,-0.0374233955343756,-0.999299499382781));
#42467=DIRECTION('',(-0.705516335778315,0.497368997894199,0.504847283724158));
#42468=DIRECTION('center_axis',(0.,0.999299499382782,-0.0374233955343756));
#42469=DIRECTION('ref_axis',(0.,0.0374233955343756,0.999299499382781));
#42470=DIRECTION('',(0.557191914001262,0.0310757794924442,0.829802064892916));
#42471=DIRECTION('',(1.,0.,0.));
#42472=DIRECTION('',(-1.,0.,0.));
#42473=DIRECTION('',(-0.55719191400123,0.031075779492445,0.829802064892937));
#42474=DIRECTION('center_axis',(0.707106781186541,0.541675220419707,0.454519477672047));
#42475=DIRECTION('ref_axis',(0.540716203060943,0.,-0.841205080671388));
#42476=DIRECTION('',(0.,0.642787609686539,-0.766044443118978));
#42477=DIRECTION('',(0.,-0.642787609686539,0.766044443118978));
#42478=DIRECTION('center_axis',(0.707106781186551,0.50616248289178,-0.493760610936944));
#42479=DIRECTION('ref_axis',(-0.572517134274666,0.,-0.819892755768658));
#42480=DIRECTION('',(0.,0.698282952552655,0.715821848069997));
#42481=DIRECTION('',(0.,-0.698282952552655,-0.715821848069997));
#42482=DIRECTION('center_axis',(-0.70710678118654,-0.398365085025227,0.584213367728653));
#42483=DIRECTION('ref_axis',(0.636934375125939,0.,0.770918025332739));
#42484=DIRECTION('',(-0.595596683047433,-0.109786128885423,-0.795745937499683));
#42485=DIRECTION('',(0.,-0.826202467961513,-0.563373306018581));
#42486=DIRECTION('',(0.,0.826202467961513,0.563373306018581));
#42487=DIRECTION('center_axis',(0.,0.766044443118978,0.642787609686539));
#42488=DIRECTION('ref_axis',(0.,-0.642787609686539,0.766044443118978));
#42489=DIRECTION('',(0.,0.642787609686539,-0.766044443118978));
#42490=DIRECTION('center_axis',(-0.70710678118654,0.541675220419708,0.454519477672048));
#42491=DIRECTION('ref_axis',(0.540716203060945,0.,0.841205080671387));
#42492=DIRECTION('',(0.595596683047426,0.802720929891721,-0.0300616010331307));
#42493=DIRECTION('',(0.,-0.642787609686539,0.766044443118978));
#42494=DIRECTION('center_axis',(-0.707106781186549,0.506162482891781,-0.493760610936946));
#42495=DIRECTION('ref_axis',(-0.572517134274668,0.,0.819892755768657));
#42496=DIRECTION('',(0.,-0.698282952552655,-0.715821848069997));
#42497=DIRECTION('',(0.,0.698282952552655,0.715821848069997));
#42498=DIRECTION('center_axis',(0.,0.715821848069997,-0.698282952552655));
#42499=DIRECTION('ref_axis',(0.,0.698282952552655,0.715821848069997));
#42500=DIRECTION('center_axis',(0.,-0.563373306018581,0.826202467961513));
#42501=DIRECTION('ref_axis',(0.,-0.826202467961513,-0.563373306018581));
#42502=DIRECTION('center_axis',(0.561006631580404,0.826783601144275,0.0412363456396565));
#42503=DIRECTION('ref_axis',(0.0733064378127414,0.,-0.997309463594529));
#42504=DIRECTION('',(0.705516335778296,-0.503591798518335,0.498640151226349));
#42505=DIRECTION('',(0.,0.0498137018801831,-0.998758526924798));
#42506=DIRECTION('',(-0.705516335778313,0.451476018710252,0.546274751823186));
#42507=DIRECTION('center_axis',(0.561006631580394,0.041236345639636,0.826783601144283));
#42508=DIRECTION('ref_axis',(0.827487445286316,0.,-0.561484218739517));
#42509=DIRECTION('',(0.705516335778303,-0.546274751823203,-0.451476018710246));
#42510=DIRECTION('',(0.,0.998758526924799,-0.049813701880158));
#42511=DIRECTION('',(-0.705516335778304,-0.498640151226356,0.503591798518316));
#42512=DIRECTION('center_axis',(-0.561006631580402,0.826783601144276,0.0412363456396566));
#42513=DIRECTION('ref_axis',(0.0733064378127418,0.,0.997309463594529));
#42514=DIRECTION('',(0.,-0.0498137018801831,0.998758526924798));
#42515=DIRECTION('',(0.705516335778297,0.503591798518334,-0.498640151226348));
#42516=DIRECTION('',(-0.705516335778315,-0.451476018710251,-0.546274751823184));
#42517=DIRECTION('center_axis',(-0.70710678118655,0.547270454615492,-0.447766735594494));
#42518=DIRECTION('ref_axis',(-0.534994468449985,0.,0.844855560867015));
#42519=DIRECTION('',(0.,0.633237790257263,0.773957299203321));
#42520=DIRECTION('',(0.,-0.633237790257263,-0.773957299203321));
#42521=DIRECTION('center_axis',(-0.561006631580393,0.0412363456396361,0.826783601144284));
#42522=DIRECTION('ref_axis',(0.827487445286317,0.,0.561484218739515));
#42523=DIRECTION('',(0.705516335778305,0.546274751823202,0.451476018710245));
#42524=DIRECTION('',(-0.705516335778306,0.498640151226354,-0.503591798518315));
#42525=DIRECTION('',(0.,-0.998758526924799,0.049813701880158));
#42526=DIRECTION('center_axis',(-0.70710678118655,-0.447766735594494,0.547270454615492));
#42527=DIRECTION('ref_axis',(0.61205637248212,0.,0.790814135498366));
#42528=DIRECTION('',(0.,0.773957299203321,0.633237790257263));
#42529=DIRECTION('',(0.,-0.773957299203321,-0.633237790257263));
#42530=DIRECTION('center_axis',(0.,0.049813701880158,0.998758526924799));
#42531=DIRECTION('ref_axis',(1.,0.,0.));
#42532=DIRECTION('',(-1.,0.,0.));
#42533=DIRECTION('',(1.,0.,0.));
#42534=DIRECTION('center_axis',(-0.707106781186538,0.500000000000007,0.500000000000007));
#42535=DIRECTION('ref_axis',(0.577350269189637,0.,0.816496580927719));
#42536=DIRECTION('',(0.,0.707106781186547,-0.707106781186548));
#42537=DIRECTION('',(0.,-0.707106781186547,0.707106781186548));
#42538=DIRECTION('center_axis',(0.,0.998758526924798,0.0498137018801831));
#42539=DIRECTION('ref_axis',(0.,-0.0498137018801831,0.998758526924798));
#42540=DIRECTION('',(-1.,0.,0.));
#42541=DIRECTION('',(1.,0.,0.));
#42542=DIRECTION('center_axis',(0.707106781186551,-0.447766735594493,0.547270454615491));
#42543=DIRECTION('ref_axis',(0.612056372482119,0.,-0.790814135498367));
#42544=DIRECTION('',(0.,0.773957299203321,0.633237790257263));
#42545=DIRECTION('',(0.,-0.773957299203321,-0.633237790257263));
#42546=DIRECTION('center_axis',(0.707106781186539,0.500000000000006,0.500000000000006));
#42547=DIRECTION('ref_axis',(0.577350269189635,0.,-0.81649658092772));
#42548=DIRECTION('',(0.,0.707106781186547,-0.707106781186548));
#42549=DIRECTION('',(0.,-0.707106781186547,0.707106781186548));
#42550=DIRECTION('center_axis',(0.707106781186551,0.547270454615491,-0.447766735594493));
#42551=DIRECTION('ref_axis',(-0.534994468449984,0.,-0.844855560867016));
#42552=DIRECTION('',(0.,0.633237790257263,0.773957299203321));
#42553=DIRECTION('',(0.,-0.633237790257263,-0.773957299203321));
#42554=DIRECTION('center_axis',(1.,0.,0.));
#42555=DIRECTION('ref_axis',(0.,-0.707106781186548,-0.707106781186547));
#42556=DIRECTION('center_axis',(0.,0.773957299203321,-0.633237790257263));
#42557=DIRECTION('ref_axis',(0.,0.633237790257263,0.773957299203321));
#42558=DIRECTION('center_axis',(0.,0.707106781186548,0.707106781186547));
#42559=DIRECTION('ref_axis',(0.,-0.707106781186547,0.707106781186548));
#42560=DIRECTION('center_axis',(0.561006631580392,0.820043455596711,0.113138367744223));
#42561=DIRECTION('ref_axis',(0.197690230426254,0.,-0.98026454225072));
#42562=DIRECTION('',(0.705516335778306,-0.545134832430383,0.452851757665851));
#42563=DIRECTION('',(0.,0.136671686945054,-0.990616399010027));
#42564=DIRECTION('',(-0.705516335778304,0.402147034415252,0.583544739211119));
#42565=DIRECTION('center_axis',(0.561006631580441,-0.0309795099544276,0.827231424261525));
#42566=DIRECTION('ref_axis',(0.827628669643362,0.,-0.561276032968057));
#42567=DIRECTION('',(0.705516335778297,-0.50484728372417,-0.497368997894212));
#42568=DIRECTION('',(0.,0.999299499382783,0.0374233955343508));
#42569=DIRECTION('',(-0.705516335778286,-0.540633592148838,0.458216126942542));
#42570=DIRECTION('center_axis',(-0.561006631580388,0.820043455596714,0.113138367744223));
#42571=DIRECTION('ref_axis',(0.197690230426256,0.,0.98026454225072));
#42572=DIRECTION('',(0.,-0.136671686945054,0.990616399010027));
#42573=DIRECTION('',(0.7055163357783,0.545134832430375,-0.45285175766587));
#42574=DIRECTION('',(-0.705516335778316,-0.402147034415257,-0.583544739211101));
#42575=DIRECTION('center_axis',(-0.707106781186557,0.584213367728639,-0.398365085025217));
#42576=DIRECTION('ref_axis',(-0.490839120629124,0.,0.871250226777605));
#42577=DIRECTION('',(0.,0.563373306018581,0.826202467961512));
#42578=DIRECTION('',(0.,-0.563373306018581,-0.826202467961512));
#42579=DIRECTION('center_axis',(-0.561006631580419,-0.0309795099544281,
0.82723142426154));
#42580=DIRECTION('ref_axis',(0.827628669643377,0.,0.561276032968035));
#42581=DIRECTION('',(0.705516335778307,0.504847283724175,0.497368997894192));
#42582=DIRECTION('',(-0.705516335778296,0.540633592148843,-0.458216126942521));
#42583=DIRECTION('',(0.,-0.999299499382783,-0.0374233955343508));
#42584=DIRECTION('center_axis',(-0.707106781186558,-0.493760610936939,0.506162482891775));
#42585=DIRECTION('ref_axis',(0.582064997116532,0.,0.813142262541882));
#42586=DIRECTION('',(0.,0.715821848069998,0.698282952552655));
#42587=DIRECTION('',(0.,-0.715821848069998,-0.698282952552655));
#42588=DIRECTION('center_axis',(0.,-0.0374233955343508,0.999299499382783));
#42589=DIRECTION('ref_axis',(1.,0.,0.));
#42590=DIRECTION('',(-1.,0.,0.));
#42591=DIRECTION('',(1.,0.,0.));
#42592=DIRECTION('center_axis',(-0.707106781186548,0.454519477672044,0.541675220419701));
#42593=DIRECTION('ref_axis',(0.608120402411342,0.,0.793844806099446));
#42594=DIRECTION('',(0.,0.766044443118978,-0.64278760968654));
#42595=DIRECTION('',(0.,-0.766044443118978,0.64278760968654));
#42596=DIRECTION('center_axis',(0.,0.990616399010027,0.136671686945054));
#42597=DIRECTION('ref_axis',(0.,-0.136671686945054,0.990616399010027));
#42598=DIRECTION('',(-1.,0.,0.));
#42599=DIRECTION('',(1.,0.,0.));
#42600=DIRECTION('center_axis',(0.70710678118656,-0.493760610936938,0.506162482891773));
#42601=DIRECTION('ref_axis',(0.58206499711653,0.,-0.813142262541883));
#42602=DIRECTION('',(0.,0.715821848069998,0.698282952552655));
#42603=DIRECTION('',(0.,-0.715821848069998,-0.698282952552655));
#42604=DIRECTION('center_axis',(0.707106781186559,0.454519477672036,0.541675220419693));
#42605=DIRECTION('ref_axis',(0.60812040241133,0.,-0.793844806099455));
#42606=DIRECTION('',(0.,0.766044443118978,-0.64278760968654));
#42607=DIRECTION('',(0.,-0.766044443118978,0.64278760968654));
#42608=DIRECTION('center_axis',(0.707106781186542,0.584213367728652,-0.398365085025226));
#42609=DIRECTION('ref_axis',(-0.490839120629141,0.,-0.871250226777595));
#42610=DIRECTION('',(0.,0.563373306018581,0.826202467961512));
#42611=DIRECTION('',(0.,-0.563373306018581,-0.826202467961512));
#42612=DIRECTION('center_axis',(1.,0.,0.));
#42613=DIRECTION('ref_axis',(0.,-0.64278760968654,-0.766044443118978));
#42614=DIRECTION('center_axis',(0.,0.826202467961512,-0.563373306018581));
#42615=DIRECTION('ref_axis',(0.,0.563373306018581,0.826202467961512));
#42616=DIRECTION('center_axis',(0.,0.64278760968654,0.766044443118978));
#42617=DIRECTION('ref_axis',(0.,-0.766044443118978,0.64278760968654));
#42618=DIRECTION('center_axis',(0.707106781186552,0.616710064355705,-0.345931635619491));
#42619=DIRECTION('ref_axis',(-0.439451044888509,0.,-0.898266541259552));
#42620=DIRECTION('',(0.595596683047423,-0.783149392358838,-0.178722187740891));
#42621=DIRECTION('',(0.,-0.489221210746995,-0.872159737063827));
#42622=DIRECTION('',(0.,0.489221210746995,0.872159737063827));
#42623=DIRECTION('',(0.557191914001246,-0.184751680075907,0.809570248762118));
#42624=DIRECTION('center_axis',(1.,0.,0.));
#42625=DIRECTION('ref_axis',(0.,-0.573576436351046,-0.819152044288992));
#42626=DIRECTION('',(0.,0.819152044288992,-0.573576436351046));
#42627=DIRECTION('',(0.,0.652238560447812,0.758013759944346));
#42628=DIRECTION('center_axis',(0.707106781186547,0.405579787672639,0.579227965339569));
#42629=DIRECTION('ref_axis',(0.633687274224642,0.,-0.773589321594955));
#42630=DIRECTION('',(0.557191914001238,0.184751680075908,-0.809570248762123));
#42631=DIRECTION('',(0.,-0.819152044288992,0.573576436351046));
#42632=DIRECTION('',(0.705516335778303,-0.459577622960939,-0.539476698684503));
#42633=DIRECTION('center_axis',(0.,0.974935082148257,0.222489517947637));
#42634=DIRECTION('ref_axis',(0.,-0.222489517947637,0.974935082148257));
#42635=DIRECTION('',(-1.,0.,0.));
#42636=DIRECTION('',(0.,-0.222489517947637,0.974935082148257));
#42637=DIRECTION('',(1.,0.,0.));
#42638=DIRECTION('center_axis',(0.561006631580418,-0.10295959277178,0.821383516744196));
#42639=DIRECTION('ref_axis',(0.825772049781954,0.,-0.564004008672731));
#42640=DIRECTION('',(0.,0.992235199256931,0.124375678311957));
#42641=DIRECTION('',(-0.705516335778302,-0.578512484991583,0.409353153962224));
#42642=DIRECTION('center_axis',(-0.561006631580406,0.807062284196265,0.184179338555426));
#42643=DIRECTION('ref_axis',(0.311921838389608,0.,0.950107765853773));
#42644=DIRECTION('',(0.705516335778296,0.582529061106236,-0.403616888790167));
#42645=DIRECTION('',(-0.705516335778309,-0.349757468365391,-0.616373598779654));
#42646=DIRECTION('center_axis',(-0.70710678118655,0.616710064355706,-0.345931635619492));
#42647=DIRECTION('ref_axis',(-0.43945104488851,0.,0.898266541259551));
#42648=DIRECTION('',(0.,0.489221210746995,0.872159737063827));
#42649=DIRECTION('',(0.,-0.489221210746995,-0.872159737063827));
#42650=DIRECTION('center_axis',(-0.561006631580395,-0.102959592771782,0.821383516744211));
#42651=DIRECTION('ref_axis',(0.82577204978197,0.,0.564004008672708));
#42652=DIRECTION('',(0.70551633577831,0.459577622960954,0.539476698684481));
#42653=DIRECTION('',(-0.705516335778316,0.57851248499158,-0.409353153962206));
#42654=DIRECTION('',(0.,-0.992235199256931,-0.124375678311957));
#42655=DIRECTION('center_axis',(-0.707106781186541,-0.535996669889364,0.461202309044004));
#42656=DIRECTION('ref_axis',(0.546305769586294,0.,0.837585820150226));
#42657=DIRECTION('',(0.,0.652238560447812,0.758013759944346));
#42658=DIRECTION('',(0.,-0.652238560447812,-0.758013759944346));
#42659=DIRECTION('center_axis',(0.,-0.124375678311957,0.992235199256931));
#42660=DIRECTION('ref_axis',(1.,0.,0.));
#42661=DIRECTION('',(-1.,0.,0.));
#42662=DIRECTION('',(1.,0.,0.));
#42663=DIRECTION('center_axis',(-0.707106781186546,0.40557978767264,0.579227965339571));
#42664=DIRECTION('ref_axis',(0.633687274224644,0.,0.773589321594954));
#42665=DIRECTION('',(0.,0.819152044288992,-0.573576436351046));
#42666=DIRECTION('',(0.,-0.819152044288992,0.573576436351046));
#42667=DIRECTION('center_axis',(0.707106781186552,-0.535996669889356,0.461202309043997));
#42668=DIRECTION('ref_axis',(0.546305769586282,0.,-0.837585820150234));
#42669=DIRECTION('',(0.,-0.652238560447812,-0.758013759944346));
#42670=DIRECTION('center_axis',(0.,0.872159737063827,-0.489221210746995));
#42671=DIRECTION('ref_axis',(0.,0.489221210746995,0.872159737063827));
#42672=DIRECTION('center_axis',(0.,0.573576436351046,0.819152044288992));
#42673=DIRECTION('ref_axis',(0.,-0.819152044288992,0.573576436351046));
#42674=DIRECTION('center_axis',(0.561006631580402,0.787938881495568,0.253818593389698));
#42675=DIRECTION('ref_axis',(0.412208150462332,0.,-0.911089699586393));
#42676=DIRECTION('',(0.7055163357783,-0.615489891886393,0.351310251680245));
#42677=DIRECTION('',(0.,0.306614069375792,-0.951833920629443));
#42678=DIRECTION('',(-0.705516335778309,0.294706036791908,0.644511483084945));
#42679=DIRECTION('center_axis',(0.561006631580397,-0.174156090919455,0.809284384699514));
#42680=DIRECTION('ref_axis',(0.821843752318944,0.,-0.569712951208166));
#42681=DIRECTION('',(0.705516335778309,-0.410810298986413,-0.577478656052882));
#42682=DIRECTION('',(0.,0.97761939013674,0.210381387077539));
#42683=DIRECTION('',(-0.705516335778306,-0.611988548508179,0.357374756306044));
#42684=DIRECTION('center_axis',(-0.561006631580411,0.787938881495565,0.253818593389687));
#42685=DIRECTION('ref_axis',(0.412208150462312,0.,0.911089699586402));
#42686=DIRECTION('',(0.,-0.306614069375792,0.951833920629443));
#42687=DIRECTION('',(0.705516335778308,0.615489891886397,-0.351310251680223));
#42688=DIRECTION('',(-0.705516335778296,-0.294706036791914,-0.644511483084956));
#42689=DIRECTION('center_axis',(-0.707106781186549,0.644513225013303,-0.290865437587467));
#42690=DIRECTION('ref_axis',(-0.380418570543387,0.,0.924814419862561));
#42691=DIRECTION('',(0.,0.411345846661781,0.911479343942638));
#42692=DIRECTION('',(0.,-0.411345846661781,-0.911479343942638));
#42693=DIRECTION('center_axis',(-0.561006631580409,-0.174156090919453,0.809284384699506));
#42694=DIRECTION('ref_axis',(0.821843752318936,0.,0.569712951208178));
#42695=DIRECTION('',(0.705516335778289,0.410810298986437,0.577478656052889));
#42696=DIRECTION('',(-0.705516335778318,0.611988548508149,-0.357374756306074));
#42697=DIRECTION('',(0.,-0.97761939013674,-0.210381387077539));
#42698=DIRECTION('center_axis',(-0.707106781186536,-0.574153470540286,0.412732107142832));
#42699=DIRECTION('ref_axis',(0.504101701135483,0.,0.863644298836224));
#42700=DIRECTION('',(0.,0.583691343548209,0.811975624921639));
#42701=DIRECTION('',(0.,-0.583691343548209,-0.811975624921639));
#42702=DIRECTION('center_axis',(0.,-0.210381387077539,0.97761939013674));
#42703=DIRECTION('ref_axis',(1.,0.,0.));
#42704=DIRECTION('',(-1.,0.,0.));
#42705=DIRECTION('',(1.,0.,0.));
#42706=DIRECTION('center_axis',(-0.707106781186558,0.353553390593269,0.612372435695785));
#42707=DIRECTION('ref_axis',(0.654653670707966,0.,0.755928946018464));
#42708=DIRECTION('',(0.,0.866025403784438,-0.5));
#42709=DIRECTION('',(0.,-0.866025403784438,0.5));
#42710=DIRECTION('center_axis',(0.,0.951833920629443,0.306614069375792));
#42711=DIRECTION('ref_axis',(0.,-0.306614069375792,0.951833920629443));
#42712=DIRECTION('',(-1.,0.,0.));
#42713=DIRECTION('',(1.,0.,0.));
#42714=DIRECTION('center_axis',(0.707106781186547,-0.574153470540276,0.412732107142825));
#42715=DIRECTION('ref_axis',(0.504101701135471,0.,-0.863644298836231));
#42716=DIRECTION('',(0.,0.583691343548209,0.811975624921639));
#42717=DIRECTION('',(0.,-0.583691343548209,-0.811975624921639));
#42718=DIRECTION('center_axis',(0.707106781186545,0.353553390593275,0.612372435695796));
#42719=DIRECTION('ref_axis',(0.654653670707979,0.,-0.755928946018453));
#42720=DIRECTION('',(0.,0.866025403784438,-0.5));
#42721=DIRECTION('',(0.,-0.866025403784438,0.5));
#42722=DIRECTION('center_axis',(0.707106781186551,0.644513225013302,-0.290865437587466));
#42723=DIRECTION('ref_axis',(-0.380418570543386,0.,-0.924814419862562));
#42724=DIRECTION('',(0.,0.411345846661781,0.911479343942638));
#42725=DIRECTION('',(0.,-0.411345846661781,-0.911479343942638));
#42726=DIRECTION('center_axis',(1.,0.,0.));
#42727=DIRECTION('ref_axis',(0.,-0.5,-0.866025403784438));
#42728=DIRECTION('center_axis',(0.,0.911479343942638,-0.411345846661781));
#42729=DIRECTION('ref_axis',(0.,0.411345846661781,0.911479343942638));
#42730=DIRECTION('center_axis',(0.,0.5,0.866025403784438));
#42731=DIRECTION('ref_axis',(0.,-0.866025403784438,0.5));
#42732=DIRECTION('center_axis',(0.561006631580396,-0.244027156056938,0.791026109827976));
#42733=DIRECTION('ref_axis',(0.815685591418261,0.,-0.578495476173014));
#42734=DIRECTION('',(0.705516335778303,-0.358916460582535,-0.611085652157587));
#42735=DIRECTION('',(0.,0.955563307154871,0.294785966455742));
#42736=DIRECTION('',(-0.705516335778307,-0.640807009641837,0.302676520965598));
#42737=DIRECTION('center_axis',(0.,-0.294785966455742,0.955563307154871));
#42738=DIRECTION('ref_axis',(1.,0.,0.));
#42739=DIRECTION('',(0.557191914001242,-0.793484241614032,-0.244785476043487));
#42740=DIRECTION('',(1.,0.,0.));
#42741=DIRECTION('',(-1.,0.,0.));
#42742=DIRECTION('',(-0.557191914001242,-0.793484241614032,-0.244785476043487));
#42743=DIRECTION('center_axis',(0.707106781186547,-0.607940616597037,0.361120764691833));
#42744=DIRECTION('ref_axis',(0.454822071931221,0.,-0.890582327965355));
#42745=DIRECTION('',(0.,0.510701883081734,0.859757865108992));
#42746=DIRECTION('',(0.,-0.510701883081734,-0.859757865108992));
#42747=DIRECTION('center_axis',(0.561006631580424,0.762818788136169,0.321526135468413));
#42748=DIRECTION('ref_axis',(0.497247150959849,0.,-0.867608938901803));
#42749=DIRECTION('',(0.705516335778299,-0.643766472946357,0.296329931428078));
#42750=DIRECTION('',(0.,0.388405102597364,-0.921488728241605));
#42751=DIRECTION('',(-0.705516335778301,0.237411714330098,0.667744245837284));
#42752=DIRECTION('center_axis',(0.,0.921488728241605,0.388405102597364));
#42753=DIRECTION('ref_axis',(0.,-0.388405102597364,0.921488728241605));
#42754=DIRECTION('',(0.557191914001242,-0.322525285311673,0.765189265022881));
#42755=DIRECTION('',(1.,0.,0.));
#42756=DIRECTION('',(-1.,0.,0.));
#42757=DIRECTION('',(-0.557191914001238,-0.322525285311674,0.765189265022883));
#42758=DIRECTION('center_axis',(0.707106781186551,0.298836238730119,0.640856382055785));
#42759=DIRECTION('ref_axis',(0.671542934237814,0.,-0.740965645273293));
#42760=DIRECTION('',(0.,0.90630778703665,-0.4226182617407));
#42761=DIRECTION('',(0.,-0.90630778703665,0.4226182617407));
#42762=DIRECTION('center_axis',(0.707106781186551,0.667411250860821,-0.233585577946046));
#42763=DIRECTION('ref_axis',(-0.313668483594039,0.,-0.949532559947165));
#42764=DIRECTION('',(0.,0.330339892306058,0.943862042647771));
#42765=DIRECTION('',(0.,-0.330339892306058,-0.943862042647771));
#42766=DIRECTION('center_axis',(-0.707106781186546,-0.607940616597038,0.361120764691834));
#42767=DIRECTION('ref_axis',(0.454822071931223,0.,0.890582327965354));
#42768=DIRECTION('',(-0.595596683047429,0.236796741375871,-0.767588362611542));
#42769=DIRECTION('',(0.,-0.510701883081734,-0.859757865108992));
#42770=DIRECTION('',(0.,0.510701883081734,0.859757865108992));
#42771=DIRECTION('center_axis',(0.,0.4226182617407,0.90630778703665));
#42772=DIRECTION('ref_axis',(0.,-0.90630778703665,0.4226182617407));
#42773=DIRECTION('',(0.,0.90630778703665,-0.4226182617407));
#42774=DIRECTION('center_axis',(-0.70710678118655,0.298836238730119,0.640856382055786));
#42775=DIRECTION('ref_axis',(0.671542934237816,0.,0.740965645273291));
#42776=DIRECTION('',(0.595596683047418,0.740216811151934,0.311999460946611));
#42777=DIRECTION('',(0.,-0.90630778703665,0.4226182617407));
#42778=DIRECTION('center_axis',(-0.70710678118655,0.667411250860823,-0.233585577946047));
#42779=DIRECTION('ref_axis',(-0.31366848359404,0.,0.949532559947164));
#42780=DIRECTION('',(0.,-0.330339892306058,-0.943862042647771));
#42781=DIRECTION('',(0.,0.330339892306058,0.943862042647771));
#42782=DIRECTION('center_axis',(0.,0.943862042647771,-0.330339892306058));
#42783=DIRECTION('ref_axis',(0.,0.330339892306058,0.943862042647771));
#42784=DIRECTION('center_axis',(0.,-0.859757865108992,0.510701883081734));
#42785=DIRECTION('ref_axis',(0.,-0.510701883081734,-0.859757865108992));
#42786=DIRECTION('center_axis',(0.561006631580406,0.731893183196498,0.386786669513448));
#42787=DIRECTION('ref_axis',(0.567619122871711,0.,-0.823291279773052));
#42788=DIRECTION('',(0.705516335778304,-0.667143602430351,0.239094361468878));
#42789=DIRECTION('',(0.,0.467240138462772,-0.884130450221736));
#42790=DIRECTION('',(-0.705516335778305,0.178310545369065,0.685895071683811));
#42791=DIRECTION('center_axis',(0.561006631580414,-0.312041027189174,0.766747648626015));
#42792=DIRECTION('ref_axis',(0.80704448738357,0.,-0.59049063953952));
#42793=DIRECTION('',(0.705516335778303,-0.304291051193915,-0.64004191746577));
#42794=DIRECTION('',(0.,0.926234810420659,0.376947046632555));
#42795=DIRECTION('',(-0.70551633577831,-0.664748542502243,0.245674734539575));
#42796=DIRECTION('center_axis',(-0.561006631580404,0.731893183196499,0.386786669513448));
#42797=DIRECTION('ref_axis',(0.567619122871712,0.,0.823291279773051));
#42798=DIRECTION('',(0.,-0.467240138462772,0.884130450221736));
#42799=DIRECTION('',(0.705516335778315,0.667143602430346,-0.239094361468855));
#42800=DIRECTION('',(-0.705516335778296,-0.178310545369049,-0.685895071683825));
#42801=DIRECTION('center_axis',(-0.707106781186539,0.685229874095371,-0.174527991013632));
#42802=DIRECTION('ref_axis',(-0.239628661022764,0.,0.97086461714105));
#42803=DIRECTION('',(0.,0.246819851905205,0.96906138128887));
#42804=DIRECTION('',(0.,-0.246819851905205,-0.96906138128887));
#42805=DIRECTION('center_axis',(-0.561006631580427,-0.312041027189171,0.766747648626007));
#42806=DIRECTION('ref_axis',(0.80704448738356,0.,0.590490639539533));
#42807=DIRECTION('',(0.705516335778291,0.304291051193921,0.640041917465781));
#42808=DIRECTION('',(-0.705516335778313,0.664748542502231,-0.2456747345396));
#42809=DIRECTION('',(0.,-0.926234810420659,-0.376947046632555));
#42810=DIRECTION('center_axis',(-0.707106781186541,-0.637100967476919,0.30676107517086));
#42811=DIRECTION('ref_axis',(0.397987666358449,0.,0.917390765937044));
#42812=DIRECTION('',(0.,0.433825672914779,0.900996828806872));
#42813=DIRECTION('',(0.,-0.433825672914779,-0.900996828806872));
#42814=DIRECTION('center_axis',(0.,-0.376947046632555,0.926234810420659));
#42815=DIRECTION('ref_axis',(1.,0.,0.));
#42816=DIRECTION('',(-1.,0.,0.));
#42817=DIRECTION('',(1.,0.,0.));
#42818=DIRECTION('center_axis',(-0.707106781186561,0.241844762647971,0.664463024388662));
#42819=DIRECTION('ref_axis',(0.684791078771722,0.,0.728739444818696));
#42820=DIRECTION('',(0.,0.939692620785908,-0.342020143325669));
#42821=DIRECTION('',(0.,-0.939692620785908,0.342020143325669));
#42822=DIRECTION('center_axis',(0.,0.884130450221736,0.467240138462772));
#42823=DIRECTION('ref_axis',(0.,-0.467240138462772,0.884130450221736));
#42824=DIRECTION('',(-1.,0.,0.));
#42825=DIRECTION('',(1.,0.,0.));
#42826=DIRECTION('center_axis',(0.707106781186543,-0.637100967476918,0.306761075170859));
#42827=DIRECTION('ref_axis',(0.397987666358448,0.,-0.917390765937044));
#42828=DIRECTION('',(0.,0.433825672914779,0.900996828806872));
#42829=DIRECTION('',(0.,-0.433825672914779,-0.900996828806872));
#42830=DIRECTION('center_axis',(0.707106781186551,0.241844762647975,0.664463024388671));
#42831=DIRECTION('ref_axis',(0.684791078771732,0.,-0.728739444818686));
#42832=DIRECTION('',(0.,0.939692620785908,-0.342020143325669));
#42833=DIRECTION('',(0.,-0.939692620785908,0.342020143325669));
#42834=DIRECTION('center_axis',(0.707106781186549,0.685229874095361,-0.174527991013629));
#42835=DIRECTION('ref_axis',(-0.239628661022757,0.,-0.970864617141052));
#42836=DIRECTION('',(0.,0.246819851905205,0.96906138128887));
#42837=DIRECTION('',(0.,-0.246819851905205,-0.96906138128887));
#42838=DIRECTION('center_axis',(1.,0.,0.));
#42839=DIRECTION('ref_axis',(0.,-0.342020143325669,-0.939692620785908));
#42840=DIRECTION('center_axis',(0.,0.96906138128887,-0.246819851905205));
#42841=DIRECTION('ref_axis',(0.,0.246819851905205,0.96906138128887));
#42842=DIRECTION('center_axis',(0.,0.342020143325669,0.939692620785908));
#42843=DIRECTION('ref_axis',(0.,-0.939692620785908,0.342020143325669));
#42844=DIRECTION('center_axis',(0.561006631580403,0.695397429203503,0.449103523455304));
#42845=DIRECTION('ref_axis',(0.62494805391789,0.,-0.780666337114802));
#42846=DIRECTION('',(0.705516335778305,-0.685443366267539,0.18003913904976));
#42847=DIRECTION('',(0.,0.542519194747167,-0.840043405623117));
#42848=DIRECTION('',(-0.705516335778305,0.117852325490942,0.698825821880052));
#42849=DIRECTION('center_axis',(0.561006631580396,-0.37768007768899,0.736633774843142));
#42850=DIRECTION('ref_axis',(0.795555689966284,0.,-0.605880470193808));
#42851=DIRECTION('',(0.705516335778306,-0.2473498031698,-0.664127077314135));
#42852=DIRECTION('',(0.,0.889857107503274,0.456239332177649));
#42853=DIRECTION('',(-0.705516335778303,-0.683630937568099,0.186803215041171));
#42854=DIRECTION('center_axis',(-0.561006631580402,0.695397429203504,0.449103523455304));
#42855=DIRECTION('ref_axis',(0.624948053917891,0.,0.780666337114801));
#42856=DIRECTION('',(0.,-0.542519194747167,0.840043405623117));
#42857=DIRECTION('',(0.705516335778306,0.685443366267538,-0.180039139049759));
#42858=DIRECTION('',(-0.705516335778307,-0.117852325490942,-0.698825821880051));
#42859=DIRECTION('center_axis',(-0.707106781186546,0.697833484234925,-0.114142140686716));
#42860=DIRECTION('ref_axis',(-0.159358523666364,0.,0.987220776186805));
#42861=DIRECTION('',(0.,0.161421363397451,0.986885577683101));
#42862=DIRECTION('',(0.,-0.161421363397451,-0.986885577683101));
#42863=DIRECTION('center_axis',(-0.561006631580394,-0.37768007768899,0.736633774843143));
#42864=DIRECTION('ref_axis',(0.795555689966285,0.,0.605880470193806));
#42865=DIRECTION('',(0.705516335778307,0.247349803169799,0.664127077314133));
#42866=DIRECTION('',(-0.705516335778305,0.683630937568098,-0.18680321504117));
#42867=DIRECTION('',(0.,-0.889857107503274,-0.456239332177649));
#42868=DIRECTION('center_axis',(-0.707106781186544,-0.661412595302213,0.25006674864043));
#42869=DIRECTION('ref_axis',(0.333412439312664,0.,0.942781069661233));
#42870=DIRECTION('',(0.,0.353647787425838,0.935378662600772));
#42871=DIRECTION('',(0.,-0.353647787425838,-0.935378662600772));
#42872=DIRECTION('center_axis',(0.,-0.456239332177649,0.889857107503274));
#42873=DIRECTION('ref_axis',(1.,0.,0.));
#42874=DIRECTION('',(-1.,0.,0.));
#42875=DIRECTION('',(1.,0.,0.));
#42876=DIRECTION('center_axis',(-0.707106781186551,0.183012701892218,0.683012701892216));
#42877=DIRECTION('ref_axis',(0.694746590606862,0.,0.719254596676407));
#42878=DIRECTION('',(0.,0.965925826289068,-0.258819045102521));
#42879=DIRECTION('',(0.,-0.965925826289068,0.258819045102521));
#42880=DIRECTION('center_axis',(0.,0.840043405623117,0.542519194747167));
#42881=DIRECTION('ref_axis',(1.,0.,0.));
#42882=DIRECTION('',(-1.,0.,0.));
#42883=DIRECTION('',(1.,0.,0.));
#42884=DIRECTION('center_axis',(0.707106781186545,-0.661412595302212,0.25006674864043));
#42885=DIRECTION('ref_axis',(0.333412439312663,0.,-0.942781069661234));
#42886=DIRECTION('',(0.,0.353647787425838,0.935378662600772));
#42887=DIRECTION('',(0.,-0.353647787425838,-0.935378662600772));
#42888=DIRECTION('center_axis',(0.707106781186552,0.183012701892218,0.683012701892215));
#42889=DIRECTION('ref_axis',(0.694746590606861,0.,-0.719254596676408));
#42890=DIRECTION('',(0.,0.965925826289068,-0.258819045102521));
#42891=DIRECTION('',(0.,-0.965925826289068,0.258819045102521));
#42892=DIRECTION('center_axis',(0.707106781186548,0.697833484234924,-0.114142140686716));
#42893=DIRECTION('ref_axis',(-0.159358523666364,0.,-0.987220776186805));
#42894=DIRECTION('',(0.,0.161421363397451,0.986885577683101));
#42895=DIRECTION('',(0.,-0.161421363397451,-0.986885577683101));
#42896=DIRECTION('center_axis',(1.,0.,0.));
#42897=DIRECTION('ref_axis',(0.,-0.258819045102521,-0.965925826289068));
#42898=DIRECTION('center_axis',(0.,0.986885577683101,-0.161421363397451));
#42899=DIRECTION('ref_axis',(0.,0.161421363397451,0.986885577683101));
#42900=DIRECTION('center_axis',(0.,0.258819045102521,0.965925826289068));
#42901=DIRECTION('ref_axis',(0.,-0.965925826289068,0.258819045102521));
#42902=DIRECTION('center_axis',(-1.,0.,-9.34622984744497E-15));
#42903=DIRECTION('ref_axis',(0.,-1.,-3.06609014182674E-17));
#42904=DIRECTION('center_axis',(-1.,0.,0.));
#42905=DIRECTION('ref_axis',(0.,-1.,-6.12323399573676E-17));
#42906=DIRECTION('center_axis',(-1.,0.,0.));
#42907=DIRECTION('ref_axis',(0.,-1.,-6.12323399573676E-17));
#42908=DIRECTION('',(0.913500063388735,-0.406838584931147,8.5751308774215E-15));
#42909=DIRECTION('center_axis',(1.,0.,0.));
#42910=DIRECTION('ref_axis',(0.,-1.,0.));
#42911=DIRECTION('center_axis',(1.,0.,0.));
#42912=DIRECTION('ref_axis',(0.,-1.,0.));
#42913=DIRECTION('center_axis',(-1.,0.,0.));
#42914=DIRECTION('ref_axis',(0.,1.,0.));
#42915=DIRECTION('',(-0.668964731622448,-0.743294146247168,-9.10272797026559E-17));
#42916=DIRECTION('center_axis',(1.,0.,0.));
#42917=DIRECTION('ref_axis',(0.,-1.,-6.12323399573677E-17));
#42918=DIRECTION('center_axis',(1.,0.,0.));
#42919=DIRECTION('ref_axis',(0.,-1.,-6.12323399573677E-17));
#42920=DIRECTION('center_axis',(1.,0.,0.));
#42921=DIRECTION('ref_axis',(0.,1.,0.));
#42922=DIRECTION('center_axis',(1.,0.,0.));
#42923=DIRECTION('ref_axis',(0.,0.,-1.));
#42924=DIRECTION('',(-1.,0.,0.));
#42925=DIRECTION('center_axis',(0.561006631580394,0.653609280881836,0.508002428407532));
#42926=DIRECTION('ref_axis',(0.671222048820192,0.,-0.741256339721708));
#42927=DIRECTION('',(0.705516335778306,-0.698526492205406,0.119613710071895));
#42928=DIRECTION('',(0.,0.613669352377473,-0.789563123475643));
#42929=DIRECTION('',(-0.70551633577831,0.0564971782546651,0.706438085609211));
#42930=DIRECTION('center_axis',(0.56100663158039,-0.44044475474812,0.700913673242072));
#42931=DIRECTION('ref_axis',(0.780718990354277,0.,-0.624882275392892));
#42932=DIRECTION('',(0.70551633577831,-0.188526073789633,-0.683157829093258));
#42933=DIRECTION('',(0.,0.846707054687377,0.532059360920026));
#42934=DIRECTION('',(-0.705516335778307,-0.697310488411391,0.126510010281474));
#42935=DIRECTION('center_axis',(-0.561006631580392,0.653609280881837,0.508002428407533));
#42936=DIRECTION('ref_axis',(0.671222048820193,0.,0.741256339721707));
#42937=DIRECTION('',(0.,-0.613669352377473,0.789563123475643));
#42938=DIRECTION('',(0.705516335778308,0.698526492205404,-0.119613710071895));
#42939=DIRECTION('',(-0.705516335778312,-0.056497178254665,-0.70643808560921));
#42940=DIRECTION('center_axis',(-0.707106781186545,0.705126160196082,-0.0528875997482675));
#42941=DIRECTION('ref_axis',(-0.0745860273602106,0.,0.997214582987344));
#42942=DIRECTION('',(0.,0.0747943608453595,0.997198978933359));
#42943=DIRECTION('',(0.,-0.0747943608453595,-0.997198978933359));
#42944=DIRECTION('center_axis',(-0.561006631580385,-0.440444754748121,0.700913673242074));
#42945=DIRECTION('ref_axis',(0.780718990354281,0.,0.624882275392888));
#42946=DIRECTION('',(0.705516335778311,0.188526073789638,0.683157829093256));
#42947=DIRECTION('',(-0.705516335778312,0.697310488411386,-0.126510010281475));
#42948=DIRECTION('',(0.,-0.846707054687377,-0.532059360920026));
#42949=DIRECTION('center_axis',(-0.707106781186541,-0.680690473905417,0.191469263158418));
#42950=DIRECTION('ref_axis',(0.261366100937227,0.,0.965239742903736));
#42951=DIRECTION('',(0.,0.270778428736215,0.962641699975202));
#42952=DIRECTION('',(0.,-0.270778428736215,-0.962641699975202));
#42953=DIRECTION('center_axis',(0.,-0.532059360920026,0.846707054687377));
#42954=DIRECTION('ref_axis',(1.,0.,0.));
#42955=DIRECTION('',(-1.,0.,0.));
#42956=DIRECTION('',(1.,0.,0.));
#42957=DIRECTION('center_axis',(-0.707106781186541,0.122787803968974,0.696364240320026));
#42958=DIRECTION('ref_axis',(0.70167384315987,0.,0.712498293208663));
#42959=DIRECTION('',(0.,0.984807753012208,-0.17364817766693));
#42960=DIRECTION('',(0.,-0.984807753012208,0.17364817766693));
#42961=DIRECTION('center_axis',(0.,0.789563123475643,0.613669352377473));
#42962=DIRECTION('ref_axis',(1.,0.,0.));
#42963=DIRECTION('',(-1.,0.,0.));
#42964=DIRECTION('',(1.,0.,0.));
#42965=DIRECTION('center_axis',(0.707106781186546,-0.680690473905413,0.191469263158417));
#42966=DIRECTION('ref_axis',(0.261366100937224,0.,-0.965239742903737));
#42967=DIRECTION('',(0.,0.270778428736215,0.962641699975202));
#42968=DIRECTION('',(0.,-0.270778428736215,-0.962641699975202));
#42969=DIRECTION('center_axis',(0.707106781186542,0.122787803968974,0.696364240320024));
#42970=DIRECTION('ref_axis',(0.701673843159868,0.,-0.712498293208665));
#42971=DIRECTION('',(0.,0.984807753012208,-0.17364817766693));
#42972=DIRECTION('',(0.,-0.984807753012208,0.17364817766693));
#42973=DIRECTION('center_axis',(0.707106781186546,0.705126160196081,-0.0528875997482674));
#42974=DIRECTION('ref_axis',(-0.0745860273602103,0.,-0.997214582987344));
#42975=DIRECTION('',(0.,0.0747943608453595,0.997198978933359));
#42976=DIRECTION('',(0.,-0.0747943608453595,-0.997198978933359));
#42977=DIRECTION('center_axis',(1.,0.,0.));
#42978=DIRECTION('ref_axis',(0.,-0.17364817766693,-0.984807753012208));
#42979=DIRECTION('center_axis',(0.,0.997198978933359,-0.0747943608453595));
#42980=DIRECTION('ref_axis',(0.,0.0747943608453595,0.997198978933359));
#42981=DIRECTION('center_axis',(0.,0.17364817766693,0.984807753012208));
#42982=DIRECTION('ref_axis',(0.,-0.984807753012208,0.17364817766693));
#42983=DIRECTION('center_axis',(0.561006631580395,0.606846771272568,0.563035128139337));
#42984=DIRECTION('ref_axis',(0.708381704532398,0.,-0.705829554980361));
#42985=DIRECTION('',(0.705516335778303,-0.706293409755772,0.0582779485356275));
#42986=DIRECTION('',(0.,0.680149115692518,-0.733073789207257));
#42987=DIRECTION('',(-0.705516335778312,-0.00528794662206119,0.708673928947909));
#42988=DIRECTION('center_axis',(0.561006631580394,-0.499857381275784,0.659859195364387));
#42989=DIRECTION('ref_axis',(0.761867344215974,0.,-0.64773308531933));
#42990=DIRECTION('',(0.705516335778315,-0.128267547152788,-0.696989337290999));
#42991=DIRECTION('',(0.,0.797113049929625,0.603830096659557));
#42992=DIRECTION('',(-0.705516335778304,-0.70568308539029,0.0652539879547269));
#42993=DIRECTION('center_axis',(-0.561006631580407,0.606846771272561,0.563035128139331));
#42994=DIRECTION('ref_axis',(0.708381704532386,0.,0.705829554980372));
#42995=DIRECTION('',(0.,-0.680149115692518,0.733073789207257));
#42996=DIRECTION('',(0.705516335778306,0.706293409755772,-0.0582779485356024));
#42997=DIRECTION('',(-0.705516335778301,0.00528794662206109,-0.70867392894792));
#42998=DIRECTION('center_axis',(-0.707106781186548,0.707052400311326,0.00876944775867122));
#42999=DIRECTION('ref_axis',(0.0124009183210272,0.,0.999923105656027));
#43000=DIRECTION('',(0.,-0.0124018719548352,0.999923093828728));
#43001=DIRECTION('',(0.,0.0124018719548352,-0.999923093828728));
#43002=DIRECTION('center_axis',(-0.561006631580406,-0.499857381275779,0.659859195364381));
#43003=DIRECTION('ref_axis',(0.761867344215965,0.,0.647733085319341));
#43004=DIRECTION('',(0.705516335778304,0.128267547152789,0.696989337291011));
#43005=DIRECTION('',(-0.705516335778308,0.705683085390284,-0.065253987954752));
#43006=DIRECTION('',(0.,-0.797113049929625,-0.603830096659557));
#43007=DIRECTION('center_axis',(-0.707106781186545,-0.694787886990049,0.131414580971466));
#43008=DIRECTION('ref_axis',(0.182719541232955,0.,0.983165077314903));
#43009=DIRECTION('',(0.,0.185848282703424,0.982578452753869));
#43010=DIRECTION('',(0.,-0.185848282703424,-0.982578452753869));
#43011=DIRECTION('center_axis',(0.,-0.603830096659558,0.797113049929625));
#43012=DIRECTION('ref_axis',(1.,0.,0.));
#43013=DIRECTION('',(-1.,0.,0.));
#43014=DIRECTION('',(1.,0.,0.));
#43015=DIRECTION('center_axis',(-0.707106781186556,0.0616284167162187,0.70441602640275));
#43016=DIRECTION('ref_axis',(0.705757556807943,0.,0.708453436019956));
#43017=DIRECTION('',(0.,0.996194698091746,-0.0871557427476583));
#43018=DIRECTION('',(0.,-0.996194698091746,0.0871557427476583));
#43019=DIRECTION('center_axis',(0.,0.733073789207257,0.680149115692518));
#43020=DIRECTION('ref_axis',(1.,0.,0.));
#43021=DIRECTION('',(-1.,0.,0.));
#43022=DIRECTION('',(1.,0.,0.));
#43023=DIRECTION('center_axis',(0.707106781186546,-0.694787886990048,0.131414580971466));
#43024=DIRECTION('ref_axis',(0.182719541232955,0.,-0.983165077314903));
#43025=DIRECTION('',(0.,0.185848282703424,0.982578452753869));
#43026=DIRECTION('',(0.,-0.185848282703424,-0.982578452753869));
#43027=DIRECTION('center_axis',(0.707106781186545,0.0616284167162197,0.704416026402761));
#43028=DIRECTION('ref_axis',(0.705757556807954,0.,-0.708453436019945));
#43029=DIRECTION('',(0.,0.996194698091746,-0.0871557427476583));
#43030=DIRECTION('',(0.,-0.996194698091746,0.0871557427476583));
#43031=DIRECTION('center_axis',(0.707106781186549,0.707052400311324,0.00876944775867119));
#43032=DIRECTION('ref_axis',(0.0124009183210271,0.,-0.999923105656027));
#43033=DIRECTION('',(0.,-0.0124018719548352,0.999923093828728));
#43034=DIRECTION('',(0.,0.0124018719548352,-0.999923093828728));
#43035=DIRECTION('center_axis',(1.,0.,0.));
#43036=DIRECTION('ref_axis',(0.,-0.0871557427476583,-0.996194698091746));
#43037=DIRECTION('center_axis',(0.,0.999923093828728,0.0124018719548352));
#43038=DIRECTION('ref_axis',(0.,-0.0124018719548352,0.999923093828728));
#43039=DIRECTION('center_axis',(0.,0.0871557427476583,0.996194698091746));
#43040=DIRECTION('ref_axis',(0.,-0.996194698091746,0.0871557427476583));
#43041=DIRECTION('center_axis',(-1.,0.,1.45673360119678E-14));
#43042=DIRECTION('ref_axis',(0.,-1.,-3.05617576116583E-17));
#43043=DIRECTION('center_axis',(-1.,0.,0.));
#43044=DIRECTION('ref_axis',(0.,-1.,-6.12323399573677E-17));
#43045=DIRECTION('center_axis',(-1.,0.,0.));
#43046=DIRECTION('ref_axis',(0.,-1.,-6.12323399573677E-17));
#43047=DIRECTION('',(-0.763019982472722,0.6463748961302,1.12140809161872E-14));
#43048=DIRECTION('center_axis',(1.,0.,0.));
#43049=DIRECTION('ref_axis',(0.,-1.,0.));
#43050=DIRECTION('center_axis',(1.,0.,0.));
#43051=DIRECTION('ref_axis',(0.,-1.,0.));
#43052=DIRECTION('center_axis',(1.,0.,0.));
#43053=DIRECTION('ref_axis',(0.,1.,0.));
#43054=DIRECTION('',(-1.,0.,0.));
#43055=DIRECTION('center_axis',(-1.,0.,0.));
#43056=DIRECTION('ref_axis',(0.,-1.,0.));
#43057=DIRECTION('center_axis',(-1.,0.,0.));
#43058=DIRECTION('ref_axis',(0.,-1.,0.));
#43059=DIRECTION('center_axis',(-1.,0.,0.));
#43060=DIRECTION('ref_axis',(0.,1.,0.));
#43061=DIRECTION('',(-0.164398987305357,-0.986393923832144,-1.20798416151943E-16));
#43062=DIRECTION('center_axis',(-1.,0.,2.35474746642391E-14));
#43063=DIRECTION('ref_axis',(0.,-1.,-3.05127853847422E-17));
#43064=DIRECTION('center_axis',(-1.,0.,0.));
#43065=DIRECTION('ref_axis',(0.,-1.,0.));
#43066=DIRECTION('',(0.358263767183369,-0.933620411689666,-8.35035881523851E-15));
#43067=DIRECTION('center_axis',(-1.,0.,0.));
#43068=DIRECTION('ref_axis',(0.,0.,1.));
#43069=DIRECTION('center_axis',(1.,0.,0.));
#43070=DIRECTION('ref_axis',(0.,-1.,0.));
#43071=DIRECTION('center_axis',(1.,0.,-9.94623938728346E-15));
#43072=DIRECTION('ref_axis',(0.,-1.,-3.05771835236612E-17));
#43073=DIRECTION('center_axis',(1.,0.,0.));
#43074=DIRECTION('ref_axis',(0.,-1.,-6.12323399573677E-17));
#43075=DIRECTION('',(0.923879532511288,0.382683432365087,-9.22429081787917E-15));
#43076=DIRECTION('center_axis',(1.,0.,0.));
#43077=DIRECTION('ref_axis',(0.,-1.,0.));
#43078=DIRECTION('',(-0.707106781186549,-0.707106781186546,-8.65956056235492E-17));
#43079=DIRECTION('center_axis',(-1.,0.,0.));
#43080=DIRECTION('ref_axis',(0.,-1.,-6.12323399573677E-17));
#43081=DIRECTION('center_axis',(1.,0.,2.39616194920574E-14));
#43082=DIRECTION('ref_axis',(0.,-1.,-3.07109033448888E-17));
#43083=DIRECTION('',(-0.382683432365081,-0.92387953251129,-9.31123057850062E-15));
#43084=DIRECTION('center_axis',(0.,-0.982578452753869,0.185848282703424));
#43085=DIRECTION('ref_axis',(0.,-0.185848282703424,-0.982578452753869));
#43086=DIRECTION('center_axis',(1.,0.,0.));
#43087=DIRECTION('ref_axis',(0.,-0.0871557427476583,-0.996194698091746));
#43088=DIRECTION('center_axis',(0.,-0.962641699975202,0.270778428736215));
#43089=DIRECTION('ref_axis',(0.,-0.270778428736215,-0.962641699975202));
#43090=DIRECTION('center_axis',(1.,0.,0.));
#43091=DIRECTION('ref_axis',(0.,-0.17364817766693,-0.984807753012208));
#43092=DIRECTION('center_axis',(0.,-0.935378662600772,0.353647787425838));
#43093=DIRECTION('ref_axis',(0.,-0.353647787425838,-0.935378662600772));
#43094=DIRECTION('center_axis',(1.,0.,0.));
#43095=DIRECTION('ref_axis',(0.,-0.258819045102521,-0.965925826289068));
#43096=DIRECTION('center_axis',(0.,-0.900996828806872,0.433825672914779));
#43097=DIRECTION('ref_axis',(0.,-0.433825672914779,-0.900996828806872));
#43098=DIRECTION('center_axis',(1.,0.,0.));
#43099=DIRECTION('ref_axis',(0.,-0.342020143325669,-0.939692620785908));
#43100=DIRECTION('center_axis',(1.,0.,0.));
#43101=DIRECTION('ref_axis',(0.,-0.4226182617407,-0.90630778703665));
#43102=DIRECTION('center_axis',(1.,0.,0.));
#43103=DIRECTION('ref_axis',(0.,-0.4226182617407,-0.90630778703665));
#43104=DIRECTION('center_axis',(0.,-0.811975624921639,0.583691343548209));
#43105=DIRECTION('ref_axis',(0.,-0.583691343548209,-0.81197562492164));
#43106=DIRECTION('center_axis',(1.,0.,0.));
#43107=DIRECTION('ref_axis',(0.,-0.5,-0.866025403784438));
#43108=DIRECTION('center_axis',(1.,0.,0.));
#43109=DIRECTION('ref_axis',(0.,-0.573576436351046,-0.819152044288992));
#43110=DIRECTION('center_axis',(0.,-0.758013759944346,0.652238560447813));
#43111=DIRECTION('ref_axis',(0.,-0.652238560447812,-0.758013759944346));
#43112=DIRECTION('center_axis',(0.,-0.698282952552655,0.715821848069998));
#43113=DIRECTION('ref_axis',(0.,-0.715821848069998,-0.698282952552655));
#43114=DIRECTION('center_axis',(1.,0.,0.));
#43115=DIRECTION('ref_axis',(0.,-0.64278760968654,-0.766044443118978));
#43116=DIRECTION('center_axis',(0.,-0.633237790257263,0.773957299203321));
#43117=DIRECTION('ref_axis',(0.,-0.773957299203321,-0.633237790257263));
#43118=DIRECTION('center_axis',(1.,0.,0.));
#43119=DIRECTION('ref_axis',(0.,-0.707106781186548,-0.707106781186547));
#43120=DIRECTION('center_axis',(1.,0.,0.));
#43121=DIRECTION('ref_axis',(0.,-0.766044443118978,-0.642787609686539));
#43122=DIRECTION('center_axis',(1.,0.,0.));
#43123=DIRECTION('ref_axis',(0.,-0.766044443118978,-0.642787609686539));
#43124=DIRECTION('center_axis',(0.,-0.489221210746995,0.872159737063827));
#43125=DIRECTION('ref_axis',(0.,-0.872159737063827,-0.489221210746995));
#43126=DIRECTION('center_axis',(1.,0.,0.));
#43127=DIRECTION('ref_axis',(0.,-0.819152044288992,-0.573576436351046));
#43128=DIRECTION('center_axis',(1.,0.,0.));
#43129=DIRECTION('ref_axis',(0.,-0.866025403784439,-0.5));
#43130=DIRECTION('center_axis',(0.,-0.411345846661781,0.911479343942639));
#43131=DIRECTION('ref_axis',(0.,-0.911479343942638,-0.411345846661781));
#43132=DIRECTION('center_axis',(0.,-0.330339892306057,0.943862042647771));
#43133=DIRECTION('ref_axis',(0.,-0.943862042647771,-0.330339892306057));
#43134=DIRECTION('center_axis',(1.,0.,0.));
#43135=DIRECTION('ref_axis',(0.,-0.90630778703665,-0.422618261740699));
#43136=DIRECTION('center_axis',(0.,-0.246819851905204,0.96906138128887));
#43137=DIRECTION('ref_axis',(0.,-0.96906138128887,-0.246819851905204));
#43138=DIRECTION('center_axis',(1.,0.,0.));
#43139=DIRECTION('ref_axis',(0.,-0.939692620785909,-0.342020143325668));
#43140=DIRECTION('center_axis',(1.,0.,0.));
#43141=DIRECTION('ref_axis',(0.,-0.965925826289068,-0.25881904510252));
#43142=DIRECTION('center_axis',(1.,0.,0.));
#43143=DIRECTION('ref_axis',(0.,-0.965925826289068,-0.25881904510252));
#43144=DIRECTION('center_axis',(0.,-0.0747943608453591,0.997198978933359));
#43145=DIRECTION('ref_axis',(0.,-0.997198978933359,-0.0747943608453591));
#43146=DIRECTION('center_axis',(1.,0.,0.));
#43147=DIRECTION('ref_axis',(0.,-0.984807753012208,-0.17364817766693));
#43148=DIRECTION('center_axis',(1.,0.,0.));
#43149=DIRECTION('ref_axis',(0.,-0.996194698091746,-0.0871557427476579));
#43150=DIRECTION('center_axis',(0.,0.0124018719548356,0.999923093828728));
#43151=DIRECTION('ref_axis',(0.,-0.999923093828728,0.0124018719548356));
#43152=DIRECTION('center_axis',(0.,0.099503719020999,0.995037190209989));
#43153=DIRECTION('ref_axis',(0.,-0.995037190209989,0.099503719020999));
#43154=DIRECTION('center_axis',(1.,0.,0.));
#43155=DIRECTION('ref_axis',(0.,-1.,1.83697019872103E-16));
#43156=DIRECTION('center_axis',(0.,0.185848282703424,0.98257845275387));
#43157=DIRECTION('ref_axis',(0.,-0.982578452753869,0.185848282703424));
#43158=DIRECTION('center_axis',(1.,0.,0.));
#43159=DIRECTION('ref_axis',(0.,-0.996194698091746,0.0871557427476582));
#43160=DIRECTION('center_axis',(1.,0.,0.));
#43161=DIRECTION('ref_axis',(0.,-0.984807753012208,0.17364817766693));
#43162=DIRECTION('center_axis',(1.,0.,0.));
#43163=DIRECTION('ref_axis',(0.,-0.984807753012208,0.17364817766693));
#43164=DIRECTION('center_axis',(0.,0.353647787425838,0.935378662600772));
#43165=DIRECTION('ref_axis',(0.,-0.935378662600772,0.353647787425838));
#43166=DIRECTION('center_axis',(1.,0.,0.));
#43167=DIRECTION('ref_axis',(0.,-0.965925826289068,0.258819045102521));
#43168=DIRECTION('center_axis',(1.,0.,0.));
#43169=DIRECTION('ref_axis',(0.,-0.939692620785908,0.342020143325669));
#43170=DIRECTION('center_axis',(0.,0.433825672914779,0.900996828806872));
#43171=DIRECTION('ref_axis',(0.,-0.900996828806872,0.433825672914779));
#43172=DIRECTION('center_axis',(0.,0.510701883081734,0.859757865108992));
#43173=DIRECTION('ref_axis',(0.,-0.859757865108992,0.510701883081734));
#43174=DIRECTION('center_axis',(1.,0.,0.));
#43175=DIRECTION('ref_axis',(0.,-0.90630778703665,0.4226182617407));
#43176=DIRECTION('center_axis',(0.,0.583691343548209,0.811975624921639));
#43177=DIRECTION('ref_axis',(0.,-0.81197562492164,0.583691343548209));
#43178=DIRECTION('center_axis',(1.,0.,0.));
#43179=DIRECTION('ref_axis',(0.,-0.866025403784438,0.5));
#43180=DIRECTION('center_axis',(1.,0.,0.));
#43181=DIRECTION('ref_axis',(0.,-0.819152044288992,0.573576436351046));
#43182=DIRECTION('center_axis',(1.,0.,0.));
#43183=DIRECTION('ref_axis',(0.,-0.819152044288992,0.573576436351046));
#43184=DIRECTION('center_axis',(0.,0.715821848069998,0.698282952552655));
#43185=DIRECTION('ref_axis',(0.,-0.698282952552655,0.715821848069998));
#43186=DIRECTION('center_axis',(1.,0.,0.));
#43187=DIRECTION('ref_axis',(0.,-0.766044443118978,0.642787609686539));
#43188=DIRECTION('center_axis',(1.,0.,0.));
#43189=DIRECTION('ref_axis',(0.,-0.707106781186547,0.707106781186548));
#43190=DIRECTION('center_axis',(0.,0.773957299203321,0.633237790257263));
#43191=DIRECTION('ref_axis',(0.,-0.633237790257263,0.773957299203321));
#43192=DIRECTION('center_axis',(0.,0.826202467961513,0.563373306018581));
#43193=DIRECTION('ref_axis',(0.,-0.563373306018581,0.826202467961513));
#43194=DIRECTION('center_axis',(1.,0.,0.));
#43195=DIRECTION('ref_axis',(0.,-0.642787609686539,0.766044443118978));
#43196=DIRECTION('center_axis',(0.,0.872159737063828,0.489221210746995));
#43197=DIRECTION('ref_axis',(0.,-0.489221210746995,0.872159737063827));
#43198=DIRECTION('center_axis',(1.,0.,0.));
#43199=DIRECTION('ref_axis',(0.,-0.573576436351046,0.819152044288992));
#43200=DIRECTION('center_axis',(1.,0.,0.));
#43201=DIRECTION('ref_axis',(0.,-0.5,0.866025403784439));
#43202=DIRECTION('center_axis',(1.,0.,0.));
#43203=DIRECTION('ref_axis',(0.,-0.5,0.866025403784439));
#43204=DIRECTION('center_axis',(0.,0.943862042647771,0.330339892306057));
#43205=DIRECTION('ref_axis',(0.,-0.330339892306057,0.943862042647771));
#43206=DIRECTION('center_axis',(1.,0.,0.));
#43207=DIRECTION('ref_axis',(0.,-0.422618261740699,0.90630778703665));
#43208=DIRECTION('center_axis',(1.,0.,0.));
#43209=DIRECTION('ref_axis',(0.,-0.342020143325669,0.939692620785909));
#43210=DIRECTION('center_axis',(0.,0.96906138128887,0.246819851905204));
#43211=DIRECTION('ref_axis',(0.,-0.246819851905204,0.96906138128887));
#43212=DIRECTION('center_axis',(0.,0.986885577683101,0.161421363397451));
#43213=DIRECTION('ref_axis',(0.,-0.161421363397451,0.986885577683101));
#43214=DIRECTION('center_axis',(1.,0.,0.));
#43215=DIRECTION('ref_axis',(0.,-0.258819045102521,0.965925826289068));
#43216=DIRECTION('center_axis',(0.,0.997198978933359,0.0747943608453591));
#43217=DIRECTION('ref_axis',(0.,-0.0747943608453591,0.997198978933359));
#43218=DIRECTION('center_axis',(1.,0.,0.));
#43219=DIRECTION('ref_axis',(0.,-0.17364817766693,0.984807753012208));
#43220=DIRECTION('center_axis',(1.,0.,0.));
#43221=DIRECTION('ref_axis',(0.,-0.0871557427476579,0.996194698091746));
#43222=DIRECTION('center_axis',(1.,0.,0.));
#43223=DIRECTION('ref_axis',(0.,-0.0871557427476579,0.996194698091746));
#43224=DIRECTION('center_axis',(0.,0.995037190209989,-0.0995037190209989));
#43225=DIRECTION('ref_axis',(0.,0.0995037190209989,0.995037190209989));
#43226=DIRECTION('center_axis',(1.,0.,0.));
#43227=DIRECTION('ref_axis',(0.,1.22464679914735E-16,1.));
#43228=DIRECTION('center_axis',(1.,0.,0.));
#43229=DIRECTION('ref_axis',(0.,0.0871557427476582,0.996194698091746));
#43230=DIRECTION('center_axis',(0.,0.98257845275387,-0.185848282703424));
#43231=DIRECTION('ref_axis',(0.,0.185848282703424,0.982578452753869));
#43232=DIRECTION('center_axis',(0.,0.962641699975202,-0.270778428736216));
#43233=DIRECTION('ref_axis',(0.,0.270778428736216,0.962641699975202));
#43234=DIRECTION('center_axis',(1.,0.,0.));
#43235=DIRECTION('ref_axis',(0.,0.173648177666931,0.984807753012208));
#43236=DIRECTION('center_axis',(0.,0.935378662600772,-0.353647787425838));
#43237=DIRECTION('ref_axis',(0.,0.353647787425838,0.935378662600772));
#43238=DIRECTION('center_axis',(1.,0.,0.));
#43239=DIRECTION('ref_axis',(0.,0.258819045102521,0.965925826289068));
#43240=DIRECTION('center_axis',(1.,0.,0.));
#43241=DIRECTION('ref_axis',(0.,0.342020143325669,0.939692620785908));
#43242=DIRECTION('center_axis',(1.,0.,0.));
#43243=DIRECTION('ref_axis',(0.,0.342020143325669,0.939692620785908));
#43244=DIRECTION('center_axis',(0.,0.859757865108992,-0.510701883081733));
#43245=DIRECTION('ref_axis',(0.,0.510701883081733,0.859757865108992));
#43246=DIRECTION('center_axis',(1.,0.,0.));
#43247=DIRECTION('ref_axis',(0.,0.422618261740699,0.90630778703665));
#43248=DIRECTION('center_axis',(1.,0.,0.));
#43249=DIRECTION('ref_axis',(0.,0.5,0.866025403784439));
#43250=DIRECTION('center_axis',(0.,0.81197562492164,-0.583691343548208));
#43251=DIRECTION('ref_axis',(0.,0.583691343548208,0.81197562492164));
#43252=DIRECTION('center_axis',(0.,0.758013759944346,-0.652238560447812));
#43253=DIRECTION('ref_axis',(0.,0.652238560447812,0.758013759944346));
#43254=DIRECTION('center_axis',(1.,0.,0.));
#43255=DIRECTION('ref_axis',(0.,0.573576436351046,0.819152044288992));
#43256=DIRECTION('center_axis',(0.,0.698282952552655,-0.715821848069998));
#43257=DIRECTION('ref_axis',(0.,0.715821848069998,0.698282952552655));
#43258=DIRECTION('center_axis',(1.,0.,0.));
#43259=DIRECTION('ref_axis',(0.,0.642787609686539,0.766044443118978));
#43260=DIRECTION('center_axis',(1.,0.,0.));
#43261=DIRECTION('ref_axis',(0.,0.707106781186548,0.707106781186547));
#43262=DIRECTION('center_axis',(1.,0.,0.));
#43263=DIRECTION('ref_axis',(0.,0.707106781186548,0.707106781186547));
#43264=DIRECTION('center_axis',(0.,0.563373306018581,-0.826202467961513));
#43265=DIRECTION('ref_axis',(0.,0.826202467961513,0.563373306018581));
#43266=DIRECTION('center_axis',(1.,0.,0.));
#43267=DIRECTION('ref_axis',(0.,0.766044443118978,0.642787609686539));
#43268=DIRECTION('center_axis',(1.,0.,0.));
#43269=DIRECTION('ref_axis',(0.,0.819152044288992,0.573576436351046));
#43270=DIRECTION('center_axis',(0.,0.489221210746995,-0.872159737063828));
#43271=DIRECTION('ref_axis',(0.,0.872159737063827,0.489221210746995));
#43272=DIRECTION('center_axis',(0.,0.411345846661781,-0.911479343942639));
#43273=DIRECTION('ref_axis',(0.,0.911479343942639,0.411345846661781));
#43274=DIRECTION('center_axis',(1.,0.,0.));
#43275=DIRECTION('ref_axis',(0.,0.866025403784439,0.5));
#43276=DIRECTION('center_axis',(0.,0.330339892306057,-0.943862042647771));
#43277=DIRECTION('ref_axis',(0.,0.943862042647771,0.330339892306057));
#43278=DIRECTION('center_axis',(1.,0.,0.));
#43279=DIRECTION('ref_axis',(0.,0.90630778703665,0.422618261740699));
#43280=DIRECTION('center_axis',(1.,0.,0.));
#43281=DIRECTION('ref_axis',(0.,0.939692620785908,0.342020143325669));
#43282=DIRECTION('center_axis',(1.,0.,0.));
#43283=DIRECTION('ref_axis',(0.,0.939692620785908,0.342020143325669));
#43284=DIRECTION('center_axis',(0.,0.161421363397451,-0.986885577683101));
#43285=DIRECTION('ref_axis',(0.,0.986885577683101,0.161421363397451));
#43286=DIRECTION('center_axis',(1.,0.,0.));
#43287=DIRECTION('ref_axis',(0.,0.965925826289068,0.258819045102521));
#43288=DIRECTION('center_axis',(1.,0.,0.));
#43289=DIRECTION('ref_axis',(0.,0.984807753012208,0.17364817766693));
#43290=DIRECTION('center_axis',(0.,0.0747943608453594,-0.997198978933359));
#43291=DIRECTION('ref_axis',(0.,0.997198978933359,0.0747943608453594));
#43292=DIRECTION('center_axis',(0.,-0.0124018719548355,-0.999923093828728));
#43293=DIRECTION('ref_axis',(0.,0.999923093828728,-0.0124018719548355));
#43294=DIRECTION('center_axis',(1.,0.,0.));
#43295=DIRECTION('ref_axis',(0.,0.996194698091746,0.087155742747658));
#43296=DIRECTION('center_axis',(0.,-0.0995037190209988,-0.995037190209989));
#43297=DIRECTION('ref_axis',(0.,0.995037190209989,-0.0995037190209988));
#43298=DIRECTION('center_axis',(1.,0.,0.));
#43299=DIRECTION('ref_axis',(0.,1.,-6.12323399573677E-17));
#43300=DIRECTION('center_axis',(1.,0.,0.));
#43301=DIRECTION('ref_axis',(0.,0.996194698091746,-0.0871557427476584));
#43302=DIRECTION('center_axis',(1.,0.,0.));
#43303=DIRECTION('ref_axis',(0.,0.996194698091746,-0.0871557427476584));
#43304=DIRECTION('center_axis',(0.,-0.270778428736215,-0.962641699975202));
#43305=DIRECTION('ref_axis',(0.,0.962641699975202,-0.270778428736215));
#43306=DIRECTION('center_axis',(1.,0.,0.));
#43307=DIRECTION('ref_axis',(0.,0.984807753012208,-0.17364817766693));
#43308=DIRECTION('center_axis',(1.,0.,0.));
#43309=DIRECTION('ref_axis',(0.,0.965925826289068,-0.258819045102521));
#43310=DIRECTION('center_axis',(0.,-0.353647787425838,-0.935378662600772));
#43311=DIRECTION('ref_axis',(0.,0.935378662600772,-0.353647787425838));
#43312=DIRECTION('center_axis',(0.,-0.433825672914778,-0.900996828806872));
#43313=DIRECTION('ref_axis',(0.,0.900996828806872,-0.433825672914778));
#43314=DIRECTION('center_axis',(1.,0.,0.));
#43315=DIRECTION('ref_axis',(0.,0.939692620785908,-0.342020143325669));
#43316=DIRECTION('center_axis',(0.,-0.510701883081733,-0.859757865108992));
#43317=DIRECTION('ref_axis',(0.,0.859757865108992,-0.510701883081733));
#43318=DIRECTION('center_axis',(1.,0.,0.));
#43319=DIRECTION('ref_axis',(0.,0.90630778703665,-0.422618261740699));
#43320=DIRECTION('center_axis',(1.,0.,0.));
#43321=DIRECTION('ref_axis',(0.,0.866025403784439,-0.5));
#43322=DIRECTION('center_axis',(1.,0.,0.));
#43323=DIRECTION('ref_axis',(0.,0.866025403784439,-0.5));
#43324=DIRECTION('center_axis',(0.,-0.652238560447812,-0.758013759944347));
#43325=DIRECTION('ref_axis',(0.,0.758013759944347,-0.652238560447812));
#43326=DIRECTION('center_axis',(1.,0.,0.));
#43327=DIRECTION('ref_axis',(0.,0.819152044288992,-0.573576436351046));
#43328=DIRECTION('center_axis',(1.,0.,0.));
#43329=DIRECTION('ref_axis',(0.,0.766044443118978,-0.642787609686539));
#43330=DIRECTION('center_axis',(0.,-0.715821848069998,-0.698282952552655));
#43331=DIRECTION('ref_axis',(0.,0.698282952552655,-0.715821848069998));
#43332=DIRECTION('center_axis',(0.,-0.773957299203321,-0.633237790257263));
#43333=DIRECTION('ref_axis',(0.,0.633237790257263,-0.773957299203321));
#43334=DIRECTION('center_axis',(1.,0.,0.));
#43335=DIRECTION('ref_axis',(0.,0.707106781186548,-0.707106781186548));
#43336=DIRECTION('center_axis',(0.,-0.826202467961513,-0.563373306018581));
#43337=DIRECTION('ref_axis',(0.,0.563373306018581,-0.826202467961513));
#43338=DIRECTION('center_axis',(1.,0.,0.));
#43339=DIRECTION('ref_axis',(0.,0.642787609686539,-0.766044443118978));
#43340=DIRECTION('center_axis',(1.,0.,0.));
#43341=DIRECTION('ref_axis',(0.,0.573576436351046,-0.819152044288992));
#43342=DIRECTION('center_axis',(1.,0.,0.));
#43343=DIRECTION('ref_axis',(0.,0.573576436351046,-0.819152044288992));
#43344=DIRECTION('center_axis',(0.,-0.911479343942639,-0.411345846661781));
#43345=DIRECTION('ref_axis',(0.,0.411345846661781,-0.911479343942639));
#43346=DIRECTION('center_axis',(1.,0.,0.));
#43347=DIRECTION('ref_axis',(0.,0.5,-0.866025403784439));
#43348=DIRECTION('center_axis',(1.,0.,0.));
#43349=DIRECTION('ref_axis',(0.,0.422618261740699,-0.90630778703665));
#43350=DIRECTION('center_axis',(0.,-0.943862042647771,-0.330339892306057));
#43351=DIRECTION('ref_axis',(0.,0.330339892306057,-0.943862042647771));
#43352=DIRECTION('center_axis',(0.,-0.96906138128887,-0.246819851905204));
#43353=DIRECTION('ref_axis',(0.,0.246819851905204,-0.96906138128887));
#43354=DIRECTION('center_axis',(1.,0.,0.));
#43355=DIRECTION('ref_axis',(0.,0.342020143325669,-0.939692620785908));
#43356=DIRECTION('center_axis',(0.,-0.986885577683101,-0.161421363397451));
#43357=DIRECTION('ref_axis',(0.,0.161421363397451,-0.986885577683101));
#43358=DIRECTION('center_axis',(1.,0.,0.));
#43359=DIRECTION('ref_axis',(0.,0.258819045102521,-0.965925826289068));
#43360=DIRECTION('center_axis',(1.,0.,0.));
#43361=DIRECTION('ref_axis',(0.,0.17364817766693,-0.984807753012208));
#43362=DIRECTION('center_axis',(1.,0.,0.));
#43363=DIRECTION('ref_axis',(0.,0.17364817766693,-0.984807753012208));
#43364=DIRECTION('center_axis',(0.,-0.999923093828728,0.0124018719548353));
#43365=DIRECTION('ref_axis',(0.,-0.0124018719548353,-0.999923093828728));
#43366=DIRECTION('center_axis',(1.,0.,0.));
#43367=DIRECTION('ref_axis',(0.,0.0871557427476582,-0.996194698091746));
#43368=DIRECTION('center_axis',(1.,0.,0.));
#43369=DIRECTION('ref_axis',(0.,0.,-1.));
#43370=DIRECTION('center_axis',(0.,-0.995037190209989,0.0995037190209988));
#43371=DIRECTION('ref_axis',(0.,-0.0995037190209988,-0.995037190209989));
#43372=DIRECTION('center_axis',(-1.,0.,0.));
#43373=DIRECTION('ref_axis',(0.,0.,-1.));
#43374=DIRECTION('',(-1.,0.,0.));
#43375=DIRECTION('center_axis',(1.,0.,0.));
#43376=DIRECTION('ref_axis',(0.,0.,-1.));
#43377=DIRECTION('center_axis',(-1.,0.,0.));
#43378=DIRECTION('ref_axis',(0.,0.,-1.));
#43379=DIRECTION('',(-1.,0.,0.));
#43380=DIRECTION('center_axis',(1.,0.,0.));
#43381=DIRECTION('ref_axis',(0.,0.,-1.));
#43382=DIRECTION('center_axis',(-1.,0.,0.));
#43383=DIRECTION('ref_axis',(0.,0.,-1.));
#43384=DIRECTION('',(-1.,0.,0.));
#43385=DIRECTION('center_axis',(1.,0.,0.));
#43386=DIRECTION('ref_axis',(0.,0.,-1.));
#43387=DIRECTION('center_axis',(-1.,0.,0.));
#43388=DIRECTION('ref_axis',(0.,0.,-1.));
#43389=DIRECTION('',(-1.,0.,0.));
#43390=DIRECTION('center_axis',(1.,0.,0.));
#43391=DIRECTION('ref_axis',(0.,0.,-1.));
#43392=DIRECTION('center_axis',(-1.,0.,0.));
#43393=DIRECTION('ref_axis',(0.,0.,-1.));
#43394=DIRECTION('',(-1.,0.,0.));
#43395=DIRECTION('center_axis',(1.,0.,0.));
#43396=DIRECTION('ref_axis',(0.,0.,-1.));
#43397=DIRECTION('center_axis',(-1.,0.,0.));
#43398=DIRECTION('ref_axis',(0.,1.,0.));
#43399=DIRECTION('center_axis',(1.,0.,0.));
#43400=DIRECTION('ref_axis',(0.,0.,-1.));
#43401=DIRECTION('',(0.447213595499958,0.894427190999916,1.09535739652841E-16));
#43402=DIRECTION('center_axis',(1.,0.,0.));
#43403=DIRECTION('ref_axis',(0.,0.,-1.));
#43404=DIRECTION('center_axis',(1.,0.,0.));
#43405=DIRECTION('ref_axis',(0.,1.,0.));
#43406=DIRECTION('',(1.,0.,0.));
#43407=DIRECTION('center_axis',(-1.,0.,0.));
#43408=DIRECTION('ref_axis',(0.,1.,0.));
#43409=DIRECTION('center_axis',(1.,0.,0.));
#43410=DIRECTION('ref_axis',(0.,-0.951056516295154,0.309016994374948));
#43411=DIRECTION('',(1.,0.,0.));
#43412=DIRECTION('center_axis',(-1.,0.,0.));
#43413=DIRECTION('ref_axis',(0.,0.,-1.));
#43414=DIRECTION('center_axis',(1.,0.,0.));
#43415=DIRECTION('ref_axis',(0.,0.,-1.));
#43416=DIRECTION('',(1.,0.,0.));
#43417=DIRECTION('center_axis',(-1.,0.,0.));
#43418=DIRECTION('ref_axis',(0.,0.,-1.));
#43419=DIRECTION('center_axis',(1.,0.,0.));
#43420=DIRECTION('ref_axis',(0.,5.66553889764798E-16,1.));
#43421=DIRECTION('',(1.,0.,0.));
#43422=DIRECTION('center_axis',(-1.,0.,0.));
#43423=DIRECTION('ref_axis',(0.,0.,-1.));
#43424=DIRECTION('center_axis',(1.,0.,0.));
#43425=DIRECTION('ref_axis',(0.,0.,-1.));
#43426=DIRECTION('center_axis',(-1.,0.,0.));
#43427=DIRECTION('ref_axis',(0.,0.,-1.));
#43428=DIRECTION('center_axis',(1.,0.,0.));
#43429=DIRECTION('ref_axis',(0.,0.,-1.));
#43430=DIRECTION('center_axis',(1.,0.,0.));
#43431=DIRECTION('ref_axis',(0.,1.,0.));
#43432=DIRECTION('',(-1.,0.,0.));
#43433=DIRECTION('center_axis',(1.,0.,0.));
#43434=DIRECTION('ref_axis',(0.,0.,-1.));
#43435=DIRECTION('center_axis',(1.,0.,0.));
#43436=DIRECTION('ref_axis',(0.,0.,-1.));
#43437=DIRECTION('center_axis',(1.,0.,0.));
#43438=DIRECTION('ref_axis',(0.,1.,0.));
#43439=DIRECTION('',(-1.,0.,0.));
#43440=DIRECTION('center_axis',(1.,0.,0.));
#43441=DIRECTION('ref_axis',(0.,0.,-1.));
#43442=DIRECTION('center_axis',(1.,0.,0.));
#43443=DIRECTION('ref_axis',(0.,0.,-1.));
#43444=DIRECTION('center_axis',(1.,0.,0.));
#43445=DIRECTION('ref_axis',(0.,1.,0.));
#43446=DIRECTION('',(-1.,0.,0.));
#43447=DIRECTION('center_axis',(1.,0.,0.));
#43448=DIRECTION('ref_axis',(0.,0.,-1.));
#43449=DIRECTION('center_axis',(-1.,0.,0.));
#43450=DIRECTION('ref_axis',(0.,0.,1.));
#43451=DIRECTION('center_axis',(1.,0.,0.));
#43452=DIRECTION('ref_axis',(0.,0.,-1.));
#43453=DIRECTION('center_axis',(1.,0.,0.));
#43454=DIRECTION('ref_axis',(0.,1.,0.));
#43455=DIRECTION('',(-1.,0.,0.));
#43456=DIRECTION('center_axis',(1.,0.,0.));
#43457=DIRECTION('ref_axis',(0.,0.,-1.));
#43458=DIRECTION('center_axis',(-1.,0.,0.));
#43459=DIRECTION('ref_axis',(0.,1.,0.));
#43460=DIRECTION('',(-0.707106781186547,-0.707106781186548,-8.65956056235494E-17));
#43461=DIRECTION('center_axis',(1.,0.,0.));
#43462=DIRECTION('ref_axis',(0.,1.,0.));
#43463=DIRECTION('center_axis',(1.,0.,0.));
#43464=DIRECTION('ref_axis',(0.,0.,-1.));
#43465=DIRECTION('',(-0.707106781186548,0.707106781186547,8.65956056235493E-17));
#43466=DIRECTION('center_axis',(-1.,0.,0.));
#43467=DIRECTION('ref_axis',(0.,0.,1.));
#43468=DIRECTION('center_axis',(1.,0.,0.));
#43469=DIRECTION('ref_axis',(0.,0.,-1.));
#43470=DIRECTION('center_axis',(-1.,0.,0.));
#43471=DIRECTION('ref_axis',(0.,1.,0.));
#43472=DIRECTION('',(-0.496138938356835,-0.868243142124459,-1.06329118488436E-16));
#43473=DIRECTION('center_axis',(1.,0.,0.));
#43474=DIRECTION('ref_axis',(0.,0.,-1.));
#43475=DIRECTION('center_axis',(-1.,0.,0.));
#43476=DIRECTION('ref_axis',(0.,1.,0.));
#43477=DIRECTION('',(-0.447213595499971,-0.89442719099991,-1.0953573965284E-16));
#47304=CARTESIAN_POINT('',(0.,0.,0.));
#47305=CARTESIAN_POINT('Origin',(6.63819660112501,0.,-1.21095483169075E-15));
#47306=CARTESIAN_POINT('',(7.,40.,-4.89858719658941E-15));
#47307=CARTESIAN_POINT('',(7.,-40.,-4.89858719658941E-15));
#47308=CARTESIAN_POINT('Origin',(7.,0.,0.));
#47309=CARTESIAN_POINT('Origin',(7.,0.,0.));
#47310=CARTESIAN_POINT('',(6.27639320225002,39.5527864045,4.84381932676299E-15));
#47311=CARTESIAN_POINT('',(6.63819660112501,39.77639320225,4.8712032616762E-15));
#47312=CARTESIAN_POINT('',(6.27639320225002,-39.5527864045,-4.84381932676299E-15));
#47313=CARTESIAN_POINT('Origin',(6.27639320225002,0.,-2.4219096633815E-15));
#47314=CARTESIAN_POINT('Origin',(6.27639320225002,0.,-2.4219096633815E-15));
#47315=CARTESIAN_POINT('Origin',(5.75,0.,0.));
#47316=CARTESIAN_POINT('',(5.22360679774998,-37.4472135955,-4.58596102667163E-15));
#47317=CARTESIAN_POINT('',(5.75,-38.5,-4.71489017671731E-15));
#47318=CARTESIAN_POINT('',(5.22360679774998,37.4472135955,-4.58596102667163E-15));
#47319=CARTESIAN_POINT('Origin',(5.22360679774998,0.,-2.29298051333581E-15));
#47320=CARTESIAN_POINT('Origin',(5.22360679774998,0.,-2.29298051333581E-15));
#47321=CARTESIAN_POINT('Origin',(31.25,0.,0.));
#47322=CARTESIAN_POINT('',(56.,-40.,-4.89858719658941E-15));
#47323=CARTESIAN_POINT('Origin',(56.,0.,0.));
#47324=CARTESIAN_POINT('',(31.25,-40.,-4.89858719658941E-15));
#47325=CARTESIAN_POINT('Origin',(5.11180339887499,0.,-1.14649025666791E-15));
#47326=CARTESIAN_POINT('',(5.,36.5,4.46996081688784E-15));
#47327=CARTESIAN_POINT('',(5.11180339887499,36.97360679775,4.52796092177973E-15));
#47328=CARTESIAN_POINT('Origin',(5.,0.,0.));
#47329=CARTESIAN_POINT('Origin',(5.,37.,0.));
#47330=CARTESIAN_POINT('',(5.,-33.2,-4.06582737316921E-15));
#47331=CARTESIAN_POINT('Origin',(5.,0.,0.));
#47332=CARTESIAN_POINT('Origin',(32.19,0.,0.));
#47333=CARTESIAN_POINT('',(31.94,26.5,-3.24531401774049E-15));
#47334=CARTESIAN_POINT('Origin',(31.94,0.,0.));
#47335=CARTESIAN_POINT('',(32.44,26.,3.18408167778312E-15));
#47336=CARTESIAN_POINT('',(32.19,26.25,-3.2146978477618E-15));
#47337=CARTESIAN_POINT('',(32.44,-26.,-3.18408167778312E-15));
#47338=CARTESIAN_POINT('Origin',(32.44,0.,0.));
#47339=CARTESIAN_POINT('Origin',(32.44,0.,0.));
#47340=CARTESIAN_POINT('Origin',(32.97,0.,0.));
#47341=CARTESIAN_POINT('',(34.,-26.,-3.18408167778312E-15));
#47342=CARTESIAN_POINT('Origin',(34.,0.,0.));
#47343=CARTESIAN_POINT('',(32.97,-26.,-3.18408167778312E-15));
#47344=CARTESIAN_POINT('Origin',(31.94,29.58,0.));
#47345=CARTESIAN_POINT('',(31.94,-29.58,-3.62250523187787E-15));
#47346=CARTESIAN_POINT('Origin',(31.94,0.,0.));
#47347=CARTESIAN_POINT('Origin',(104.823223304703,0.,-9.90541890020826E-16));
#47348=CARTESIAN_POINT('',(105.,31.5,-3.85763741731416E-15));
#47349=CARTESIAN_POINT('Origin',(105.,0.,0.));
#47350=CARTESIAN_POINT('',(104.646446609407,32.3535533905933,3.96216756008331E-15));
#47351=CARTESIAN_POINT('',(104.823223304703,31.9267766952966,3.90990248869873E-15));
#47352=CARTESIAN_POINT('',(104.646446609407,-32.3535533905933,-3.96216756008331E-15));
#47353=CARTESIAN_POINT('Origin',(104.646446609407,0.,-1.98108378004165E-15));
#47354=CARTESIAN_POINT('Origin',(104.646446609407,0.,-1.98108378004165E-15));
#47355=CARTESIAN_POINT('Origin',(104.,0.,0.));
#47356=CARTESIAN_POINT('',(103.353553390593,-33.6464466094067,-4.12050131428923E-15));
#47357=CARTESIAN_POINT('',(104.,-33.,-4.04133443718627E-15));
#47358=CARTESIAN_POINT('',(103.353553390593,33.6464466094067,-4.12050131428923E-15));
#47359=CARTESIAN_POINT('Origin',(103.353553390593,0.,-2.06025065714461E-15));
#47360=CARTESIAN_POINT('Origin',(103.353553390593,0.,-2.06025065714461E-15));
#47361=CARTESIAN_POINT('Origin',(105.,25.16,0.));
#47362=CARTESIAN_POINT('',(105.,-25.16,-3.08121134665474E-15));
#47363=CARTESIAN_POINT('Origin',(105.,0.,0.));
#47364=CARTESIAN_POINT('Origin',(102.928240579529,0.,-2.07272928697064E-15));
#47365=CARTESIAN_POINT('',(102.502927768465,34.0540295903842,4.17041583359333E-15));
#47366=CARTESIAN_POINT('',(102.928240579529,33.8502380998955,4.14545857394128E-15));
#47367=CARTESIAN_POINT('',(102.502927768465,-34.0540295903842,-4.17041583359333E-15));
#47368=CARTESIAN_POINT('Origin',(102.502927768465,0.,-2.08520791679666E-15));
#47369=CARTESIAN_POINT('Origin',(102.502927768465,0.,-2.08520791679666E-15));
#47370=CARTESIAN_POINT('Origin',(91.5,0.,0.));
#47371=CARTESIAN_POINT('',(80.,-36.5,-4.46996081688784E-15));
#47372=CARTESIAN_POINT('',(91.5,-35.25,-4.31687996699442E-15));
#47373=CARTESIAN_POINT('Origin',(80.,0.,0.));
#47374=CARTESIAN_POINT('Origin',(70.90242469777,0.,-7.77414446918783E-15));
#47375=CARTESIAN_POINT('',(71.0821994936527,126.506803038084,-1.54926151410954E-14));
#47376=CARTESIAN_POINT('',(71.0821994936527,-126.506803038084,-1.54926151410954E-14));
#47377=CARTESIAN_POINT('Origin',(71.0821994936527,0.,-7.74630757054771E-15));
#47378=CARTESIAN_POINT('Origin',(71.0821994936527,0.,-7.74630757054771E-15));
#47379=CARTESIAN_POINT('',(70.7226499018874,127.416025147169,1.56039627356559E-14));
#47380=CARTESIAN_POINT('',(70.90242469777,126.961414092626,1.55482889383757E-14));
#47381=CARTESIAN_POINT('',(70.7226499018874,-127.416025147169,-1.56039627356559E-14));
#47382=CARTESIAN_POINT('Origin',(70.7226499018874,0.,-7.80198136782795E-15));
#47383=CARTESIAN_POINT('Origin',(70.7226499018874,0.,-7.80198136782795E-15));
#47384=CARTESIAN_POINT('Origin',(69.5,0.,0.));
#47385=CARTESIAN_POINT('',(68.2773500981126,-131.083974852831,-1.60531570223032E-14));
#47386=CARTESIAN_POINT('',(69.5,-129.25,-1.58285598789795E-14));
#47387=CARTESIAN_POINT('',(68.2773500981126,131.083974852831,-1.60531570223032E-14));
#47388=CARTESIAN_POINT('Origin',(68.2773500981126,0.,-8.02657851115159E-15));
#47389=CARTESIAN_POINT('Origin',(68.2773500981126,0.,-8.02657851115159E-15));
#47390=CARTESIAN_POINT('Origin',(71.5,0.,0.));
#47391=CARTESIAN_POINT('',(72.,-121.,-1.4818226269683E-14));
#47392=CARTESIAN_POINT('Origin',(72.,0.,0.));
#47393=CARTESIAN_POINT('',(71.5,-124.,-1.51856203094272E-14));
#47394=CARTESIAN_POINT('Origin',(67.9386750490563,0.,-8.04850045876632E-15));
#47395=CARTESIAN_POINT('',(67.6,131.8,1.61408448127621E-14));
#47396=CARTESIAN_POINT('',(67.9386750490563,131.441987426416,1.60970009175327E-14));
#47397=CARTESIAN_POINT('',(67.6,-131.8,-1.61408448127621E-14));
#47398=CARTESIAN_POINT('Origin',(67.6,0.,-8.07042240638106E-15));
#47399=CARTESIAN_POINT('Origin',(67.6,0.,-8.07042240638106E-15));
#47400=CARTESIAN_POINT('Origin',(66.,0.,0.));
#47401=CARTESIAN_POINT('',(64.4,-134.2,-1.64347600445575E-14));
#47402=CARTESIAN_POINT('',(66.,-133.,-1.62878024286598E-14));
#47403=CARTESIAN_POINT('',(64.4,134.2,-1.64347600445575E-14));
#47404=CARTESIAN_POINT('Origin',(64.4,0.,-8.21738002227874E-15));
#47405=CARTESIAN_POINT('Origin',(64.4,0.,-8.21738002227874E-15));
#47406=CARTESIAN_POINT('Origin',(63.9659177056077,0.,-8.23193990075793E-15));
#47407=CARTESIAN_POINT('',(63.5318354112155,134.675561720794,1.64929995584742E-14));
#47408=CARTESIAN_POINT('',(63.9659177056077,134.437780860397,1.64638798015159E-14));
#47409=CARTESIAN_POINT('',(63.5318354112155,-134.675561720794,-1.64929995584742E-14));
#47410=CARTESIAN_POINT('Origin',(63.5318354112155,0.,-8.24649977923712E-15));
#47411=CARTESIAN_POINT('Origin',(63.5318354112155,0.,-8.24649977923712E-15));
#47412=CARTESIAN_POINT('Origin',(62.,0.,0.));
#47413=CARTESIAN_POINT('',(60.4681645887845,-135.824438279206,-1.66336963584617E-14));
#47414=CARTESIAN_POINT('',(62.,-135.25,-1.6563347958468E-14));
#47415=CARTESIAN_POINT('',(60.4681645887845,135.824438279206,-1.66336963584617E-14));
#47416=CARTESIAN_POINT('Origin',(60.4681645887845,0.,-8.31684817923083E-15));
#47417=CARTESIAN_POINT('Origin',(60.4681645887845,0.,-8.31684817923083E-15));
#47418=CARTESIAN_POINT('Origin',(59.9840822943923,0.,-4.15842408961541E-15));
#47419=CARTESIAN_POINT('',(59.5,136.,1.6655196468404E-14));
#47420=CARTESIAN_POINT('',(59.9840822943923,135.912219139603,1.66444464134328E-14));
#47421=CARTESIAN_POINT('',(59.5,-136.,-1.6655196468404E-14));
#47422=CARTESIAN_POINT('Origin',(59.5,0.,0.));
#47423=CARTESIAN_POINT('Origin',(59.5,0.,0.));
#47424=CARTESIAN_POINT('Origin',(36.,0.,0.));
#47425=CARTESIAN_POINT('',(58.,-136.,-1.6655196468404E-14));
#47426=CARTESIAN_POINT('',(36.,-136.,-1.6655196468404E-14));
#47427=CARTESIAN_POINT('',(58.,-135.997660312937,-0.797740187650247));
#47428=CARTESIAN_POINT('Origin',(58.,0.,0.));
#47429=CARTESIAN_POINT('',(57.5,-135.993780676136,-1.30062193238639));
#47430=CARTESIAN_POINT('Origin',(72.3260541341288,0.,0.));
#47431=CARTESIAN_POINT('',(14.5,-135.993780676136,-1.30062193238639));
#47432=CARTESIAN_POINT('',(36.,-135.993780676136,-1.30062193238639));
#47433=CARTESIAN_POINT('',(14.,-135.997660312937,-0.797740187650244));
#47434=CARTESIAN_POINT('Origin',(-0.32605413412881,0.,0.));
#47435=CARTESIAN_POINT('',(14.,-136.,-1.6655196468404E-14));
#47436=CARTESIAN_POINT('Origin',(14.,0.,0.));
#47437=CARTESIAN_POINT('',(12.,-136.,-1.6655196468404E-14));
#47438=CARTESIAN_POINT('',(36.,-136.,-1.6655196468404E-14));
#47439=CARTESIAN_POINT('Origin',(12.,0.,0.));
#47440=CARTESIAN_POINT('',(14.,-135.997660312937,0.797740187650262));
#47441=CARTESIAN_POINT('Origin',(14.,0.,0.));
#47442=CARTESIAN_POINT('',(14.5,-135.993780676136,1.3006219323864));
#47443=CARTESIAN_POINT('Origin',(-0.32605413412885,0.,0.));
#47444=CARTESIAN_POINT('',(57.5,-135.993780676136,1.3006219323864));
#47445=CARTESIAN_POINT('',(36.,-135.993780676136,1.3006219323864));
#47446=CARTESIAN_POINT('',(58.,-135.997660312937,0.797740187650262));
#47447=CARTESIAN_POINT('Origin',(72.3260541341288,0.,0.));
#47448=CARTESIAN_POINT('Origin',(58.,0.,0.));
#47449=CARTESIAN_POINT('',(57.5,-1.3006219323864,135.993780676136));
#47450=CARTESIAN_POINT('',(14.5,-1.3006219323864,135.993780676136));
#47451=CARTESIAN_POINT('',(36.,-1.3006219323864,135.993780676136));
#47452=CARTESIAN_POINT('',(14.,-0.797740187650253,135.997660312937));
#47453=CARTESIAN_POINT('Origin',(-0.326054134128819,0.,0.));
#47454=CARTESIAN_POINT('',(14.,0.797740187650255,135.997660312937));
#47455=CARTESIAN_POINT('Origin',(14.,0.,0.));
#47456=CARTESIAN_POINT('',(14.5,1.3006219323864,135.993780676136));
#47457=CARTESIAN_POINT('Origin',(-0.326054134128837,0.,0.));
#47458=CARTESIAN_POINT('',(57.5,1.3006219323864,135.993780676136));
#47459=CARTESIAN_POINT('',(36.,1.3006219323864,135.993780676136));
#47460=CARTESIAN_POINT('',(58.,0.797740187650255,135.997660312937));
#47461=CARTESIAN_POINT('Origin',(72.3260541341288,0.,0.));
#47462=CARTESIAN_POINT('',(58.,-0.797740187650253,135.997660312937));
#47463=CARTESIAN_POINT('Origin',(58.,0.,0.));
#47464=CARTESIAN_POINT('Origin',(72.3260541341288,0.,0.));
#47465=CARTESIAN_POINT('',(57.5,-13.1483116371559,135.362926612467));
#47466=CARTESIAN_POINT('',(14.5,-13.1483116371559,135.362926612467));
#47467=CARTESIAN_POINT('',(36.,-13.1483116371559,135.362926612467));
#47468=CARTESIAN_POINT('',(14.,-12.6476816419096,135.410620518056));
#47469=CARTESIAN_POINT('Origin',(-0.32605413412881,0.,0.));
#47470=CARTESIAN_POINT('',(14.,-11.0582725511258,135.549675795204));
#47471=CARTESIAN_POINT('Origin',(14.,0.,0.));
#47472=CARTESIAN_POINT('',(14.5,-10.5569662906256,135.589639953569));
#47473=CARTESIAN_POINT('Origin',(-0.326054134128801,0.,0.));
#47474=CARTESIAN_POINT('',(57.5,-10.5569662906256,135.589639953569));
#47475=CARTESIAN_POINT('',(36.,-10.5569662906256,135.589639953569));
#47476=CARTESIAN_POINT('',(58.,-11.0582725511258,135.549675795204));
#47477=CARTESIAN_POINT('Origin',(72.3260541341287,0.,0.));
#47478=CARTESIAN_POINT('',(58.,-12.6476816419096,135.410620518056));
#47479=CARTESIAN_POINT('Origin',(58.,0.,0.));
#47480=CARTESIAN_POINT('Origin',(72.3260541341288,0.,0.));
#47481=CARTESIAN_POINT('',(57.5,-24.8959347511991,133.701878942908));
#47482=CARTESIAN_POINT('',(14.5,-24.8959347511991,133.701878942908));
#47483=CARTESIAN_POINT('',(36.,-24.8959347511991,133.701878942908));
#47484=CARTESIAN_POINT('',(14.,-24.4013666019951,133.793024137864));
#47485=CARTESIAN_POINT('Origin',(-0.326054134128935,0.,0.));
#47486=CARTESIAN_POINT('',(14.,-22.8301251586203,134.070076397538));
#47487=CARTESIAN_POINT('Origin',(14.,0.,0.));
#47488=CARTESIAN_POINT('',(14.5,-22.3342096256954,134.153580199693));
#47489=CARTESIAN_POINT('Origin',(-0.32605413412921,0.,0.));
#47490=CARTESIAN_POINT('',(57.5,-22.3342096256954,134.153580199693));
#47491=CARTESIAN_POINT('',(36.,-22.3342096256954,134.153580199693));
#47492=CARTESIAN_POINT('',(58.,-22.8301251586203,134.070076397538));
#47493=CARTESIAN_POINT('Origin',(72.326054134129,0.,0.));
#47494=CARTESIAN_POINT('',(58.,-24.4013666019951,133.793024137864));
#47495=CARTESIAN_POINT('Origin',(58.,0.,0.));
#47496=CARTESIAN_POINT('Origin',(72.3260541341287,0.,0.));
#47497=CARTESIAN_POINT('',(57.5,-36.4540847692092,131.023279243191));
#47498=CARTESIAN_POINT('',(14.5,-36.4540847692092,131.023279243191));
#47499=CARTESIAN_POINT('',(36.,-36.4540847692092,131.023279243191));
#47500=CARTESIAN_POINT('',(14.,-35.9693424282914,131.157182057546));
#47501=CARTESIAN_POINT('Origin',(-0.326054134128735,0.,0.));
#47502=CARTESIAN_POINT('',(14.,-34.4282267284513,131.570122764761));
#47503=CARTESIAN_POINT('Origin',(14.,0.,0.));
#47504=CARTESIAN_POINT('',(14.5,-33.9414761397491,131.696530696351));
#47505=CARTESIAN_POINT('Origin',(-0.326054134129108,0.,0.));
#47506=CARTESIAN_POINT('',(57.5,-33.9414761397491,131.696530696351));
#47507=CARTESIAN_POINT('',(36.,-33.9414761397491,131.696530696351));
#47508=CARTESIAN_POINT('',(58.,-34.4282267284513,131.570122764761));
#47509=CARTESIAN_POINT('Origin',(72.3260541341289,0.,0.));
#47510=CARTESIAN_POINT('',(58.,-35.9693424282914,131.157182057546));
#47511=CARTESIAN_POINT('Origin',(58.,0.,0.));
#47512=CARTESIAN_POINT('Origin',(72.3260541341287,0.,0.));
#47513=CARTESIAN_POINT('',(57.5,-47.7347971905474,127.347513274415));
#47514=CARTESIAN_POINT('',(14.5,-47.7347971905474,127.347513274415));
#47515=CARTESIAN_POINT('',(36.,-47.7347971905474,127.347513274415));
#47516=CARTESIAN_POINT('',(14.,-47.2635698398256,127.523154626899));
#47517=CARTESIAN_POINT('Origin',(-0.326054134129197,0.,0.));
#47518=CARTESIAN_POINT('',(14.,-45.764308704547,128.068841053532));
#47519=CARTESIAN_POINT('Origin',(14.,0.,0.));
#47520=CARTESIAN_POINT('',(14.5,-45.2904275259558,128.23719107387));
#47521=CARTESIAN_POINT('Origin',(-0.326054134128597,0.,0.));
#47522=CARTESIAN_POINT('',(57.5,-45.2904275259558,128.23719107387));
#47523=CARTESIAN_POINT('',(36.,-45.2904275259558,128.23719107387));
#47524=CARTESIAN_POINT('',(58.,-45.764308704547,128.068841053532));
#47525=CARTESIAN_POINT('Origin',(72.3260541341288,0.,0.));
#47526=CARTESIAN_POINT('',(58.,-47.2635698398257,127.523154626899));
#47527=CARTESIAN_POINT('Origin',(58.,0.,0.));
#47528=CARTESIAN_POINT('Origin',(72.3260541341294,0.,0.));
#47529=CARTESIAN_POINT('',(57.5,-58.652218982207,122.702555835089));
#47530=CARTESIAN_POINT('',(14.5,-58.652218982207,122.702555835089));
#47531=CARTESIAN_POINT('',(36.,-58.652218982207,122.702555835089));
#47532=CARTESIAN_POINT('',(14.,-58.198092946355,122.918598988955));
#47533=CARTESIAN_POINT('Origin',(-0.326054134128229,0.,0.));
#47534=CARTESIAN_POINT('',(14.,-56.7520966581561,123.592878131805));
#47535=CARTESIAN_POINT('Origin',(14.,0.,0.));
#47536=CARTESIAN_POINT('',(14.5,-56.2946914115821,123.801888995583));
#47537=CARTESIAN_POINT('Origin',(-0.326054134128895,0.,0.));
#47538=CARTESIAN_POINT('',(57.5,-56.2946914115821,123.801888995583));
#47539=CARTESIAN_POINT('',(36.,-56.2946914115821,123.801888995583));
#47540=CARTESIAN_POINT('',(58.,-56.7520966581561,123.592878131805));
#47541=CARTESIAN_POINT('Origin',(72.3260541341286,0.,0.));
#47542=CARTESIAN_POINT('',(58.,-58.198092946355,122.918598988955));
#47543=CARTESIAN_POINT('Origin',(58.,0.,0.));
#47544=CARTESIAN_POINT('Origin',(72.3260541341284,0.,0.));
#47545=CARTESIAN_POINT('',(57.5,-69.1232619722338,117.12375785603));
#47546=CARTESIAN_POINT('',(14.5,-69.1232619722338,117.12375785603));
#47547=CARTESIAN_POINT('',(36.,-69.1232619722338,117.12375785603));
#47548=CARTESIAN_POINT('',(14.,-68.6896934245934,117.378558592425));
#47549=CARTESIAN_POINT('Origin',(-0.326054134128499,0.,0.));
#47550=CARTESIAN_POINT('',(14.,-67.3079668883436,118.176298780075));
#47551=CARTESIAN_POINT('Origin',(14.,0.,0.));
#47552=CARTESIAN_POINT('',(14.5,-66.8705187039022,118.424379788416));
#47553=CARTESIAN_POINT('Origin',(-0.326054134129121,0.,0.));
#47554=CARTESIAN_POINT('',(57.5,-66.8705187039022,118.424379788416));
#47555=CARTESIAN_POINT('',(36.,-66.8705187039022,118.424379788416));
#47556=CARTESIAN_POINT('',(58.,-67.3079668883436,118.176298780075));
#47557=CARTESIAN_POINT('Origin',(72.3260541341291,0.,0.));
#47558=CARTESIAN_POINT('',(58.,-68.6896934245934,117.378558592425));
#47559=CARTESIAN_POINT('Origin',(58.,0.,0.));
#47560=CARTESIAN_POINT('Origin',(72.3260541341284,0.,0.));
#47561=CARTESIAN_POINT('',(57.5,-79.0682352008853,110.653577358427));
#47562=CARTESIAN_POINT('',(14.5,-79.0682352008853,110.653577358427));
#47563=CARTESIAN_POINT('',(36.,-79.0682352008853,110.653577358427));
#47564=CARTESIAN_POINT('',(14.,-78.6585238598997,110.945196489896));
#47565=CARTESIAN_POINT('Origin',(-0.326054134129188,0.,0.));
#47566=CARTESIAN_POINT('',(14.,-77.3515828488493,111.860326437829));
#47567=CARTESIAN_POINT('Origin',(14.,0.,0.));
#47568=CARTESIAN_POINT('',(14.5,-76.9374209713625,112.145589544464));
#47569=CARTESIAN_POINT('Origin',(-0.326054134128935,0.,0.));
#47570=CARTESIAN_POINT('',(57.5,-76.9374209713625,112.145589544464));
#47571=CARTESIAN_POINT('',(36.,-76.9374209713625,112.145589544464));
#47572=CARTESIAN_POINT('',(58.,-77.3515828488493,111.860326437829));
#47573=CARTESIAN_POINT('Origin',(72.3260541341289,0.,0.));
#47574=CARTESIAN_POINT('',(58.,-78.6585238598997,110.945196489896));
#47575=CARTESIAN_POINT('Origin',(58.,0.,0.));
#47576=CARTESIAN_POINT('Origin',(72.3260541341289,0.,0.));
#47577=CARTESIAN_POINT('',(57.5,-88.4114514169522,103.341256322671));
#47578=CARTESIAN_POINT('',(14.5,-88.4114514169522,103.341256322671));
#47579=CARTESIAN_POINT('',(36.,-88.4114514169522,103.341256322671));
#47580=CARTESIAN_POINT('',(14.,-88.0287154333169,103.667474451537));
#47581=CARTESIAN_POINT('Origin',(-0.326054134129112,0.,0.));
#47582=CARTESIAN_POINT('',(14.,-86.8065065577125,104.693029468278));
#47583=CARTESIAN_POINT('Origin',(14.,0.,0.));
#47584=CARTESIAN_POINT('',(14.5,-86.4187830091457,105.01330364872));
#47585=CARTESIAN_POINT('Origin',(-0.326054134129139,0.,0.));
#47586=CARTESIAN_POINT('',(57.5,-86.4187830091457,105.01330364872));
#47587=CARTESIAN_POINT('',(36.,-86.4187830091457,105.01330364872));
#47588=CARTESIAN_POINT('',(58.,-86.8065065577126,104.693029468278));
#47589=CARTESIAN_POINT('Origin',(72.3260541341287,0.,0.));
#47590=CARTESIAN_POINT('',(58.,-88.0287154333169,103.667474451537));
#47591=CARTESIAN_POINT('Origin',(58.,0.,0.));
#47592=CARTESIAN_POINT('Origin',(72.3260541341291,0.,0.));
#47593=CARTESIAN_POINT('',(57.5,-97.0818031034423,95.2424459271415));
#47594=CARTESIAN_POINT('',(14.5,-97.0818031034423,95.2424459271415));
#47595=CARTESIAN_POINT('',(36.,-97.0818031034423,95.2424459271415));
#47596=CARTESIAN_POINT('',(14.,-96.7289553290949,95.6007803364699));
#47597=CARTESIAN_POINT('Origin',(-0.32605413412873,0.,0.));
#47598=CARTESIAN_POINT('',(14.,-95.6007803364699,96.7289553290949));
#47599=CARTESIAN_POINT('Origin',(14.,0.,0.));
#47600=CARTESIAN_POINT('',(14.5,-95.2424459271415,97.0818031034423));
#47601=CARTESIAN_POINT('Origin',(-0.326054134128722,0.,0.));
#47602=CARTESIAN_POINT('',(57.5,-95.2424459271415,97.0818031034423));
#47603=CARTESIAN_POINT('',(36.,-95.2424459271415,97.0818031034423));
#47604=CARTESIAN_POINT('',(58.,-95.6007803364699,96.7289553290949));
#47605=CARTESIAN_POINT('Origin',(72.3260541341287,0.,0.));
#47606=CARTESIAN_POINT('',(58.,-96.7289553290949,95.6007803364699));
#47607=CARTESIAN_POINT('Origin',(58.,0.,0.));
#47608=CARTESIAN_POINT('Origin',(72.3260541341287,0.,0.));
#47609=CARTESIAN_POINT('',(57.5,-105.01330364872,86.4187830091457));
#47610=CARTESIAN_POINT('',(14.5,-105.01330364872,86.4187830091457));
#47611=CARTESIAN_POINT('',(36.,-105.01330364872,86.4187830091457));
#47612=CARTESIAN_POINT('',(14.,-104.693029468278,86.8065065577126));
#47613=CARTESIAN_POINT('Origin',(-0.326054134128375,0.,0.));
#47614=CARTESIAN_POINT('',(14.,-103.667474451537,88.0287154333169));
#47615=CARTESIAN_POINT('Origin',(14.,0.,0.));
#47616=CARTESIAN_POINT('',(14.5,-103.341256322671,88.4114514169522));
#47617=CARTESIAN_POINT('Origin',(-0.326054134128864,0.,0.));
#47618=CARTESIAN_POINT('',(57.5,-103.341256322671,88.4114514169522));
#47619=CARTESIAN_POINT('',(36.,-103.341256322671,88.4114514169522));
#47620=CARTESIAN_POINT('',(58.,-103.667474451537,88.0287154333169));
#47621=CARTESIAN_POINT('Origin',(72.3260541341288,0.,0.));
#47622=CARTESIAN_POINT('',(58.,-104.693029468278,86.8065065577126));
#47623=CARTESIAN_POINT('Origin',(58.,0.,0.));
#47624=CARTESIAN_POINT('Origin',(72.3260541341287,0.,0.));
#47625=CARTESIAN_POINT('',(57.5,-112.145589544464,76.9374209713625));
#47626=CARTESIAN_POINT('',(14.5,-112.145589544464,76.9374209713625));
#47627=CARTESIAN_POINT('',(36.,-112.145589544464,76.9374209713625));
#47628=CARTESIAN_POINT('',(14.,-111.860326437829,77.3515828488493));
#47629=CARTESIAN_POINT('Origin',(-0.32605413412869,0.,0.));
#47630=CARTESIAN_POINT('',(14.,-110.945196489896,78.6585238598997));
#47631=CARTESIAN_POINT('Origin',(14.,0.,0.));
#47632=CARTESIAN_POINT('',(14.5,-110.653577358427,79.0682352008853));
#47633=CARTESIAN_POINT('Origin',(-0.326054134128939,0.,0.));
#47634=CARTESIAN_POINT('',(57.5,-110.653577358427,79.0682352008853));
#47635=CARTESIAN_POINT('',(36.,-110.653577358427,79.0682352008853));
#47636=CARTESIAN_POINT('',(58.,-110.945196489896,78.6585238598997));
#47637=CARTESIAN_POINT('Origin',(72.3260541341289,0.,0.));
#47638=CARTESIAN_POINT('',(58.,-111.860326437829,77.3515828488493));
#47639=CARTESIAN_POINT('Origin',(58.,0.,0.));
#47640=CARTESIAN_POINT('Origin',(72.3260541341286,0.,0.));
#47641=CARTESIAN_POINT('',(57.5,-118.424379788416,66.8705187039022));
#47642=CARTESIAN_POINT('',(14.5,-118.424379788416,66.8705187039022));
#47643=CARTESIAN_POINT('',(36.,-118.424379788416,66.8705187039022));
#47644=CARTESIAN_POINT('',(14.,-118.176298780075,67.3079668883436));
#47645=CARTESIAN_POINT('Origin',(-0.326054134129148,0.,0.));
#47646=CARTESIAN_POINT('',(14.,-117.378558592425,68.6896934245934));
#47647=CARTESIAN_POINT('Origin',(14.,0.,0.));
#47648=CARTESIAN_POINT('',(14.5,-117.12375785603,69.1232619722339));
#47649=CARTESIAN_POINT('Origin',(-0.326054134128753,0.,0.));
#47650=CARTESIAN_POINT('',(57.5,-117.12375785603,69.1232619722339));
#47651=CARTESIAN_POINT('',(36.,-117.12375785603,69.1232619722339));
#47652=CARTESIAN_POINT('',(58.,-117.378558592425,68.6896934245934));
#47653=CARTESIAN_POINT('Origin',(72.3260541341287,0.,0.));
#47654=CARTESIAN_POINT('',(58.,-118.176298780075,67.3079668883436));
#47655=CARTESIAN_POINT('Origin',(58.,0.,0.));
#47656=CARTESIAN_POINT('Origin',(72.3260541341285,0.,0.));
#47657=CARTESIAN_POINT('',(57.5,-123.801888995583,56.2946914115821));
#47658=CARTESIAN_POINT('',(14.5,-123.801888995583,56.2946914115821));
#47659=CARTESIAN_POINT('',(36.,-123.801888995583,56.2946914115821));
#47660=CARTESIAN_POINT('',(14.,-123.592878131805,56.7520966581561));
#47661=CARTESIAN_POINT('Origin',(-0.32605413412869,0.,0.));
#47662=CARTESIAN_POINT('',(14.,-122.918598988955,58.198092946355));
#47663=CARTESIAN_POINT('Origin',(14.,0.,0.));
#47664=CARTESIAN_POINT('',(14.5,-122.702555835089,58.652218982207));
#47665=CARTESIAN_POINT('Origin',(-0.326054134128726,0.,0.));
#47666=CARTESIAN_POINT('',(57.5,-122.702555835089,58.652218982207));
#47667=CARTESIAN_POINT('',(36.,-122.702555835089,58.652218982207));
#47668=CARTESIAN_POINT('',(58.,-122.918598988955,58.198092946355));
#47669=CARTESIAN_POINT('Origin',(72.3260541341287,0.,0.));
#47670=CARTESIAN_POINT('',(58.,-123.592878131805,56.7520966581561));
#47671=CARTESIAN_POINT('Origin',(58.,0.,0.));
#47672=CARTESIAN_POINT('Origin',(72.3260541341286,0.,0.));
#47673=CARTESIAN_POINT('',(57.5,-128.23719107387,45.2904275259558));
#47674=CARTESIAN_POINT('',(14.5,-128.23719107387,45.2904275259558));
#47675=CARTESIAN_POINT('',(36.,-128.23719107387,45.2904275259558));
#47676=CARTESIAN_POINT('',(14.,-128.068841053532,45.764308704547));
#47677=CARTESIAN_POINT('Origin',(-0.326054134128846,0.,0.));
#47678=CARTESIAN_POINT('',(14.,-127.523154626899,47.2635698398257));
#47679=CARTESIAN_POINT('Origin',(14.,0.,0.));
#47680=CARTESIAN_POINT('',(14.5,-127.347513274415,47.7347971905474));
#47681=CARTESIAN_POINT('Origin',(-0.326054134129197,0.,0.));
#47682=CARTESIAN_POINT('',(57.5,-127.347513274415,47.7347971905474));
#47683=CARTESIAN_POINT('',(36.,-127.347513274415,47.7347971905474));
#47684=CARTESIAN_POINT('',(58.,-127.523154626899,47.2635698398257));
#47685=CARTESIAN_POINT('Origin',(72.3260541341291,0.,0.));
#47686=CARTESIAN_POINT('',(58.,-128.068841053532,45.764308704547));
#47687=CARTESIAN_POINT('Origin',(58.,0.,0.));
#47688=CARTESIAN_POINT('Origin',(72.3260541341288,0.,0.));
#47689=CARTESIAN_POINT('',(57.5,-131.696530696351,33.9414761397492));
#47690=CARTESIAN_POINT('',(14.5,-131.696530696351,33.9414761397492));
#47691=CARTESIAN_POINT('',(36.,-131.696530696351,33.9414761397492));
#47692=CARTESIAN_POINT('',(14.,-131.570122764761,34.4282267284513));
#47693=CARTESIAN_POINT('Origin',(-0.326054134128975,0.,0.));
#47694=CARTESIAN_POINT('',(14.,-131.157182057546,35.9693424282914));
#47695=CARTESIAN_POINT('Origin',(14.,0.,0.));
#47696=CARTESIAN_POINT('',(14.5,-131.023279243191,36.4540847692092));
#47697=CARTESIAN_POINT('Origin',(-0.326054134128864,0.,0.));
#47698=CARTESIAN_POINT('',(57.5,-131.023279243191,36.4540847692092));
#47699=CARTESIAN_POINT('',(36.,-131.023279243191,36.4540847692092));
#47700=CARTESIAN_POINT('',(58.,-131.157182057546,35.9693424282914));
#47701=CARTESIAN_POINT('Origin',(72.3260541341288,0.,0.));
#47702=CARTESIAN_POINT('',(58.,-131.570122764761,34.4282267284513));
#47703=CARTESIAN_POINT('Origin',(58.,0.,0.));
#47704=CARTESIAN_POINT('Origin',(72.3260541341289,0.,0.));
#47705=CARTESIAN_POINT('',(57.5,-134.153580199693,22.3342096256954));
#47706=CARTESIAN_POINT('',(14.5,-134.153580199693,22.3342096256954));
#47707=CARTESIAN_POINT('',(36.,-134.153580199693,22.3342096256954));
#47708=CARTESIAN_POINT('',(14.,-134.070076397538,22.8301251586204));
#47709=CARTESIAN_POINT('Origin',(-0.326054134128957,0.,0.));
#47710=CARTESIAN_POINT('',(14.,-133.793024137864,24.4013666019951));
#47711=CARTESIAN_POINT('Origin',(14.,0.,0.));
#47712=CARTESIAN_POINT('',(14.5,-133.701878942908,24.8959347511991));
#47713=CARTESIAN_POINT('Origin',(-0.326054134128939,0.,0.));
#47714=CARTESIAN_POINT('',(57.5,-133.701878942908,24.8959347511991));
#47715=CARTESIAN_POINT('',(36.,-133.701878942908,24.8959347511991));
#47716=CARTESIAN_POINT('',(58.,-133.793024137864,24.4013666019951));
#47717=CARTESIAN_POINT('Origin',(72.3260541341289,0.,0.));
#47718=CARTESIAN_POINT('',(58.,-134.070076397538,22.8301251586204));
#47719=CARTESIAN_POINT('Origin',(58.,0.,0.));
#47720=CARTESIAN_POINT('Origin',(72.3260541341289,0.,0.));
#47721=CARTESIAN_POINT('',(57.5,-135.589639953569,10.5569662906256));
#47722=CARTESIAN_POINT('',(14.5,-135.589639953569,10.5569662906256));
#47723=CARTESIAN_POINT('',(36.,-135.589639953569,10.5569662906256));
#47724=CARTESIAN_POINT('',(14.,-135.549675795204,11.0582725511259));
#47725=CARTESIAN_POINT('Origin',(-0.32605413412893,0.,0.));
#47726=CARTESIAN_POINT('',(14.,-135.410620518056,12.6476816419097));
#47727=CARTESIAN_POINT('Origin',(14.,0.,0.));
#47728=CARTESIAN_POINT('',(14.5,-135.362926612467,13.148311637156));
#47729=CARTESIAN_POINT('Origin',(-0.32605413412881,0.,0.));
#47730=CARTESIAN_POINT('',(57.5,-135.362926612467,13.148311637156));
#47731=CARTESIAN_POINT('',(36.,-135.362926612467,13.148311637156));
#47732=CARTESIAN_POINT('',(58.,-135.410620518056,12.6476816419097));
#47733=CARTESIAN_POINT('Origin',(72.3260541341288,0.,0.));
#47734=CARTESIAN_POINT('',(58.,-135.549675795204,11.0582725511259));
#47735=CARTESIAN_POINT('Origin',(58.,0.,0.));
#47736=CARTESIAN_POINT('Origin',(72.3260541341289,0.,0.));
#47737=CARTESIAN_POINT('',(57.5,-135.362926612467,-13.1483116371559));
#47738=CARTESIAN_POINT('',(14.5,-135.362926612467,-13.1483116371559));
#47739=CARTESIAN_POINT('',(36.,-135.362926612467,-13.1483116371559));
#47740=CARTESIAN_POINT('',(14.,-135.410620518056,-12.6476816419096));
#47741=CARTESIAN_POINT('Origin',(-0.32605413412881,0.,0.));
#47742=CARTESIAN_POINT('',(14.,-135.549675795204,-11.0582725511258));
#47743=CARTESIAN_POINT('Origin',(14.,0.,0.));
#47744=CARTESIAN_POINT('',(14.5,-135.589639953569,-10.5569662906256));
#47745=CARTESIAN_POINT('Origin',(-0.326054134128806,0.,0.));
#47746=CARTESIAN_POINT('',(57.5,-135.589639953569,-10.5569662906256));
#47747=CARTESIAN_POINT('',(36.,-135.589639953569,-10.5569662906256));
#47748=CARTESIAN_POINT('',(58.,-135.549675795204,-11.0582725511258));
#47749=CARTESIAN_POINT('Origin',(72.3260541341287,0.,0.));
#47750=CARTESIAN_POINT('',(58.,-135.410620518056,-12.6476816419096));
#47751=CARTESIAN_POINT('Origin',(58.,0.,0.));
#47752=CARTESIAN_POINT('Origin',(72.3260541341288,0.,0.));
#47753=CARTESIAN_POINT('',(57.5,-133.701878942908,-24.8959347511991));
#47754=CARTESIAN_POINT('',(14.5,-133.701878942908,-24.8959347511991));
#47755=CARTESIAN_POINT('',(36.,-133.701878942908,-24.8959347511991));
#47756=CARTESIAN_POINT('',(14.,-133.793024137864,-24.4013666019951));
#47757=CARTESIAN_POINT('Origin',(-0.326054134128806,0.,0.));
#47758=CARTESIAN_POINT('',(14.,-134.070076397538,-22.8301251586203));
#47759=CARTESIAN_POINT('Origin',(14.,0.,0.));
#47760=CARTESIAN_POINT('',(14.5,-134.153580199693,-22.3342096256954));
#47761=CARTESIAN_POINT('Origin',(-0.32605413412921,0.,0.));
#47762=CARTESIAN_POINT('',(57.5,-134.153580199693,-22.3342096256954));
#47763=CARTESIAN_POINT('',(36.,-134.153580199693,-22.3342096256954));
#47764=CARTESIAN_POINT('',(58.,-134.070076397538,-22.8301251586203));
#47765=CARTESIAN_POINT('Origin',(72.3260541341289,0.,0.));
#47766=CARTESIAN_POINT('',(58.,-133.793024137864,-24.4013666019951));
#47767=CARTESIAN_POINT('Origin',(58.,0.,0.));
#47768=CARTESIAN_POINT('Origin',(72.3260541341287,0.,0.));
#47769=CARTESIAN_POINT('',(57.5,-131.023279243191,-36.4540847692092));
#47770=CARTESIAN_POINT('',(14.5,-131.023279243191,-36.4540847692092));
#47771=CARTESIAN_POINT('',(36.,-131.023279243191,-36.4540847692092));
#47772=CARTESIAN_POINT('',(14.,-131.157182057546,-35.9693424282914));
#47773=CARTESIAN_POINT('Origin',(-0.326054134128735,0.,0.));
#47774=CARTESIAN_POINT('',(14.,-131.570122764761,-34.4282267284513));
#47775=CARTESIAN_POINT('Origin',(14.,0.,0.));
#47776=CARTESIAN_POINT('',(14.5,-131.696530696351,-33.9414761397491));
#47777=CARTESIAN_POINT('Origin',(-0.326054134128984,0.,0.));
#47778=CARTESIAN_POINT('',(57.5,-131.696530696351,-33.9414761397491));
#47779=CARTESIAN_POINT('',(36.,-131.696530696351,-33.9414761397491));
#47780=CARTESIAN_POINT('',(58.,-131.570122764761,-34.4282267284513));
#47781=CARTESIAN_POINT('Origin',(72.3260541341289,0.,0.));
#47782=CARTESIAN_POINT('',(58.,-131.157182057546,-35.9693424282914));
#47783=CARTESIAN_POINT('Origin',(58.,0.,0.));
#47784=CARTESIAN_POINT('Origin',(72.3260541341289,0.,0.));
#47785=CARTESIAN_POINT('',(57.5,-127.347513274415,-47.7347971905474));
#47786=CARTESIAN_POINT('',(14.5,-127.347513274415,-47.7347971905474));
#47787=CARTESIAN_POINT('',(36.,-127.347513274415,-47.7347971905474));
#47788=CARTESIAN_POINT('',(14.,-127.523154626899,-47.2635698398256));
#47789=CARTESIAN_POINT('Origin',(-0.326054134129197,0.,0.));
#47790=CARTESIAN_POINT('',(14.,-128.068841053532,-45.764308704547));
#47791=CARTESIAN_POINT('Origin',(14.,0.,0.));
#47792=CARTESIAN_POINT('',(14.5,-128.23719107387,-45.2904275259558));
#47793=CARTESIAN_POINT('Origin',(-0.326054134128606,0.,0.));
#47794=CARTESIAN_POINT('',(57.5,-128.23719107387,-45.2904275259558));
#47795=CARTESIAN_POINT('',(36.,-128.23719107387,-45.2904275259558));
#47796=CARTESIAN_POINT('',(58.,-128.068841053532,-45.764308704547));
#47797=CARTESIAN_POINT('Origin',(72.3260541341288,0.,0.));
#47798=CARTESIAN_POINT('',(58.,-127.523154626899,-47.2635698398257));
#47799=CARTESIAN_POINT('Origin',(58.,0.,0.));
#47800=CARTESIAN_POINT('Origin',(72.3260541341294,0.,0.));
#47801=CARTESIAN_POINT('',(57.5,-122.702555835089,-58.652218982207));
#47802=CARTESIAN_POINT('',(14.5,-122.702555835089,-58.652218982207));
#47803=CARTESIAN_POINT('',(36.,-122.702555835089,-58.652218982207));
#47804=CARTESIAN_POINT('',(14.,-122.918598988955,-58.198092946355));
#47805=CARTESIAN_POINT('Origin',(-0.326054134128735,0.,0.));
#47806=CARTESIAN_POINT('',(14.,-123.592878131805,-56.752096658156));
#47807=CARTESIAN_POINT('Origin',(14.,0.,0.));
#47808=CARTESIAN_POINT('',(14.5,-123.801888995583,-56.2946914115821));
#47809=CARTESIAN_POINT('Origin',(-0.326054134129112,0.,0.));
#47810=CARTESIAN_POINT('',(57.5,-123.801888995583,-56.2946914115821));
#47811=CARTESIAN_POINT('',(36.,-123.801888995583,-56.2946914115821));
#47812=CARTESIAN_POINT('',(58.,-123.592878131805,-56.752096658156));
#47813=CARTESIAN_POINT('Origin',(72.3260541341288,0.,0.));
#47814=CARTESIAN_POINT('',(58.,-122.918598988955,-58.198092946355));
#47815=CARTESIAN_POINT('Origin',(58.,0.,0.));
#47816=CARTESIAN_POINT('Origin',(72.3260541341287,0.,0.));
#47817=CARTESIAN_POINT('',(57.5,-117.12375785603,-69.1232619722338));
#47818=CARTESIAN_POINT('',(14.5,-117.12375785603,-69.1232619722338));
#47819=CARTESIAN_POINT('',(36.,-117.12375785603,-69.1232619722338));
#47820=CARTESIAN_POINT('',(14.,-117.378558592425,-68.6896934245934));
#47821=CARTESIAN_POINT('Origin',(-0.32605413412877,0.,0.));
#47822=CARTESIAN_POINT('',(14.,-118.176298780075,-67.3079668883436));
#47823=CARTESIAN_POINT('Origin',(14.,0.,0.));
#47824=CARTESIAN_POINT('',(14.5,-118.424379788416,-66.8705187039022));
#47825=CARTESIAN_POINT('Origin',(-0.326054134129108,0.,0.));
#47826=CARTESIAN_POINT('',(57.5,-118.424379788416,-66.8705187039022));
#47827=CARTESIAN_POINT('',(36.,-118.424379788416,-66.8705187039022));
#47828=CARTESIAN_POINT('',(58.,-118.176298780075,-67.3079668883436));
#47829=CARTESIAN_POINT('Origin',(72.3260541341291,0.,0.));
#47830=CARTESIAN_POINT('',(58.,-117.378558592425,-68.6896934245934));
#47831=CARTESIAN_POINT('Origin',(58.,0.,0.));
#47832=CARTESIAN_POINT('Origin',(72.3260541341287,0.,0.));
#47833=CARTESIAN_POINT('',(57.5,-110.653577358427,-79.0682352008852));
#47834=CARTESIAN_POINT('',(14.5,-110.653577358427,-79.0682352008852));
#47835=CARTESIAN_POINT('',(36.,-110.653577358427,-79.0682352008852));
#47836=CARTESIAN_POINT('',(14.,-110.945196489896,-78.6585238598997));
#47837=CARTESIAN_POINT('Origin',(-0.326054134128948,0.,0.));
#47838=CARTESIAN_POINT('',(14.,-111.860326437829,-77.3515828488493));
#47839=CARTESIAN_POINT('Origin',(14.,0.,0.));
#47840=CARTESIAN_POINT('',(14.5,-112.145589544464,-76.9374209713624));
#47841=CARTESIAN_POINT('Origin',(-0.326054134128895,0.,0.));
#47842=CARTESIAN_POINT('',(57.5,-112.145589544464,-76.9374209713624));
#47843=CARTESIAN_POINT('',(36.,-112.145589544464,-76.9374209713624));
#47844=CARTESIAN_POINT('',(58.,-111.860326437829,-77.3515828488493));
#47845=CARTESIAN_POINT('Origin',(72.3260541341289,0.,0.));
#47846=CARTESIAN_POINT('',(58.,-110.945196489896,-78.6585238598997));
#47847=CARTESIAN_POINT('Origin',(58.,0.,0.));
#47848=CARTESIAN_POINT('Origin',(72.3260541341289,0.,0.));
#47849=CARTESIAN_POINT('',(57.5,-103.341256322671,-88.4114514169522));
#47850=CARTESIAN_POINT('',(14.5,-103.341256322671,-88.4114514169522));
#47851=CARTESIAN_POINT('',(36.,-103.341256322671,-88.4114514169522));
#47852=CARTESIAN_POINT('',(14.,-103.667474451537,-88.0287154333169));
#47853=CARTESIAN_POINT('Origin',(-0.326054134129112,0.,0.));
#47854=CARTESIAN_POINT('',(14.,-104.693029468278,-86.8065065577126));
#47855=CARTESIAN_POINT('Origin',(14.,0.,0.));
#47856=CARTESIAN_POINT('',(14.5,-105.01330364872,-86.4187830091457));
#47857=CARTESIAN_POINT('Origin',(-0.326054134128748,0.,0.));
#47858=CARTESIAN_POINT('',(57.5,-105.01330364872,-86.4187830091457));
#47859=CARTESIAN_POINT('',(36.,-105.01330364872,-86.4187830091457));
#47860=CARTESIAN_POINT('',(58.,-104.693029468278,-86.8065065577126));
#47861=CARTESIAN_POINT('Origin',(72.3260541341287,0.,0.));
#47862=CARTESIAN_POINT('',(58.,-103.667474451537,-88.0287154333169));
#47863=CARTESIAN_POINT('Origin',(58.,0.,0.));
#47864=CARTESIAN_POINT('Origin',(72.3260541341291,0.,0.));
#47865=CARTESIAN_POINT('',(57.5,-95.2424459271415,-97.0818031034422));
#47866=CARTESIAN_POINT('',(14.5,-95.2424459271415,-97.0818031034422));
#47867=CARTESIAN_POINT('',(36.,-95.2424459271415,-97.0818031034422));
#47868=CARTESIAN_POINT('',(14.,-95.6007803364699,-96.7289553290949));
#47869=CARTESIAN_POINT('Origin',(-0.326054134128722,0.,0.));
#47870=CARTESIAN_POINT('',(14.,-96.7289553290949,-95.6007803364699));
#47871=CARTESIAN_POINT('Origin',(14.,0.,0.));
#47872=CARTESIAN_POINT('',(14.5,-97.0818031034423,-95.2424459271415));
#47873=CARTESIAN_POINT('Origin',(-0.326054134128717,0.,0.));
#47874=CARTESIAN_POINT('',(57.5,-97.0818031034423,-95.2424459271415));
#47875=CARTESIAN_POINT('',(36.,-97.0818031034423,-95.2424459271415));
#47876=CARTESIAN_POINT('',(58.,-96.7289553290949,-95.6007803364698));
#47877=CARTESIAN_POINT('Origin',(72.3260541341287,0.,0.));
#47878=CARTESIAN_POINT('',(58.,-95.6007803364699,-96.7289553290949));
#47879=CARTESIAN_POINT('Origin',(58.,0.,0.));
#47880=CARTESIAN_POINT('Origin',(72.3260541341287,0.,0.));
#47881=CARTESIAN_POINT('',(57.5,-86.4187830091457,-105.01330364872));
#47882=CARTESIAN_POINT('',(14.5,-86.4187830091457,-105.01330364872));
#47883=CARTESIAN_POINT('',(36.,-86.4187830091457,-105.01330364872));
#47884=CARTESIAN_POINT('',(14.,-86.8065065577126,-104.693029468278));
#47885=CARTESIAN_POINT('Origin',(-0.326054134128375,0.,0.));
#47886=CARTESIAN_POINT('',(14.,-88.0287154333169,-103.667474451537));
#47887=CARTESIAN_POINT('Origin',(14.,0.,0.));
#47888=CARTESIAN_POINT('',(14.5,-88.4114514169522,-103.34125632267));
#47889=CARTESIAN_POINT('Origin',(-0.326054134128846,0.,0.));
#47890=CARTESIAN_POINT('',(57.5,-88.4114514169522,-103.34125632267));
#47891=CARTESIAN_POINT('',(36.,-88.4114514169522,-103.34125632267));
#47892=CARTESIAN_POINT('',(58.,-88.0287154333169,-103.667474451537));
#47893=CARTESIAN_POINT('Origin',(72.3260541341288,0.,0.));
#47894=CARTESIAN_POINT('',(58.,-86.8065065577126,-104.693029468278));
#47895=CARTESIAN_POINT('Origin',(58.,0.,0.));
#47896=CARTESIAN_POINT('Origin',(72.3260541341283,0.,0.));
#47897=CARTESIAN_POINT('',(57.5,-76.9374209713625,-112.145589544464));
#47898=CARTESIAN_POINT('',(14.5,-76.9374209713625,-112.145589544464));
#47899=CARTESIAN_POINT('',(36.,-76.9374209713625,-112.145589544464));
#47900=CARTESIAN_POINT('',(14.,-77.3515828488493,-111.860326437829));
#47901=CARTESIAN_POINT('Origin',(-0.326054134129095,0.,0.));
#47902=CARTESIAN_POINT('',(14.,-78.6585238598997,-110.945196489896));
#47903=CARTESIAN_POINT('Origin',(14.,0.,0.));
#47904=CARTESIAN_POINT('',(14.5,-79.0682352008853,-110.653577358427));
#47905=CARTESIAN_POINT('Origin',(-0.326054134128939,0.,0.));
#47906=CARTESIAN_POINT('',(57.5,-79.0682352008853,-110.653577358427));
#47907=CARTESIAN_POINT('',(36.,-79.0682352008853,-110.653577358427));
#47908=CARTESIAN_POINT('',(58.,-78.6585238598997,-110.945196489896));
#47909=CARTESIAN_POINT('Origin',(72.3260541341289,0.,0.));
#47910=CARTESIAN_POINT('',(58.,-77.3515828488494,-111.860326437829));
#47911=CARTESIAN_POINT('Origin',(58.,0.,0.));
#47912=CARTESIAN_POINT('Origin',(72.3260541341286,0.,0.));
#47913=CARTESIAN_POINT('',(57.5,-66.8705187039022,-118.424379788416));
#47914=CARTESIAN_POINT('',(14.5,-66.8705187039022,-118.424379788416));
#47915=CARTESIAN_POINT('',(36.,-66.8705187039022,-118.424379788416));
#47916=CARTESIAN_POINT('',(14.,-67.3079668883436,-118.176298780075));
#47917=CARTESIAN_POINT('Origin',(-0.326054134128908,0.,0.));
#47918=CARTESIAN_POINT('',(14.,-68.6896934245934,-117.378558592425));
#47919=CARTESIAN_POINT('Origin',(14.,0.,0.));
#47920=CARTESIAN_POINT('',(14.5,-69.1232619722338,-117.12375785603));
#47921=CARTESIAN_POINT('Origin',(-0.326054134128504,0.,0.));
#47922=CARTESIAN_POINT('',(57.5,-69.1232619722338,-117.12375785603));
#47923=CARTESIAN_POINT('',(36.,-69.1232619722338,-117.12375785603));
#47924=CARTESIAN_POINT('',(58.,-68.6896934245934,-117.378558592425));
#47925=CARTESIAN_POINT('Origin',(72.3260541341287,0.,0.));
#47926=CARTESIAN_POINT('',(58.,-67.3079668883436,-118.176298780075));
#47927=CARTESIAN_POINT('Origin',(58.,0.,0.));
#47928=CARTESIAN_POINT('Origin',(72.3260541341288,0.,0.));
#47929=CARTESIAN_POINT('',(57.5,-56.2946914115821,-123.801888995583));
#47930=CARTESIAN_POINT('',(14.5,-56.2946914115821,-123.801888995583));
#47931=CARTESIAN_POINT('',(36.,-56.2946914115821,-123.801888995583));
#47932=CARTESIAN_POINT('',(14.,-56.7520966581561,-123.592878131805));
#47933=CARTESIAN_POINT('Origin',(-0.326054134128895,0.,0.));
#47934=CARTESIAN_POINT('',(14.,-58.198092946355,-122.918598988955));
#47935=CARTESIAN_POINT('Origin',(14.,0.,0.));
#47936=CARTESIAN_POINT('',(14.5,-58.652218982207,-122.702555835089));
#47937=CARTESIAN_POINT('Origin',(-0.326054134128477,0.,0.));
#47938=CARTESIAN_POINT('',(57.5,-58.652218982207,-122.702555835089));
#47939=CARTESIAN_POINT('',(36.,-58.652218982207,-122.702555835089));
#47940=CARTESIAN_POINT('',(58.,-58.198092946355,-122.918598988955));
#47941=CARTESIAN_POINT('Origin',(72.3260541341284,0.,0.));
#47942=CARTESIAN_POINT('',(58.,-56.7520966581561,-123.592878131805));
#47943=CARTESIAN_POINT('Origin',(58.,0.,0.));
#47944=CARTESIAN_POINT('Origin',(72.3260541341288,0.,0.));
#47945=CARTESIAN_POINT('',(57.5,-45.2904275259558,-128.23719107387));
#47946=CARTESIAN_POINT('',(14.5,-45.2904275259558,-128.23719107387));
#47947=CARTESIAN_POINT('',(36.,-45.2904275259558,-128.23719107387));
#47948=CARTESIAN_POINT('',(14.,-45.764308704547,-128.068841053532));
#47949=CARTESIAN_POINT('Origin',(-0.326054134129086,0.,0.));
#47950=CARTESIAN_POINT('',(14.,-47.2635698398257,-127.523154626899));
#47951=CARTESIAN_POINT('Origin',(14.,0.,0.));
#47952=CARTESIAN_POINT('',(14.5,-47.7347971905474,-127.347513274415));
#47953=CARTESIAN_POINT('Origin',(-0.326054134129183,0.,0.));
#47954=CARTESIAN_POINT('',(57.5,-47.7347971905474,-127.347513274415));
#47955=CARTESIAN_POINT('',(36.,-47.7347971905474,-127.347513274415));
#47956=CARTESIAN_POINT('',(58.,-47.2635698398257,-127.523154626899));
#47957=CARTESIAN_POINT('Origin',(72.3260541341291,0.,0.));
#47958=CARTESIAN_POINT('',(58.,-45.764308704547,-128.068841053532));
#47959=CARTESIAN_POINT('Origin',(58.,0.,0.));
#47960=CARTESIAN_POINT('Origin',(72.3260541341288,0.,0.));
#47961=CARTESIAN_POINT('',(57.5,-33.9414761397492,-131.696530696351));
#47962=CARTESIAN_POINT('',(14.5,-33.9414761397492,-131.696530696351));
#47963=CARTESIAN_POINT('',(36.,-33.9414761397492,-131.696530696351));
#47964=CARTESIAN_POINT('',(14.,-34.4282267284513,-131.570122764761));
#47965=CARTESIAN_POINT('Origin',(-0.326054134128837,0.,0.));
#47966=CARTESIAN_POINT('',(14.,-35.9693424282914,-131.157182057546));
#47967=CARTESIAN_POINT('Origin',(14.,0.,0.));
#47968=CARTESIAN_POINT('',(14.5,-36.4540847692092,-131.023279243191));
#47969=CARTESIAN_POINT('Origin',(-0.326054134128855,0.,0.));
#47970=CARTESIAN_POINT('',(57.5,-36.4540847692092,-131.023279243191));
#47971=CARTESIAN_POINT('',(36.,-36.4540847692092,-131.023279243191));
#47972=CARTESIAN_POINT('',(58.,-35.9693424282914,-131.157182057546));
#47973=CARTESIAN_POINT('Origin',(72.3260541341288,0.,0.));
#47974=CARTESIAN_POINT('',(58.,-34.4282267284513,-131.570122764761));
#47975=CARTESIAN_POINT('Origin',(58.,0.,0.));
#47976=CARTESIAN_POINT('Origin',(72.3260541341289,0.,0.));
#47977=CARTESIAN_POINT('',(57.5,-22.3342096256954,-134.153580199693));
#47978=CARTESIAN_POINT('',(14.5,-22.3342096256954,-134.153580199693));
#47979=CARTESIAN_POINT('',(36.,-22.3342096256954,-134.153580199693));
#47980=CARTESIAN_POINT('',(14.,-22.8301251586204,-134.070076397538));
#47981=CARTESIAN_POINT('Origin',(-0.326054134129081,0.,0.));
#47982=CARTESIAN_POINT('',(14.,-24.4013666019952,-133.793024137864));
#47983=CARTESIAN_POINT('Origin',(14.,0.,0.));
#47984=CARTESIAN_POINT('',(14.5,-24.8959347511991,-133.701878942908));
#47985=CARTESIAN_POINT('Origin',(-0.326054134128686,0.,0.));
#47986=CARTESIAN_POINT('',(57.5,-24.8959347511991,-133.701878942908));
#47987=CARTESIAN_POINT('',(36.,-24.8959347511991,-133.701878942908));
#47988=CARTESIAN_POINT('',(58.,-24.4013666019952,-133.793024137864));
#47989=CARTESIAN_POINT('Origin',(72.3260541341286,0.,0.));
#47990=CARTESIAN_POINT('',(58.,-22.8301251586204,-134.070076397538));
#47991=CARTESIAN_POINT('Origin',(58.,0.,0.));
#47992=CARTESIAN_POINT('Origin',(72.326054134129,0.,0.));
#47993=CARTESIAN_POINT('',(57.5,-10.5569662906256,-135.589639953569));
#47994=CARTESIAN_POINT('',(14.5,-10.5569662906256,-135.589639953569));
#47995=CARTESIAN_POINT('',(36.,-10.5569662906256,-135.589639953569));
#47996=CARTESIAN_POINT('',(14.,-11.0582725511258,-135.549675795204));
#47997=CARTESIAN_POINT('Origin',(-0.326054134128864,0.,0.));
#47998=CARTESIAN_POINT('',(14.,-12.6476816419096,-135.410620518056));
#47999=CARTESIAN_POINT('Origin',(14.,0.,0.));
#48000=CARTESIAN_POINT('',(14.5,-13.1483116371559,-135.362926612467));
#48001=CARTESIAN_POINT('Origin',(-0.326054134128744,0.,0.));
#48002=CARTESIAN_POINT('',(57.5,-13.1483116371559,-135.362926612467));
#48003=CARTESIAN_POINT('',(36.,-13.1483116371559,-135.362926612467));
#48004=CARTESIAN_POINT('',(58.,-12.6476816419096,-135.410620518056));
#48005=CARTESIAN_POINT('Origin',(72.3260541341288,0.,0.));
#48006=CARTESIAN_POINT('',(58.,-11.0582725511258,-135.549675795204));
#48007=CARTESIAN_POINT('Origin',(58.,0.,0.));
#48008=CARTESIAN_POINT('Origin',(72.3260541341289,0.,0.));
#48009=CARTESIAN_POINT('',(57.5,1.30062193238638,-135.993780676136));
#48010=CARTESIAN_POINT('',(14.5,1.30062193238638,-135.993780676136));
#48011=CARTESIAN_POINT('',(36.,1.30062193238638,-135.993780676136));
#48012=CARTESIAN_POINT('',(14.,0.797740187650235,-135.997660312937));
#48013=CARTESIAN_POINT('Origin',(-0.326054134128824,0.,0.));
#48014=CARTESIAN_POINT('',(14.,-0.797740187650269,-135.997660312937));
#48015=CARTESIAN_POINT('Origin',(14.,0.,0.));
#48016=CARTESIAN_POINT('',(14.5,-1.30062193238641,-135.993780676136));
#48017=CARTESIAN_POINT('Origin',(-0.326054134128819,0.,0.));
#48018=CARTESIAN_POINT('',(57.5,-1.30062193238641,-135.993780676136));
#48019=CARTESIAN_POINT('',(36.,-1.30062193238641,-135.993780676136));
#48020=CARTESIAN_POINT('',(58.,-0.797740187650269,-135.997660312937));
#48021=CARTESIAN_POINT('Origin',(72.3260541341288,0.,0.));
#48022=CARTESIAN_POINT('',(58.,0.797740187650238,-135.997660312937));
#48023=CARTESIAN_POINT('Origin',(58.,0.,0.));
#48024=CARTESIAN_POINT('Origin',(72.3260541341288,0.,0.));
#48025=CARTESIAN_POINT('',(57.5,13.1483116371559,-135.362926612467));
#48026=CARTESIAN_POINT('',(14.5,13.1483116371559,-135.362926612467));
#48027=CARTESIAN_POINT('',(36.,13.1483116371559,-135.362926612467));
#48028=CARTESIAN_POINT('',(14.,12.6476816419096,-135.410620518056));
#48029=CARTESIAN_POINT('Origin',(-0.32605413412881,0.,0.));
#48030=CARTESIAN_POINT('',(14.,11.0582725511258,-135.549675795204));
#48031=CARTESIAN_POINT('Origin',(14.,0.,0.));
#48032=CARTESIAN_POINT('',(14.5,10.5569662906256,-135.589639953569));
#48033=CARTESIAN_POINT('Origin',(-0.326054134128806,0.,0.));
#48034=CARTESIAN_POINT('',(57.5,10.5569662906256,-135.589639953569));
#48035=CARTESIAN_POINT('',(36.,10.5569662906256,-135.589639953569));
#48036=CARTESIAN_POINT('',(58.,11.0582725511258,-135.549675795204));
#48037=CARTESIAN_POINT('Origin',(72.3260541341287,0.,0.));
#48038=CARTESIAN_POINT('',(58.,12.6476816419096,-135.410620518056));
#48039=CARTESIAN_POINT('Origin',(58.,0.,0.));
#48040=CARTESIAN_POINT('Origin',(72.3260541341288,0.,0.));
#48041=CARTESIAN_POINT('',(57.5,24.895934751199,-133.701878942908));
#48042=CARTESIAN_POINT('',(14.5,24.895934751199,-133.701878942908));
#48043=CARTESIAN_POINT('',(36.,24.895934751199,-133.701878942908));
#48044=CARTESIAN_POINT('',(14.,24.4013666019951,-133.793024137864));
#48045=CARTESIAN_POINT('Origin',(-0.326054134128935,0.,0.));
#48046=CARTESIAN_POINT('',(14.,22.8301251586203,-134.070076397538));
#48047=CARTESIAN_POINT('Origin',(14.,0.,0.));
#48048=CARTESIAN_POINT('',(14.5,22.3342096256953,-134.153580199693));
#48049=CARTESIAN_POINT('Origin',(-0.32605413412921,0.,0.));
#48050=CARTESIAN_POINT('',(57.5,22.3342096256953,-134.153580199693));
#48051=CARTESIAN_POINT('',(36.,22.3342096256953,-134.153580199693));
#48052=CARTESIAN_POINT('',(58.,22.8301251586203,-134.070076397538));
#48053=CARTESIAN_POINT('Origin',(72.326054134129,0.,0.));
#48054=CARTESIAN_POINT('',(58.,24.4013666019951,-133.793024137864));
#48055=CARTESIAN_POINT('Origin',(58.,0.,0.));
#48056=CARTESIAN_POINT('Origin',(72.3260541341287,0.,0.));
#48057=CARTESIAN_POINT('',(57.5,36.4540847692092,-131.023279243191));
#48058=CARTESIAN_POINT('',(14.5,36.4540847692092,-131.023279243191));
#48059=CARTESIAN_POINT('',(36.,36.4540847692092,-131.023279243191));
#48060=CARTESIAN_POINT('',(14.,35.9693424282914,-131.157182057546));
#48061=CARTESIAN_POINT('Origin',(-0.326054134128868,0.,0.));
#48062=CARTESIAN_POINT('',(14.,34.4282267284513,-131.570122764761));
#48063=CARTESIAN_POINT('Origin',(14.,0.,0.));
#48064=CARTESIAN_POINT('',(14.5,33.9414761397492,-131.696530696351));
#48065=CARTESIAN_POINT('Origin',(-0.326054134128984,0.,0.));
#48066=CARTESIAN_POINT('',(57.5,33.9414761397492,-131.696530696351));
#48067=CARTESIAN_POINT('',(36.,33.9414761397492,-131.696530696351));
#48068=CARTESIAN_POINT('',(58.,34.4282267284513,-131.570122764761));
#48069=CARTESIAN_POINT('Origin',(72.3260541341289,0.,0.));
#48070=CARTESIAN_POINT('',(58.,35.9693424282914,-131.157182057546));
#48071=CARTESIAN_POINT('Origin',(58.,0.,0.));
#48072=CARTESIAN_POINT('Origin',(72.3260541341287,0.,0.));
#48073=CARTESIAN_POINT('',(57.5,47.7347971905474,-127.347513274415));
#48074=CARTESIAN_POINT('',(14.5,47.7347971905474,-127.347513274415));
#48075=CARTESIAN_POINT('',(36.,47.7347971905474,-127.347513274415));
#48076=CARTESIAN_POINT('',(14.,47.2635698398257,-127.523154626899));
#48077=CARTESIAN_POINT('Origin',(-0.326054134129454,0.,0.));
#48078=CARTESIAN_POINT('',(14.,45.764308704547,-128.068841053532));
#48079=CARTESIAN_POINT('Origin',(14.,0.,0.));
#48080=CARTESIAN_POINT('',(14.5,45.2904275259558,-128.23719107387));
#48081=CARTESIAN_POINT('Origin',(-0.326054134128611,0.,0.));
#48082=CARTESIAN_POINT('',(57.5,45.2904275259558,-128.23719107387));
#48083=CARTESIAN_POINT('',(36.,45.2904275259558,-128.23719107387));
#48084=CARTESIAN_POINT('',(58.,45.764308704547,-128.068841053532));
#48085=CARTESIAN_POINT('Origin',(72.3260541341288,0.,0.));
#48086=CARTESIAN_POINT('',(58.,47.2635698398257,-127.523154626899));
#48087=CARTESIAN_POINT('Origin',(58.,0.,0.));
#48088=CARTESIAN_POINT('Origin',(72.3260541341294,0.,0.));
#48089=CARTESIAN_POINT('',(57.5,58.652218982207,-122.702555835089));
#48090=CARTESIAN_POINT('',(14.5,58.652218982207,-122.702555835089));
#48091=CARTESIAN_POINT('',(36.,58.652218982207,-122.702555835089));
#48092=CARTESIAN_POINT('',(14.,58.198092946355,-122.918598988955));
#48093=CARTESIAN_POINT('Origin',(-0.326054134128477,0.,0.));
#48094=CARTESIAN_POINT('',(14.,56.752096658156,-123.592878131805));
#48095=CARTESIAN_POINT('Origin',(14.,0.,0.));
#48096=CARTESIAN_POINT('',(14.5,56.2946914115821,-123.801888995583));
#48097=CARTESIAN_POINT('Origin',(-0.326054134128873,0.,0.));
#48098=CARTESIAN_POINT('',(57.5,56.2946914115821,-123.801888995583));
#48099=CARTESIAN_POINT('',(36.,56.2946914115821,-123.801888995583));
#48100=CARTESIAN_POINT('',(58.,56.752096658156,-123.592878131805));
#48101=CARTESIAN_POINT('Origin',(72.3260541341288,0.,0.));
#48102=CARTESIAN_POINT('',(58.,58.198092946355,-122.918598988955));
#48103=CARTESIAN_POINT('Origin',(58.,0.,0.));
#48104=CARTESIAN_POINT('Origin',(72.3260541341284,0.,0.));
#48105=CARTESIAN_POINT('',(57.5,69.1232619722338,-117.12375785603));
#48106=CARTESIAN_POINT('',(14.5,69.1232619722338,-117.12375785603));
#48107=CARTESIAN_POINT('',(36.,69.1232619722338,-117.12375785603));
#48108=CARTESIAN_POINT('',(14.,68.6896934245934,-117.378558592425));
#48109=CARTESIAN_POINT('Origin',(-0.326054134128757,0.,0.));
#48110=CARTESIAN_POINT('',(14.,67.3079668883436,-118.176298780075));
#48111=CARTESIAN_POINT('Origin',(14.,0.,0.));
#48112=CARTESIAN_POINT('',(14.5,66.8705187039021,-118.424379788416));
#48113=CARTESIAN_POINT('Origin',(-0.326054134129086,0.,0.));
#48114=CARTESIAN_POINT('',(57.5,66.8705187039021,-118.424379788416));
#48115=CARTESIAN_POINT('',(36.,66.8705187039021,-118.424379788416));
#48116=CARTESIAN_POINT('',(58.,67.3079668883436,-118.176298780075));
#48117=CARTESIAN_POINT('Origin',(72.326054134129,0.,0.));
#48118=CARTESIAN_POINT('',(58.,68.6896934245934,-117.378558592425));
#48119=CARTESIAN_POINT('Origin',(58.,0.,0.));
#48120=CARTESIAN_POINT('Origin',(72.3260541341287,0.,0.));
#48121=CARTESIAN_POINT('',(57.5,79.0682352008852,-110.653577358427));
#48122=CARTESIAN_POINT('',(14.5,79.0682352008852,-110.653577358427));
#48123=CARTESIAN_POINT('',(36.,79.0682352008852,-110.653577358427));
#48124=CARTESIAN_POINT('',(14.,78.6585238598996,-110.945196489896));
#48125=CARTESIAN_POINT('Origin',(-0.326054134128921,0.,0.));
#48126=CARTESIAN_POINT('',(14.,77.3515828488492,-111.860326437829));
#48127=CARTESIAN_POINT('Origin',(14.,0.,0.));
#48128=CARTESIAN_POINT('',(14.5,76.9374209713624,-112.145589544464));
#48129=CARTESIAN_POINT('Origin',(-0.326054134128895,0.,0.));
#48130=CARTESIAN_POINT('',(57.5,76.9374209713624,-112.145589544464));
#48131=CARTESIAN_POINT('',(36.,76.9374209713624,-112.145589544464));
#48132=CARTESIAN_POINT('',(58.,77.3515828488492,-111.860326437829));
#48133=CARTESIAN_POINT('Origin',(72.3260541341288,0.,0.));
#48134=CARTESIAN_POINT('',(58.,78.6585238598996,-110.945196489896));
#48135=CARTESIAN_POINT('Origin',(58.,0.,0.));
#48136=CARTESIAN_POINT('Origin',(72.3260541341289,0.,0.));
#48137=CARTESIAN_POINT('',(57.5,88.4114514169522,-103.341256322671));
#48138=CARTESIAN_POINT('',(14.5,88.4114514169522,-103.341256322671));
#48139=CARTESIAN_POINT('',(36.,88.4114514169522,-103.341256322671));
#48140=CARTESIAN_POINT('',(14.,88.0287154333169,-103.667474451537));
#48141=CARTESIAN_POINT('Origin',(-0.326054134129112,0.,0.));
#48142=CARTESIAN_POINT('',(14.,86.8065065577125,-104.693029468278));
#48143=CARTESIAN_POINT('Origin',(14.,0.,0.));
#48144=CARTESIAN_POINT('',(14.5,86.4187830091457,-105.01330364872));
#48145=CARTESIAN_POINT('Origin',(-0.326054134129139,0.,0.));
#48146=CARTESIAN_POINT('',(57.5,86.4187830091457,-105.01330364872));
#48147=CARTESIAN_POINT('',(36.,86.4187830091457,-105.01330364872));
#48148=CARTESIAN_POINT('',(58.,86.8065065577126,-104.693029468278));
#48149=CARTESIAN_POINT('Origin',(72.3260541341287,0.,0.));
#48150=CARTESIAN_POINT('',(58.,88.0287154333169,-103.667474451537));
#48151=CARTESIAN_POINT('Origin',(58.,0.,0.));
#48152=CARTESIAN_POINT('Origin',(72.3260541341291,0.,0.));
#48153=CARTESIAN_POINT('',(57.5,97.0818031034422,-95.2424459271415));
#48154=CARTESIAN_POINT('',(14.5,97.0818031034422,-95.2424459271415));
#48155=CARTESIAN_POINT('',(36.,97.0818031034422,-95.2424459271415));
#48156=CARTESIAN_POINT('',(14.,96.7289553290949,-95.6007803364699));
#48157=CARTESIAN_POINT('Origin',(-0.326054134128397,0.,0.));
#48158=CARTESIAN_POINT('',(14.,95.6007803364699,-96.7289553290949));
#48159=CARTESIAN_POINT('Origin',(14.,0.,0.));
#48160=CARTESIAN_POINT('',(14.5,95.2424459271415,-97.0818031034423));
#48161=CARTESIAN_POINT('Origin',(-0.326054134128722,0.,0.));
#48162=CARTESIAN_POINT('',(57.5,95.2424459271415,-97.0818031034423));
#48163=CARTESIAN_POINT('',(36.,95.2424459271415,-97.0818031034423));
#48164=CARTESIAN_POINT('',(58.,95.6007803364699,-96.7289553290949));
#48165=CARTESIAN_POINT('Origin',(72.3260541341287,0.,0.));
#48166=CARTESIAN_POINT('',(58.,96.7289553290949,-95.6007803364699));
#48167=CARTESIAN_POINT('Origin',(58.,0.,0.));
#48168=CARTESIAN_POINT('Origin',(72.3260541341287,0.,0.));
#48169=CARTESIAN_POINT('',(57.5,105.01330364872,-86.4187830091457));
#48170=CARTESIAN_POINT('',(14.5,105.01330364872,-86.4187830091457));
#48171=CARTESIAN_POINT('',(36.,105.01330364872,-86.4187830091457));
#48172=CARTESIAN_POINT('',(14.,104.693029468278,-86.8065065577126));
#48173=CARTESIAN_POINT('Origin',(-0.326054134128375,0.,0.));
#48174=CARTESIAN_POINT('',(14.,103.667474451537,-88.0287154333169));
#48175=CARTESIAN_POINT('Origin',(14.,0.,0.));
#48176=CARTESIAN_POINT('',(14.5,103.34125632267,-88.4114514169522));
#48177=CARTESIAN_POINT('Origin',(-0.326054134128846,0.,0.));
#48178=CARTESIAN_POINT('',(57.5,103.34125632267,-88.4114514169522));
#48179=CARTESIAN_POINT('',(36.,103.34125632267,-88.4114514169522));
#48180=CARTESIAN_POINT('',(58.,103.667474451537,-88.0287154333169));
#48181=CARTESIAN_POINT('Origin',(72.3260541341288,0.,0.));
#48182=CARTESIAN_POINT('',(58.,104.693029468278,-86.8065065577126));
#48183=CARTESIAN_POINT('Origin',(58.,0.,0.));
#48184=CARTESIAN_POINT('Origin',(72.3260541341283,0.,0.));
#48185=CARTESIAN_POINT('',(57.5,112.145589544464,-76.9374209713625));
#48186=CARTESIAN_POINT('',(14.5,112.145589544464,-76.9374209713625));
#48187=CARTESIAN_POINT('',(36.,112.145589544464,-76.9374209713625));
#48188=CARTESIAN_POINT('',(14.,111.860326437829,-77.3515828488493));
#48189=CARTESIAN_POINT('Origin',(-0.32605413412909,0.,0.));
#48190=CARTESIAN_POINT('',(14.,110.945196489896,-78.6585238598997));
#48191=CARTESIAN_POINT('Origin',(14.,0.,0.));
#48192=CARTESIAN_POINT('',(14.5,110.653577358427,-79.0682352008853));
#48193=CARTESIAN_POINT('Origin',(-0.326054134128935,0.,0.));
#48194=CARTESIAN_POINT('',(57.5,110.653577358427,-79.0682352008853));
#48195=CARTESIAN_POINT('',(36.,110.653577358427,-79.0682352008853));
#48196=CARTESIAN_POINT('',(58.,110.945196489896,-78.6585238598997));
#48197=CARTESIAN_POINT('Origin',(72.3260541341289,0.,0.));
#48198=CARTESIAN_POINT('',(58.,111.860326437829,-77.3515828488494));
#48199=CARTESIAN_POINT('Origin',(58.,0.,0.));
#48200=CARTESIAN_POINT('Origin',(72.3260541341286,0.,0.));
#48201=CARTESIAN_POINT('',(57.5,118.424379788416,-66.8705187039023));
#48202=CARTESIAN_POINT('',(14.5,118.424379788416,-66.8705187039023));
#48203=CARTESIAN_POINT('',(36.,118.424379788416,-66.8705187039023));
#48204=CARTESIAN_POINT('',(14.,118.176298780075,-67.3079668883437));
#48205=CARTESIAN_POINT('Origin',(-0.326054134129321,0.,0.));
#48206=CARTESIAN_POINT('',(14.,117.378558592425,-68.6896934245934));
#48207=CARTESIAN_POINT('Origin',(14.,0.,0.));
#48208=CARTESIAN_POINT('',(14.5,117.12375785603,-69.1232619722339));
#48209=CARTESIAN_POINT('Origin',(-0.326054134128744,0.,0.));
#48210=CARTESIAN_POINT('',(57.5,117.12375785603,-69.1232619722339));
#48211=CARTESIAN_POINT('',(36.,117.12375785603,-69.1232619722339));
#48212=CARTESIAN_POINT('',(58.,117.378558592425,-68.6896934245935));
#48213=CARTESIAN_POINT('Origin',(72.3260541341287,0.,0.));
#48214=CARTESIAN_POINT('',(58.,118.176298780075,-67.3079668883437));
#48215=CARTESIAN_POINT('Origin',(58.,0.,0.));
#48216=CARTESIAN_POINT('Origin',(72.3260541341288,0.,0.));
#48217=CARTESIAN_POINT('',(57.5,123.801888995583,-56.2946914115822));
#48218=CARTESIAN_POINT('',(14.5,123.801888995583,-56.2946914115822));
#48219=CARTESIAN_POINT('',(36.,123.801888995583,-56.2946914115822));
#48220=CARTESIAN_POINT('',(14.,123.592878131805,-56.7520966581561));
#48221=CARTESIAN_POINT('Origin',(-0.326054134128881,0.,0.));
#48222=CARTESIAN_POINT('',(14.,122.918598988954,-58.1980929463551));
#48223=CARTESIAN_POINT('Origin',(14.,0.,0.));
#48224=CARTESIAN_POINT('',(14.5,122.702555835089,-58.652218982207));
#48225=CARTESIAN_POINT('Origin',(-0.32605413412873,0.,0.));
#48226=CARTESIAN_POINT('',(57.5,122.702555835089,-58.652218982207));
#48227=CARTESIAN_POINT('',(36.,122.702555835089,-58.652218982207));
#48228=CARTESIAN_POINT('',(58.,122.918598988954,-58.1980929463551));
#48229=CARTESIAN_POINT('Origin',(72.3260541341287,0.,0.));
#48230=CARTESIAN_POINT('',(58.,123.592878131805,-56.7520966581561));
#48231=CARTESIAN_POINT('Origin',(58.,0.,0.));
#48232=CARTESIAN_POINT('Origin',(72.3260541341288,0.,0.));
#48233=CARTESIAN_POINT('',(57.5,128.23719107387,-45.2904275259559));
#48234=CARTESIAN_POINT('',(14.5,128.23719107387,-45.2904275259559));
#48235=CARTESIAN_POINT('',(36.,128.23719107387,-45.2904275259559));
#48236=CARTESIAN_POINT('',(14.,128.068841053532,-45.7643087045471));
#48237=CARTESIAN_POINT('Origin',(-0.326054134128855,0.,0.));
#48238=CARTESIAN_POINT('',(14.,127.523154626899,-47.2635698398257));
#48239=CARTESIAN_POINT('Origin',(14.,0.,0.));
#48240=CARTESIAN_POINT('',(14.5,127.347513274415,-47.7347971905475));
#48241=CARTESIAN_POINT('Origin',(-0.326054134128952,0.,0.));
#48242=CARTESIAN_POINT('',(57.5,127.347513274415,-47.7347971905475));
#48243=CARTESIAN_POINT('',(36.,127.347513274415,-47.7347971905475));
#48244=CARTESIAN_POINT('',(58.,127.523154626899,-47.2635698398257));
#48245=CARTESIAN_POINT('Origin',(72.3260541341289,0.,0.));
#48246=CARTESIAN_POINT('',(58.,128.068841053532,-45.7643087045471));
#48247=CARTESIAN_POINT('Origin',(58.,0.,0.));
#48248=CARTESIAN_POINT('Origin',(72.3260541341288,0.,0.));
#48249=CARTESIAN_POINT('',(57.5,131.696530696351,-33.9414761397491));
#48250=CARTESIAN_POINT('',(14.5,131.696530696351,-33.9414761397491));
#48251=CARTESIAN_POINT('',(36.,131.696530696351,-33.9414761397491));
#48252=CARTESIAN_POINT('',(14.,131.570122764761,-34.4282267284513));
#48253=CARTESIAN_POINT('Origin',(-0.326054134128864,0.,0.));
#48254=CARTESIAN_POINT('',(14.,131.157182057546,-35.9693424282914));
#48255=CARTESIAN_POINT('Origin',(14.,0.,0.));
#48256=CARTESIAN_POINT('',(14.5,131.023279243191,-36.4540847692092));
#48257=CARTESIAN_POINT('Origin',(-0.326054134128739,0.,0.));
#48258=CARTESIAN_POINT('',(57.5,131.023279243191,-36.4540847692092));
#48259=CARTESIAN_POINT('',(36.,131.023279243191,-36.4540847692092));
#48260=CARTESIAN_POINT('',(58.,131.157182057546,-35.9693424282914));
#48261=CARTESIAN_POINT('Origin',(72.3260541341289,0.,0.));
#48262=CARTESIAN_POINT('',(58.,131.570122764761,-34.4282267284513));
#48263=CARTESIAN_POINT('Origin',(58.,0.,0.));
#48264=CARTESIAN_POINT('Origin',(72.3260541341289,0.,0.));
#48265=CARTESIAN_POINT('',(57.5,134.153580199693,-22.3342096256954));
#48266=CARTESIAN_POINT('',(14.5,134.153580199693,-22.3342096256954));
#48267=CARTESIAN_POINT('',(36.,134.153580199693,-22.3342096256954));
#48268=CARTESIAN_POINT('',(14.,134.070076397538,-22.8301251586203));
#48269=CARTESIAN_POINT('Origin',(-0.326054134129072,0.,0.));
#48270=CARTESIAN_POINT('',(14.,133.793024137864,-24.4013666019951));
#48271=CARTESIAN_POINT('Origin',(14.,0.,0.));
#48272=CARTESIAN_POINT('',(14.5,133.701878942908,-24.8959347511991));
#48273=CARTESIAN_POINT('Origin',(-0.326054134128939,0.,0.));
#48274=CARTESIAN_POINT('',(57.5,133.701878942908,-24.8959347511991));
#48275=CARTESIAN_POINT('',(36.,133.701878942908,-24.8959347511991));
#48276=CARTESIAN_POINT('',(58.,133.793024137864,-24.4013666019951));
#48277=CARTESIAN_POINT('Origin',(72.3260541341289,0.,0.));
#48278=CARTESIAN_POINT('',(58.,134.070076397538,-22.8301251586204));
#48279=CARTESIAN_POINT('Origin',(58.,0.,0.));
#48280=CARTESIAN_POINT('Origin',(72.3260541341289,0.,0.));
#48281=CARTESIAN_POINT('',(57.5,135.589639953569,-10.5569662906256));
#48282=CARTESIAN_POINT('',(14.5,135.589639953569,-10.5569662906256));
#48283=CARTESIAN_POINT('',(36.,135.589639953569,-10.5569662906256));
#48284=CARTESIAN_POINT('',(14.,135.549675795204,-11.0582725511259));
#48285=CARTESIAN_POINT('Origin',(-0.32605413412893,0.,0.));
#48286=CARTESIAN_POINT('',(14.,135.410620518056,-12.6476816419096));
#48287=CARTESIAN_POINT('Origin',(14.,0.,0.));
#48288=CARTESIAN_POINT('',(14.5,135.362926612467,-13.1483116371559));
#48289=CARTESIAN_POINT('Origin',(-0.326054134128819,0.,0.));
#48290=CARTESIAN_POINT('',(57.5,135.362926612467,-13.1483116371559));
#48291=CARTESIAN_POINT('',(36.,135.362926612467,-13.1483116371559));
#48292=CARTESIAN_POINT('',(58.,135.410620518056,-12.6476816419096));
#48293=CARTESIAN_POINT('Origin',(72.3260541341288,0.,0.));
#48294=CARTESIAN_POINT('',(58.,135.549675795204,-11.0582725511259));
#48295=CARTESIAN_POINT('Origin',(58.,0.,0.));
#48296=CARTESIAN_POINT('Origin',(72.3260541341289,0.,0.));
#48297=CARTESIAN_POINT('',(57.5,135.993780676136,1.30062193238637));
#48298=CARTESIAN_POINT('',(14.5,135.993780676136,1.30062193238637));
#48299=CARTESIAN_POINT('',(36.,135.993780676136,1.30062193238637));
#48300=CARTESIAN_POINT('',(14.,135.997660312937,0.797740187650231));
#48301=CARTESIAN_POINT('Origin',(-0.326054134128819,0.,0.));
#48302=CARTESIAN_POINT('',(14.,135.997660312937,-0.797740187650278));
#48303=CARTESIAN_POINT('Origin',(14.,0.,0.));
#48304=CARTESIAN_POINT('',(14.5,135.993780676136,-1.30062193238642));
#48305=CARTESIAN_POINT('Origin',(-0.326054134128824,0.,0.));
#48306=CARTESIAN_POINT('',(57.5,135.993780676136,-1.30062193238642));
#48307=CARTESIAN_POINT('',(36.,135.993780676136,-1.30062193238642));
#48308=CARTESIAN_POINT('',(58.,135.997660312937,-0.797740187650278));
#48309=CARTESIAN_POINT('Origin',(72.3260541341288,0.,0.));
#48310=CARTESIAN_POINT('',(58.,135.997660312937,0.797740187650231));
#48311=CARTESIAN_POINT('Origin',(58.,0.,0.));
#48312=CARTESIAN_POINT('Origin',(72.3260541341288,0.,0.));
#48313=CARTESIAN_POINT('',(57.5,135.362926612467,13.1483116371559));
#48314=CARTESIAN_POINT('',(14.5,135.362926612467,13.1483116371559));
#48315=CARTESIAN_POINT('',(36.,135.362926612467,13.1483116371559));
#48316=CARTESIAN_POINT('',(14.,135.410620518056,12.6476816419096));
#48317=CARTESIAN_POINT('Origin',(-0.32605413412881,0.,0.));
#48318=CARTESIAN_POINT('',(14.,135.549675795204,11.0582725511258));
#48319=CARTESIAN_POINT('Origin',(14.,0.,0.));
#48320=CARTESIAN_POINT('',(14.5,135.589639953569,10.5569662906256));
#48321=CARTESIAN_POINT('Origin',(-0.326054134128806,0.,0.));
#48322=CARTESIAN_POINT('',(57.5,135.589639953569,10.5569662906256));
#48323=CARTESIAN_POINT('',(36.,135.589639953569,10.5569662906256));
#48324=CARTESIAN_POINT('',(58.,135.549675795204,11.0582725511258));
#48325=CARTESIAN_POINT('Origin',(72.3260541341288,0.,0.));
#48326=CARTESIAN_POINT('',(58.,135.410620518056,12.6476816419096));
#48327=CARTESIAN_POINT('Origin',(58.,0.,0.));
#48328=CARTESIAN_POINT('Origin',(72.3260541341288,0.,0.));
#48329=CARTESIAN_POINT('',(57.5,133.701878942908,24.895934751199));
#48330=CARTESIAN_POINT('',(14.5,133.701878942908,24.895934751199));
#48331=CARTESIAN_POINT('',(36.,133.701878942908,24.895934751199));
#48332=CARTESIAN_POINT('',(14.,133.793024137864,24.4013666019951));
#48333=CARTESIAN_POINT('Origin',(-0.32605413412893,0.,0.));
#48334=CARTESIAN_POINT('',(14.,134.070076397538,22.8301251586203));
#48335=CARTESIAN_POINT('Origin',(14.,0.,0.));
#48336=CARTESIAN_POINT('',(14.5,134.153580199693,22.3342096256953));
#48337=CARTESIAN_POINT('Origin',(-0.326054134128952,0.,0.));
#48338=CARTESIAN_POINT('',(57.5,134.153580199693,22.3342096256953));
#48339=CARTESIAN_POINT('',(36.,134.153580199693,22.3342096256953));
#48340=CARTESIAN_POINT('',(58.,134.070076397538,22.8301251586203));
#48341=CARTESIAN_POINT('Origin',(72.3260541341289,0.,0.));
#48342=CARTESIAN_POINT('',(58.,133.793024137864,24.4013666019951));
#48343=CARTESIAN_POINT('Origin',(58.,0.,0.));
#48344=CARTESIAN_POINT('Origin',(72.3260541341287,0.,0.));
#48345=CARTESIAN_POINT('',(57.5,131.023279243191,36.4540847692091));
#48346=CARTESIAN_POINT('',(14.5,131.023279243191,36.4540847692091));
#48347=CARTESIAN_POINT('',(36.,131.023279243191,36.4540847692091));
#48348=CARTESIAN_POINT('',(14.,131.157182057546,35.9693424282913));
#48349=CARTESIAN_POINT('Origin',(-0.326054134128735,0.,0.));
#48350=CARTESIAN_POINT('',(14.,131.570122764761,34.4282267284512));
#48351=CARTESIAN_POINT('Origin',(14.,0.,0.));
#48352=CARTESIAN_POINT('',(14.5,131.696530696351,33.9414761397491));
#48353=CARTESIAN_POINT('Origin',(-0.326054134128992,0.,0.));
#48354=CARTESIAN_POINT('',(57.5,131.696530696351,33.9414761397491));
#48355=CARTESIAN_POINT('',(36.,131.696530696351,33.9414761397491));
#48356=CARTESIAN_POINT('',(58.,131.570122764761,34.4282267284512));
#48357=CARTESIAN_POINT('Origin',(72.3260541341289,0.,0.));
#48358=CARTESIAN_POINT('',(58.,131.157182057546,35.9693424282913));
#48359=CARTESIAN_POINT('Origin',(58.,0.,0.));
#48360=CARTESIAN_POINT('Origin',(72.3260541341287,0.,0.));
#48361=CARTESIAN_POINT('',(57.5,127.347513274415,47.7347971905473));
#48362=CARTESIAN_POINT('',(14.5,127.347513274415,47.7347971905473));
#48363=CARTESIAN_POINT('',(36.,127.347513274415,47.7347971905473));
#48364=CARTESIAN_POINT('',(14.,127.523154626899,47.2635698398256));
#48365=CARTESIAN_POINT('Origin',(-0.326054134128948,0.,0.));
#48366=CARTESIAN_POINT('',(14.,128.068841053532,45.7643087045469));
#48367=CARTESIAN_POINT('Origin',(14.,0.,0.));
#48368=CARTESIAN_POINT('',(14.5,128.23719107387,45.2904275259557));
#48369=CARTESIAN_POINT('Origin',(-0.326054134128855,0.,0.));
#48370=CARTESIAN_POINT('',(57.5,128.23719107387,45.2904275259557));
#48371=CARTESIAN_POINT('',(36.,128.23719107387,45.2904275259557));
#48372=CARTESIAN_POINT('',(58.,128.068841053532,45.7643087045469));
#48373=CARTESIAN_POINT('Origin',(72.3260541341288,0.,0.));
#48374=CARTESIAN_POINT('',(58.,127.523154626899,47.2635698398256));
#48375=CARTESIAN_POINT('Origin',(58.,0.,0.));
#48376=CARTESIAN_POINT('Origin',(72.3260541341292,0.,0.));
#48377=CARTESIAN_POINT('',(57.5,122.702555835089,58.6522189822069));
#48378=CARTESIAN_POINT('',(14.5,122.702555835089,58.6522189822069));
#48379=CARTESIAN_POINT('',(36.,122.702555835089,58.6522189822069));
#48380=CARTESIAN_POINT('',(14.,122.918598988955,58.198092946355));
#48381=CARTESIAN_POINT('Origin',(-0.326054134128726,0.,0.));
#48382=CARTESIAN_POINT('',(14.,123.592878131805,56.752096658156));
#48383=CARTESIAN_POINT('Origin',(14.,0.,0.));
#48384=CARTESIAN_POINT('',(14.5,123.801888995583,56.294691411582));
#48385=CARTESIAN_POINT('Origin',(-0.326054134129121,0.,0.));
#48386=CARTESIAN_POINT('',(57.5,123.801888995583,56.294691411582));
#48387=CARTESIAN_POINT('',(36.,123.801888995583,56.294691411582));
#48388=CARTESIAN_POINT('',(58.,123.592878131805,56.752096658156));
#48389=CARTESIAN_POINT('Origin',(72.3260541341291,0.,0.));
#48390=CARTESIAN_POINT('',(58.,122.918598988955,58.198092946355));
#48391=CARTESIAN_POINT('Origin',(58.,0.,0.));
#48392=CARTESIAN_POINT('Origin',(72.3260541341287,0.,0.));
#48393=CARTESIAN_POINT('',(57.5,117.12375785603,69.1232619722339));
#48394=CARTESIAN_POINT('',(14.5,117.12375785603,69.1232619722339));
#48395=CARTESIAN_POINT('',(36.,117.12375785603,69.1232619722339));
#48396=CARTESIAN_POINT('',(14.,117.378558592425,68.6896934245934));
#48397=CARTESIAN_POINT('Origin',(-0.326054134128504,0.,0.));
#48398=CARTESIAN_POINT('',(14.,118.176298780075,67.3079668883437));
#48399=CARTESIAN_POINT('Origin',(14.,0.,0.));
#48400=CARTESIAN_POINT('',(14.5,118.424379788416,66.8705187039022));
#48401=CARTESIAN_POINT('Origin',(-0.326054134128895,0.,0.));
#48402=CARTESIAN_POINT('',(57.5,118.424379788416,66.8705187039022));
#48403=CARTESIAN_POINT('',(36.,118.424379788416,66.8705187039022));
#48404=CARTESIAN_POINT('',(58.,118.176298780075,67.3079668883437));
#48405=CARTESIAN_POINT('Origin',(72.3260541341288,0.,0.));
#48406=CARTESIAN_POINT('',(58.,117.378558592425,68.6896934245934));
#48407=CARTESIAN_POINT('Origin',(58.,0.,0.));
#48408=CARTESIAN_POINT('Origin',(72.3260541341284,0.,0.));
#48409=CARTESIAN_POINT('',(57.5,110.653577358427,79.0682352008853));
#48410=CARTESIAN_POINT('',(14.5,110.653577358427,79.0682352008853));
#48411=CARTESIAN_POINT('',(36.,110.653577358427,79.0682352008853));
#48412=CARTESIAN_POINT('',(14.,110.945196489896,78.6585238598997));
#48413=CARTESIAN_POINT('Origin',(-0.326054134129183,0.,0.));
#48414=CARTESIAN_POINT('',(14.,111.860326437829,77.3515828488493));
#48415=CARTESIAN_POINT('Origin',(14.,0.,0.));
#48416=CARTESIAN_POINT('',(14.5,112.145589544464,76.9374209713625));
#48417=CARTESIAN_POINT('Origin',(-0.326054134128935,0.,0.));
#48418=CARTESIAN_POINT('',(57.5,112.145589544464,76.9374209713625));
#48419=CARTESIAN_POINT('',(36.,112.145589544464,76.9374209713625));
#48420=CARTESIAN_POINT('',(58.,111.860326437829,77.3515828488493));
#48421=CARTESIAN_POINT('Origin',(72.3260541341289,0.,0.));
#48422=CARTESIAN_POINT('',(58.,110.945196489896,78.6585238598997));
#48423=CARTESIAN_POINT('Origin',(58.,0.,0.));
#48424=CARTESIAN_POINT('Origin',(72.3260541341289,0.,0.));
#48425=CARTESIAN_POINT('',(57.5,103.341256322671,88.4114514169522));
#48426=CARTESIAN_POINT('',(14.5,103.341256322671,88.4114514169522));
#48427=CARTESIAN_POINT('',(36.,103.341256322671,88.4114514169522));
#48428=CARTESIAN_POINT('',(14.,103.667474451537,88.0287154333169));
#48429=CARTESIAN_POINT('Origin',(-0.326054134129126,0.,0.));
#48430=CARTESIAN_POINT('',(14.,104.693029468278,86.8065065577125));
#48431=CARTESIAN_POINT('Origin',(14.,0.,0.));
#48432=CARTESIAN_POINT('',(14.5,105.01330364872,86.4187830091457));
#48433=CARTESIAN_POINT('Origin',(-0.32605413412873,0.,0.));
#48434=CARTESIAN_POINT('',(57.5,105.01330364872,86.4187830091457));
#48435=CARTESIAN_POINT('',(36.,105.01330364872,86.4187830091457));
#48436=CARTESIAN_POINT('',(58.,104.693029468278,86.8065065577125));
#48437=CARTESIAN_POINT('Origin',(72.3260541341287,0.,0.));
#48438=CARTESIAN_POINT('',(58.,103.667474451537,88.0287154333169));
#48439=CARTESIAN_POINT('Origin',(58.,0.,0.));
#48440=CARTESIAN_POINT('Origin',(72.3260541341291,0.,0.));
#48441=CARTESIAN_POINT('',(57.5,95.2424459271415,97.0818031034422));
#48442=CARTESIAN_POINT('',(14.5,95.2424459271415,97.0818031034422));
#48443=CARTESIAN_POINT('',(36.,95.2424459271415,97.0818031034422));
#48444=CARTESIAN_POINT('',(14.,95.6007803364699,96.7289553290949));
#48445=CARTESIAN_POINT('Origin',(-0.326054134128722,0.,0.));
#48446=CARTESIAN_POINT('',(14.,96.7289553290949,95.6007803364699));
#48447=CARTESIAN_POINT('Origin',(14.,0.,0.));
#48448=CARTESIAN_POINT('',(14.5,97.0818031034423,95.2424459271415));
#48449=CARTESIAN_POINT('Origin',(-0.326054134128722,0.,0.));
#48450=CARTESIAN_POINT('',(57.5,97.0818031034423,95.2424459271415));
#48451=CARTESIAN_POINT('',(36.,97.0818031034423,95.2424459271415));
#48452=CARTESIAN_POINT('',(58.,96.7289553290949,95.6007803364699));
#48453=CARTESIAN_POINT('Origin',(72.3260541341287,0.,0.));
#48454=CARTESIAN_POINT('',(58.,95.6007803364699,96.7289553290949));
#48455=CARTESIAN_POINT('Origin',(58.,0.,0.));
#48456=CARTESIAN_POINT('Origin',(72.3260541341287,0.,0.));
#48457=CARTESIAN_POINT('',(57.5,86.4187830091458,105.01330364872));
#48458=CARTESIAN_POINT('',(14.5,86.4187830091458,105.01330364872));
#48459=CARTESIAN_POINT('',(36.,86.4187830091458,105.01330364872));
#48460=CARTESIAN_POINT('',(14.,86.8065065577126,104.693029468278));
#48461=CARTESIAN_POINT('Origin',(-0.326054134128388,0.,0.));
#48462=CARTESIAN_POINT('',(14.,88.0287154333169,103.667474451537));
#48463=CARTESIAN_POINT('Origin',(14.,0.,0.));
#48464=CARTESIAN_POINT('',(14.5,88.4114514169523,103.34125632267));
#48465=CARTESIAN_POINT('Origin',(-0.326054134128415,0.,0.));
#48466=CARTESIAN_POINT('',(57.5,88.4114514169523,103.34125632267));
#48467=CARTESIAN_POINT('',(36.,88.4114514169523,103.34125632267));
#48468=CARTESIAN_POINT('',(58.,88.0287154333169,103.667474451537));
#48469=CARTESIAN_POINT('Origin',(72.3260541341291,0.,0.));
#48470=CARTESIAN_POINT('',(58.,86.8065065577126,104.693029468278));
#48471=CARTESIAN_POINT('Origin',(58.,0.,0.));
#48472=CARTESIAN_POINT('Origin',(72.3260541341283,0.,0.));
#48473=CARTESIAN_POINT('',(57.5,76.9374209713625,112.145589544464));
#48474=CARTESIAN_POINT('',(14.5,76.9374209713625,112.145589544464));
#48475=CARTESIAN_POINT('',(36.,76.9374209713625,112.145589544464));
#48476=CARTESIAN_POINT('',(14.,77.3515828488493,111.860326437829));
#48477=CARTESIAN_POINT('Origin',(-0.326054134129108,0.,0.));
#48478=CARTESIAN_POINT('',(14.,78.6585238598997,110.945196489896));
#48479=CARTESIAN_POINT('Origin',(14.,0.,0.));
#48480=CARTESIAN_POINT('',(14.5,79.0682352008854,110.653577358427));
#48481=CARTESIAN_POINT('Origin',(-0.326054134128699,0.,0.));
#48482=CARTESIAN_POINT('',(57.5,79.0682352008854,110.653577358427));
#48483=CARTESIAN_POINT('',(36.,79.0682352008854,110.653577358427));
#48484=CARTESIAN_POINT('',(58.,78.6585238598997,110.945196489896));
#48485=CARTESIAN_POINT('Origin',(72.3260541341286,0.,0.));
#48486=CARTESIAN_POINT('',(58.,77.3515828488494,111.860326437829));
#48487=CARTESIAN_POINT('Origin',(58.,0.,0.));
#48488=CARTESIAN_POINT('Origin',(72.3260541341286,0.,0.));
#48489=CARTESIAN_POINT('',(57.5,66.8705187039023,118.424379788416));
#48490=CARTESIAN_POINT('',(14.5,66.8705187039023,118.424379788416));
#48491=CARTESIAN_POINT('',(36.,66.8705187039023,118.424379788416));
#48492=CARTESIAN_POINT('',(14.,67.3079668883437,118.176298780075));
#48493=CARTESIAN_POINT('Origin',(-0.326054134129325,0.,0.));
#48494=CARTESIAN_POINT('',(14.,68.6896934245934,117.378558592425));
#48495=CARTESIAN_POINT('Origin',(14.,0.,0.));
#48496=CARTESIAN_POINT('',(14.5,69.1232619722339,117.12375785603));
#48497=CARTESIAN_POINT('Origin',(-0.326054134128744,0.,0.));
#48498=CARTESIAN_POINT('',(57.5,69.1232619722339,117.12375785603));
#48499=CARTESIAN_POINT('',(36.,69.1232619722339,117.12375785603));
#48500=CARTESIAN_POINT('',(58.,68.6896934245935,117.378558592425));
#48501=CARTESIAN_POINT('Origin',(72.3260541341287,0.,0.));
#48502=CARTESIAN_POINT('',(58.,67.3079668883437,118.176298780075));
#48503=CARTESIAN_POINT('Origin',(58.,0.,0.));
#48504=CARTESIAN_POINT('Origin',(72.3260541341288,0.,0.));
#48505=CARTESIAN_POINT('',(57.5,56.2946914115822,123.801888995583));
#48506=CARTESIAN_POINT('',(14.5,56.2946914115822,123.801888995583));
#48507=CARTESIAN_POINT('',(36.,56.2946914115822,123.801888995583));
#48508=CARTESIAN_POINT('',(14.,56.7520966581561,123.592878131805));
#48509=CARTESIAN_POINT('Origin',(-0.326054134128895,0.,0.));
#48510=CARTESIAN_POINT('',(14.,58.1980929463551,122.918598988954));
#48511=CARTESIAN_POINT('Origin',(14.,0.,0.));
#48512=CARTESIAN_POINT('',(14.5,58.652218982207,122.702555835089));
#48513=CARTESIAN_POINT('Origin',(-0.326054134128717,0.,0.));
#48514=CARTESIAN_POINT('',(57.5,58.652218982207,122.702555835089));
#48515=CARTESIAN_POINT('',(36.,58.652218982207,122.702555835089));
#48516=CARTESIAN_POINT('',(58.,58.1980929463551,122.918598988954));
#48517=CARTESIAN_POINT('Origin',(72.3260541341287,0.,0.));
#48518=CARTESIAN_POINT('',(58.,56.7520966581561,123.592878131805));
#48519=CARTESIAN_POINT('Origin',(58.,0.,0.));
#48520=CARTESIAN_POINT('Origin',(72.3260541341288,0.,0.));
#48521=CARTESIAN_POINT('',(57.5,45.2904275259559,128.23719107387));
#48522=CARTESIAN_POINT('',(14.5,45.2904275259559,128.23719107387));
#48523=CARTESIAN_POINT('',(36.,45.2904275259559,128.23719107387));
#48524=CARTESIAN_POINT('',(14.,45.7643087045471,128.068841053532));
#48525=CARTESIAN_POINT('Origin',(-0.326054134129072,0.,0.));
#48526=CARTESIAN_POINT('',(14.,47.2635698398257,127.523154626899));
#48527=CARTESIAN_POINT('Origin',(14.,0.,0.));
#48528=CARTESIAN_POINT('',(14.5,47.7347971905475,127.347513274415));
#48529=CARTESIAN_POINT('Origin',(-0.326054134129192,0.,0.));
#48530=CARTESIAN_POINT('',(57.5,47.7347971905475,127.347513274415));
#48531=CARTESIAN_POINT('',(36.,47.7347971905475,127.347513274415));
#48532=CARTESIAN_POINT('',(58.,47.2635698398257,127.523154626899));
#48533=CARTESIAN_POINT('Origin',(72.3260541341288,0.,0.));
#48534=CARTESIAN_POINT('',(58.,45.7643087045471,128.068841053532));
#48535=CARTESIAN_POINT('Origin',(58.,0.,0.));
#48536=CARTESIAN_POINT('Origin',(72.326054134129,0.,0.));
#48537=CARTESIAN_POINT('',(57.5,33.9414761397491,131.696530696351));
#48538=CARTESIAN_POINT('',(14.5,33.9414761397491,131.696530696351));
#48539=CARTESIAN_POINT('',(36.,33.9414761397491,131.696530696351));
#48540=CARTESIAN_POINT('',(14.,34.4282267284513,131.570122764761));
#48541=CARTESIAN_POINT('Origin',(-0.326054134128975,0.,0.));
#48542=CARTESIAN_POINT('',(14.,35.9693424282914,131.157182057546));
#48543=CARTESIAN_POINT('Origin',(14.,0.,0.));
#48544=CARTESIAN_POINT('',(14.5,36.4540847692092,131.023279243191));
#48545=CARTESIAN_POINT('Origin',(-0.326054134128868,0.,0.));
#48546=CARTESIAN_POINT('',(57.5,36.4540847692092,131.023279243191));
#48547=CARTESIAN_POINT('',(36.,36.4540847692092,131.023279243191));
#48548=CARTESIAN_POINT('',(58.,35.9693424282914,131.157182057546));
#48549=CARTESIAN_POINT('Origin',(72.3260541341288,0.,0.));
#48550=CARTESIAN_POINT('',(58.,34.4282267284513,131.570122764761));
#48551=CARTESIAN_POINT('Origin',(58.,0.,0.));
#48552=CARTESIAN_POINT('Origin',(72.3260541341289,0.,0.));
#48553=CARTESIAN_POINT('',(57.5,22.3342096256954,134.153580199693));
#48554=CARTESIAN_POINT('',(14.5,22.3342096256954,134.153580199693));
#48555=CARTESIAN_POINT('',(36.,22.3342096256954,134.153580199693));
#48556=CARTESIAN_POINT('',(14.,22.8301251586204,134.070076397538));
#48557=CARTESIAN_POINT('Origin',(-0.326054134129081,0.,0.));
#48558=CARTESIAN_POINT('',(14.,24.4013666019951,133.793024137864));
#48559=CARTESIAN_POINT('Origin',(14.,0.,0.));
#48560=CARTESIAN_POINT('',(14.5,24.8959347511991,133.701878942908));
#48561=CARTESIAN_POINT('Origin',(-0.326054134128939,0.,0.));
#48562=CARTESIAN_POINT('',(57.5,24.8959347511991,133.701878942908));
#48563=CARTESIAN_POINT('',(36.,24.8959347511991,133.701878942908));
#48564=CARTESIAN_POINT('',(58.,24.4013666019951,133.793024137864));
#48565=CARTESIAN_POINT('Origin',(72.3260541341289,0.,0.));
#48566=CARTESIAN_POINT('',(58.,22.8301251586204,134.070076397538));
#48567=CARTESIAN_POINT('Origin',(58.,0.,0.));
#48568=CARTESIAN_POINT('Origin',(72.3260541341289,0.,0.));
#48569=CARTESIAN_POINT('',(57.5,10.5569662906256,135.589639953569));
#48570=CARTESIAN_POINT('',(14.5,10.5569662906256,135.589639953569));
#48571=CARTESIAN_POINT('',(36.,10.5569662906256,135.589639953569));
#48572=CARTESIAN_POINT('',(14.,11.0582725511259,135.549675795204));
#48573=CARTESIAN_POINT('Origin',(-0.326054134128935,0.,0.));
#48574=CARTESIAN_POINT('',(14.,12.6476816419097,135.410620518056));
#48575=CARTESIAN_POINT('Origin',(14.,0.,0.));
#48576=CARTESIAN_POINT('',(14.5,13.1483116371559,135.362926612467));
#48577=CARTESIAN_POINT('Origin',(-0.32605413412881,0.,0.));
#48578=CARTESIAN_POINT('',(57.5,13.1483116371559,135.362926612467));
#48579=CARTESIAN_POINT('',(36.,13.1483116371559,135.362926612467));
#48580=CARTESIAN_POINT('',(58.,12.6476816419097,135.410620518056));
#48581=CARTESIAN_POINT('Origin',(72.3260541341288,0.,0.));
#48582=CARTESIAN_POINT('',(58.,11.0582725511259,135.549675795204));
#48583=CARTESIAN_POINT('Origin',(58.,0.,0.));
#48584=CARTESIAN_POINT('Origin',(72.3260541341289,0.,0.));
#48585=CARTESIAN_POINT('Origin',(79.75,0.,0.));
#48586=CARTESIAN_POINT('',(80.,-39.531555373985,-33.0076677412016));
#48587=CARTESIAN_POINT('',(80.,-51.3831204224764,3.46769889830224));
#48588=CARTESIAN_POINT('Origin',(80.,0.,0.));
#48589=CARTESIAN_POINT('',(79.5,-51.9213615157264,2.85870921103307));
#48590=CARTESIAN_POINT('Ctrl Pts',(80.,-51.3831204224764,3.46769889830225));
#48591=CARTESIAN_POINT('Ctrl Pts',(79.8355728101073,-51.5617816321932,3.26232634574879));
#48592=CARTESIAN_POINT('Ctrl Pts',(79.6687511538102,-51.7413105700118,3.05929982841873));
#48593=CARTESIAN_POINT('Ctrl Pts',(79.5,-51.9213615157264,2.85870921103307));
#48594=CARTESIAN_POINT('',(79.5,-40.3249567224702,-32.8313549115919));
#48595=CARTESIAN_POINT('Origin',(79.5,0.,0.));
#48596=CARTESIAN_POINT('Ctrl Pts',(80.,-39.5315553739849,-33.0076677412016));
#48597=CARTESIAN_POINT('Ctrl Pts',(79.8355728101073,-39.7968102864981,-32.946532280236));
#48598=CARTESIAN_POINT('Ctrl Pts',(79.6687511538101,-40.0613882408863,-32.8878048394167));
#48599=CARTESIAN_POINT('Ctrl Pts',(79.5,-40.3249567224702,-32.8313549115919));
#48600=CARTESIAN_POINT('Origin',(79.75,-54.352879906268,17.6603212285283));
#48601=CARTESIAN_POINT('',(80.,-43.6080799176108,27.396813060998));
#48602=CARTESIAN_POINT('Origin',(80.,-54.352879906268,17.6603212285283));
#48603=CARTESIAN_POINT('',(79.5,-43.6855709521459,28.205866244188));
#48604=CARTESIAN_POINT('Ctrl Pts',(80.,-43.6080799176108,27.396813060998));
#48605=CARTESIAN_POINT('Ctrl Pts',(79.8355728101073,-43.6319049148906,27.6679773704202));
#48606=CARTESIAN_POINT('Ctrl Pts',(79.6687511538101,-43.6578108838571,27.9377537352586));
#48607=CARTESIAN_POINT('Ctrl Pts',(79.5,-43.6855709521459,28.205866244188));
#48608=CARTESIAN_POINT('Origin',(79.5,-54.352879906268,17.6603212285283));
#48609=CARTESIAN_POINT('Origin',(79.75,0.,0.));
#48610=CARTESIAN_POINT('',(80.,-12.5802798007798,49.9398293963255));
#48611=CARTESIAN_POINT('Origin',(80.,0.,0.));
#48612=CARTESIAN_POINT('',(79.5,-13.3257890560989,50.2635389326334));
#48613=CARTESIAN_POINT('Ctrl Pts',(80.,-12.5802798007798,49.9398293963255));
#48614=CARTESIAN_POINT('Ctrl Pts',(79.8355728101072,-12.8308100551922,50.0462826951187));
#48615=CARTESIAN_POINT('Ctrl Pts',(79.6687511538099,-13.0793772402478,50.1542862171309));
#48616=CARTESIAN_POINT('Ctrl Pts',(79.5,-13.3257890560989,50.2635389326334));
#48617=CARTESIAN_POINT('Origin',(79.5,0.,0.));
#48618=CARTESIAN_POINT('Origin',(79.75,3.49942822856356E-15,57.15));
#48619=CARTESIAN_POINT('',(80.,12.5802798007798,49.9398293963255));
#48620=CARTESIAN_POINT('Origin',(80.,3.49942822856356E-15,57.15));
#48621=CARTESIAN_POINT('',(79.5,13.3257890560989,50.2635389326334));
#48622=CARTESIAN_POINT('Ctrl Pts',(80.,12.5802798007798,49.9398293963255));
#48623=CARTESIAN_POINT('Ctrl Pts',(79.8355728101074,12.8308100551919,50.0462826951186));
#48624=CARTESIAN_POINT('Ctrl Pts',(79.6687511538103,13.0793772402473,50.1542862171307));
#48625=CARTESIAN_POINT('Ctrl Pts',(79.5,13.3257890560989,50.2635389326334));
#48626=CARTESIAN_POINT('Origin',(79.5,3.49942822856356E-15,57.15));
#48627=CARTESIAN_POINT('Origin',(79.75,0.,0.));
#48628=CARTESIAN_POINT('',(80.,43.6080799176108,27.396813060998));
#48629=CARTESIAN_POINT('Origin',(80.,0.,0.));
#48630=CARTESIAN_POINT('',(79.5,43.6855709521459,28.205866244188));
#48631=CARTESIAN_POINT('Ctrl Pts',(80.,43.6080799176108,27.396813060998));
#48632=CARTESIAN_POINT('Ctrl Pts',(79.8355728101071,43.6319049148907,27.6679773704205));
#48633=CARTESIAN_POINT('Ctrl Pts',(79.6687511538098,43.6578108838571,27.9377537352591));
#48634=CARTESIAN_POINT('Ctrl Pts',(79.5,43.6855709521459,28.205866244188));
#48635=CARTESIAN_POINT('Origin',(79.5,0.,0.));
#48636=CARTESIAN_POINT('Origin',(79.75,54.352879906268,17.6603212285282));
#48637=CARTESIAN_POINT('',(80.,51.3831204224764,3.46769889830222));
#48638=CARTESIAN_POINT('Origin',(80.,54.352879906268,17.6603212285282));
#48639=CARTESIAN_POINT('',(79.5,51.9213615157264,2.85870921103304));
#48640=CARTESIAN_POINT('Ctrl Pts',(80.,51.3831204224764,3.46769889830223));
#48641=CARTESIAN_POINT('Ctrl Pts',(79.8355728101072,51.5617816321933,3.26232634574865));
#48642=CARTESIAN_POINT('Ctrl Pts',(79.66875115381,51.741310570012,3.05929982841845));
#48643=CARTESIAN_POINT('Ctrl Pts',(79.5,51.9213615157264,2.85870921103305));
#48644=CARTESIAN_POINT('Origin',(79.5,54.352879906268,17.6603212285282));
#48645=CARTESIAN_POINT('Origin',(79.75,0.,0.));
#48646=CARTESIAN_POINT('',(79.5,40.3249567224702,-32.8313549115919));
#48647=CARTESIAN_POINT('Origin',(79.5,0.,0.));
#48648=CARTESIAN_POINT('',(80.,39.5315553739849,-33.0076677412016));
#48649=CARTESIAN_POINT('Origin',(80.,0.,0.));
#48650=CARTESIAN_POINT('Ctrl Pts',(80.,39.5315553739849,-33.0076677412016));
#48651=CARTESIAN_POINT('Ctrl Pts',(79.8355728101073,39.796810286498,-32.946532280236));
#48652=CARTESIAN_POINT('Ctrl Pts',(79.6687511538102,40.0613882408862,-32.8878048394167));
#48653=CARTESIAN_POINT('Ctrl Pts',(79.5,40.3249567224702,-32.8313549115919));
#48654=CARTESIAN_POINT('Origin',(79.75,33.5919271685148,-46.2353212285282));
#48655=CARTESIAN_POINT('',(79.5,18.7633771027908,-48.4967594762626));
#48656=CARTESIAN_POINT('Origin',(79.5,33.5919271685148,-46.2353212285282));
#48657=CARTESIAN_POINT('',(80.,19.1762350683395,-47.7966736144241));
#48658=CARTESIAN_POINT('Origin',(80.,33.5919271685148,-46.2353212285282));
#48659=CARTESIAN_POINT('Ctrl Pts',(80.,19.1762350683395,-47.7966736144241));
#48660=CARTESIAN_POINT('Ctrl Pts',(79.8355728101073,19.0361235140034,-48.0300541310517));
#48661=CARTESIAN_POINT('Ctrl Pts',(79.6687511538101,18.8985113144839,-48.2635349413914));
#48662=CARTESIAN_POINT('Ctrl Pts',(79.5,18.7633771027908,-48.4967594762626));
#48663=CARTESIAN_POINT('Origin',(79.75,0.,0.));
#48664=CARTESIAN_POINT('',(79.5,-18.7633771027908,-48.4967594762626));
#48665=CARTESIAN_POINT('Origin',(79.5,0.,0.));
#48666=CARTESIAN_POINT('',(80.,-19.1762350683395,-47.7966736144241));
#48667=CARTESIAN_POINT('Origin',(80.,0.,0.));
#48668=CARTESIAN_POINT('Ctrl Pts',(80.,-19.1762350683395,-47.7966736144241));
#48669=CARTESIAN_POINT('Ctrl Pts',(79.8355728101073,-19.0361235140034,-48.0300541310517));
#48670=CARTESIAN_POINT('Ctrl Pts',(79.66875115381,-18.8985113144839,-48.2635349413915));
#48671=CARTESIAN_POINT('Ctrl Pts',(79.5,-18.7633771027908,-48.4967594762626));
#48672=CARTESIAN_POINT('Origin',(79.75,-33.5919271685148,-46.2353212285282));
#48673=CARTESIAN_POINT('Origin',(79.5,-33.5919271685148,-46.2353212285282));
#48674=CARTESIAN_POINT('Origin',(80.,-33.5919271685148,-46.2353212285282));
#48675=CARTESIAN_POINT('Origin',(72.,54.352879906268,17.6603212285282));
#48676=CARTESIAN_POINT('',(72.,51.9213615157264,2.85870921103304));
#48677=CARTESIAN_POINT('',(72.,51.9213615157264,2.85870921103304));
#48678=CARTESIAN_POINT('',(72.,43.6855709521459,28.205866244188));
#48679=CARTESIAN_POINT('Origin',(72.,54.352879906268,17.6603212285282));
#48680=CARTESIAN_POINT('',(72.,43.6855709521459,28.205866244188));
#48681=CARTESIAN_POINT('Origin',(72.,0.,0.));
#48682=CARTESIAN_POINT('',(72.,40.3249567224702,-32.8313549115919));
#48683=CARTESIAN_POINT('',(72.,40.3249567224702,-32.8313549115919));
#48684=CARTESIAN_POINT('Origin',(72.,0.,0.));
#48685=CARTESIAN_POINT('Origin',(72.,33.5919271685148,-46.2353212285282));
#48686=CARTESIAN_POINT('',(72.,18.7633771027908,-48.4967594762626));
#48687=CARTESIAN_POINT('',(72.,18.7633771027908,-48.4967594762626));
#48688=CARTESIAN_POINT('Origin',(72.,33.5919271685148,-46.2353212285282));
#48689=CARTESIAN_POINT('Origin',(72.,0.,0.));
#48690=CARTESIAN_POINT('',(72.,-18.7633771027908,-48.4967594762626));
#48691=CARTESIAN_POINT('',(72.,-18.7633771027908,-48.4967594762626));
#48692=CARTESIAN_POINT('Origin',(72.,0.,0.));
#48693=CARTESIAN_POINT('Origin',(72.,-33.5919271685148,-46.2353212285282));
#48694=CARTESIAN_POINT('',(72.,-40.3249567224702,-32.8313549115919));
#48695=CARTESIAN_POINT('',(72.,-40.3249567224702,-32.8313549115919));
#48696=CARTESIAN_POINT('Origin',(72.,-33.5919271685148,-46.2353212285282));
#48697=CARTESIAN_POINT('Origin',(72.,0.,0.));
#48698=CARTESIAN_POINT('',(72.,-51.9213615157264,2.85870921103307));
#48699=CARTESIAN_POINT('',(72.,-51.9213615157264,2.85870921103307));
#48700=CARTESIAN_POINT('Origin',(72.,0.,0.));
#48701=CARTESIAN_POINT('Origin',(80.,0.,5.45733938573587));
#48702=CARTESIAN_POINT('',(80.,33.5919271685148,-39.0553212285282));
#48703=CARTESIAN_POINT('Origin',(80.,33.5919271685148,-46.2353212285282));
#48704=CARTESIAN_POINT('',(80.,-33.5919271685148,-39.0553212285282));
#48705=CARTESIAN_POINT('Origin',(80.,-33.5919271685148,-46.2353212285282));
#48706=CARTESIAN_POINT('',(80.,-54.352879906268,24.8403212285282));
#48707=CARTESIAN_POINT('Origin',(80.,-54.352879906268,17.6603212285283));
#48708=CARTESIAN_POINT('',(80.,2.62013182677576E-15,64.33));
#48709=CARTESIAN_POINT('Origin',(80.,3.49942822856356E-15,57.15));
#48710=CARTESIAN_POINT('',(80.,54.352879906268,24.8403212285282));
#48711=CARTESIAN_POINT('Origin',(80.,54.352879906268,17.6603212285282));
#48712=CARTESIAN_POINT('Origin',(57.75,1.0453001083881,136.034530010839));
#48713=CARTESIAN_POINT('',(57.7487592975525,0.77487592975525,138.751240702447));
#48714=CARTESIAN_POINT('',(58.,0.547506218943957,138.5));
#48715=CARTESIAN_POINT('',(58.2319907935076,0.337557436295053,138.268009206492));
#48716=CARTESIAN_POINT('',(58.,0.7965408108356,136.009654081084));
#48717=CARTESIAN_POINT('',(57.5,1.0497518595105,138.502481404895));
#48718=CARTESIAN_POINT('',(57.5,1.29405940594059,136.059405940594));
#48719=CARTESIAN_POINT('',(50.4896657310026,8.79608403300078,131.492147135898));
#48720=CARTESIAN_POINT('Origin',(58.,0.,137.));
#48721=CARTESIAN_POINT('',(58.,-0.547506218943957,138.5));
#48722=CARTESIAN_POINT('',(58.,0.5,138.5));
#48723=CARTESIAN_POINT('',(58.,-0.596540810835601,138.009654081084));
#48724=CARTESIAN_POINT('Origin',(57.75,0.5,138.75));
#48725=CARTESIAN_POINT('',(57.5,0.499999999999999,139.));
#48726=CARTESIAN_POINT('',(57.5,0.499999999999999,139.));
#48727=CARTESIAN_POINT('',(57.5,-0.500000000000002,139.));
#48728=CARTESIAN_POINT('',(57.5,0.5,139.));
#48729=CARTESIAN_POINT('',(57.5,-0.500000000000002,139.));
#48730=CARTESIAN_POINT('Origin',(14.,0.774875929755249,138.751240702448));
#48731=CARTESIAN_POINT('',(14.5,1.0497518595105,138.502481404895));
#48732=CARTESIAN_POINT('',(14.,1.0497518595105,138.502481404895));
#48733=CARTESIAN_POINT('',(14.5,0.499999999999999,139.));
#48734=CARTESIAN_POINT('',(14.5,1.0497518595105,138.502481404895));
#48735=CARTESIAN_POINT('',(14.,0.499999999999999,139.));
#48736=CARTESIAN_POINT('Origin',(57.5,-1.0497518595105,138.502481404895));
#48737=CARTESIAN_POINT('',(57.5,-1.0497518595105,138.502481404895));
#48738=CARTESIAN_POINT('',(57.5,-1.0497518595105,138.502481404895));
#48739=CARTESIAN_POINT('',(58.,-0.547506218943957,138.5));
#48740=CARTESIAN_POINT('Origin',(14.,0.547506218943958,138.5));
#48741=CARTESIAN_POINT('',(14.,0.547506218943958,138.5));
#48742=CARTESIAN_POINT('',(14.,0.547506218943958,138.5));
#48743=CARTESIAN_POINT('',(14.5,0.499999999999999,139.));
#48744=CARTESIAN_POINT('Origin',(14.25,1.0453001083881,136.034530010839));
#48745=CARTESIAN_POINT('',(14.,0.7965408108356,136.009654081084));
#48746=CARTESIAN_POINT('',(14.5,1.29405940594059,136.059405940594));
#48747=CARTESIAN_POINT('Origin',(14.5,-1.0497518595105,138.502481404895));
#48748=CARTESIAN_POINT('',(14.,-0.547506218943957,138.5));
#48749=CARTESIAN_POINT('',(14.5,-0.500000000000002,139.));
#48750=CARTESIAN_POINT('',(14.,-0.547506218943957,138.5));
#48751=CARTESIAN_POINT('',(14.5,-1.0497518595105,138.502481404895));
#48752=CARTESIAN_POINT('',(14.5,-1.0497518595105,138.502481404895));
#48753=CARTESIAN_POINT('',(14.5,-0.500000000000002,139.));
#48754=CARTESIAN_POINT('Origin',(14.25,-0.845300108388097,138.034530010839));
#48755=CARTESIAN_POINT('',(14.5,-1.09405940594059,138.059405940594));
#48756=CARTESIAN_POINT('',(14.,-0.5965408108356,138.009654081084));
#48757=CARTESIAN_POINT('Origin',(14.,-0.774875929755251,138.751240702447));
#48758=CARTESIAN_POINT('',(14.,-0.500000000000002,139.));
#48759=CARTESIAN_POINT('',(14.,-1.0497518595105,138.502481404895));
#48760=CARTESIAN_POINT('Origin',(14.25,0.5,138.75));
#48761=CARTESIAN_POINT('',(14.5,0.5,139.));
#48762=CARTESIAN_POINT('',(14.,0.5,138.5));
#48763=CARTESIAN_POINT('Origin',(57.75,-0.845300108388097,138.034530010839));
#48764=CARTESIAN_POINT('',(57.5,-1.09405940594059,138.059405940594));
#48765=CARTESIAN_POINT('Origin',(14.,1.4,135.));
#48766=CARTESIAN_POINT('Origin',(14.,1.,139.));
#48767=CARTESIAN_POINT('Origin',(57.5,-11.6165508928786,138.514640906126));
#48768=CARTESIAN_POINT('',(57.5,-11.025529402481,138.066929551123));
#48769=CARTESIAN_POINT('',(58.,-11.5256475780664,138.020683996878));
#48770=CARTESIAN_POINT('',(57.5,-11.025529402481,138.066929551123));
#48771=CARTESIAN_POINT('',(57.5,-11.6165508928786,138.514640906126));
#48772=CARTESIAN_POINT('',(57.5,-11.6165508928786,138.514640906126));
#48773=CARTESIAN_POINT('',(58.,-11.5256475780664,138.020683996878));
#48774=CARTESIAN_POINT('Origin',(57.5,-13.1170438759936,137.883945745091));
#48775=CARTESIAN_POINT('',(57.5,-12.6127455909704,138.427485163379));
#48776=CARTESIAN_POINT('',(58.,-12.6164931630349,137.925247374536));
#48777=CARTESIAN_POINT('',(57.5,-12.6127455909704,138.427485163379));
#48778=CARTESIAN_POINT('',(57.5,-13.1170438759936,137.883945745091));
#48779=CARTESIAN_POINT('',(57.5,-13.1170438759936,137.883945745091));
#48780=CARTESIAN_POINT('',(58.,-12.6164931630349,137.925247374536));
#48781=CARTESIAN_POINT('Origin',(14.,-11.5256475780664,138.020683996878));
#48782=CARTESIAN_POINT('',(14.5,-11.025529402481,138.066929551123));
#48783=CARTESIAN_POINT('',(14.5,-11.6165508928786,138.514640906126));
#48784=CARTESIAN_POINT('',(14.5,-11.025529402481,138.066929551123));
#48785=CARTESIAN_POINT('',(14.,-11.5256475780664,138.020683996878));
#48786=CARTESIAN_POINT('',(14.,-11.5256475780664,138.020683996878));
#48787=CARTESIAN_POINT('',(14.5,-11.6165508928786,138.514640906126));
#48788=CARTESIAN_POINT('Origin',(14.25,-10.8148680765323,135.607981461541));
#48789=CARTESIAN_POINT('',(14.,-11.0605126897208,135.561519390865));
#48790=CARTESIAN_POINT('',(14.5,-10.5692234633438,135.654443532217));
#48791=CARTESIAN_POINT('Origin',(14.5,-13.1170438759936,137.883945745091));
#48792=CARTESIAN_POINT('',(14.,-12.6164931630349,137.925247374536));
#48793=CARTESIAN_POINT('',(14.5,-12.6127455909704,138.427485163379));
#48794=CARTESIAN_POINT('',(14.,-12.6164931630349,137.925247374536));
#48795=CARTESIAN_POINT('',(14.5,-13.1170438759936,137.883945745091));
#48796=CARTESIAN_POINT('',(14.5,-13.1170438759936,137.883945745091));
#48797=CARTESIAN_POINT('',(14.5,-12.6127455909704,138.427485163379));
#48798=CARTESIAN_POINT('Origin',(14.25,-12.8725854741912,137.435594191592));
#48799=CARTESIAN_POINT('',(14.5,-13.1225662476484,137.438694659581));
#48800=CARTESIAN_POINT('',(14.,-12.622604700734,137.432493723604));
#48801=CARTESIAN_POINT('Origin',(14.,-12.864894733482,138.155715454235));
#48802=CARTESIAN_POINT('',(14.,-12.6127455909704,138.427485163379));
#48803=CARTESIAN_POINT('',(14.,-13.1170438759936,137.883945745091));
#48804=CARTESIAN_POINT('Origin',(14.25,-11.5947619571917,138.265592231604));
#48805=CARTESIAN_POINT('',(14.5,-11.6165508928786,138.514640906126));
#48806=CARTESIAN_POINT('',(14.,-11.5729730215048,138.016543557081));
#48807=CARTESIAN_POINT('Origin',(14.,-11.3210401476798,138.290785228625));
#48808=CARTESIAN_POINT('',(14.,-11.025529402481,138.066929551123));
#48809=CARTESIAN_POINT('',(14.,-11.6165508928786,138.514640906126));
#48810=CARTESIAN_POINT('Origin',(57.75,-12.8725854741912,137.435594191592));
#48811=CARTESIAN_POINT('',(58.,-12.622604700734,137.432493723604));
#48812=CARTESIAN_POINT('',(57.5,-13.1225662476484,137.438694659581));
#48813=CARTESIAN_POINT('Origin',(57.75,-11.5947619571917,138.265592231604));
#48814=CARTESIAN_POINT('',(58.,-11.5729730215048,138.016543557081));
#48815=CARTESIAN_POINT('',(57.5,-11.6165508928786,138.514640906126));
#48816=CARTESIAN_POINT('Origin',(57.75,-10.8148680765323,135.607981461541));
#48817=CARTESIAN_POINT('',(57.5,-10.5692234633438,135.654443532217));
#48818=CARTESIAN_POINT('',(58.,-11.0605126897208,135.561519390865));
#48819=CARTESIAN_POINT('Origin',(14.,-11.9403367564292,136.478673638569));
#48820=CARTESIAN_POINT('Origin',(14.,-10.3713526936054,134.608302282232));
#48821=CARTESIAN_POINT('Origin',(14.,-11.1184535438327,138.5582187775));
#48822=CARTESIAN_POINT('Origin',(57.5,-25.0845072682928,136.216030001563));
#48823=CARTESIAN_POINT('',(57.5,-24.6295005722094,136.801453579863));
#48824=CARTESIAN_POINT('',(58.,-24.5894609761083,136.30080033501));
#48825=CARTESIAN_POINT('',(57.5,-24.6295005722094,136.801453579863));
#48826=CARTESIAN_POINT('',(57.5,-25.0845072682928,136.216030001563));
#48827=CARTESIAN_POINT('',(57.5,-25.0845072682928,136.216030001563));
#48828=CARTESIAN_POINT('',(58.,-24.5894609761083,136.30080033501));
#48829=CARTESIAN_POINT('Origin',(14.,-24.8570039202511,136.508741790713));
#48830=CARTESIAN_POINT('',(14.2512407024475,-24.8570039202511,136.508741790713));
#48831=CARTESIAN_POINT('',(14.5,-25.0845072682928,136.216030001563));
#48832=CARTESIAN_POINT('',(14.3353834448874,-24.9339568454557,136.409732133885));
#48833=CARTESIAN_POINT('',(14.,-25.0845072682928,136.216030001563));
#48834=CARTESIAN_POINT('',(14.5,-24.6295005722094,136.801453579863));
#48835=CARTESIAN_POINT('',(14.,-24.6295005722094,136.801453579863));
#48836=CARTESIAN_POINT('',(14.4305329766294,-24.693031787126,136.719712648378));
#48837=CARTESIAN_POINT('Origin',(57.75,-24.801902691856,135.790690514667));
#48838=CARTESIAN_POINT('',(58.,-24.5526029471227,135.809389104878));
#48839=CARTESIAN_POINT('',(57.5,-25.0512024365894,135.771991924456));
#48840=CARTESIAN_POINT('Origin',(57.5,-23.6446928191972,136.97510175753));
#48841=CARTESIAN_POINT('',(57.5,-23.016899728323,136.580604996376));
#48842=CARTESIAN_POINT('',(58.,-23.5110842376314,136.490947249372));
#48843=CARTESIAN_POINT('',(57.5,-23.016899728323,136.580604996376));
#48844=CARTESIAN_POINT('',(57.5,-23.6446928191972,136.97510175753));
#48845=CARTESIAN_POINT('',(57.5,-23.6446928191972,136.97510175753));
#48846=CARTESIAN_POINT('',(58.,-23.5110842376314,136.490947249372));
#48847=CARTESIAN_POINT('Origin',(14.,-23.3307962737601,136.777853376953));
#48848=CARTESIAN_POINT('',(14.2512407024475,-23.3307962737601,136.777853376953));
#48849=CARTESIAN_POINT('',(14.5,-23.6446928191972,136.97510175753));
#48850=CARTESIAN_POINT('',(14.2590041943422,-23.3405926243297,136.784009272306));
#48851=CARTESIAN_POINT('',(14.,-23.6446928191972,136.97510175753));
#48852=CARTESIAN_POINT('',(14.5,-23.016899728323,136.580604996376));
#48853=CARTESIAN_POINT('',(14.,-23.016899728323,136.580604996376));
#48854=CARTESIAN_POINT('',(14.6801520303733,-22.7895751597781,136.437757285362));
#48855=CARTESIAN_POINT('Origin',(57.75,-23.6012807747805,136.728899819277));
#48856=CARTESIAN_POINT('',(58.,-23.5578687303638,136.482697881024));
#48857=CARTESIAN_POINT('',(57.5,-23.6446928191972,136.97510175753));
#48858=CARTESIAN_POINT('Origin',(57.75,-22.5927285851944,134.149374290983));
#48859=CARTESIAN_POINT('',(57.5,-22.3520681602006,134.217068898167));
#48860=CARTESIAN_POINT('',(58.,-22.8333890101882,134.081679683799));
#48861=CARTESIAN_POINT('Origin',(14.25,-24.801902691856,135.790690514667));
#48862=CARTESIAN_POINT('',(14.,-24.5894609761083,136.30080033501));
#48863=CARTESIAN_POINT('',(14.5,-25.1219044487155,136.71462949103));
#48864=CARTESIAN_POINT('',(14.,-24.5526029471227,135.809389104878));
#48865=CARTESIAN_POINT('',(14.5,-25.0512024365894,135.771991924456));
#48866=CARTESIAN_POINT('Origin',(14.,-23.1522889426911,137.061925846364));
#48867=CARTESIAN_POINT('',(14.5,-23.6446928191972,136.97510175753));
#48868=CARTESIAN_POINT('Origin',(14.25,-23.6012807747805,136.728899819277));
#48869=CARTESIAN_POINT('',(14.,-23.5110842376314,136.490947249372));
#48870=CARTESIAN_POINT('',(14.,-23.5110842376314,136.490947249372));
#48871=CARTESIAN_POINT('',(14.,-23.5578687303638,136.482697881024));
#48872=CARTESIAN_POINT('Origin',(14.25,-22.5927285851944,134.149374290983));
#48873=CARTESIAN_POINT('',(14.5,-22.3520681602006,134.217068898167));
#48874=CARTESIAN_POINT('',(14.,-22.8333890101882,134.081679683799));
#48875=CARTESIAN_POINT('Origin',(14.,-22.0637731308185,133.192154105382));
#48876=CARTESIAN_POINT('Origin',(14.,-25.1219044487155,136.71462949103));
#48877=CARTESIAN_POINT('Origin',(57.5,-35.4928843561059,134.393099376732));
#48878=CARTESIAN_POINT('',(57.5,-34.8330975492484,134.054819567983));
#48879=CARTESIAN_POINT('',(58.,-35.3175873497673,133.922431977811));
#48880=CARTESIAN_POINT('',(57.5,-34.8330975492484,134.054819567983));
#48881=CARTESIAN_POINT('',(57.5,-35.4928843561059,134.393099376732));
#48882=CARTESIAN_POINT('',(57.5,-35.4928843561059,134.393099376732));
#48883=CARTESIAN_POINT('',(58.,-35.3175873497673,133.922431977811));
#48884=CARTESIAN_POINT('Origin',(57.5,-36.8610624138407,133.511428020236));
#48885=CARTESIAN_POINT('',(57.5,-36.4588101823949,134.134280331629));
#48886=CARTESIAN_POINT('',(58.,-36.375288143631,133.639021904261));
#48887=CARTESIAN_POINT('',(57.5,-36.4588101823949,134.134280331629));
#48888=CARTESIAN_POINT('',(57.5,-36.8610624138407,133.511428020236));
#48889=CARTESIAN_POINT('',(57.5,-36.8610624138407,133.511428020236));
#48890=CARTESIAN_POINT('',(58.,-36.375288143631,133.639021904261));
#48891=CARTESIAN_POINT('Origin',(14.,-35.3175873497673,133.922431977811));
#48892=CARTESIAN_POINT('',(14.5,-34.8330975492484,134.054819567983));
#48893=CARTESIAN_POINT('',(14.5,-35.4928843561059,134.393099376732));
#48894=CARTESIAN_POINT('',(14.5,-34.8330975492484,134.054819567983));
#48895=CARTESIAN_POINT('',(14.,-35.3175873497673,133.922431977811));
#48896=CARTESIAN_POINT('',(14.,-35.3175873497673,133.922431977811));
#48897=CARTESIAN_POINT('',(14.5,-35.4928843561059,134.393099376732));
#48898=CARTESIAN_POINT('Origin',(14.25,-34.1986447874607,131.669809380463));
#48899=CARTESIAN_POINT('',(14.,-34.4324894531109,131.581397433607));
#48900=CARTESIAN_POINT('',(14.5,-33.9648001218105,131.75822132732));
#48901=CARTESIAN_POINT('Origin',(14.5,-36.8610624138407,133.511428020236));
#48902=CARTESIAN_POINT('',(14.,-36.375288143631,133.639021904261));
#48903=CARTESIAN_POINT('',(14.5,-36.4588101823949,134.134280331629));
#48904=CARTESIAN_POINT('',(14.,-36.375288143631,133.639021904261));
#48905=CARTESIAN_POINT('',(14.5,-36.8610624138407,133.511428020236));
#48906=CARTESIAN_POINT('',(14.5,-36.8610624138407,133.511428020236));
#48907=CARTESIAN_POINT('',(14.5,-36.4588101823949,134.134280331629));
#48908=CARTESIAN_POINT('Origin',(14.25,-36.5424624542376,133.112337690265));
#48909=CARTESIAN_POINT('',(14.5,-36.7891838486583,133.071982349415));
#48910=CARTESIAN_POINT('',(14.,-36.2957410598168,133.152693031114));
#48911=CARTESIAN_POINT('Origin',(14.,-36.6599362981178,133.822854175933));
#48912=CARTESIAN_POINT('',(14.,-36.4588101823949,134.134280331629));
#48913=CARTESIAN_POINT('',(14.,-36.8610624138407,133.511428020236));
#48914=CARTESIAN_POINT('Origin',(14.25,-35.4281795948302,134.151617920159));
#48915=CARTESIAN_POINT('',(14.5,-35.4928843561059,134.393099376732));
#48916=CARTESIAN_POINT('',(14.,-35.3634748335546,133.910136463587));
#48917=CARTESIAN_POINT('Origin',(14.,-35.1629909526771,134.223959472357));
#48918=CARTESIAN_POINT('',(14.,-34.8330975492484,134.054819567983));
#48919=CARTESIAN_POINT('',(14.,-35.4928843561059,134.393099376732));
#48920=CARTESIAN_POINT('Origin',(57.75,-36.5424624542376,133.112337690265));
#48921=CARTESIAN_POINT('',(58.,-36.2957410598168,133.152693031114));
#48922=CARTESIAN_POINT('',(57.5,-36.7891838486583,133.071982349415));
#48923=CARTESIAN_POINT('Origin',(57.75,-35.4281795948302,134.151617920159));
#48924=CARTESIAN_POINT('',(58.,-35.3634748335546,133.910136463587));
#48925=CARTESIAN_POINT('',(57.5,-35.4928843561059,134.393099376732));
#48926=CARTESIAN_POINT('Origin',(57.75,-34.1986447874607,131.669809380463));
#48927=CARTESIAN_POINT('',(57.5,-33.9648001218105,131.75822132732));
#48928=CARTESIAN_POINT('',(58.,-34.4324894531109,131.581397433607));
#48929=CARTESIAN_POINT('Origin',(14.,-35.4582091790453,132.331838201602));
#48930=CARTESIAN_POINT('Origin',(14.,-33.5882749320356,130.762333212168));
#48931=CARTESIAN_POINT('Origin',(14.,-35.0099214429613,134.522508899283));
#48932=CARTESIAN_POINT('Origin',(57.5,-47.070953611875,130.788284360904));
#48933=CARTESIAN_POINT('',(57.5,-46.3841944650247,130.508796018164));
#48934=CARTESIAN_POINT('',(58.,-46.8553022968291,130.334686134323));
#48935=CARTESIAN_POINT('',(57.5,-46.3841944650247,130.508796018164));
#48936=CARTESIAN_POINT('',(57.5,-47.070953611875,130.788284360904));
#48937=CARTESIAN_POINT('',(57.5,-47.070953611875,130.788284360904));
#48938=CARTESIAN_POINT('',(58.,-46.8553022968291,130.334686134323));
#48939=CARTESIAN_POINT('Origin',(57.5,-48.3570826171013,129.790723455271));
#48940=CARTESIAN_POINT('',(57.5,-48.0106462326609,130.446264217578));
#48941=CARTESIAN_POINT('',(58.,-47.8842774043812,129.960169823373));
#48942=CARTESIAN_POINT('',(57.5,-48.0106462326609,130.446264217578));
#48943=CARTESIAN_POINT('',(57.5,-48.3570826171013,129.790723455271));
#48944=CARTESIAN_POINT('',(57.5,-48.3570826171013,129.790723455271));
#48945=CARTESIAN_POINT('',(58.,-47.8842774043812,129.960169823373));
#48946=CARTESIAN_POINT('Origin',(14.,-46.8553022968291,130.334686134323));
#48947=CARTESIAN_POINT('',(14.5,-46.3841944650247,130.508796018164));
#48948=CARTESIAN_POINT('',(14.5,-47.070953611875,130.788284360904));
#48949=CARTESIAN_POINT('',(14.5,-46.3841944650247,130.508796018164));
#48950=CARTESIAN_POINT('',(14.,-46.8553022968291,130.334686134323));
#48951=CARTESIAN_POINT('',(14.,-46.8553022968291,130.334686134323));
#48952=CARTESIAN_POINT('',(14.5,-47.070953611875,130.788284360904));
#48953=CARTESIAN_POINT('Origin',(14.25,-45.5442886531881,128.188157716154));
#48954=CARTESIAN_POINT('',(14.,-45.7695378603898,128.079701297925));
#48955=CARTESIAN_POINT('',(14.5,-45.3190394459863,128.296614134382));
#48956=CARTESIAN_POINT('Origin',(14.5,-48.3570826171013,129.790723455271));
#48957=CARTESIAN_POINT('',(14.,-47.8842774043812,129.960169823373));
#48958=CARTESIAN_POINT('',(14.5,-48.0106462326609,130.446264217578));
#48959=CARTESIAN_POINT('',(14.,-47.8842774043812,129.960169823373));
#48960=CARTESIAN_POINT('',(14.5,-48.3570826171013,129.790723455271));
#48961=CARTESIAN_POINT('',(14.5,-48.3570826171013,129.790723455271));
#48962=CARTESIAN_POINT('',(14.5,-48.0106462326609,130.446264217578));
#48963=CARTESIAN_POINT('Origin',(14.25,-48.0049120124002,129.420919600612));
#48964=CARTESIAN_POINT('',(14.5,-48.2471773577224,129.359214637636));
#48965=CARTESIAN_POINT('',(14.,-47.762646667078,129.482624563588));
#48966=CARTESIAN_POINT('Origin',(14.,-48.1838644248811,130.118493836425));
#48967=CARTESIAN_POINT('',(14.,-48.0106462326609,130.446264217578));
#48968=CARTESIAN_POINT('',(14.,-48.3570826171013,129.790723455271));
#48969=CARTESIAN_POINT('Origin',(14.25,-46.9854485760436,130.553361205708));
#48970=CARTESIAN_POINT('',(14.5,-47.070953611875,130.788284360904));
#48971=CARTESIAN_POINT('',(14.,-46.8999435402122,130.318438050511));
#48972=CARTESIAN_POINT('Origin',(14.,-46.7275740384498,130.648540189534));
#48973=CARTESIAN_POINT('',(14.,-46.3841944650247,130.508796018164));
#48974=CARTESIAN_POINT('',(14.,-47.070953611875,130.788284360904));
#48975=CARTESIAN_POINT('Origin',(57.75,-48.0049120124002,129.420919600612));
#48976=CARTESIAN_POINT('',(58.,-47.762646667078,129.482624563588));
#48977=CARTESIAN_POINT('',(57.5,-48.2471773577224,129.359214637636));
#48978=CARTESIAN_POINT('Origin',(57.75,-46.9854485760436,130.553361205708));
#48979=CARTESIAN_POINT('',(58.,-46.8999435402122,130.318438050511));
#48980=CARTESIAN_POINT('',(57.5,-47.070953611875,130.788284360904));
#48981=CARTESIAN_POINT('Origin',(57.75,-45.5442886531881,128.188157716154));
#48982=CARTESIAN_POINT('',(57.5,-45.3190394459863,128.296614134382));
#48983=CARTESIAN_POINT('',(58.,-45.7695378603898,128.079701297925));
#48984=CARTESIAN_POINT('Origin',(14.,-46.8567596356166,128.737889047669));
#48985=CARTESIAN_POINT('Origin',(14.,-44.857149679865,127.337332006754));
#48986=CARTESIAN_POINT('Origin',(14.,-46.601107301482,130.959294432567));
#48987=CARTESIAN_POINT('Origin',(57.75,-56.5433129818713,123.730916769498));
#48988=CARTESIAN_POINT('',(57.7487592975525,-57.9365320709093,126.078806628123));
#48989=CARTESIAN_POINT('',(58.,-58.036420101407,125.755014631118));
#48990=CARTESIAN_POINT('',(58.2319907935076,-58.1286547721085,125.456031378864));
#48991=CARTESIAN_POINT('',(58.,-56.7582524481486,123.603241298728));
#48992=CARTESIAN_POINT('',(57.5,-57.5822796533797,125.969521727281));
#48993=CARTESIAN_POINT('',(57.5,-56.3283735155941,123.858592240269));
#48994=CARTESIAN_POINT('',(50.4896657310029,-47.5990232005882,122.889742627585));
#48995=CARTESIAN_POINT('Origin',(58.,-57.8987018584758,124.164166824021));
#48996=CARTESIAN_POINT('',(58.,-59.0288384007668,125.292242378034));
#48997=CARTESIAN_POINT('',(58.,-58.0794753575685,125.734937635446));
#48998=CARTESIAN_POINT('',(58.,-58.8660496933282,124.827115139388));
#48999=CARTESIAN_POINT('Origin',(57.75,-58.1851299230037,125.961514582206));
#49000=CARTESIAN_POINT('',(57.5,-58.2907844884389,126.188091528965));
#49001=CARTESIAN_POINT('',(57.5,-58.2907844884389,126.188091528965));
#49002=CARTESIAN_POINT('',(57.5,-59.1970922754756,125.765473267224));
#49003=CARTESIAN_POINT('',(57.5,-58.2907844884389,126.188091528965));
#49004=CARTESIAN_POINT('',(57.5,-59.1970922754756,125.765473267224));
#49005=CARTESIAN_POINT('Origin',(14.,-57.9365320709093,126.078806628123));
#49006=CARTESIAN_POINT('',(14.5,-57.5822796533797,125.969521727281));
#49007=CARTESIAN_POINT('',(14.,-57.5822796533797,125.969521727281));
#49008=CARTESIAN_POINT('',(14.5,-58.2907844884389,126.188091528965));
#49009=CARTESIAN_POINT('',(14.5,-57.5822796533797,125.969521727281));
#49010=CARTESIAN_POINT('',(14.,-58.2907844884389,126.188091528965));
#49011=CARTESIAN_POINT('Origin',(57.5,-59.4850762228408,125.08223311503));
#49012=CARTESIAN_POINT('',(57.5,-59.4850762228408,125.08223311503));
#49013=CARTESIAN_POINT('',(57.5,-59.4850762228408,125.08223311503));
#49014=CARTESIAN_POINT('',(58.,-59.0288384007668,125.292242378034));
#49015=CARTESIAN_POINT('Origin',(14.,-58.036420101407,125.755014631118));
#49016=CARTESIAN_POINT('',(14.,-58.036420101407,125.755014631118));
#49017=CARTESIAN_POINT('',(14.,-58.036420101407,125.755014631118));
#49018=CARTESIAN_POINT('',(14.5,-58.2907844884389,126.188091528965));
#49019=CARTESIAN_POINT('Origin',(14.25,-56.5433129818713,123.730916769498));
#49020=CARTESIAN_POINT('',(14.,-56.7582524481486,123.603241298728));
#49021=CARTESIAN_POINT('',(14.5,-56.3283735155941,123.858592240269));
#49022=CARTESIAN_POINT('Origin',(14.5,-59.4850762228408,125.08223311503));
#49023=CARTESIAN_POINT('',(14.,-59.0288384007668,125.292242378034));
#49024=CARTESIAN_POINT('',(14.5,-59.1970922754756,125.765473267224));
#49025=CARTESIAN_POINT('',(14.,-59.0288384007668,125.292242378034));
#49026=CARTESIAN_POINT('',(14.5,-59.4850762228408,125.08223311503));
#49027=CARTESIAN_POINT('',(14.5,-59.4850762228408,125.08223311503));
#49028=CARTESIAN_POINT('',(14.5,-59.1970922754756,125.765473267224));
#49029=CARTESIAN_POINT('Origin',(14.25,-59.1020152039901,124.744530166311));
#49030=CARTESIAN_POINT('',(14.5,-59.3379807146521,124.661945193235));
#49031=CARTESIAN_POINT('',(14.,-58.8660496933282,124.827115139388));
#49032=CARTESIAN_POINT('Origin',(14.,-59.3410842491582,125.423853191127));
#49033=CARTESIAN_POINT('',(14.,-59.1970922754756,125.765473267224));
#49034=CARTESIAN_POINT('',(14.,-59.4850762228408,125.08223311503));
#49035=CARTESIAN_POINT('Origin',(14.25,-58.1851299230037,125.961514582206));
#49036=CARTESIAN_POINT('',(14.5,-58.2907844884389,126.188091528965));
#49037=CARTESIAN_POINT('',(14.,-58.0794753575686,125.734937635446));
#49038=CARTESIAN_POINT('Origin',(57.75,-59.1020152039902,124.744530166311));
#49039=CARTESIAN_POINT('',(57.5,-59.3379807146521,124.661945193235));
#49040=CARTESIAN_POINT('Origin',(14.,-55.7846344331431,122.943216816385));
#49041=CARTESIAN_POINT('Origin',(14.,-57.8376305949206,126.399400659835));
#49042=CARTESIAN_POINT('Origin',(57.5,-69.0669872981078,120.627531126037));
#49043=CARTESIAN_POINT('',(57.5,-68.3421289244415,120.471543313576));
#49044=CARTESIAN_POINT('',(58.,-68.7758457056646,120.218271533617));
#49045=CARTESIAN_POINT('',(57.5,-68.3421289244415,120.471543313576));
#49046=CARTESIAN_POINT('',(57.5,-69.0669872981078,120.627531126037));
#49047=CARTESIAN_POINT('',(57.5,-69.0669872981078,120.627531126037));
#49048=CARTESIAN_POINT('',(58.,-68.7758457056646,120.218271533617));
#49049=CARTESIAN_POINT('Origin',(57.5,-70.1603524804535,119.421791454066));
#49050=CARTESIAN_POINT('',(57.5,-69.9330127018922,120.127531126037));
#49051=CARTESIAN_POINT('',(58.,-69.7241542943354,119.670765314673));
#49052=CARTESIAN_POINT('',(57.5,-69.9330127018922,120.127531126037));
#49053=CARTESIAN_POINT('',(57.5,-70.1603524804535,119.421791454066));
#49054=CARTESIAN_POINT('',(57.5,-70.1603524804535,119.421791454066));
#49055=CARTESIAN_POINT('',(58.,-69.7241542943354,119.670765314673));
#49056=CARTESIAN_POINT('Origin',(14.,-68.7758457056646,120.218271533617));
#49057=CARTESIAN_POINT('',(14.5,-68.3421289244415,120.471543313576));
#49058=CARTESIAN_POINT('',(14.5,-69.0669872981078,120.627531126037));
#49059=CARTESIAN_POINT('',(14.5,-68.3421289244415,120.471543313576));
#49060=CARTESIAN_POINT('',(14.,-68.7758457056646,120.218271533617));
#49061=CARTESIAN_POINT('',(14.,-68.7758457056646,120.218271533617));
#49062=CARTESIAN_POINT('',(14.5,-69.0669872981078,120.627531126037));
#49063=CARTESIAN_POINT('Origin',(14.25,-67.1120085569767,118.332008835457));
#49064=CARTESIAN_POINT('',(14.,-67.3150024632071,118.18608599957));
#49065=CARTESIAN_POINT('',(14.5,-66.9090146507463,118.477931671344));
#49066=CARTESIAN_POINT('Origin',(14.5,-70.1603524804535,119.421791454066));
#49067=CARTESIAN_POINT('',(14.,-69.7241542943354,119.670765314673));
#49068=CARTESIAN_POINT('',(14.5,-69.9330127018922,120.127531126037));
#49069=CARTESIAN_POINT('',(14.,-69.7241542943354,119.670765314673));
#49070=CARTESIAN_POINT('',(14.5,-70.1603524804535,119.421791454066));
#49071=CARTESIAN_POINT('',(14.5,-70.1603524804535,119.421791454066));
#49072=CARTESIAN_POINT('',(14.5,-69.9330127018922,120.127531126037));
#49073=CARTESIAN_POINT('Origin',(14.25,-69.7493163731052,119.118759534638));
#49074=CARTESIAN_POINT('',(14.5,-69.9771862090909,119.015923072972));
#49075=CARTESIAN_POINT('',(14.,-69.5214465371196,119.221595996303));
#49076=CARTESIAN_POINT('Origin',(14.,-70.0466825911729,119.774661290051));
#49077=CARTESIAN_POINT('',(14.,-69.9330127018922,120.127531126037));
#49078=CARTESIAN_POINT('',(14.,-70.1603524804535,119.421791454066));
#49079=CARTESIAN_POINT('Origin',(14.25,-68.9419872981078,120.411024775091));
#49080=CARTESIAN_POINT('',(14.5,-69.0669872981078,120.627531126037));
#49081=CARTESIAN_POINT('',(14.,-68.8169872981078,120.194518424145));
#49082=CARTESIAN_POINT('Origin',(14.,-68.7045581112746,120.549537219807));
#49083=CARTESIAN_POINT('',(14.,-68.3421289244415,120.471543313576));
#49084=CARTESIAN_POINT('',(14.,-69.0669872981078,120.627531126037));
#49085=CARTESIAN_POINT('Origin',(57.75,-69.7493163731052,119.118759534638));
#49086=CARTESIAN_POINT('',(58.,-69.5214465371196,119.221595996303));
#49087=CARTESIAN_POINT('',(57.5,-69.9771862090909,119.015923072972));
#49088=CARTESIAN_POINT('Origin',(57.75,-68.9419872981078,120.411024775091));
#49089=CARTESIAN_POINT('',(58.,-68.8169872981078,120.194518424145));
#49090=CARTESIAN_POINT('',(57.5,-69.0669872981078,120.627531126037));
#49091=CARTESIAN_POINT('Origin',(57.75,-67.1120085569767,118.332008835457));
#49092=CARTESIAN_POINT('',(57.5,-66.9090146507463,118.477931671344));
#49093=CARTESIAN_POINT('',(58.,-67.3150024632071,118.18608599957));
#49094=CARTESIAN_POINT('Origin',(14.,-68.5,118.645480318468));
#49095=CARTESIAN_POINT('Origin',(14.,-66.2875644347018,117.613429510899));
#49096=CARTESIAN_POINT('Origin',(14.,-68.6339745962156,120.877531126037));
#49097=CARTESIAN_POINT('Origin',(57.5,-80.3016660917109,112.852477851287));
#49098=CARTESIAN_POINT('',(57.5,-80.1367006749399,113.575345937994));
#49099=CARTESIAN_POINT('',(58.,-79.8888272731288,113.138521468083));
#49100=CARTESIAN_POINT('',(57.5,-80.1367006749399,113.575345937994));
#49101=CARTESIAN_POINT('',(57.5,-80.3016660917109,112.852477851287));
#49102=CARTESIAN_POINT('',(57.5,-80.3016660917109,112.852477851287));
#49103=CARTESIAN_POINT('',(58.,-79.8888272731288,113.138521468083));
#49104=CARTESIAN_POINT('Origin',(14.,-80.2191833833254,113.213911894641));
#49105=CARTESIAN_POINT('',(14.2512407024475,-80.2191833833254,113.213911894641));
#49106=CARTESIAN_POINT('',(14.5,-80.3016660917109,112.852477851287));
#49107=CARTESIAN_POINT('',(14.3353834448875,-80.2470831296091,113.091656960179));
#49108=CARTESIAN_POINT('',(14.,-80.3016660917109,112.852477851287));
#49109=CARTESIAN_POINT('',(14.5,-80.1367006749399,113.575345937994));
#49110=CARTESIAN_POINT('',(14.,-80.1367006749399,113.575345937994));
#49111=CARTESIAN_POINT('',(14.4305329766294,-80.159734299361,113.474414043655));
#49112=CARTESIAN_POINT('Origin',(57.75,-79.8657831288323,112.586423217032));
#49113=CARTESIAN_POINT('',(58.,-79.6477431945663,112.708728519719));
#49114=CARTESIAN_POINT('',(57.5,-80.0838230630982,112.464117914346));
#49115=CARTESIAN_POINT('Origin',(57.5,-79.3175486306509,114.148922374345));
#49116=CARTESIAN_POINT('',(57.5,-78.5818533282825,114.056703712549));
#49117=CARTESIAN_POINT('',(58.,-78.991845596111,113.766594799967));
#49118=CARTESIAN_POINT('',(57.5,-78.5818533282825,114.056703712549));
#49119=CARTESIAN_POINT('',(57.5,-79.3175486306509,114.148922374345));
#49120=CARTESIAN_POINT('',(57.5,-79.3175486306509,114.148922374345));
#49121=CARTESIAN_POINT('',(58.,-78.991845596111,113.766594799967));
#49122=CARTESIAN_POINT('Origin',(14.,-78.9497009794667,114.102813043447));
#49123=CARTESIAN_POINT('',(14.2512407024475,-78.9497009794667,114.102813043447));
#49124=CARTESIAN_POINT('',(14.5,-79.3175486306509,114.148922374345));
#49125=CARTESIAN_POINT('',(14.2590041943422,-78.9611810820661,114.104252062693));
#49126=CARTESIAN_POINT('',(14.,-79.3175486306509,114.148922374345));
#49127=CARTESIAN_POINT('',(14.5,-78.5818533282825,114.056703712549));
#49128=CARTESIAN_POINT('',(14.,-78.5818533282825,114.056703712549));
#49129=CARTESIAN_POINT('',(14.6801520303733,-78.3154572503032,114.023311233706));
#49130=CARTESIAN_POINT('Origin',(57.75,-79.1741545215632,113.944134363273));
#49131=CARTESIAN_POINT('',(58.,-79.0307604124754,113.739346352201));
#49132=CARTESIAN_POINT('',(57.5,-79.3175486306509,114.148922374345));
#49133=CARTESIAN_POINT('Origin',(57.75,-77.1699412236247,112.032522863357));
#49134=CARTESIAN_POINT('',(57.5,-76.9804377836387,112.195582503469));
#49135=CARTESIAN_POINT('',(58.,-77.3594446636108,111.869463223246));
#49136=CARTESIAN_POINT('Origin',(14.25,-79.8657831288323,112.586423217032));
#49137=CARTESIAN_POINT('',(14.,-79.8888272731288,113.138521468083));
#49138=CARTESIAN_POINT('',(14.5,-80.5462766970844,113.288557719819));
#49139=CARTESIAN_POINT('',(14.,-79.6477431945663,112.708728519719));
#49140=CARTESIAN_POINT('',(14.5,-80.0838230630982,112.464117914346));
#49141=CARTESIAN_POINT('Origin',(14.,-78.9079726085064,114.435710592521));
#49142=CARTESIAN_POINT('',(14.5,-79.3175486306509,114.148922374345));
#49143=CARTESIAN_POINT('Origin',(14.25,-79.1741545215632,113.944134363273));
#49144=CARTESIAN_POINT('',(14.,-78.991845596111,113.766594799967));
#49145=CARTESIAN_POINT('',(14.,-78.991845596111,113.766594799967));
#49146=CARTESIAN_POINT('',(14.,-79.0307604124754,113.739346352201));
#49147=CARTESIAN_POINT('Origin',(14.25,-77.1699412236247,112.032522863357));
#49148=CARTESIAN_POINT('',(14.5,-76.9804377836387,112.195582503469));
#49149=CARTESIAN_POINT('',(14.,-77.3594446636108,111.869463223246));
#49150=CARTESIAN_POINT('Origin',(14.,-76.2860060453866,111.388532989905));
#49151=CARTESIAN_POINT('Origin',(14.,-80.5462766970844,113.288557719819));
#49152=CARTESIAN_POINT('Origin',(57.5,-88.9644555248695,106.801571398381));
#49153=CARTESIAN_POINT('',(57.5,-88.223522379275,106.773823726948));
#49154=CARTESIAN_POINT('',(58.,-88.6066698449906,106.449085585742));
#49155=CARTESIAN_POINT('',(57.5,-88.223522379275,106.773823726948));
#49156=CARTESIAN_POINT('',(57.5,-88.9644555248695,106.801571398381));
#49157=CARTESIAN_POINT('',(57.5,-88.9644555248695,106.801571398381));
#49158=CARTESIAN_POINT('',(58.,-88.6066698449906,106.449085585742));
#49159=CARTESIAN_POINT('Origin',(57.5,-89.8318355365387,105.424288749871));
#49160=CARTESIAN_POINT('',(57.5,-89.7304999679885,106.158783788695));
#49161=CARTESIAN_POINT('',(58.,-89.4454980381808,105.745225158215));
#49162=CARTESIAN_POINT('',(57.5,-89.7304999679885,106.158783788695));
#49163=CARTESIAN_POINT('',(57.5,-89.8318355365387,105.424288749871));
#49164=CARTESIAN_POINT('',(57.5,-89.8318355365387,105.424288749871));
#49165=CARTESIAN_POINT('',(58.,-89.4454980381808,105.745225158215));
#49166=CARTESIAN_POINT('Origin',(14.,-88.6066698449906,106.449085585742));
#49167=CARTESIAN_POINT('',(14.5,-88.223522379275,106.773823726948));
#49168=CARTESIAN_POINT('',(14.5,-88.9644555248695,106.801571398381));
#49169=CARTESIAN_POINT('',(14.5,-88.223522379275,106.773823726948));
#49170=CARTESIAN_POINT('',(14.,-88.6066698449906,106.449085585742));
#49171=CARTESIAN_POINT('',(14.,-88.6066698449906,106.449085585742));
#49172=CARTESIAN_POINT('',(14.5,-88.9644555248695,106.801571398381));
#49173=CARTESIAN_POINT('Origin',(14.25,-86.6405640410765,104.880401745181));
#49174=CARTESIAN_POINT('',(14.,-86.8151347792147,104.701446283163));
#49175=CARTESIAN_POINT('',(14.5,-86.4659933029384,105.059357207198));
#49176=CARTESIAN_POINT('Origin',(14.5,-89.8318355365387,105.424288749871));
#49177=CARTESIAN_POINT('',(14.,-89.4454980381808,105.745225158215));
#49178=CARTESIAN_POINT('',(14.5,-89.7304999679885,106.158783788695));
#49179=CARTESIAN_POINT('',(14.,-89.4454980381808,105.745225158215));
#49180=CARTESIAN_POINT('',(14.5,-89.8318355365387,105.424288749871));
#49181=CARTESIAN_POINT('',(14.5,-89.8318355365387,105.424288749871));
#49182=CARTESIAN_POINT('',(14.5,-89.7304999679885,106.158783788695));
#49183=CARTESIAN_POINT('Origin',(14.25,-89.3744230506705,105.197236237204));
#49184=CARTESIAN_POINT('',(14.5,-89.5809736676609,105.0563929107));
#49185=CARTESIAN_POINT('',(14.,-89.1678724336801,105.338079563709));
#49186=CARTESIAN_POINT('Origin',(14.,-89.7811677522636,105.791536269283));
#49187=CARTESIAN_POINT('',(14.,-89.7304999679885,106.158783788695));
#49188=CARTESIAN_POINT('',(14.,-89.8318355365387,105.424288749871));
#49189=CARTESIAN_POINT('Origin',(14.25,-88.8037586224479,106.610060287601));
#49190=CARTESIAN_POINT('',(14.5,-88.9644555248695,106.801571398381));
#49191=CARTESIAN_POINT('',(14.,-88.6430617200262,106.418549176822));
#49192=CARTESIAN_POINT('Origin',(14.,-88.5939889520722,106.787697562665));
#49193=CARTESIAN_POINT('',(14.,-88.223522379275,106.773823726948));
#49194=CARTESIAN_POINT('',(14.,-88.9644555248695,106.801571398381));
#49195=CARTESIAN_POINT('Origin',(57.75,-89.3744230506705,105.197236237204));
#49196=CARTESIAN_POINT('',(58.,-89.1678724336801,105.338079563709));
#49197=CARTESIAN_POINT('',(57.5,-89.5809736676609,105.0563929107));
#49198=CARTESIAN_POINT('Origin',(57.75,-88.8037586224478,106.610060287601));
#49199=CARTESIAN_POINT('',(58.,-88.6430617200262,106.418549176822));
#49200=CARTESIAN_POINT('',(57.5,-88.9644555248695,106.801571398381));
#49201=CARTESIAN_POINT('Origin',(57.75,-86.6405640410765,104.880401745181));
#49202=CARTESIAN_POINT('',(57.5,-86.4659933029383,105.059357207198));
#49203=CARTESIAN_POINT('',(58.,-86.8151347792147,104.701446283163));
#49204=CARTESIAN_POINT('Origin',(14.,-88.0619025270559,104.9480887073));
#49205=CARTESIAN_POINT('Origin',(14.,-85.7038650873162,104.315902474623));
#49206=CARTESIAN_POINT('Origin',(14.,-88.58143330331,107.122965203225));
#49207=CARTESIAN_POINT('Origin',(57.5,-97.9342891943368,98.6413959755234));
#49208=CARTESIAN_POINT('',(57.5,-97.1937571541419,98.678330470988));
#49209=CARTESIAN_POINT('',(58.,-97.5471438341797,98.3214345544939));
#49210=CARTESIAN_POINT('',(57.5,-97.1937571541419,98.678330470988));
#49211=CARTESIAN_POINT('',(57.5,-97.9342891943368,98.6413959755234));
#49212=CARTESIAN_POINT('',(57.5,-97.9342891943368,98.6413959755234));
#49213=CARTESIAN_POINT('',(58.,-97.5471438341797,98.3214345544939));
#49214=CARTESIAN_POINT('Origin',(57.5,-98.678330470988,97.1937571541419));
#49215=CARTESIAN_POINT('',(57.5,-98.6413959755234,97.9342891943368));
#49216=CARTESIAN_POINT('',(58.,-98.3214345544939,97.5471438341798));
#49217=CARTESIAN_POINT('',(57.5,-98.6413959755234,97.9342891943368));
#49218=CARTESIAN_POINT('',(57.5,-98.678330470988,97.1937571541419));
#49219=CARTESIAN_POINT('',(57.5,-98.678330470988,97.1937571541419));
#49220=CARTESIAN_POINT('',(58.,-98.3214345544939,97.5471438341798));
#49221=CARTESIAN_POINT('Origin',(14.,-97.5471438341798,98.3214345544939));
#49222=CARTESIAN_POINT('',(14.5,-97.1937571541419,98.678330470988));
#49223=CARTESIAN_POINT('',(14.5,-97.9342891943368,98.6413959755234));
#49224=CARTESIAN_POINT('',(14.5,-97.1937571541419,98.678330470988));
#49225=CARTESIAN_POINT('',(14.,-97.5471438341798,98.3214345544939));
#49226=CARTESIAN_POINT('',(14.,-97.5471438341798,98.3214345544939));
#49227=CARTESIAN_POINT('',(14.5,-97.9342891943368,98.6413959755234));
#49228=CARTESIAN_POINT('Origin',(14.25,-95.4517998511728,96.9300774412053));
#49229=CARTESIAN_POINT('',(14.,-95.6101092987371,96.7365881164044));
#49230=CARTESIAN_POINT('',(14.5,-95.2934904036084,97.1235667660061));
#49231=CARTESIAN_POINT('Origin',(14.5,-98.678330470988,97.1937571541419));
#49232=CARTESIAN_POINT('',(14.,-98.3214345544939,97.5471438341798));
#49233=CARTESIAN_POINT('',(14.5,-98.6413959755234,97.9342891943368));
#49234=CARTESIAN_POINT('',(14.,-98.3214345544939,97.5471438341798));
#49235=CARTESIAN_POINT('',(14.5,-98.678330470988,97.1937571541419));
#49236=CARTESIAN_POINT('',(14.5,-98.678330470988,97.1937571541419));
#49237=CARTESIAN_POINT('',(14.5,-98.6413959755234,97.9342891943368));
#49238=CARTESIAN_POINT('Origin',(14.25,-98.2028696473411,97.0074347697832));
#49239=CARTESIAN_POINT('',(14.5,-98.3963589721419,96.8491253222189));
#49240=CARTESIAN_POINT('',(14.,-98.0093803225402,97.1657442173475));
#49241=CARTESIAN_POINT('Origin',(14.,-98.6598632232557,97.5640231742394));
#49242=CARTESIAN_POINT('',(14.,-98.6413959755234,97.9342891943368));
#49243=CARTESIAN_POINT('',(14.,-98.678330470988,97.1937571541419));
#49244=CARTESIAN_POINT('Origin',(14.25,-97.7575124990402,98.4646192802267));
#49245=CARTESIAN_POINT('',(14.5,-97.9342891943368,98.6413959755234));
#49246=CARTESIAN_POINT('',(14.,-97.5807358037436,98.2878425849301));
#49247=CARTESIAN_POINT('Origin',(14.,-97.5640231742394,98.6598632232557));
#49248=CARTESIAN_POINT('',(14.,-97.1937571541419,98.678330470988));
#49249=CARTESIAN_POINT('',(14.,-97.9342891943368,98.6413959755234));
#49250=CARTESIAN_POINT('Origin',(57.75,-98.2028696473411,97.0074347697832));
#49251=CARTESIAN_POINT('',(58.,-98.0093803225402,97.1657442173475));
#49252=CARTESIAN_POINT('',(57.5,-98.3963589721419,96.8491253222189));
#49253=CARTESIAN_POINT('Origin',(57.75,-97.7575124990402,98.4646192802267));
#49254=CARTESIAN_POINT('',(58.,-97.5807358037436,98.2878425849301));
#49255=CARTESIAN_POINT('',(57.5,-97.9342891943368,98.6413959755234));
#49256=CARTESIAN_POINT('Origin',(57.75,-95.4517998511728,96.9300774412053));
#49257=CARTESIAN_POINT('',(57.5,-95.2934904036084,97.1235667660061));
#49258=CARTESIAN_POINT('',(58.,-95.6101092987371,96.7365881164045));
#49259=CARTESIAN_POINT('Origin',(14.,-96.873629022557,96.873629022557));
#49260=CARTESIAN_POINT('Origin',(14.,-94.4694659665227,96.4493649538451));
#49261=CARTESIAN_POINT('Origin',(14.,-97.5807358037436,98.9949493661167));
#49262=CARTESIAN_POINT('Origin',(57.75,-103.536589829029,88.2420567199213));
#49263=CARTESIAN_POINT('',(57.7487592975525,-105.791536269283,89.7811677522636));
#49264=CARTESIAN_POINT('',(58.,-105.745225158215,89.4454980381808));
#49265=CARTESIAN_POINT('',(58.2319907935076,-105.702462376149,89.1355471322649));
#49266=CARTESIAN_POINT('',(58.,-103.677433155534,88.0355061029309));
#49267=CARTESIAN_POINT('',(57.5,-105.424288749871,89.8318355365387));
#49268=CARTESIAN_POINT('',(57.5,-103.395746502524,88.4486073369116));
#49269=CARTESIAN_POINT('',(50.4896657310024,-95.0748147970629,91.2597142447225));
#49270=CARTESIAN_POINT('Origin',(58.,-104.9480887073,88.0619025270559));
#49271=CARTESIAN_POINT('',(58.,-106.449085585742,88.6066698449906));
#49272=CARTESIAN_POINT('',(58.,-105.775761567135,89.4091061631452));
#49273=CARTESIAN_POINT('',(58.,-106.104977647464,88.2539188872116));
#49274=CARTESIAN_POINT('Origin',(57.75,-105.967272677915,89.5698030655668));
#49275=CARTESIAN_POINT('',(57.5,-106.158783788695,89.7304999679884));
#49276=CARTESIAN_POINT('',(57.5,-106.158783788695,89.7304999679884));
#49277=CARTESIAN_POINT('',(57.5,-106.801571398381,88.9644555248695));
#49278=CARTESIAN_POINT('',(57.5,-106.158783788695,89.7304999679885));
#49279=CARTESIAN_POINT('',(57.5,-106.801571398381,88.9644555248695));
#49280=CARTESIAN_POINT('Origin',(14.,-105.791536269283,89.7811677522635));
#49281=CARTESIAN_POINT('',(14.5,-105.424288749871,89.8318355365387));
#49282=CARTESIAN_POINT('',(14.,-105.424288749871,89.8318355365387));
#49283=CARTESIAN_POINT('',(14.5,-106.158783788695,89.7304999679884));
#49284=CARTESIAN_POINT('',(14.5,-105.424288749871,89.8318355365387));
#49285=CARTESIAN_POINT('',(14.,-106.158783788695,89.7304999679884));
#49286=CARTESIAN_POINT('Origin',(57.5,-106.773823726948,88.223522379275));
#49287=CARTESIAN_POINT('',(57.5,-106.773823726948,88.223522379275));
#49288=CARTESIAN_POINT('',(57.5,-106.773823726948,88.223522379275));
#49289=CARTESIAN_POINT('',(58.,-106.449085585742,88.6066698449906));
#49290=CARTESIAN_POINT('Origin',(14.,-105.745225158215,89.4454980381808));
#49291=CARTESIAN_POINT('',(14.,-105.745225158215,89.4454980381808));
#49292=CARTESIAN_POINT('',(14.,-105.745225158215,89.4454980381808));
#49293=CARTESIAN_POINT('',(14.5,-106.158783788695,89.7304999679884));
#49294=CARTESIAN_POINT('Origin',(14.25,-103.536589829029,88.2420567199213));
#49295=CARTESIAN_POINT('',(14.,-103.677433155534,88.0355061029309));
#49296=CARTESIAN_POINT('',(14.5,-103.395746502524,88.4486073369116));
#49297=CARTESIAN_POINT('Origin',(14.5,-106.773823726948,88.223522379275));
#49298=CARTESIAN_POINT('',(14.,-106.449085585742,88.6066698449906));
#49299=CARTESIAN_POINT('',(14.5,-106.801571398381,88.9644555248695));
#49300=CARTESIAN_POINT('',(14.,-106.449085585742,88.6066698449906));
#49301=CARTESIAN_POINT('',(14.5,-106.773823726948,88.223522379275));
#49302=CARTESIAN_POINT('',(14.5,-106.773823726948,88.223522379275));
#49303=CARTESIAN_POINT('',(14.5,-106.801571398381,88.9644555248695));
#49304=CARTESIAN_POINT('Origin',(14.25,-106.283933109481,88.0793481490734));
#49305=CARTESIAN_POINT('',(14.5,-106.462888571499,87.9047774109352));
#49306=CARTESIAN_POINT('',(14.,-106.104977647464,88.2539188872116));
#49307=CARTESIAN_POINT('Origin',(14.,-106.787697562665,88.5939889520722));
#49308=CARTESIAN_POINT('',(14.,-106.801571398381,88.9644555248695));
#49309=CARTESIAN_POINT('',(14.,-106.773823726948,88.223522379275));
#49310=CARTESIAN_POINT('Origin',(14.25,-105.967272677915,89.5698030655668));
#49311=CARTESIAN_POINT('',(14.5,-106.158783788695,89.7304999679885));
#49312=CARTESIAN_POINT('',(14.,-105.775761567135,89.4091061631452));
#49313=CARTESIAN_POINT('Origin',(57.75,-106.283933109481,88.0793481490734));
#49314=CARTESIAN_POINT('',(57.5,-106.462888571499,87.9047774109352));
#49315=CARTESIAN_POINT('Origin',(14.,-102.516097167501,87.8487895280494));
#49316=CARTESIAN_POINT('Origin',(14.,-105.837389983851,90.113522189548));
#49317=CARTESIAN_POINT('Origin',(57.5,-113.575345937994,80.1367006749399));
#49318=CARTESIAN_POINT('',(57.5,-112.852477851287,80.3016660917109));
#49319=CARTESIAN_POINT('',(58.,-113.138521468083,79.8888272731288));
#49320=CARTESIAN_POINT('',(57.5,-112.852477851287,80.3016660917109));
#49321=CARTESIAN_POINT('',(57.5,-113.575345937994,80.1367006749399));
#49322=CARTESIAN_POINT('',(57.5,-113.575345937994,80.1367006749399));
#49323=CARTESIAN_POINT('',(58.,-113.138521468083,79.8888272731288));
#49324=CARTESIAN_POINT('Origin',(57.5,-114.056703712549,78.5818533282825));
#49325=CARTESIAN_POINT('',(57.5,-114.148922374345,79.3175486306509));
#49326=CARTESIAN_POINT('',(58.,-113.766594799967,78.991845596111));
#49327=CARTESIAN_POINT('',(57.5,-114.148922374345,79.3175486306509));
#49328=CARTESIAN_POINT('',(57.5,-114.056703712549,78.5818533282825));
#49329=CARTESIAN_POINT('',(57.5,-114.056703712549,78.5818533282825));
#49330=CARTESIAN_POINT('',(58.,-113.766594799967,78.991845596111));
#49331=CARTESIAN_POINT('Origin',(14.,-113.138521468083,79.8888272731288));
#49332=CARTESIAN_POINT('',(14.5,-112.852477851287,80.3016660917109));
#49333=CARTESIAN_POINT('',(14.5,-113.575345937994,80.1367006749399));
#49334=CARTESIAN_POINT('',(14.5,-112.852477851287,80.3016660917109));
#49335=CARTESIAN_POINT('',(14.,-113.138521468083,79.8888272731288));
#49336=CARTESIAN_POINT('',(14.,-113.138521468083,79.8888272731288));
#49337=CARTESIAN_POINT('',(14.5,-113.575345937994,80.1367006749399));
#49338=CARTESIAN_POINT('Origin',(14.25,-110.833403841184,78.882460664988));
#49339=CARTESIAN_POINT('',(14.,-110.955709143871,78.664420730722));
#49340=CARTESIAN_POINT('',(14.5,-110.711098538497,79.1005005992539));
#49341=CARTESIAN_POINT('Origin',(14.5,-114.056703712549,78.5818533282825));
#49342=CARTESIAN_POINT('',(14.,-113.766594799967,78.991845596111));
#49343=CARTESIAN_POINT('',(14.5,-114.148922374345,79.3175486306509));
#49344=CARTESIAN_POINT('',(14.,-113.766594799967,78.991845596111));
#49345=CARTESIAN_POINT('',(14.5,-114.056703712549,78.5818533282825));
#49346=CARTESIAN_POINT('',(14.5,-114.056703712549,78.5818533282825));
#49347=CARTESIAN_POINT('',(14.5,-114.148922374345,79.3175486306509));
#49348=CARTESIAN_POINT('Origin',(14.25,-113.556111664665,78.4809245051846));
#49349=CARTESIAN_POINT('',(14.5,-113.719171304777,78.2914210651985));
#49350=CARTESIAN_POINT('',(14.,-113.393052024553,78.6704279451707));
#49351=CARTESIAN_POINT('Origin',(14.,-114.102813043447,78.9497009794667));
#49352=CARTESIAN_POINT('',(14.,-114.148922374345,79.3175486306509));
#49353=CARTESIAN_POINT('',(14.,-114.056703712549,78.5818533282825));
#49354=CARTESIAN_POINT('Origin',(14.25,-113.370557926922,79.9933065658522));
#49355=CARTESIAN_POINT('',(14.5,-113.575345937994,80.1367006749399));
#49356=CARTESIAN_POINT('',(14.,-113.16576991585,79.8499124567644));
#49357=CARTESIAN_POINT('Origin',(14.,-113.213911894641,80.2191833833254));
#49358=CARTESIAN_POINT('',(14.,-112.852477851287,80.3016660917109));
#49359=CARTESIAN_POINT('',(14.,-113.575345937994,80.1367006749399));
#49360=CARTESIAN_POINT('Origin',(57.75,-113.556111664665,78.4809245051846));
#49361=CARTESIAN_POINT('',(58.,-113.393052024553,78.6704279451707));
#49362=CARTESIAN_POINT('',(57.5,-113.719171304777,78.2914210651985));
#49363=CARTESIAN_POINT('Origin',(57.75,-113.370557926922,79.9933065658522));
#49364=CARTESIAN_POINT('',(58.,-113.16576991585,79.8499124567644));
#49365=CARTESIAN_POINT('',(57.5,-113.575345937994,80.1367006749399));
#49366=CARTESIAN_POINT('Origin',(57.75,-110.833403841184,78.882460664988));
#49367=CARTESIAN_POINT('',(57.5,-110.711098538497,79.1005005992539));
#49368=CARTESIAN_POINT('',(58.,-110.955709143871,78.664420730722));
#49369=CARTESIAN_POINT('Origin',(14.,-112.223830067592,78.5799717800933));
#49370=CARTESIAN_POINT('Origin',(14.,-109.782518968122,78.5796317693958));
#49371=CARTESIAN_POINT('Origin',(14.,-113.288557719819,80.5462766970844));
#49372=CARTESIAN_POINT('Origin',(57.5,-120.471543313576,68.3421289244415));
#49373=CARTESIAN_POINT('',(57.5,-120.627531126037,69.0669872981078));
#49374=CARTESIAN_POINT('',(58.,-120.218271533617,68.7758457056646));
#49375=CARTESIAN_POINT('',(57.5,-120.627531126037,69.0669872981078));
#49376=CARTESIAN_POINT('',(57.5,-120.471543313576,68.3421289244415));
#49377=CARTESIAN_POINT('',(57.5,-120.471543313576,68.3421289244415));
#49378=CARTESIAN_POINT('',(58.,-120.218271533617,68.7758457056646));
#49379=CARTESIAN_POINT('Origin',(14.,-120.549537219807,68.7045581112746));
#49380=CARTESIAN_POINT('',(14.2512407024475,-120.549537219807,68.7045581112746));
#49381=CARTESIAN_POINT('',(14.5,-120.471543313576,68.3421289244415));
#49382=CARTESIAN_POINT('',(14.3353834448874,-120.523155809229,68.5819665698912));
#49383=CARTESIAN_POINT('',(14.,-120.471543313576,68.3421289244415));
#49384=CARTESIAN_POINT('',(14.5,-120.627531126037,69.0669872981078));
#49385=CARTESIAN_POINT('',(14.,-120.627531126037,69.0669872981078));
#49386=CARTESIAN_POINT('',(14.4305329766294,-120.605751017473,68.965777505993));
#49387=CARTESIAN_POINT('Origin',(57.75,-119.964059643026,68.2852136377336));
#49388=CARTESIAN_POINT('',(58.,-119.818136807139,68.488207543964));
#49389=CARTESIAN_POINT('',(57.5,-120.109982478913,68.0822197315032));
#49390=CARTESIAN_POINT('Origin',(57.5,-120.127531126037,69.9330127018922));
#49391=CARTESIAN_POINT('',(57.5,-119.421791454066,70.1603524804536));
#49392=CARTESIAN_POINT('',(58.,-119.670765314673,69.7241542943354));
#49393=CARTESIAN_POINT('',(57.5,-119.421791454066,70.1603524804536));
#49394=CARTESIAN_POINT('',(57.5,-120.127531126037,69.9330127018922));
#49395=CARTESIAN_POINT('',(57.5,-120.127531126037,69.9330127018922));
#49396=CARTESIAN_POINT('',(58.,-119.670765314673,69.7241542943354));
#49397=CARTESIAN_POINT('Origin',(14.,-119.774661290051,70.0466825911729));
#49398=CARTESIAN_POINT('',(14.2512407024475,-119.774661290051,70.0466825911729));
#49399=CARTESIAN_POINT('',(14.5,-120.127531126037,69.9330127018922));
#49400=CARTESIAN_POINT('',(14.2590041943422,-119.785673952245,70.0431350845157));
#49401=CARTESIAN_POINT('',(14.,-120.127531126037,69.9330127018922));
#49402=CARTESIAN_POINT('',(14.5,-119.421791454066,70.1603524804536));
#49403=CARTESIAN_POINT('',(14.,-119.421791454066,70.1603524804536));
#49404=CARTESIAN_POINT('',(14.6801520303733,-119.166242342793,70.24267246426));
#49405=CARTESIAN_POINT('Origin',(57.75,-119.911024775091,69.8080127018922));
#49406=CARTESIAN_POINT('',(58.,-119.694518424145,69.6830127018922));
#49407=CARTESIAN_POINT('',(57.5,-120.127531126037,69.9330127018922));
#49408=CARTESIAN_POINT('Origin',(57.75,-117.286708727069,68.9225214538621));
#49409=CARTESIAN_POINT('',(57.5,-117.183872265404,69.1503912898478));
#49410=CARTESIAN_POINT('',(58.,-117.389545188734,68.6946516178765));
#49411=CARTESIAN_POINT('Origin',(14.25,-119.964059643026,68.2852136377336));
#49412=CARTESIAN_POINT('',(14.,-120.218271533617,68.7758457056646));
#49413=CARTESIAN_POINT('',(14.5,-120.877531126037,68.6339745962156));
#49414=CARTESIAN_POINT('',(14.,-119.818136807139,68.488207543964));
#49415=CARTESIAN_POINT('',(14.5,-120.109982478913,68.0822197315032));
#49416=CARTESIAN_POINT('Origin',(14.,-119.877531126037,70.3660254037845));
#49417=CARTESIAN_POINT('',(14.5,-120.127531126037,69.9330127018922));
#49418=CARTESIAN_POINT('Origin',(14.25,-119.911024775091,69.8080127018922));
#49419=CARTESIAN_POINT('',(14.,-119.670765314673,69.7241542943354));
#49420=CARTESIAN_POINT('',(14.,-119.670765314673,69.7241542943354));
#49421=CARTESIAN_POINT('',(14.,-119.694518424145,69.6830127018922));
#49422=CARTESIAN_POINT('Origin',(14.25,-117.286708727069,68.9225214538621));
#49423=CARTESIAN_POINT('',(14.5,-117.183872265404,69.1503912898478));
#49424=CARTESIAN_POINT('',(14.,-117.389545188734,68.6946516178765));
#49425=CARTESIAN_POINT('Origin',(14.,-116.213429510899,68.7124355652982));
#49426=CARTESIAN_POINT('Origin',(14.,-120.877531126037,68.6339745962156));
#49427=CARTESIAN_POINT('Origin',(57.5,-125.765473267224,59.1970922754756));
#49428=CARTESIAN_POINT('',(57.5,-125.08223311503,59.4850762228408));
#49429=CARTESIAN_POINT('',(58.,-125.292242378034,59.0288384007668));
#49430=CARTESIAN_POINT('',(57.5,-125.08223311503,59.4850762228408));
#49431=CARTESIAN_POINT('',(57.5,-125.765473267224,59.1970922754756));
#49432=CARTESIAN_POINT('',(57.5,-125.765473267224,59.1970922754756));
#49433=CARTESIAN_POINT('',(58.,-125.292242378034,59.0288384007668));
#49434=CARTESIAN_POINT('Origin',(57.5,-125.969521727281,57.5822796533797));
#49435=CARTESIAN_POINT('',(57.5,-126.188091528965,58.2907844884389));
#49436=CARTESIAN_POINT('',(58.,-125.755014631118,58.036420101407));
#49437=CARTESIAN_POINT('',(57.5,-126.188091528965,58.2907844884389));
#49438=CARTESIAN_POINT('',(57.5,-125.969521727281,57.5822796533797));
#49439=CARTESIAN_POINT('',(57.5,-125.969521727281,57.5822796533797));
#49440=CARTESIAN_POINT('',(58.,-125.755014631118,58.036420101407));
#49441=CARTESIAN_POINT('Origin',(14.,-125.292242378034,59.0288384007668));
#49442=CARTESIAN_POINT('',(14.5,-125.08223311503,59.4850762228408));
#49443=CARTESIAN_POINT('',(14.5,-125.765473267224,59.1970922754756));
#49444=CARTESIAN_POINT('',(14.5,-125.08223311503,59.4850762228408));
#49445=CARTESIAN_POINT('',(14.,-125.292242378034,59.0288384007668));
#49446=CARTESIAN_POINT('',(14.,-125.292242378034,59.0288384007668));
#49447=CARTESIAN_POINT('',(14.5,-125.765473267224,59.1970922754756));
#49448=CARTESIAN_POINT('Origin',(14.25,-122.84739093989,58.4380402379161));
#49449=CARTESIAN_POINT('',(14.,-122.929975912966,58.2020747272541));
#49450=CARTESIAN_POINT('',(14.5,-122.764805966813,58.674005748578));
#49451=CARTESIAN_POINT('Origin',(14.5,-125.969521727281,57.5822796533797));
#49452=CARTESIAN_POINT('',(14.,-125.755014631118,58.036420101407));
#49453=CARTESIAN_POINT('',(14.5,-126.188091528965,58.2907844884389));
#49454=CARTESIAN_POINT('',(14.,-125.755014631118,58.036420101407));
#49455=CARTESIAN_POINT('',(14.5,-125.969521727281,57.5822796533797));
#49456=CARTESIAN_POINT('',(14.5,-125.969521727281,57.5822796533797));
#49457=CARTESIAN_POINT('',(14.5,-126.188091528965,58.2907844884389));
#49458=CARTESIAN_POINT('Origin',(14.25,-125.459008691224,57.56981106276));
#49459=CARTESIAN_POINT('',(14.5,-125.586684161994,57.3548715964828));
#49460=CARTESIAN_POINT('',(14.,-125.331333220453,57.7847505290373));
#49461=CARTESIAN_POINT('Origin',(14.,-126.078806628123,57.9365320709093));
#49462=CARTESIAN_POINT('',(14.,-126.188091528965,58.2907844884389));
#49463=CARTESIAN_POINT('',(14.,-125.969521727281,57.5822796533797));
#49464=CARTESIAN_POINT('Origin',(14.25,-125.538896320465,59.0914377100404));
#49465=CARTESIAN_POINT('',(14.5,-125.765473267224,59.1970922754756));
#49466=CARTESIAN_POINT('',(14.,-125.312319373706,58.9857831446052));
#49467=CARTESIAN_POINT('Origin',(14.,-125.423853191127,59.3410842491582));
#49468=CARTESIAN_POINT('',(14.,-125.08223311503,59.4850762228408));
#49469=CARTESIAN_POINT('',(14.,-125.765473267224,59.1970922754756));
#49470=CARTESIAN_POINT('Origin',(57.75,-125.459008691224,57.56981106276));
#49471=CARTESIAN_POINT('',(58.,-125.331333220453,57.7847505290373));
#49472=CARTESIAN_POINT('',(57.5,-125.586684161994,57.3548715964828));
#49473=CARTESIAN_POINT('Origin',(57.75,-125.538896320465,59.0914377100404));
#49474=CARTESIAN_POINT('',(58.,-125.312319373706,58.9857831446052));
#49475=CARTESIAN_POINT('',(57.5,-125.765473267224,59.1970922754756));
#49476=CARTESIAN_POINT('Origin',(57.75,-122.84739093989,58.4380402379161));
#49477=CARTESIAN_POINT('',(57.5,-122.764805966813,58.674005748578));
#49478=CARTESIAN_POINT('',(58.,-122.929975912966,58.2020747272541));
#49479=CARTESIAN_POINT('Origin',(14.,-124.164166824021,57.8987018584758));
#49480=CARTESIAN_POINT('Origin',(14.,-121.759885683511,58.3222962368457));
#49481=CARTESIAN_POINT('Origin',(14.,-125.554164136354,59.6502461689939));
#49482=CARTESIAN_POINT('Origin',(57.5,-130.446264217578,48.0106462326609));
#49483=CARTESIAN_POINT('',(57.5,-129.790723455271,48.3570826171013));
#49484=CARTESIAN_POINT('',(58.,-129.960169823373,47.8842774043812));
#49485=CARTESIAN_POINT('',(57.5,-129.790723455271,48.3570826171013));
#49486=CARTESIAN_POINT('',(57.5,-130.446264217578,48.0106462326609));
#49487=CARTESIAN_POINT('',(57.5,-130.446264217578,48.0106462326609));
#49488=CARTESIAN_POINT('',(58.,-129.960169823373,47.8842774043812));
#49489=CARTESIAN_POINT('Origin',(57.5,-130.508796018164,46.3841944650247));
#49490=CARTESIAN_POINT('',(57.5,-130.788284360904,47.070953611875));
#49491=CARTESIAN_POINT('',(58.,-130.334686134323,46.8553022968291));
#49492=CARTESIAN_POINT('',(57.5,-130.788284360904,47.070953611875));
#49493=CARTESIAN_POINT('',(57.5,-130.508796018164,46.3841944650247));
#49494=CARTESIAN_POINT('',(57.5,-130.508796018164,46.3841944650247));
#49495=CARTESIAN_POINT('',(58.,-130.334686134323,46.8553022968291));
#49496=CARTESIAN_POINT('Origin',(14.,-129.960169823373,47.8842774043812));
#49497=CARTESIAN_POINT('',(14.5,-129.790723455271,48.3570826171013));
#49498=CARTESIAN_POINT('',(14.5,-130.446264217578,48.0106462326609));
#49499=CARTESIAN_POINT('',(14.5,-129.790723455271,48.3570826171013));
#49500=CARTESIAN_POINT('',(14.,-129.960169823373,47.8842774043812));
#49501=CARTESIAN_POINT('',(14.,-129.960169823373,47.8842774043812));
#49502=CARTESIAN_POINT('',(14.5,-130.446264217578,48.0106462326609));
#49503=CARTESIAN_POINT('Origin',(14.25,-127.473130330375,47.5088102499061));
#49504=CARTESIAN_POINT('',(14.,-127.534835293351,47.2665449045839));
#49505=CARTESIAN_POINT('',(14.5,-127.411425367399,47.7510755952283));
#49506=CARTESIAN_POINT('Origin',(14.5,-130.508796018164,46.3841944650247));
#49507=CARTESIAN_POINT('',(14.,-130.334686134323,46.8553022968291));
#49508=CARTESIAN_POINT('',(14.5,-130.788284360904,47.070953611875));
#49509=CARTESIAN_POINT('',(14.,-130.334686134323,46.8553022968291));
#49510=CARTESIAN_POINT('',(14.5,-130.508796018164,46.3841944650247));
#49511=CARTESIAN_POINT('',(14.5,-130.508796018164,46.3841944650247));
#49512=CARTESIAN_POINT('',(14.5,-130.788284360904,47.070953611875));
#49513=CARTESIAN_POINT('Origin',(14.25,-129.99913892906,46.4162674639966));
#49514=CARTESIAN_POINT('',(14.5,-130.107595347289,46.1910182567949));
#49515=CARTESIAN_POINT('',(14.,-129.890682510832,46.6415166711983));
#49516=CARTESIAN_POINT('Origin',(14.,-130.648540189534,46.7275740384498));
#49517=CARTESIAN_POINT('',(14.,-130.788284360904,47.070953611875));
#49518=CARTESIAN_POINT('',(14.,-130.508796018164,46.3841944650247));
#49519=CARTESIAN_POINT('Origin',(14.25,-130.211341062382,47.9251411968295));
#49520=CARTESIAN_POINT('',(14.5,-130.446264217578,48.0106462326609));
#49521=CARTESIAN_POINT('',(14.,-129.976417907185,47.8396361609981));
#49522=CARTESIAN_POINT('Origin',(14.,-130.118493836425,48.1838644248811));
#49523=CARTESIAN_POINT('',(14.,-129.790723455271,48.3570826171013));
#49524=CARTESIAN_POINT('',(14.,-130.446264217578,48.0106462326609));
#49525=CARTESIAN_POINT('Origin',(57.75,-129.99913892906,46.4162674639966));
#49526=CARTESIAN_POINT('',(58.,-129.890682510832,46.6415166711983));
#49527=CARTESIAN_POINT('',(57.5,-130.107595347289,46.1910182567949));
#49528=CARTESIAN_POINT('Origin',(57.75,-130.211341062382,47.9251411968295));
#49529=CARTESIAN_POINT('',(58.,-129.976417907185,47.8396361609981));
#49530=CARTESIAN_POINT('',(57.5,-130.446264217578,48.0106462326609));
#49531=CARTESIAN_POINT('Origin',(57.75,-127.473130330375,47.5088102499061));
#49532=CARTESIAN_POINT('',(57.5,-127.411425367399,47.7510755952283));
#49533=CARTESIAN_POINT('',(58.,-127.534835293351,47.2665449045839));
#49534=CARTESIAN_POINT('Origin',(14.,-128.737889047669,46.8567596356166));
#49535=CARTESIAN_POINT('Origin',(14.,-126.379675605442,47.4882890180656));
#49536=CARTESIAN_POINT('Origin',(14.,-130.275254145916,48.4804925430539));
#49537=CARTESIAN_POINT('Origin',(57.75,-131.128722228666,36.2180095292903));
#49538=CARTESIAN_POINT('',(57.7487592975525,-133.822854175933,36.6599362981178));
#49539=CARTESIAN_POINT('',(58.,-133.639021904261,36.375288143631));
#49540=CARTESIAN_POINT('',(58.2319907935076,-133.469274748797,36.1124495566242));
#49541=CARTESIAN_POINT('',(58.,-131.169077569515,35.9712881348696));
#49542=CARTESIAN_POINT('',(57.5,-133.511428020236,36.8610624138407));
#49543=CARTESIAN_POINT('',(57.5,-131.088366887817,36.4647309237111));
#49544=CARTESIAN_POINT('',(50.4896657310026,-124.735066802703,42.5290366978776));
#49545=CARTESIAN_POINT('Origin',(58.,-132.331838201602,35.4582091790453));
#49546=CARTESIAN_POINT('',(58.,-133.922431977811,35.3175873497673));
#49547=CARTESIAN_POINT('',(58.,-133.651317418485,36.3294006598437));
#49548=CARTESIAN_POINT('',(58.,-133.461485277164,35.1433127085737));
#49549=CARTESIAN_POINT('Origin',(57.75,-133.892798875057,36.3941054211193));
#49550=CARTESIAN_POINT('',(57.5,-134.134280331629,36.4588101823949));
#49551=CARTESIAN_POINT('',(57.5,-134.134280331629,36.4588101823949));
#49552=CARTESIAN_POINT('',(57.5,-134.393099376732,35.4928843561059));
#49553=CARTESIAN_POINT('',(57.5,-134.134280331629,36.4588101823949));
#49554=CARTESIAN_POINT('',(57.5,-134.393099376732,35.4928843561059));
#49555=CARTESIAN_POINT('Origin',(14.,-133.822854175933,36.6599362981178));
#49556=CARTESIAN_POINT('',(14.5,-133.511428020236,36.8610624138407));
#49557=CARTESIAN_POINT('',(14.,-133.511428020236,36.8610624138407));
#49558=CARTESIAN_POINT('',(14.5,-134.134280331629,36.4588101823949));
#49559=CARTESIAN_POINT('',(14.5,-133.511428020236,36.8610624138407));
#49560=CARTESIAN_POINT('',(14.,-134.134280331629,36.4588101823949));
#49561=CARTESIAN_POINT('Origin',(57.5,-134.054819567983,34.8330975492484));
#49562=CARTESIAN_POINT('',(57.5,-134.054819567983,34.8330975492484));
#49563=CARTESIAN_POINT('',(57.5,-134.054819567983,34.8330975492484));
#49564=CARTESIAN_POINT('',(58.,-133.922431977811,35.3175873497673));
#49565=CARTESIAN_POINT('Origin',(14.,-133.639021904261,36.375288143631));
#49566=CARTESIAN_POINT('',(14.,-133.639021904261,36.375288143631));
#49567=CARTESIAN_POINT('',(14.,-133.639021904261,36.375288143631));
#49568=CARTESIAN_POINT('',(14.5,-134.134280331629,36.4588101823949));
#49569=CARTESIAN_POINT('Origin',(14.25,-131.128722228666,36.2180095292903));
#49570=CARTESIAN_POINT('',(14.,-131.169077569515,35.9712881348696));
#49571=CARTESIAN_POINT('',(14.5,-131.088366887817,36.4647309237111));
#49572=CARTESIAN_POINT('Origin',(14.5,-134.054819567983,34.8330975492484));
#49573=CARTESIAN_POINT('',(14.,-133.922431977811,35.3175873497673));
#49574=CARTESIAN_POINT('',(14.5,-134.393099376732,35.4928843561059));
#49575=CARTESIAN_POINT('',(14.,-133.922431977811,35.3175873497673));
#49576=CARTESIAN_POINT('',(14.5,-134.054819567983,34.8330975492484));
#49577=CARTESIAN_POINT('',(14.5,-134.054819567983,34.8330975492484));
#49578=CARTESIAN_POINT('',(14.5,-134.393099376732,35.4928843561059));
#49579=CARTESIAN_POINT('Origin',(14.25,-133.549897224021,34.9094680429235));
#49580=CARTESIAN_POINT('',(14.5,-133.638309170877,34.6756233772733));
#49581=CARTESIAN_POINT('',(14.,-133.461485277164,35.1433127085737));
#49582=CARTESIAN_POINT('Origin',(14.,-134.223959472357,35.1629909526771));
#49583=CARTESIAN_POINT('',(14.,-134.393099376732,35.4928843561059));
#49584=CARTESIAN_POINT('',(14.,-134.054819567983,34.8330975492484));
#49585=CARTESIAN_POINT('Origin',(14.25,-133.892798875057,36.3941054211193));
#49586=CARTESIAN_POINT('',(14.5,-134.134280331629,36.4588101823949));
#49587=CARTESIAN_POINT('',(14.,-133.651317418485,36.3294006598437));
#49588=CARTESIAN_POINT('Origin',(57.75,-133.549897224021,34.9094680429235));
#49589=CARTESIAN_POINT('',(57.5,-133.638309170877,34.6756233772733));
#49590=CARTESIAN_POINT('Origin',(14.,-130.037639885881,36.292867245645));
#49591=CARTESIAN_POINT('Origin',(14.,-134.004870809078,36.9417730955394));
#49592=CARTESIAN_POINT('Origin',(57.5,-136.801453579863,24.6295005722094));
#49593=CARTESIAN_POINT('',(57.5,-136.216030001563,25.0845072682929));
#49594=CARTESIAN_POINT('',(58.,-136.30080033501,24.5894609761083));
#49595=CARTESIAN_POINT('',(57.5,-136.216030001563,25.0845072682929));
#49596=CARTESIAN_POINT('',(57.5,-136.801453579863,24.6295005722094));
#49597=CARTESIAN_POINT('',(57.5,-136.801453579863,24.6295005722094));
#49598=CARTESIAN_POINT('',(58.,-136.30080033501,24.5894609761083));
#49599=CARTESIAN_POINT('Origin',(57.5,-136.580604996376,23.016899728323));
#49600=CARTESIAN_POINT('',(57.5,-136.97510175753,23.6446928191972));
#49601=CARTESIAN_POINT('',(58.,-136.490947249372,23.5110842376315));
#49602=CARTESIAN_POINT('',(57.5,-136.97510175753,23.6446928191972));
#49603=CARTESIAN_POINT('',(57.5,-136.580604996376,23.016899728323));
#49604=CARTESIAN_POINT('',(57.5,-136.580604996376,23.016899728323));
#49605=CARTESIAN_POINT('',(58.,-136.490947249372,23.5110842376315));
#49606=CARTESIAN_POINT('Origin',(14.,-136.30080033501,24.5894609761083));
#49607=CARTESIAN_POINT('',(14.5,-136.216030001563,25.0845072682929));
#49608=CARTESIAN_POINT('',(14.5,-136.801453579863,24.6295005722094));
#49609=CARTESIAN_POINT('',(14.5,-136.216030001563,25.0845072682929));
#49610=CARTESIAN_POINT('',(14.,-136.30080033501,24.5894609761083));
#49611=CARTESIAN_POINT('',(14.,-136.30080033501,24.5894609761083));
#49612=CARTESIAN_POINT('',(14.5,-136.801453579863,24.6295005722094));
#49613=CARTESIAN_POINT('Origin',(14.25,-133.786345373109,24.6515678871246));
#49614=CARTESIAN_POINT('',(14.,-133.805043963321,24.4022681423913));
#49615=CARTESIAN_POINT('',(14.5,-133.767646782898,24.900867631858));
#49616=CARTESIAN_POINT('Origin',(14.5,-136.580604996376,23.016899728323));
#49617=CARTESIAN_POINT('',(14.,-136.490947249372,23.5110842376315));
#49618=CARTESIAN_POINT('',(14.5,-136.97510175753,23.6446928191972));
#49619=CARTESIAN_POINT('',(14.,-136.490947249372,23.5110842376315));
#49620=CARTESIAN_POINT('',(14.5,-136.580604996376,23.016899728323));
#49621=CARTESIAN_POINT('',(14.5,-136.580604996376,23.016899728323));
#49622=CARTESIAN_POINT('',(14.5,-136.97510175753,23.6446928191972));
#49623=CARTESIAN_POINT('Origin',(14.25,-136.084260161474,23.1369864911307));
#49624=CARTESIAN_POINT('',(14.5,-136.151954768658,22.8963260661369));
#49625=CARTESIAN_POINT('',(14.,-136.01656555429,23.3776469161245));
#49626=CARTESIAN_POINT('Origin',(14.,-136.777853376953,23.3307962737601));
#49627=CARTESIAN_POINT('',(14.,-136.97510175753,23.6446928191972));
#49628=CARTESIAN_POINT('',(14.,-136.580604996376,23.016899728323));
#49629=CARTESIAN_POINT('Origin',(14.25,-136.55525164161,24.5860885277927));
#49630=CARTESIAN_POINT('',(14.5,-136.801453579863,24.6295005722094));
#49631=CARTESIAN_POINT('',(14.,-136.309049703357,24.542676483376));
#49632=CARTESIAN_POINT('Origin',(14.,-136.508741790713,24.8570039202512));
#49633=CARTESIAN_POINT('',(14.,-136.216030001563,25.0845072682929));
#49634=CARTESIAN_POINT('',(14.,-136.801453579863,24.6295005722094));
#49635=CARTESIAN_POINT('Origin',(57.75,-136.084260161474,23.1369864911307));
#49636=CARTESIAN_POINT('',(58.,-136.01656555429,23.3776469161245));
#49637=CARTESIAN_POINT('',(57.5,-136.151954768658,22.8963260661369));
#49638=CARTESIAN_POINT('Origin',(57.75,-136.55525164161,24.5860885277927));
#49639=CARTESIAN_POINT('',(58.,-136.309049703357,24.542676483376));
#49640=CARTESIAN_POINT('',(57.5,-136.801453579863,24.6295005722094));
#49641=CARTESIAN_POINT('Origin',(57.75,-133.786345373109,24.6515678871246));
#49642=CARTESIAN_POINT('',(57.5,-133.767646782898,24.900867631858));
#49643=CARTESIAN_POINT('',(58.,-133.805043963321,24.4022681423913));
#49644=CARTESIAN_POINT('Origin',(14.,-134.918662162673,23.7898003403695));
#49645=CARTESIAN_POINT('Origin',(14.,-132.705939207914,24.8212348392527));
#49646=CARTESIAN_POINT('Origin',(14.,-136.71462949103,25.1219044487155));
#49647=CARTESIAN_POINT('Origin',(57.5,-138.066929551123,11.0255294024811));
#49648=CARTESIAN_POINT('',(57.5,-138.514640906126,11.6165508928786));
#49649=CARTESIAN_POINT('',(58.,-138.020683996878,11.5256475780665));
#49650=CARTESIAN_POINT('',(57.5,-138.514640906126,11.6165508928786));
#49651=CARTESIAN_POINT('',(57.5,-138.066929551123,11.0255294024811));
#49652=CARTESIAN_POINT('',(57.5,-138.066929551123,11.0255294024811));
#49653=CARTESIAN_POINT('',(58.,-138.020683996878,11.5256475780665));
#49654=CARTESIAN_POINT('Origin',(14.,-138.290785228625,11.3210401476799));
#49655=CARTESIAN_POINT('',(14.2512407024475,-138.290785228625,11.3210401476798));
#49656=CARTESIAN_POINT('',(14.5,-138.066929551123,11.0255294024811));
#49657=CARTESIAN_POINT('',(14.3353834448875,-138.215066126661,11.22108374498));
#49658=CARTESIAN_POINT('',(14.,-138.066929551123,11.0255294024811));
#49659=CARTESIAN_POINT('',(14.5,-138.514640906126,11.6165508928786));
#49660=CARTESIAN_POINT('',(14.,-138.514640906126,11.6165508928786));
#49661=CARTESIAN_POINT('',(14.4305329766294,-138.452128317718,11.5340283417823));
#49662=CARTESIAN_POINT('Origin',(57.75,-137.582939709175,11.188418501646));
#49663=CARTESIAN_POINT('',(58.,-137.536477638499,11.4340631148345));
#49664=CARTESIAN_POINT('',(57.5,-137.629401779851,10.9427738884575));
#49665=CARTESIAN_POINT('Origin',(57.5,-138.427485163379,12.6127455909704));
#49666=CARTESIAN_POINT('',(57.5,-137.883945745091,13.1170438759937));
#49667=CARTESIAN_POINT('',(58.,-137.925247374536,12.6164931630349));
#49668=CARTESIAN_POINT('',(57.5,-137.883945745091,13.1170438759937));
#49669=CARTESIAN_POINT('',(57.5,-138.427485163379,12.6127455909704));
#49670=CARTESIAN_POINT('',(57.5,-138.427485163379,12.6127455909704));
#49671=CARTESIAN_POINT('',(58.,-137.925247374536,12.6164931630349));
#49672=CARTESIAN_POINT('Origin',(14.,-138.155715454235,12.864894733482));
#49673=CARTESIAN_POINT('',(14.2512407024475,-138.155715454235,12.864894733482));
#49674=CARTESIAN_POINT('',(14.5,-138.427485163379,12.6127455909704));
#49675=CARTESIAN_POINT('',(14.2590041943422,-138.16419707464,12.8570254484205));
#49676=CARTESIAN_POINT('',(14.,-138.427485163379,12.6127455909704));
#49677=CARTESIAN_POINT('',(14.5,-137.883945745091,13.1170438759937));
#49678=CARTESIAN_POINT('',(14.,-137.883945745091,13.1170438759937));
#49679=CARTESIAN_POINT('',(14.6801520303733,-137.687129524037,13.2996508395415));
#49680=CARTESIAN_POINT('Origin',(57.75,-138.178436488856,12.5909566552835));
#49681=CARTESIAN_POINT('',(58.,-137.929387814333,12.5691677195966));
#49682=CARTESIAN_POINT('',(57.5,-138.427485163379,12.6127455909704));
#49683=CARTESIAN_POINT('Origin',(57.75,-135.425773646859,12.8975129283142));
#49684=CARTESIAN_POINT('',(57.5,-135.428874114848,13.1474937017714));
#49685=CARTESIAN_POINT('',(58.,-135.422673178871,12.647532154857));
#49686=CARTESIAN_POINT('Origin',(14.25,-137.582939709175,11.188418501646));
#49687=CARTESIAN_POINT('',(14.,-138.020683996878,11.5256475780665));
#49688=CARTESIAN_POINT('',(14.5,-138.5582187775,11.1184535438328));
#49689=CARTESIAN_POINT('',(14.,-137.536477638499,11.4340631148345));
#49690=CARTESIAN_POINT('',(14.5,-137.629401779851,10.9427738884575));
#49691=CARTESIAN_POINT('Origin',(14.,-138.383907292005,13.1108429400163));
#49692=CARTESIAN_POINT('',(14.5,-138.427485163379,12.6127455909704));
#49693=CARTESIAN_POINT('Origin',(14.25,-138.178436488856,12.5909566552835));
#49694=CARTESIAN_POINT('',(14.,-137.925247374536,12.6164931630349));
#49695=CARTESIAN_POINT('',(14.,-137.925247374536,12.6164931630349));
#49696=CARTESIAN_POINT('',(14.,-137.929387814333,12.5691677195966));
#49697=CARTESIAN_POINT('Origin',(14.25,-135.425773646859,12.8975129283142));
#49698=CARTESIAN_POINT('',(14.5,-135.428874114848,13.1474937017714));
#49699=CARTESIAN_POINT('',(14.,-135.422673178871,12.647532154857));
#49700=CARTESIAN_POINT('Origin',(14.,-134.364266202539,13.1606978482623));
#49701=CARTESIAN_POINT('Origin',(14.,-138.5582187775,11.1184535438328));
#49702=CARTESIAN_POINT('Origin',(57.5,-139.,0.500000000000008));
#49703=CARTESIAN_POINT('',(57.5,-138.502481404895,1.04975185951051));
#49704=CARTESIAN_POINT('',(58.,-138.5,0.547506218943965));
#49705=CARTESIAN_POINT('',(57.5,-138.502481404895,1.04975185951051));
#49706=CARTESIAN_POINT('',(57.5,-139.,0.500000000000008));
#49707=CARTESIAN_POINT('',(57.5,-139.,0.500000000000008));
#49708=CARTESIAN_POINT('',(58.,-138.5,0.547506218943965));
#49709=CARTESIAN_POINT('Origin',(57.5,-138.502481404895,-1.04975185951049));
#49710=CARTESIAN_POINT('',(57.5,-139.,-0.499999999999992));
#49711=CARTESIAN_POINT('',(58.,-138.5,-0.547506218943948));
#49712=CARTESIAN_POINT('',(57.5,-139.,-0.499999999999992));
#49713=CARTESIAN_POINT('',(57.5,-138.502481404895,-1.04975185951049));
#49714=CARTESIAN_POINT('',(57.5,-138.502481404895,-1.04975185951049));
#49715=CARTESIAN_POINT('',(58.,-138.5,-0.547506218943948));
#49716=CARTESIAN_POINT('Origin',(14.,-138.5,0.547506218943967));
#49717=CARTESIAN_POINT('',(14.5,-138.502481404895,1.04975185951051));
#49718=CARTESIAN_POINT('',(14.5,-139.,0.500000000000008));
#49719=CARTESIAN_POINT('',(14.5,-138.502481404895,1.04975185951051));
#49720=CARTESIAN_POINT('',(14.,-138.5,0.547506218943967));
#49721=CARTESIAN_POINT('',(14.,-138.5,0.547506218943967));
#49722=CARTESIAN_POINT('',(14.5,-139.,0.500000000000008));
#49723=CARTESIAN_POINT('Origin',(14.25,-136.034530010839,1.0453001083881));
#49724=CARTESIAN_POINT('',(14.,-136.009654081084,0.796540810835608));
#49725=CARTESIAN_POINT('',(14.5,-136.059405940594,1.2940594059406));
#49726=CARTESIAN_POINT('Origin',(14.5,-138.502481404895,-1.04975185951049));
#49727=CARTESIAN_POINT('',(14.,-138.5,-0.547506218943949));
#49728=CARTESIAN_POINT('',(14.5,-139.,-0.499999999999992));
#49729=CARTESIAN_POINT('',(14.,-138.5,-0.547506218943949));
#49730=CARTESIAN_POINT('',(14.5,-138.502481404895,-1.04975185951049));
#49731=CARTESIAN_POINT('',(14.5,-138.502481404895,-1.04975185951049));
#49732=CARTESIAN_POINT('',(14.5,-139.,-0.499999999999992));
#49733=CARTESIAN_POINT('Origin',(14.25,-138.034530010839,-0.845300108388089));
#49734=CARTESIAN_POINT('',(14.5,-138.059405940594,-1.09405940594059));
#49735=CARTESIAN_POINT('',(14.,-138.009654081084,-0.596540810835591));
#49736=CARTESIAN_POINT('Origin',(14.,-138.751240702448,-0.774875929755241));
#49737=CARTESIAN_POINT('',(14.,-139.,-0.499999999999992));
#49738=CARTESIAN_POINT('',(14.,-138.502481404895,-1.04975185951049));
#49739=CARTESIAN_POINT('Origin',(14.25,-138.75,0.500000000000008));
#49740=CARTESIAN_POINT('',(14.5,-139.,0.500000000000008));
#49741=CARTESIAN_POINT('',(14.,-138.5,0.500000000000008));
#49742=CARTESIAN_POINT('Origin',(14.,-138.751240702448,0.774875929755257));
#49743=CARTESIAN_POINT('',(14.,-138.502481404895,1.04975185951051));
#49744=CARTESIAN_POINT('',(14.,-139.,0.500000000000008));
#49745=CARTESIAN_POINT('Origin',(57.75,-138.034530010839,-0.845300108388089));
#49746=CARTESIAN_POINT('',(58.,-138.009654081084,-0.596540810835592));
#49747=CARTESIAN_POINT('',(57.5,-138.059405940594,-1.09405940594059));
#49748=CARTESIAN_POINT('Origin',(57.75,-138.75,0.500000000000008));
#49749=CARTESIAN_POINT('',(58.,-138.5,0.500000000000008));
#49750=CARTESIAN_POINT('',(57.5,-139.,0.500000000000008));
#49751=CARTESIAN_POINT('Origin',(57.75,-136.034530010839,1.0453001083881));
#49752=CARTESIAN_POINT('',(57.5,-136.059405940594,1.2940594059406));
#49753=CARTESIAN_POINT('',(58.,-136.009654081084,0.796540810835608));
#49754=CARTESIAN_POINT('Origin',(14.,-137.,8.38883057415937E-15));
#49755=CARTESIAN_POINT('Origin',(14.,-135.,1.40000000000001));
#49756=CARTESIAN_POINT('Origin',(14.,-139.,1.00000000000001));
#49757=CARTESIAN_POINT('Origin',(57.5,-138.514640906126,-11.6165508928786));
#49758=CARTESIAN_POINT('',(57.5,-138.066929551123,-11.025529402481));
#49759=CARTESIAN_POINT('',(58.,-138.020683996878,-11.5256475780664));
#49760=CARTESIAN_POINT('',(57.5,-138.066929551123,-11.025529402481));
#49761=CARTESIAN_POINT('',(57.5,-138.514640906126,-11.6165508928786));
#49762=CARTESIAN_POINT('',(57.5,-138.514640906126,-11.6165508928786));
#49763=CARTESIAN_POINT('',(58.,-138.020683996878,-11.5256475780664));
#49764=CARTESIAN_POINT('Origin',(57.5,-137.883945745091,-13.1170438759936));
#49765=CARTESIAN_POINT('',(57.5,-138.427485163379,-12.6127455909703));
#49766=CARTESIAN_POINT('',(58.,-137.925247374536,-12.6164931630349));
#49767=CARTESIAN_POINT('',(57.5,-138.427485163379,-12.6127455909703));
#49768=CARTESIAN_POINT('',(57.5,-137.883945745091,-13.1170438759936));
#49769=CARTESIAN_POINT('',(57.5,-137.883945745091,-13.1170438759936));
#49770=CARTESIAN_POINT('',(58.,-137.925247374536,-12.6164931630349));
#49771=CARTESIAN_POINT('Origin',(14.,-138.020683996878,-11.5256475780664));
#49772=CARTESIAN_POINT('',(14.5,-138.066929551123,-11.025529402481));
#49773=CARTESIAN_POINT('',(14.5,-138.514640906126,-11.6165508928786));
#49774=CARTESIAN_POINT('',(14.5,-138.066929551123,-11.025529402481));
#49775=CARTESIAN_POINT('',(14.,-138.020683996878,-11.5256475780664));
#49776=CARTESIAN_POINT('',(14.,-138.020683996878,-11.5256475780664));
#49777=CARTESIAN_POINT('',(14.5,-138.514640906126,-11.6165508928786));
#49778=CARTESIAN_POINT('Origin',(14.25,-135.607981461541,-10.8148680765323));
#49779=CARTESIAN_POINT('',(14.,-135.561519390865,-11.0605126897207));
#49780=CARTESIAN_POINT('',(14.5,-135.654443532217,-10.5692234633438));
#49781=CARTESIAN_POINT('Origin',(14.5,-137.883945745091,-13.1170438759936));
#49782=CARTESIAN_POINT('',(14.,-137.925247374536,-12.6164931630349));
#49783=CARTESIAN_POINT('',(14.5,-138.427485163379,-12.6127455909703));
#49784=CARTESIAN_POINT('',(14.,-137.925247374536,-12.6164931630349));
#49785=CARTESIAN_POINT('',(14.5,-137.883945745091,-13.1170438759936));
#49786=CARTESIAN_POINT('',(14.5,-137.883945745091,-13.1170438759936));
#49787=CARTESIAN_POINT('',(14.5,-138.427485163379,-12.6127455909703));
#49788=CARTESIAN_POINT('Origin',(14.25,-137.435594191592,-12.8725854741911));
#49789=CARTESIAN_POINT('',(14.5,-137.438694659581,-13.1225662476483));
#49790=CARTESIAN_POINT('',(14.,-137.432493723604,-12.622604700734));
#49791=CARTESIAN_POINT('Origin',(14.,-138.155715454235,-12.864894733482));
#49792=CARTESIAN_POINT('',(14.,-138.427485163379,-12.6127455909703));
#49793=CARTESIAN_POINT('',(14.,-137.883945745091,-13.1170438759936));
#49794=CARTESIAN_POINT('Origin',(14.25,-138.265592231604,-11.5947619571917));
#49795=CARTESIAN_POINT('',(14.5,-138.514640906126,-11.6165508928786));
#49796=CARTESIAN_POINT('',(14.,-138.016543557081,-11.5729730215048));
#49797=CARTESIAN_POINT('Origin',(14.,-138.290785228625,-11.3210401476798));
#49798=CARTESIAN_POINT('',(14.,-138.066929551123,-11.025529402481));
#49799=CARTESIAN_POINT('',(14.,-138.514640906126,-11.6165508928786));
#49800=CARTESIAN_POINT('Origin',(57.75,-137.435594191592,-12.8725854741911));
#49801=CARTESIAN_POINT('',(58.,-137.432493723604,-12.622604700734));
#49802=CARTESIAN_POINT('',(57.5,-137.438694659581,-13.1225662476483));
#49803=CARTESIAN_POINT('Origin',(57.75,-138.265592231604,-11.5947619571917));
#49804=CARTESIAN_POINT('',(58.,-138.016543557081,-11.5729730215048));
#49805=CARTESIAN_POINT('',(57.5,-138.514640906126,-11.6165508928786));
#49806=CARTESIAN_POINT('Origin',(57.75,-135.607981461541,-10.8148680765323));
#49807=CARTESIAN_POINT('',(57.5,-135.654443532217,-10.5692234633438));
#49808=CARTESIAN_POINT('',(58.,-135.561519390865,-11.0605126897207));
#49809=CARTESIAN_POINT('Origin',(14.,-136.478673638569,-11.9403367564291));
#49810=CARTESIAN_POINT('Origin',(14.,-134.608302282232,-10.3713526936054));
#49811=CARTESIAN_POINT('Origin',(14.,-138.5582187775,-11.1184535438327));
#49812=CARTESIAN_POINT('Origin',(57.75,-134.149374290983,-22.5927285851944));
#49813=CARTESIAN_POINT('',(57.7487592975525,-136.777853376953,-23.3307962737601));
#49814=CARTESIAN_POINT('',(58.,-136.490947249372,-23.5110842376314));
#49815=CARTESIAN_POINT('',(58.2319907935076,-136.226023693788,-23.6775586479915));
#49816=CARTESIAN_POINT('',(58.,-134.081679683799,-22.8333890101882));
#49817=CARTESIAN_POINT('',(57.5,-136.580604996376,-23.016899728323));
#49818=CARTESIAN_POINT('',(57.5,-134.217068898167,-22.3520681602006));
#49819=CARTESIAN_POINT('',(50.4896657310027,-131.02190992259,-14.1709199758145));
#49820=CARTESIAN_POINT('Origin',(58.,-134.918662162673,-23.7898003403695));
#49821=CARTESIAN_POINT('',(58.,-136.30080033501,-24.5894609761083));
#49822=CARTESIAN_POINT('',(58.,-136.482697881024,-23.5578687303638));
#49823=CARTESIAN_POINT('',(58.,-135.809389104878,-24.5526029471227));
#49824=CARTESIAN_POINT('Origin',(57.75,-136.728899819277,-23.6012807747805));
#49825=CARTESIAN_POINT('',(57.5,-136.97510175753,-23.6446928191972));
#49826=CARTESIAN_POINT('',(57.5,-136.97510175753,-23.6446928191972));
#49827=CARTESIAN_POINT('',(57.5,-136.801453579863,-24.6295005722094));
#49828=CARTESIAN_POINT('',(57.5,-136.97510175753,-23.6446928191972));
#49829=CARTESIAN_POINT('',(57.5,-136.801453579863,-24.6295005722094));
#49830=CARTESIAN_POINT('Origin',(14.,-136.777853376953,-23.3307962737601));
#49831=CARTESIAN_POINT('',(14.5,-136.580604996376,-23.016899728323));
#49832=CARTESIAN_POINT('',(14.,-136.580604996376,-23.016899728323));
#49833=CARTESIAN_POINT('',(14.5,-136.97510175753,-23.6446928191972));
#49834=CARTESIAN_POINT('',(14.5,-136.580604996376,-23.016899728323));
#49835=CARTESIAN_POINT('',(14.,-136.97510175753,-23.6446928191972));
#49836=CARTESIAN_POINT('Origin',(57.5,-136.216030001563,-25.0845072682928));
#49837=CARTESIAN_POINT('',(57.5,-136.216030001563,-25.0845072682928));
#49838=CARTESIAN_POINT('',(57.5,-136.216030001563,-25.0845072682928));
#49839=CARTESIAN_POINT('',(58.,-136.30080033501,-24.5894609761083));
#49840=CARTESIAN_POINT('Origin',(14.,-136.490947249372,-23.5110842376314));
#49841=CARTESIAN_POINT('',(14.,-136.490947249372,-23.5110842376314));
#49842=CARTESIAN_POINT('',(14.,-136.490947249372,-23.5110842376314));
#49843=CARTESIAN_POINT('',(14.5,-136.97510175753,-23.6446928191972));
#49844=CARTESIAN_POINT('Origin',(14.25,-134.149374290983,-22.5927285851944));
#49845=CARTESIAN_POINT('',(14.,-134.081679683799,-22.8333890101882));
#49846=CARTESIAN_POINT('',(14.5,-134.217068898167,-22.3520681602006));
#49847=CARTESIAN_POINT('Origin',(14.5,-136.216030001563,-25.0845072682928));
#49848=CARTESIAN_POINT('',(14.,-136.30080033501,-24.5894609761083));
#49849=CARTESIAN_POINT('',(14.5,-136.801453579863,-24.6295005722094));
#49850=CARTESIAN_POINT('',(14.,-136.30080033501,-24.5894609761083));
#49851=CARTESIAN_POINT('',(14.5,-136.216030001563,-25.0845072682928));
#49852=CARTESIAN_POINT('',(14.5,-136.216030001563,-25.0845072682928));
#49853=CARTESIAN_POINT('',(14.5,-136.801453579863,-24.6295005722094));
#49854=CARTESIAN_POINT('Origin',(14.25,-135.790690514667,-24.801902691856));
#49855=CARTESIAN_POINT('',(14.5,-135.771991924456,-25.0512024365894));
#49856=CARTESIAN_POINT('',(14.,-135.809389104878,-24.5526029471227));
#49857=CARTESIAN_POINT('Origin',(14.,-136.508741790713,-24.8570039202511));
#49858=CARTESIAN_POINT('',(14.,-136.801453579863,-24.6295005722094));
#49859=CARTESIAN_POINT('',(14.,-136.216030001563,-25.0845072682928));
#49860=CARTESIAN_POINT('Origin',(14.25,-136.728899819277,-23.6012807747805));
#49861=CARTESIAN_POINT('',(14.5,-136.97510175753,-23.6446928191972));
#49862=CARTESIAN_POINT('',(14.,-136.482697881024,-23.5578687303637));
#49863=CARTESIAN_POINT('Origin',(57.75,-135.790690514667,-24.801902691856));
#49864=CARTESIAN_POINT('',(57.5,-135.771991924456,-25.0512024365894));
#49865=CARTESIAN_POINT('Origin',(14.,-133.192154105382,-22.0637731308185));
#49866=CARTESIAN_POINT('Origin',(14.,-137.061925846364,-23.1522889426911));
#49867=CARTESIAN_POINT('Origin',(57.5,-134.393099376732,-35.4928843561058));
#49868=CARTESIAN_POINT('',(57.5,-134.054819567983,-34.8330975492484));
#49869=CARTESIAN_POINT('',(58.,-133.922431977811,-35.3175873497673));
#49870=CARTESIAN_POINT('',(57.5,-134.054819567983,-34.8330975492484));
#49871=CARTESIAN_POINT('',(57.5,-134.393099376732,-35.4928843561058));
#49872=CARTESIAN_POINT('',(57.5,-134.393099376732,-35.4928843561058));
#49873=CARTESIAN_POINT('',(58.,-133.922431977811,-35.3175873497673));
#49874=CARTESIAN_POINT('Origin',(57.5,-133.511428020236,-36.8610624138407));
#49875=CARTESIAN_POINT('',(57.5,-134.134280331629,-36.4588101823949));
#49876=CARTESIAN_POINT('',(58.,-133.639021904261,-36.375288143631));
#49877=CARTESIAN_POINT('',(57.5,-134.134280331629,-36.4588101823949));
#49878=CARTESIAN_POINT('',(57.5,-133.511428020236,-36.8610624138407));
#49879=CARTESIAN_POINT('',(57.5,-133.511428020236,-36.8610624138407));
#49880=CARTESIAN_POINT('',(58.,-133.639021904261,-36.375288143631));
#49881=CARTESIAN_POINT('Origin',(14.,-133.922431977811,-35.3175873497673));
#49882=CARTESIAN_POINT('',(14.5,-134.054819567983,-34.8330975492484));
#49883=CARTESIAN_POINT('',(14.5,-134.393099376732,-35.4928843561058));
#49884=CARTESIAN_POINT('',(14.5,-134.054819567983,-34.8330975492484));
#49885=CARTESIAN_POINT('',(14.,-133.922431977811,-35.3175873497673));
#49886=CARTESIAN_POINT('',(14.,-133.922431977811,-35.3175873497673));
#49887=CARTESIAN_POINT('',(14.5,-134.393099376732,-35.4928843561058));
#49888=CARTESIAN_POINT('Origin',(14.25,-131.669809380463,-34.1986447874607));
#49889=CARTESIAN_POINT('',(14.,-131.581397433607,-34.4324894531108));
#49890=CARTESIAN_POINT('',(14.5,-131.75822132732,-33.9648001218105));
#49891=CARTESIAN_POINT('Origin',(14.5,-133.511428020236,-36.8610624138407));
#49892=CARTESIAN_POINT('',(14.,-133.639021904261,-36.3752881436309));
#49893=CARTESIAN_POINT('',(14.5,-134.134280331629,-36.4588101823949));
#49894=CARTESIAN_POINT('',(14.,-133.639021904261,-36.3752881436309));
#49895=CARTESIAN_POINT('',(14.5,-133.511428020236,-36.8610624138407));
#49896=CARTESIAN_POINT('',(14.5,-133.511428020236,-36.8610624138407));
#49897=CARTESIAN_POINT('',(14.5,-134.134280331629,-36.4588101823949));
#49898=CARTESIAN_POINT('Origin',(14.25,-133.112337690265,-36.5424624542375));
#49899=CARTESIAN_POINT('',(14.5,-133.071982349415,-36.7891838486583));
#49900=CARTESIAN_POINT('',(14.,-133.152693031114,-36.2957410598168));
#49901=CARTESIAN_POINT('Origin',(14.,-133.822854175933,-36.6599362981178));
#49902=CARTESIAN_POINT('',(14.,-134.134280331629,-36.4588101823949));
#49903=CARTESIAN_POINT('',(14.,-133.511428020236,-36.8610624138407));
#49904=CARTESIAN_POINT('Origin',(14.25,-134.151617920159,-35.4281795948302));
#49905=CARTESIAN_POINT('',(14.5,-134.393099376732,-35.4928843561058));
#49906=CARTESIAN_POINT('',(14.,-133.910136463587,-35.3634748335546));
#49907=CARTESIAN_POINT('Origin',(14.,-134.223959472357,-35.1629909526771));
#49908=CARTESIAN_POINT('',(14.,-134.054819567983,-34.8330975492484));
#49909=CARTESIAN_POINT('',(14.,-134.393099376732,-35.4928843561058));
#49910=CARTESIAN_POINT('Origin',(57.75,-133.112337690265,-36.5424624542375));
#49911=CARTESIAN_POINT('',(58.,-133.152693031114,-36.2957410598168));
#49912=CARTESIAN_POINT('',(57.5,-133.071982349415,-36.7891838486583));
#49913=CARTESIAN_POINT('Origin',(57.75,-134.151617920159,-35.4281795948302));
#49914=CARTESIAN_POINT('',(58.,-133.910136463587,-35.3634748335546));
#49915=CARTESIAN_POINT('',(57.5,-134.393099376732,-35.4928843561058));
#49916=CARTESIAN_POINT('Origin',(57.75,-131.669809380463,-34.1986447874607));
#49917=CARTESIAN_POINT('',(57.5,-131.75822132732,-33.9648001218105));
#49918=CARTESIAN_POINT('',(58.,-131.581397433607,-34.4324894531108));
#49919=CARTESIAN_POINT('Origin',(14.,-132.331838201602,-35.4582091790453));
#49920=CARTESIAN_POINT('Origin',(14.,-130.762333212168,-33.5882749320356));
#49921=CARTESIAN_POINT('Origin',(14.,-134.522508899283,-35.0099214429613));
#49922=CARTESIAN_POINT('Origin',(57.5,-129.790723455271,-48.3570826171013));
#49923=CARTESIAN_POINT('',(57.5,-130.446264217578,-48.0106462326609));
#49924=CARTESIAN_POINT('',(58.,-129.960169823373,-47.8842774043812));
#49925=CARTESIAN_POINT('',(57.5,-130.446264217578,-48.0106462326609));
#49926=CARTESIAN_POINT('',(57.5,-129.790723455271,-48.3570826171013));
#49927=CARTESIAN_POINT('',(57.5,-129.790723455271,-48.3570826171013));
#49928=CARTESIAN_POINT('',(58.,-129.960169823373,-47.8842774043812));
#49929=CARTESIAN_POINT('Origin',(14.,-130.118493836425,-48.1838644248811));
#49930=CARTESIAN_POINT('',(14.2512407024475,-130.118493836425,-48.1838644248811));
#49931=CARTESIAN_POINT('',(14.5,-129.790723455271,-48.3570826171013));
#49932=CARTESIAN_POINT('',(14.3353834448875,-130.007625623529,-48.2424554157598));
#49933=CARTESIAN_POINT('',(14.,-129.790723455271,-48.3570826171013));
#49934=CARTESIAN_POINT('',(14.5,-130.446264217578,-48.0106462326609));
#49935=CARTESIAN_POINT('',(14.,-130.446264217578,-48.0106462326609));
#49936=CARTESIAN_POINT('',(14.4305329766294,-130.354733034817,-48.0590181018757));
#49937=CARTESIAN_POINT('Origin',(57.75,-129.420919600612,-48.0049120124002));
#49938=CARTESIAN_POINT('',(58.,-129.482624563588,-47.762646667078));
#49939=CARTESIAN_POINT('',(57.5,-129.359214637636,-48.2471773577224));
#49940=CARTESIAN_POINT('Origin',(57.5,-130.788284360904,-47.070953611875));
#49941=CARTESIAN_POINT('',(57.5,-130.508796018164,-46.3841944650247));
#49942=CARTESIAN_POINT('',(58.,-130.334686134323,-46.8553022968291));
#49943=CARTESIAN_POINT('',(57.5,-130.508796018164,-46.3841944650247));
#49944=CARTESIAN_POINT('',(57.5,-130.788284360904,-47.070953611875));
#49945=CARTESIAN_POINT('',(57.5,-130.788284360904,-47.070953611875));
#49946=CARTESIAN_POINT('',(58.,-130.334686134323,-46.8553022968291));
#49947=CARTESIAN_POINT('Origin',(14.,-130.648540189534,-46.7275740384498));
#49948=CARTESIAN_POINT('',(14.2512407024475,-130.648540189534,-46.7275740384498));
#49949=CARTESIAN_POINT('',(14.5,-130.788284360904,-47.070953611875));
#49950=CARTESIAN_POINT('',(14.2590041943422,-130.65290144458,-46.738290520452));
#49951=CARTESIAN_POINT('',(14.,-130.788284360904,-47.070953611875));
#49952=CARTESIAN_POINT('',(14.5,-130.508796018164,-46.3841944650247));
#49953=CARTESIAN_POINT('',(14.,-130.508796018164,-46.3841944650247));
#49954=CARTESIAN_POINT('',(14.6801520303733,-130.407592981924,-46.13551822277));
#49955=CARTESIAN_POINT('Origin',(57.75,-130.553361205708,-46.9854485760436));
#49956=CARTESIAN_POINT('',(58.,-130.318438050511,-46.8999435402122));
#49957=CARTESIAN_POINT('',(57.5,-130.788284360904,-47.070953611875));
#49958=CARTESIAN_POINT('Origin',(57.75,-128.188157716154,-45.5442886531881));
#49959=CARTESIAN_POINT('',(57.5,-128.296614134382,-45.3190394459863));
#49960=CARTESIAN_POINT('',(58.,-128.079701297925,-45.7695378603898));
#49961=CARTESIAN_POINT('Origin',(14.25,-129.420919600612,-48.0049120124002));
#49962=CARTESIAN_POINT('',(14.,-129.960169823373,-47.8842774043812));
#49963=CARTESIAN_POINT('',(14.5,-130.275254145916,-48.4804925430539));
#49964=CARTESIAN_POINT('',(14.,-129.482624563588,-47.762646667078));
#49965=CARTESIAN_POINT('',(14.5,-129.359214637636,-48.2471773577224));
#49966=CARTESIAN_POINT('Origin',(14.,-130.959294432567,-46.601107301482));
#49967=CARTESIAN_POINT('',(14.5,-130.788284360904,-47.070953611875));
#49968=CARTESIAN_POINT('Origin',(14.25,-130.553361205708,-46.9854485760436));
#49969=CARTESIAN_POINT('',(14.,-130.334686134323,-46.8553022968291));
#49970=CARTESIAN_POINT('',(14.,-130.334686134323,-46.8553022968291));
#49971=CARTESIAN_POINT('',(14.,-130.318438050511,-46.8999435402122));
#49972=CARTESIAN_POINT('Origin',(14.25,-128.188157716154,-45.5442886531881));
#49973=CARTESIAN_POINT('',(14.5,-128.296614134382,-45.3190394459863));
#49974=CARTESIAN_POINT('',(14.,-128.079701297925,-45.7695378603898));
#49975=CARTESIAN_POINT('Origin',(14.,-127.337332006754,-44.857149679865));
#49976=CARTESIAN_POINT('Origin',(14.,-130.275254145916,-48.4804925430539));
#49977=CARTESIAN_POINT('Origin',(57.5,-126.188091528965,-58.2907844884389));
#49978=CARTESIAN_POINT('',(57.5,-125.969521727281,-57.5822796533797));
#49979=CARTESIAN_POINT('',(58.,-125.755014631118,-58.036420101407));
#49980=CARTESIAN_POINT('',(57.5,-125.969521727281,-57.5822796533797));
#49981=CARTESIAN_POINT('',(57.5,-126.188091528965,-58.2907844884389));
#49982=CARTESIAN_POINT('',(57.5,-126.188091528965,-58.2907844884389));
#49983=CARTESIAN_POINT('',(58.,-125.755014631118,-58.036420101407));
#49984=CARTESIAN_POINT('Origin',(57.5,-125.08223311503,-59.4850762228408));
#49985=CARTESIAN_POINT('',(57.5,-125.765473267224,-59.1970922754755));
#49986=CARTESIAN_POINT('',(58.,-125.292242378034,-59.0288384007668));
#49987=CARTESIAN_POINT('',(57.5,-125.765473267224,-59.1970922754755));
#49988=CARTESIAN_POINT('',(57.5,-125.08223311503,-59.4850762228408));
#49989=CARTESIAN_POINT('',(57.5,-125.08223311503,-59.4850762228408));
#49990=CARTESIAN_POINT('',(58.,-125.292242378034,-59.0288384007668));
#49991=CARTESIAN_POINT('Origin',(14.,-125.755014631118,-58.0364201014069));
#49992=CARTESIAN_POINT('',(14.5,-125.969521727281,-57.5822796533797));
#49993=CARTESIAN_POINT('',(14.5,-126.188091528965,-58.2907844884389));
#49994=CARTESIAN_POINT('',(14.5,-125.969521727281,-57.5822796533797));
#49995=CARTESIAN_POINT('',(14.,-125.755014631118,-58.0364201014069));
#49996=CARTESIAN_POINT('',(14.,-125.755014631118,-58.0364201014069));
#49997=CARTESIAN_POINT('',(14.5,-126.188091528965,-58.2907844884389));
#49998=CARTESIAN_POINT('Origin',(14.25,-123.730916769498,-56.5433129818713));
#49999=CARTESIAN_POINT('',(14.,-123.603241298728,-56.7582524481485));
#50000=CARTESIAN_POINT('',(14.5,-123.858592240269,-56.3283735155941));
#50001=CARTESIAN_POINT('Origin',(14.5,-125.08223311503,-59.4850762228408));
#50002=CARTESIAN_POINT('',(14.,-125.292242378034,-59.0288384007668));
#50003=CARTESIAN_POINT('',(14.5,-125.765473267224,-59.1970922754756));
#50004=CARTESIAN_POINT('',(14.,-125.292242378034,-59.0288384007668));
#50005=CARTESIAN_POINT('',(14.5,-125.08223311503,-59.4850762228408));
#50006=CARTESIAN_POINT('',(14.5,-125.08223311503,-59.4850762228408));
#50007=CARTESIAN_POINT('',(14.5,-125.765473267224,-59.1970922754755));
#50008=CARTESIAN_POINT('Origin',(14.25,-124.744530166311,-59.1020152039901));
#50009=CARTESIAN_POINT('',(14.5,-124.661945193235,-59.3379807146521));
#50010=CARTESIAN_POINT('',(14.,-124.827115139388,-58.8660496933282));
#50011=CARTESIAN_POINT('Origin',(14.,-125.423853191127,-59.3410842491582));
#50012=CARTESIAN_POINT('',(14.,-125.765473267224,-59.1970922754755));
#50013=CARTESIAN_POINT('',(14.,-125.08223311503,-59.4850762228408));
#50014=CARTESIAN_POINT('Origin',(14.25,-125.961514582206,-58.1851299230037));
#50015=CARTESIAN_POINT('',(14.5,-126.188091528965,-58.2907844884389));
#50016=CARTESIAN_POINT('',(14.,-125.734937635446,-58.0794753575685));
#50017=CARTESIAN_POINT('Origin',(14.,-126.078806628123,-57.9365320709093));
#50018=CARTESIAN_POINT('',(14.,-125.969521727281,-57.5822796533797));
#50019=CARTESIAN_POINT('',(14.,-126.188091528965,-58.2907844884389));
#50020=CARTESIAN_POINT('Origin',(57.75,-124.744530166311,-59.1020152039901));
#50021=CARTESIAN_POINT('',(58.,-124.827115139388,-58.8660496933282));
#50022=CARTESIAN_POINT('',(57.5,-124.661945193235,-59.3379807146521));
#50023=CARTESIAN_POINT('Origin',(57.75,-125.961514582206,-58.1851299230037));
#50024=CARTESIAN_POINT('',(58.,-125.734937635446,-58.0794753575685));
#50025=CARTESIAN_POINT('',(57.5,-126.188091528965,-58.2907844884389));
#50026=CARTESIAN_POINT('Origin',(57.75,-123.730916769498,-56.5433129818713));
#50027=CARTESIAN_POINT('',(57.5,-123.858592240269,-56.3283735155941));
#50028=CARTESIAN_POINT('',(58.,-123.603241298728,-56.7582524481486));
#50029=CARTESIAN_POINT('Origin',(14.,-124.164166824021,-57.8987018584758));
#50030=CARTESIAN_POINT('Origin',(14.,-122.943216816385,-55.7846344331431));
#50031=CARTESIAN_POINT('Origin',(14.,-126.399400659835,-57.8376305949206));
#50032=CARTESIAN_POINT('Origin',(57.5,-120.627531126037,-69.0669872981078));
#50033=CARTESIAN_POINT('',(57.5,-120.471543313576,-68.3421289244414));
#50034=CARTESIAN_POINT('',(58.,-120.218271533617,-68.7758457056645));
#50035=CARTESIAN_POINT('',(57.5,-120.471543313576,-68.3421289244414));
#50036=CARTESIAN_POINT('',(57.5,-120.627531126037,-69.0669872981078));
#50037=CARTESIAN_POINT('',(57.5,-120.627531126037,-69.0669872981078));
#50038=CARTESIAN_POINT('',(58.,-120.218271533617,-68.7758457056645));
#50039=CARTESIAN_POINT('Origin',(57.5,-119.421791454066,-70.1603524804535));
#50040=CARTESIAN_POINT('',(57.5,-120.127531126037,-69.9330127018922));
#50041=CARTESIAN_POINT('',(58.,-119.670765314673,-69.7241542943354));
#50042=CARTESIAN_POINT('',(57.5,-120.127531126037,-69.9330127018922));
#50043=CARTESIAN_POINT('',(57.5,-119.421791454066,-70.1603524804535));
#50044=CARTESIAN_POINT('',(57.5,-119.421791454066,-70.1603524804535));
#50045=CARTESIAN_POINT('',(58.,-119.670765314673,-69.7241542943354));
#50046=CARTESIAN_POINT('Origin',(14.,-120.218271533617,-68.7758457056646));
#50047=CARTESIAN_POINT('',(14.5,-120.471543313576,-68.3421289244414));
#50048=CARTESIAN_POINT('',(14.5,-120.627531126037,-69.0669872981078));
#50049=CARTESIAN_POINT('',(14.5,-120.471543313576,-68.3421289244414));
#50050=CARTESIAN_POINT('',(14.,-120.218271533617,-68.7758457056646));
#50051=CARTESIAN_POINT('',(14.,-120.218271533617,-68.7758457056646));
#50052=CARTESIAN_POINT('',(14.5,-120.627531126037,-69.0669872981078));
#50053=CARTESIAN_POINT('Origin',(14.25,-118.332008835457,-67.1120085569767));
#50054=CARTESIAN_POINT('',(14.,-118.18608599957,-67.3150024632071));
#50055=CARTESIAN_POINT('',(14.5,-118.477931671344,-66.9090146507463));
#50056=CARTESIAN_POINT('Origin',(14.5,-119.421791454066,-70.1603524804535));
#50057=CARTESIAN_POINT('',(14.,-119.670765314673,-69.7241542943354));
#50058=CARTESIAN_POINT('',(14.5,-120.127531126037,-69.9330127018922));
#50059=CARTESIAN_POINT('',(14.,-119.670765314673,-69.7241542943354));
#50060=CARTESIAN_POINT('',(14.5,-119.421791454066,-70.1603524804535));
#50061=CARTESIAN_POINT('',(14.5,-119.421791454066,-70.1603524804535));
#50062=CARTESIAN_POINT('',(14.5,-120.127531126037,-69.9330127018922));
#50063=CARTESIAN_POINT('Origin',(14.25,-119.118759534638,-69.7493163731052));
#50064=CARTESIAN_POINT('',(14.5,-119.015923072972,-69.9771862090909));
#50065=CARTESIAN_POINT('',(14.,-119.221595996303,-69.5214465371196));
#50066=CARTESIAN_POINT('Origin',(14.,-119.774661290051,-70.0466825911729));
#50067=CARTESIAN_POINT('',(14.,-120.127531126037,-69.9330127018922));
#50068=CARTESIAN_POINT('',(14.,-119.421791454066,-70.1603524804535));
#50069=CARTESIAN_POINT('Origin',(14.25,-120.411024775091,-68.9419872981077));
#50070=CARTESIAN_POINT('',(14.5,-120.627531126037,-69.0669872981077));
#50071=CARTESIAN_POINT('',(14.,-120.194518424145,-68.8169872981078));
#50072=CARTESIAN_POINT('Origin',(14.,-120.549537219807,-68.7045581112746));
#50073=CARTESIAN_POINT('',(14.,-120.471543313576,-68.3421289244414));
#50074=CARTESIAN_POINT('',(14.,-120.627531126037,-69.0669872981078));
#50075=CARTESIAN_POINT('Origin',(57.75,-119.118759534638,-69.7493163731052));
#50076=CARTESIAN_POINT('',(58.,-119.221595996303,-69.5214465371196));
#50077=CARTESIAN_POINT('',(57.5,-119.015923072972,-69.9771862090909));
#50078=CARTESIAN_POINT('Origin',(57.75,-120.411024775091,-68.9419872981077));
#50079=CARTESIAN_POINT('',(58.,-120.194518424145,-68.8169872981077));
#50080=CARTESIAN_POINT('',(57.5,-120.627531126037,-69.0669872981077));
#50081=CARTESIAN_POINT('Origin',(57.75,-118.332008835457,-67.1120085569767));
#50082=CARTESIAN_POINT('',(57.5,-118.477931671344,-66.9090146507463));
#50083=CARTESIAN_POINT('',(58.,-118.18608599957,-67.3150024632071));
#50084=CARTESIAN_POINT('Origin',(14.,-118.645480318468,-68.5));
#50085=CARTESIAN_POINT('Origin',(14.,-117.613429510899,-66.2875644347018));
#50086=CARTESIAN_POINT('Origin',(14.,-120.877531126037,-68.6339745962155));
#50087=CARTESIAN_POINT('Origin',(57.75,-112.032522863357,-77.1699412236247));
#50088=CARTESIAN_POINT('',(57.7487592975525,-114.102813043447,-78.9497009794667));
#50089=CARTESIAN_POINT('',(58.,-113.766594799967,-78.991845596111));
#50090=CARTESIAN_POINT('',(58.2319907935076,-113.456137392641,-79.0307611180075));
#50091=CARTESIAN_POINT('',(58.,-111.869463223246,-77.3594446636108));
#50092=CARTESIAN_POINT('',(57.5,-114.056703712549,-78.5818533282824));
#50093=CARTESIAN_POINT('',(57.5,-112.195582503469,-76.9804377836386));
#50094=CARTESIAN_POINT('',(50.4896657310026,-112.757287667812,-68.2154669449852));
#50095=CARTESIAN_POINT('Origin',(58.,-112.223830067592,-78.5799717800933));
#50096=CARTESIAN_POINT('',(58.,-113.138521468083,-79.8888272731287));
#50097=CARTESIAN_POINT('',(58.,-113.739346352201,-79.0307604124754));
#50098=CARTESIAN_POINT('',(58.,-112.708728519719,-79.6477431945663));
#50099=CARTESIAN_POINT('Origin',(57.75,-113.944134363273,-79.1741545215631));
#50100=CARTESIAN_POINT('',(57.5,-114.148922374345,-79.3175486306509));
#50101=CARTESIAN_POINT('',(57.5,-114.148922374345,-79.3175486306509));
#50102=CARTESIAN_POINT('',(57.5,-113.575345937994,-80.1367006749399));
#50103=CARTESIAN_POINT('',(57.5,-114.148922374345,-79.3175486306509));
#50104=CARTESIAN_POINT('',(57.5,-113.575345937994,-80.1367006749399));
#50105=CARTESIAN_POINT('Origin',(14.,-114.102813043447,-78.9497009794667));
#50106=CARTESIAN_POINT('',(14.5,-114.056703712549,-78.5818533282824));
#50107=CARTESIAN_POINT('',(14.,-114.056703712549,-78.5818533282824));
#50108=CARTESIAN_POINT('',(14.5,-114.148922374345,-79.3175486306509));
#50109=CARTESIAN_POINT('',(14.5,-114.056703712549,-78.5818533282824));
#50110=CARTESIAN_POINT('',(14.,-114.148922374345,-79.3175486306509));
#50111=CARTESIAN_POINT('Origin',(57.5,-112.852477851287,-80.3016660917109));
#50112=CARTESIAN_POINT('',(57.5,-112.852477851287,-80.3016660917109));
#50113=CARTESIAN_POINT('',(57.5,-112.852477851287,-80.3016660917109));
#50114=CARTESIAN_POINT('',(58.,-113.138521468083,-79.8888272731287));
#50115=CARTESIAN_POINT('Origin',(14.,-113.766594799967,-78.991845596111));
#50116=CARTESIAN_POINT('',(14.,-113.766594799967,-78.991845596111));
#50117=CARTESIAN_POINT('',(14.,-113.766594799967,-78.991845596111));
#50118=CARTESIAN_POINT('',(14.5,-114.148922374345,-79.3175486306509));
#50119=CARTESIAN_POINT('Origin',(14.25,-112.032522863357,-77.1699412236247));
#50120=CARTESIAN_POINT('',(14.,-111.869463223246,-77.3594446636108));
#50121=CARTESIAN_POINT('',(14.5,-112.195582503469,-76.9804377836386));
#50122=CARTESIAN_POINT('Origin',(14.5,-112.852477851287,-80.3016660917109));
#50123=CARTESIAN_POINT('',(14.,-113.138521468083,-79.8888272731287));
#50124=CARTESIAN_POINT('',(14.5,-113.575345937994,-80.1367006749399));
#50125=CARTESIAN_POINT('',(14.,-113.138521468083,-79.8888272731287));
#50126=CARTESIAN_POINT('',(14.5,-112.852477851287,-80.3016660917109));
#50127=CARTESIAN_POINT('',(14.5,-112.852477851287,-80.3016660917109));
#50128=CARTESIAN_POINT('',(14.5,-113.575345937994,-80.1367006749399));
#50129=CARTESIAN_POINT('Origin',(14.25,-112.586423217032,-79.8657831288322));
#50130=CARTESIAN_POINT('',(14.5,-112.464117914346,-80.0838230630982));
#50131=CARTESIAN_POINT('',(14.,-112.708728519719,-79.6477431945663));
#50132=CARTESIAN_POINT('Origin',(14.,-113.213911894641,-80.2191833833254));
#50133=CARTESIAN_POINT('',(14.,-113.575345937994,-80.1367006749399));
#50134=CARTESIAN_POINT('',(14.,-112.852477851287,-80.3016660917109));
#50135=CARTESIAN_POINT('Origin',(14.25,-113.944134363273,-79.1741545215631));
#50136=CARTESIAN_POINT('',(14.5,-114.148922374345,-79.3175486306509));
#50137=CARTESIAN_POINT('',(14.,-113.739346352201,-79.0307604124754));
#50138=CARTESIAN_POINT('Origin',(57.75,-112.586423217032,-79.8657831288322));
#50139=CARTESIAN_POINT('',(57.5,-112.464117914346,-80.0838230630982));
#50140=CARTESIAN_POINT('Origin',(14.,-111.388532989905,-76.2860060453866));
#50141=CARTESIAN_POINT('Origin',(14.,-114.435710592521,-78.9079726085064));
#50142=CARTESIAN_POINT('Origin',(57.5,-106.801571398381,-88.9644555248695));
#50143=CARTESIAN_POINT('',(57.5,-106.773823726948,-88.223522379275));
#50144=CARTESIAN_POINT('',(58.,-106.449085585742,-88.6066698449906));
#50145=CARTESIAN_POINT('',(57.5,-106.773823726948,-88.223522379275));
#50146=CARTESIAN_POINT('',(57.5,-106.801571398381,-88.9644555248695));
#50147=CARTESIAN_POINT('',(57.5,-106.801571398381,-88.9644555248695));
#50148=CARTESIAN_POINT('',(58.,-106.449085585742,-88.6066698449906));
#50149=CARTESIAN_POINT('Origin',(57.5,-105.424288749871,-89.8318355365386));
#50150=CARTESIAN_POINT('',(57.5,-106.158783788695,-89.7304999679885));
#50151=CARTESIAN_POINT('',(58.,-105.745225158215,-89.4454980381808));
#50152=CARTESIAN_POINT('',(57.5,-106.158783788695,-89.7304999679885));
#50153=CARTESIAN_POINT('',(57.5,-105.424288749871,-89.8318355365386));
#50154=CARTESIAN_POINT('',(57.5,-105.424288749871,-89.8318355365386));
#50155=CARTESIAN_POINT('',(58.,-105.745225158215,-89.4454980381808));
#50156=CARTESIAN_POINT('Origin',(14.,-106.449085585742,-88.6066698449906));
#50157=CARTESIAN_POINT('',(14.5,-106.773823726948,-88.223522379275));
#50158=CARTESIAN_POINT('',(14.5,-106.801571398381,-88.9644555248695));
#50159=CARTESIAN_POINT('',(14.5,-106.773823726948,-88.223522379275));
#50160=CARTESIAN_POINT('',(14.,-106.449085585742,-88.6066698449906));
#50161=CARTESIAN_POINT('',(14.,-106.449085585742,-88.6066698449906));
#50162=CARTESIAN_POINT('',(14.5,-106.801571398381,-88.9644555248695));
#50163=CARTESIAN_POINT('Origin',(14.25,-104.880401745181,-86.6405640410765));
#50164=CARTESIAN_POINT('',(14.,-104.701446283163,-86.8151347792147));
#50165=CARTESIAN_POINT('',(14.5,-105.059357207198,-86.4659933029383));
#50166=CARTESIAN_POINT('Origin',(14.5,-105.424288749871,-89.8318355365386));
#50167=CARTESIAN_POINT('',(14.,-105.745225158215,-89.4454980381808));
#50168=CARTESIAN_POINT('',(14.5,-106.158783788695,-89.7304999679885));
#50169=CARTESIAN_POINT('',(14.,-105.745225158215,-89.4454980381808));
#50170=CARTESIAN_POINT('',(14.5,-105.424288749871,-89.8318355365386));
#50171=CARTESIAN_POINT('',(14.5,-105.424288749871,-89.8318355365386));
#50172=CARTESIAN_POINT('',(14.5,-106.158783788695,-89.7304999679885));
#50173=CARTESIAN_POINT('Origin',(14.25,-105.197236237204,-89.3744230506705));
#50174=CARTESIAN_POINT('',(14.5,-105.0563929107,-89.5809736676609));
#50175=CARTESIAN_POINT('',(14.,-105.338079563709,-89.1678724336801));
#50176=CARTESIAN_POINT('Origin',(14.,-105.791536269283,-89.7811677522635));
#50177=CARTESIAN_POINT('',(14.,-106.158783788695,-89.7304999679885));
#50178=CARTESIAN_POINT('',(14.,-105.424288749871,-89.8318355365386));
#50179=CARTESIAN_POINT('Origin',(14.25,-106.610060287601,-88.8037586224479));
#50180=CARTESIAN_POINT('',(14.5,-106.801571398381,-88.9644555248695));
#50181=CARTESIAN_POINT('',(14.,-106.418549176822,-88.6430617200262));
#50182=CARTESIAN_POINT('Origin',(14.,-106.787697562665,-88.5939889520722));
#50183=CARTESIAN_POINT('',(14.,-106.773823726948,-88.223522379275));
#50184=CARTESIAN_POINT('',(14.,-106.801571398381,-88.9644555248695));
#50185=CARTESIAN_POINT('Origin',(57.75,-105.197236237204,-89.3744230506705));
#50186=CARTESIAN_POINT('',(58.,-105.338079563709,-89.1678724336801));
#50187=CARTESIAN_POINT('',(57.5,-105.0563929107,-89.5809736676609));
#50188=CARTESIAN_POINT('Origin',(57.75,-106.610060287601,-88.8037586224479));
#50189=CARTESIAN_POINT('',(58.,-106.418549176822,-88.6430617200262));
#50190=CARTESIAN_POINT('',(57.5,-106.801571398381,-88.9644555248695));
#50191=CARTESIAN_POINT('Origin',(57.75,-104.880401745181,-86.6405640410765));
#50192=CARTESIAN_POINT('',(57.5,-105.059357207198,-86.4659933029383));
#50193=CARTESIAN_POINT('',(58.,-104.701446283163,-86.8151347792147));
#50194=CARTESIAN_POINT('Origin',(14.,-104.9480887073,-88.0619025270559));
#50195=CARTESIAN_POINT('Origin',(14.,-104.315902474623,-85.7038650873162));
#50196=CARTESIAN_POINT('Origin',(14.,-107.122965203224,-88.58143330331));
#50197=CARTESIAN_POINT('Origin',(57.5,-97.1937571541419,-98.678330470988));
#50198=CARTESIAN_POINT('',(57.5,-97.9342891943368,-98.6413959755234));
#50199=CARTESIAN_POINT('',(58.,-97.5471438341798,-98.3214345544939));
#50200=CARTESIAN_POINT('',(57.5,-97.9342891943368,-98.6413959755234));
#50201=CARTESIAN_POINT('',(57.5,-97.1937571541419,-98.678330470988));
#50202=CARTESIAN_POINT('',(57.5,-97.1937571541419,-98.678330470988));
#50203=CARTESIAN_POINT('',(58.,-97.5471438341798,-98.3214345544939));
#50204=CARTESIAN_POINT('Origin',(14.,-97.5640231742394,-98.6598632232557));
#50205=CARTESIAN_POINT('',(14.2512407024475,-97.5640231742394,-98.6598632232557));
#50206=CARTESIAN_POINT('',(14.5,-97.1937571541419,-98.678330470988));
#50207=CARTESIAN_POINT('',(14.3353834448875,-97.4387808268383,-98.666109763123));
#50208=CARTESIAN_POINT('',(14.,-97.1937571541419,-98.678330470988));
#50209=CARTESIAN_POINT('',(14.5,-97.9342891943368,-98.6413959755234));
#50210=CARTESIAN_POINT('',(14.,-97.9342891943368,-98.6413959755234));
#50211=CARTESIAN_POINT('',(14.4305329766294,-97.8308909353592,-98.6465530279127));
#50212=CARTESIAN_POINT('Origin',(57.75,-97.0074347697832,-98.2028696473411));
#50213=CARTESIAN_POINT('',(58.,-97.1657442173475,-98.0093803225402));
#50214=CARTESIAN_POINT('',(57.5,-96.8491253222189,-98.3963589721419));
#50215=CARTESIAN_POINT('Origin',(57.5,-98.6413959755234,-97.9342891943368));
#50216=CARTESIAN_POINT('',(57.5,-98.678330470988,-97.1937571541419));
#50217=CARTESIAN_POINT('',(58.,-98.3214345544939,-97.5471438341797));
#50218=CARTESIAN_POINT('',(57.5,-98.678330470988,-97.1937571541419));
#50219=CARTESIAN_POINT('',(57.5,-98.6413959755234,-97.9342891943368));
#50220=CARTESIAN_POINT('',(57.5,-98.6413959755234,-97.9342891943368));
#50221=CARTESIAN_POINT('',(58.,-98.3214345544939,-97.5471438341797));
#50222=CARTESIAN_POINT('Origin',(14.,-98.6598632232557,-97.5640231742394));
#50223=CARTESIAN_POINT('',(14.2512407024475,-98.6598632232557,-97.5640231742394));
#50224=CARTESIAN_POINT('',(14.5,-98.6413959755234,-97.9342891943368));
#50225=CARTESIAN_POINT('',(14.2590041943422,-98.6592868816697,-97.5755787513542));
#50226=CARTESIAN_POINT('',(14.,-98.6413959755234,-97.9342891943368));
#50227=CARTESIAN_POINT('',(14.5,-98.678330470988,-97.1937571541419));
#50228=CARTESIAN_POINT('',(14.,-98.678330470988,-97.1937571541419));
#50229=CARTESIAN_POINT('',(14.6801520303733,-98.69170449241,-96.925609688077));
#50230=CARTESIAN_POINT('Origin',(57.75,-98.4646192802267,-97.7575124990402));
#50231=CARTESIAN_POINT('',(58.,-98.2878425849301,-97.5807358037436));
#50232=CARTESIAN_POINT('',(57.5,-98.6413959755234,-97.9342891943368));
#50233=CARTESIAN_POINT('Origin',(57.75,-96.9300774412053,-95.4517998511728));
#50234=CARTESIAN_POINT('',(57.5,-97.1235667660061,-95.2934904036084));
#50235=CARTESIAN_POINT('',(58.,-96.7365881164045,-95.6101092987371));
#50236=CARTESIAN_POINT('Origin',(14.25,-97.0074347697832,-98.2028696473411));
#50237=CARTESIAN_POINT('',(14.,-97.5471438341798,-98.3214345544939));
#50238=CARTESIAN_POINT('',(14.5,-97.5807358037436,-98.9949493661167));
#50239=CARTESIAN_POINT('',(14.,-97.1657442173475,-98.0093803225402));
#50240=CARTESIAN_POINT('',(14.5,-96.8491253222189,-98.3963589721419));
#50241=CARTESIAN_POINT('Origin',(14.,-98.9949493661167,-97.5807358037436));
#50242=CARTESIAN_POINT('',(14.5,-98.6413959755234,-97.9342891943368));
#50243=CARTESIAN_POINT('Origin',(14.25,-98.4646192802267,-97.7575124990402));
#50244=CARTESIAN_POINT('',(14.,-98.3214345544939,-97.5471438341797));
#50245=CARTESIAN_POINT('',(14.,-98.3214345544939,-97.5471438341797));
#50246=CARTESIAN_POINT('',(14.,-98.2878425849301,-97.5807358037436));
#50247=CARTESIAN_POINT('Origin',(14.25,-96.9300774412053,-95.4517998511728));
#50248=CARTESIAN_POINT('',(14.5,-97.1235667660061,-95.2934904036084));
#50249=CARTESIAN_POINT('',(14.,-96.7365881164044,-95.6101092987371));
#50250=CARTESIAN_POINT('Origin',(14.,-96.4493649538451,-94.4694659665227));
#50251=CARTESIAN_POINT('Origin',(14.,-97.5807358037436,-98.9949493661167));
#50252=CARTESIAN_POINT('Origin',(57.5,-89.7304999679885,-106.158783788695));
#50253=CARTESIAN_POINT('',(57.5,-89.8318355365387,-105.424288749871));
#50254=CARTESIAN_POINT('',(58.,-89.4454980381808,-105.745225158215));
#50255=CARTESIAN_POINT('',(57.5,-89.8318355365387,-105.424288749871));
#50256=CARTESIAN_POINT('',(57.5,-89.7304999679885,-106.158783788695));
#50257=CARTESIAN_POINT('',(57.5,-89.7304999679885,-106.158783788695));
#50258=CARTESIAN_POINT('',(58.,-89.4454980381808,-105.745225158215));
#50259=CARTESIAN_POINT('Origin',(57.5,-88.223522379275,-106.773823726948));
#50260=CARTESIAN_POINT('',(57.5,-88.9644555248695,-106.801571398381));
#50261=CARTESIAN_POINT('',(58.,-88.6066698449906,-106.449085585742));
#50262=CARTESIAN_POINT('',(57.5,-88.9644555248695,-106.801571398381));
#50263=CARTESIAN_POINT('',(57.5,-88.223522379275,-106.773823726948));
#50264=CARTESIAN_POINT('',(57.5,-88.223522379275,-106.773823726948));
#50265=CARTESIAN_POINT('',(58.,-88.6066698449906,-106.449085585742));
#50266=CARTESIAN_POINT('Origin',(14.,-89.4454980381808,-105.745225158215));
#50267=CARTESIAN_POINT('',(14.5,-89.8318355365387,-105.424288749871));
#50268=CARTESIAN_POINT('',(14.5,-89.7304999679885,-106.158783788695));
#50269=CARTESIAN_POINT('',(14.5,-89.8318355365387,-105.424288749871));
#50270=CARTESIAN_POINT('',(14.,-89.4454980381808,-105.745225158215));
#50271=CARTESIAN_POINT('',(14.,-89.4454980381808,-105.745225158215));
#50272=CARTESIAN_POINT('',(14.5,-89.7304999679885,-106.158783788695));
#50273=CARTESIAN_POINT('Origin',(14.25,-88.2420567199213,-103.536589829029));
#50274=CARTESIAN_POINT('',(14.,-88.0355061029309,-103.677433155534));
#50275=CARTESIAN_POINT('',(14.5,-88.4486073369116,-103.395746502524));
#50276=CARTESIAN_POINT('Origin',(14.5,-88.223522379275,-106.773823726948));
#50277=CARTESIAN_POINT('',(14.,-88.6066698449906,-106.449085585742));
#50278=CARTESIAN_POINT('',(14.5,-88.9644555248695,-106.801571398381));
#50279=CARTESIAN_POINT('',(14.,-88.6066698449906,-106.449085585742));
#50280=CARTESIAN_POINT('',(14.5,-88.223522379275,-106.773823726948));
#50281=CARTESIAN_POINT('',(14.5,-88.223522379275,-106.773823726948));
#50282=CARTESIAN_POINT('',(14.5,-88.9644555248695,-106.801571398381));
#50283=CARTESIAN_POINT('Origin',(14.25,-88.0793481490734,-106.283933109481));
#50284=CARTESIAN_POINT('',(14.5,-87.9047774109353,-106.462888571499));
#50285=CARTESIAN_POINT('',(14.,-88.2539188872116,-106.104977647464));
#50286=CARTESIAN_POINT('Origin',(14.,-88.5939889520723,-106.787697562665));
#50287=CARTESIAN_POINT('',(14.,-88.9644555248695,-106.801571398381));
#50288=CARTESIAN_POINT('',(14.,-88.223522379275,-106.773823726948));
#50289=CARTESIAN_POINT('Origin',(14.25,-89.5698030655668,-105.967272677915));
#50290=CARTESIAN_POINT('',(14.5,-89.7304999679885,-106.158783788695));
#50291=CARTESIAN_POINT('',(14.,-89.4091061631452,-105.775761567135));
#50292=CARTESIAN_POINT('Origin',(14.,-89.7811677522636,-105.791536269283));
#50293=CARTESIAN_POINT('',(14.,-89.8318355365387,-105.424288749871));
#50294=CARTESIAN_POINT('',(14.,-89.7304999679885,-106.158783788695));
#50295=CARTESIAN_POINT('Origin',(57.75,-88.0793481490734,-106.283933109481));
#50296=CARTESIAN_POINT('',(58.,-88.2539188872116,-106.104977647464));
#50297=CARTESIAN_POINT('',(57.5,-87.9047774109353,-106.462888571499));
#50298=CARTESIAN_POINT('Origin',(57.75,-89.5698030655668,-105.967272677915));
#50299=CARTESIAN_POINT('',(58.,-89.4091061631452,-105.775761567135));
#50300=CARTESIAN_POINT('',(57.5,-89.7304999679885,-106.158783788695));
#50301=CARTESIAN_POINT('Origin',(57.75,-88.2420567199213,-103.536589829029));
#50302=CARTESIAN_POINT('',(57.5,-88.4486073369116,-103.395746502524));
#50303=CARTESIAN_POINT('',(58.,-88.0355061029309,-103.677433155534));
#50304=CARTESIAN_POINT('Origin',(14.,-88.0619025270559,-104.9480887073));
#50305=CARTESIAN_POINT('Origin',(14.,-87.8487895280494,-102.516097167501));
#50306=CARTESIAN_POINT('Origin',(14.,-90.113522189548,-105.837389983851));
#50307=CARTESIAN_POINT('Origin',(57.5,-80.13670067494,-113.575345937994));
#50308=CARTESIAN_POINT('',(57.5,-80.301666091711,-112.852477851287));
#50309=CARTESIAN_POINT('',(58.,-79.8888272731288,-113.138521468083));
#50310=CARTESIAN_POINT('',(57.5,-80.301666091711,-112.852477851287));
#50311=CARTESIAN_POINT('',(57.5,-80.13670067494,-113.575345937994));
#50312=CARTESIAN_POINT('',(57.5,-80.13670067494,-113.575345937994));
#50313=CARTESIAN_POINT('',(58.,-79.8888272731288,-113.138521468083));
#50314=CARTESIAN_POINT('Origin',(57.5,-78.5818533282825,-114.056703712549));
#50315=CARTESIAN_POINT('',(57.5,-79.317548630651,-114.148922374345));
#50316=CARTESIAN_POINT('',(58.,-78.9918455961111,-113.766594799967));
#50317=CARTESIAN_POINT('',(57.5,-79.317548630651,-114.148922374345));
#50318=CARTESIAN_POINT('',(57.5,-78.5818533282825,-114.056703712549));
#50319=CARTESIAN_POINT('',(57.5,-78.5818533282825,-114.056703712549));
#50320=CARTESIAN_POINT('',(58.,-78.9918455961111,-113.766594799967));
#50321=CARTESIAN_POINT('Origin',(14.,-79.8888272731288,-113.138521468083));
#50322=CARTESIAN_POINT('',(14.5,-80.301666091711,-112.852477851287));
#50323=CARTESIAN_POINT('',(14.5,-80.13670067494,-113.575345937994));
#50324=CARTESIAN_POINT('',(14.5,-80.301666091711,-112.852477851287));
#50325=CARTESIAN_POINT('',(14.,-79.8888272731288,-113.138521468083));
#50326=CARTESIAN_POINT('',(14.,-79.8888272731288,-113.138521468083));
#50327=CARTESIAN_POINT('',(14.5,-80.13670067494,-113.575345937994));
#50328=CARTESIAN_POINT('Origin',(14.25,-78.882460664988,-110.833403841184));
#50329=CARTESIAN_POINT('',(14.,-78.6644207307221,-110.955709143871));
#50330=CARTESIAN_POINT('',(14.5,-79.100500599254,-110.711098538497));
#50331=CARTESIAN_POINT('Origin',(14.5,-78.5818533282825,-114.056703712549));
#50332=CARTESIAN_POINT('',(14.,-78.991845596111,-113.766594799967));
#50333=CARTESIAN_POINT('',(14.5,-79.317548630651,-114.148922374345));
#50334=CARTESIAN_POINT('',(14.,-78.991845596111,-113.766594799967));
#50335=CARTESIAN_POINT('',(14.5,-78.5818533282825,-114.056703712549));
#50336=CARTESIAN_POINT('',(14.5,-78.5818533282825,-114.056703712549));
#50337=CARTESIAN_POINT('',(14.5,-79.317548630651,-114.148922374345));
#50338=CARTESIAN_POINT('Origin',(14.25,-78.4809245051847,-113.556111664665));
#50339=CARTESIAN_POINT('',(14.5,-78.2914210651986,-113.719171304777));
#50340=CARTESIAN_POINT('',(14.,-78.6704279451708,-113.393052024553));
#50341=CARTESIAN_POINT('Origin',(14.,-78.9497009794668,-114.102813043447));
#50342=CARTESIAN_POINT('',(14.,-79.317548630651,-114.148922374345));
#50343=CARTESIAN_POINT('',(14.,-78.5818533282825,-114.056703712549));
#50344=CARTESIAN_POINT('Origin',(14.25,-79.9933065658522,-113.370557926922));
#50345=CARTESIAN_POINT('',(14.5,-80.13670067494,-113.575345937994));
#50346=CARTESIAN_POINT('',(14.,-79.8499124567644,-113.16576991585));
#50347=CARTESIAN_POINT('Origin',(14.,-80.2191833833255,-113.213911894641));
#50348=CARTESIAN_POINT('',(14.,-80.301666091711,-112.852477851287));
#50349=CARTESIAN_POINT('',(14.,-80.13670067494,-113.575345937994));
#50350=CARTESIAN_POINT('Origin',(57.75,-78.4809245051847,-113.556111664665));
#50351=CARTESIAN_POINT('',(58.,-78.6704279451708,-113.393052024553));
#50352=CARTESIAN_POINT('',(57.5,-78.2914210651986,-113.719171304777));
#50353=CARTESIAN_POINT('Origin',(57.75,-79.9933065658522,-113.370557926922));
#50354=CARTESIAN_POINT('',(58.,-79.8499124567644,-113.16576991585));
#50355=CARTESIAN_POINT('',(57.5,-80.13670067494,-113.575345937994));
#50356=CARTESIAN_POINT('Origin',(57.75,-78.882460664988,-110.833403841184));
#50357=CARTESIAN_POINT('',(57.5,-79.100500599254,-110.711098538497));
#50358=CARTESIAN_POINT('',(58.,-78.6644207307221,-110.955709143871));
#50359=CARTESIAN_POINT('Origin',(14.,-78.5799717800934,-112.223830067592));
#50360=CARTESIAN_POINT('Origin',(14.,-78.5796317693959,-109.782518968122));
#50361=CARTESIAN_POINT('Origin',(14.,-80.5462766970845,-113.288557719819));
#50362=CARTESIAN_POINT('Origin',(57.75,-68.9225214538621,-117.286708727069));
#50363=CARTESIAN_POINT('',(57.7487592975525,-70.0466825911729,-119.774661290051));
#50364=CARTESIAN_POINT('',(58.,-69.7241542943354,-119.670765314673));
#50365=CARTESIAN_POINT('',(58.2319907935076,-69.4263379183141,-119.574829785376));
#50366=CARTESIAN_POINT('',(58.,-68.6946516178765,-117.389545188734));
#50367=CARTESIAN_POINT('',(57.5,-70.1603524804535,-119.421791454066));
#50368=CARTESIAN_POINT('',(57.5,-69.1503912898478,-117.183872265404));
#50369=CARTESIAN_POINT('',(50.4896657310027,-73.3637057943502,-109.477497801348));
#50370=CARTESIAN_POINT('Origin',(58.,-68.5,-118.645480318468));
#50371=CARTESIAN_POINT('',(58.,-68.7758457056646,-120.218271533617));
#50372=CARTESIAN_POINT('',(58.,-69.6830127018922,-119.694518424145));
#50373=CARTESIAN_POINT('',(58.,-68.488207543964,-119.818136807139));
#50374=CARTESIAN_POINT('Origin',(57.75,-69.8080127018922,-119.911024775091));
#50375=CARTESIAN_POINT('',(57.5,-69.9330127018922,-120.127531126037));
#50376=CARTESIAN_POINT('',(57.5,-69.9330127018922,-120.127531126037));
#50377=CARTESIAN_POINT('',(57.5,-69.0669872981078,-120.627531126037));
#50378=CARTESIAN_POINT('',(57.5,-69.9330127018922,-120.127531126037));
#50379=CARTESIAN_POINT('',(57.5,-69.0669872981078,-120.627531126037));
#50380=CARTESIAN_POINT('Origin',(14.,-70.0466825911729,-119.774661290051));
#50381=CARTESIAN_POINT('',(14.5,-70.1603524804535,-119.421791454066));
#50382=CARTESIAN_POINT('',(14.,-70.1603524804535,-119.421791454066));
#50383=CARTESIAN_POINT('',(14.5,-69.9330127018922,-120.127531126037));
#50384=CARTESIAN_POINT('',(14.5,-70.1603524804535,-119.421791454066));
#50385=CARTESIAN_POINT('',(14.,-69.9330127018922,-120.127531126037));
#50386=CARTESIAN_POINT('Origin',(57.5,-68.3421289244414,-120.471543313576));
#50387=CARTESIAN_POINT('',(57.5,-68.3421289244414,-120.471543313576));
#50388=CARTESIAN_POINT('',(57.5,-68.3421289244414,-120.471543313576));
#50389=CARTESIAN_POINT('',(58.,-68.7758457056646,-120.218271533617));
#50390=CARTESIAN_POINT('Origin',(14.,-69.7241542943354,-119.670765314673));
#50391=CARTESIAN_POINT('',(14.,-69.7241542943354,-119.670765314673));
#50392=CARTESIAN_POINT('',(14.,-69.7241542943354,-119.670765314673));
#50393=CARTESIAN_POINT('',(14.5,-69.9330127018922,-120.127531126037));
#50394=CARTESIAN_POINT('Origin',(14.25,-68.9225214538621,-117.286708727069));
#50395=CARTESIAN_POINT('',(14.,-68.6946516178764,-117.389545188734));
#50396=CARTESIAN_POINT('',(14.5,-69.1503912898478,-117.183872265404));
#50397=CARTESIAN_POINT('Origin',(14.5,-68.3421289244414,-120.471543313576));
#50398=CARTESIAN_POINT('',(14.,-68.7758457056646,-120.218271533617));
#50399=CARTESIAN_POINT('',(14.5,-69.0669872981078,-120.627531126037));
#50400=CARTESIAN_POINT('',(14.,-68.7758457056646,-120.218271533617));
#50401=CARTESIAN_POINT('',(14.5,-68.3421289244414,-120.471543313576));
#50402=CARTESIAN_POINT('',(14.5,-68.3421289244414,-120.471543313576));
#50403=CARTESIAN_POINT('',(14.5,-69.0669872981078,-120.627531126037));
#50404=CARTESIAN_POINT('Origin',(14.25,-68.2852136377336,-119.964059643026));
#50405=CARTESIAN_POINT('',(14.5,-68.0822197315031,-120.109982478913));
#50406=CARTESIAN_POINT('',(14.,-68.488207543964,-119.818136807139));
#50407=CARTESIAN_POINT('Origin',(14.,-68.7045581112746,-120.549537219807));
#50408=CARTESIAN_POINT('',(14.,-69.0669872981078,-120.627531126037));
#50409=CARTESIAN_POINT('',(14.,-68.3421289244414,-120.471543313576));
#50410=CARTESIAN_POINT('Origin',(14.25,-69.8080127018922,-119.911024775091));
#50411=CARTESIAN_POINT('',(14.5,-69.9330127018922,-120.127531126037));
#50412=CARTESIAN_POINT('',(14.,-69.6830127018922,-119.694518424145));
#50413=CARTESIAN_POINT('Origin',(57.75,-68.2852136377336,-119.964059643026));
#50414=CARTESIAN_POINT('',(57.5,-68.0822197315031,-120.109982478913));
#50415=CARTESIAN_POINT('Origin',(14.,-68.7124355652982,-116.213429510899));
#50416=CARTESIAN_POINT('Origin',(14.,-70.3660254037844,-119.877531126037));
#50417=CARTESIAN_POINT('Origin',(57.5,-59.1970922754756,-125.765473267224));
#50418=CARTESIAN_POINT('',(57.5,-59.4850762228409,-125.08223311503));
#50419=CARTESIAN_POINT('',(58.,-59.0288384007668,-125.292242378034));
#50420=CARTESIAN_POINT('',(57.5,-59.4850762228408,-125.08223311503));
#50421=CARTESIAN_POINT('',(57.5,-59.1970922754756,-125.765473267224));
#50422=CARTESIAN_POINT('',(57.5,-59.1970922754756,-125.765473267224));
#50423=CARTESIAN_POINT('',(58.,-59.0288384007668,-125.292242378034));
#50424=CARTESIAN_POINT('Origin',(57.5,-57.5822796533797,-125.969521727281));
#50425=CARTESIAN_POINT('',(57.5,-58.2907844884389,-126.188091528965));
#50426=CARTESIAN_POINT('',(58.,-58.036420101407,-125.755014631118));
#50427=CARTESIAN_POINT('',(57.5,-58.2907844884389,-126.188091528965));
#50428=CARTESIAN_POINT('',(57.5,-57.5822796533797,-125.969521727281));
#50429=CARTESIAN_POINT('',(57.5,-57.5822796533797,-125.969521727281));
#50430=CARTESIAN_POINT('',(58.,-58.036420101407,-125.755014631118));
#50431=CARTESIAN_POINT('Origin',(14.,-59.0288384007668,-125.292242378034));
#50432=CARTESIAN_POINT('',(14.5,-59.4850762228408,-125.08223311503));
#50433=CARTESIAN_POINT('',(14.5,-59.1970922754756,-125.765473267224));
#50434=CARTESIAN_POINT('',(14.5,-59.4850762228409,-125.08223311503));
#50435=CARTESIAN_POINT('',(14.,-59.0288384007668,-125.292242378034));
#50436=CARTESIAN_POINT('',(14.,-59.0288384007668,-125.292242378034));
#50437=CARTESIAN_POINT('',(14.5,-59.1970922754756,-125.765473267224));
#50438=CARTESIAN_POINT('Origin',(14.25,-58.4380402379161,-122.84739093989));
#50439=CARTESIAN_POINT('',(14.,-58.2020747272541,-122.929975912966));
#50440=CARTESIAN_POINT('',(14.5,-58.674005748578,-122.764805966813));
#50441=CARTESIAN_POINT('Origin',(14.5,-57.5822796533797,-125.969521727281));
#50442=CARTESIAN_POINT('',(14.,-58.036420101407,-125.755014631118));
#50443=CARTESIAN_POINT('',(14.5,-58.2907844884389,-126.188091528965));
#50444=CARTESIAN_POINT('',(14.,-58.036420101407,-125.755014631118));
#50445=CARTESIAN_POINT('',(14.5,-57.5822796533797,-125.969521727281));
#50446=CARTESIAN_POINT('',(14.5,-57.5822796533797,-125.969521727281));
#50447=CARTESIAN_POINT('',(14.5,-58.2907844884389,-126.188091528965));
#50448=CARTESIAN_POINT('Origin',(14.25,-57.56981106276,-125.459008691224));
#50449=CARTESIAN_POINT('',(14.5,-57.3548715964828,-125.586684161994));
#50450=CARTESIAN_POINT('',(14.,-57.7847505290373,-125.331333220453));
#50451=CARTESIAN_POINT('Origin',(14.,-57.9365320709093,-126.078806628123));
#50452=CARTESIAN_POINT('',(14.,-58.2907844884389,-126.188091528965));
#50453=CARTESIAN_POINT('',(14.,-57.5822796533797,-125.969521727281));
#50454=CARTESIAN_POINT('Origin',(14.25,-59.0914377100404,-125.538896320465));
#50455=CARTESIAN_POINT('',(14.5,-59.1970922754756,-125.765473267224));
#50456=CARTESIAN_POINT('',(14.,-58.9857831446052,-125.312319373706));
#50457=CARTESIAN_POINT('Origin',(14.,-59.3410842491582,-125.423853191127));
#50458=CARTESIAN_POINT('',(14.,-59.4850762228409,-125.08223311503));
#50459=CARTESIAN_POINT('',(14.,-59.1970922754756,-125.765473267224));
#50460=CARTESIAN_POINT('Origin',(57.75,-57.56981106276,-125.459008691224));
#50461=CARTESIAN_POINT('',(58.,-57.7847505290373,-125.331333220453));
#50462=CARTESIAN_POINT('',(57.5,-57.3548715964828,-125.586684161994));
#50463=CARTESIAN_POINT('Origin',(57.75,-59.0914377100404,-125.538896320465));
#50464=CARTESIAN_POINT('',(58.,-58.9857831446052,-125.312319373706));
#50465=CARTESIAN_POINT('',(57.5,-59.1970922754756,-125.765473267224));
#50466=CARTESIAN_POINT('Origin',(57.75,-58.4380402379161,-122.84739093989));
#50467=CARTESIAN_POINT('',(57.5,-58.674005748578,-122.764805966813));
#50468=CARTESIAN_POINT('',(58.,-58.2020747272541,-122.929975912966));
#50469=CARTESIAN_POINT('Origin',(14.,-57.8987018584758,-124.164166824021));
#50470=CARTESIAN_POINT('Origin',(14.,-58.3222962368457,-121.759885683511));
#50471=CARTESIAN_POINT('Origin',(14.,-59.6502461689939,-125.554164136354));
#50472=CARTESIAN_POINT('Origin',(57.5,-46.3841944650247,-130.508796018164));
#50473=CARTESIAN_POINT('',(57.5,-47.070953611875,-130.788284360904));
#50474=CARTESIAN_POINT('',(58.,-46.8553022968291,-130.334686134323));
#50475=CARTESIAN_POINT('',(57.5,-47.070953611875,-130.788284360904));
#50476=CARTESIAN_POINT('',(57.5,-46.3841944650247,-130.508796018164));
#50477=CARTESIAN_POINT('',(57.5,-46.3841944650247,-130.508796018164));
#50478=CARTESIAN_POINT('',(58.,-46.8553022968291,-130.334686134323));
#50479=CARTESIAN_POINT('Origin',(14.,-46.7275740384498,-130.648540189534));
#50480=CARTESIAN_POINT('',(14.2512407024475,-46.7275740384498,-130.648540189534));
#50481=CARTESIAN_POINT('',(14.5,-46.3841944650247,-130.508796018164));
#50482=CARTESIAN_POINT('',(14.3353834448874,-46.6114260219129,-130.601271774103));
#50483=CARTESIAN_POINT('',(14.,-46.3841944650247,-130.508796018164));
#50484=CARTESIAN_POINT('',(14.5,-47.070953611875,-130.788284360904));
#50485=CARTESIAN_POINT('',(14.,-47.070953611875,-130.788284360904));
#50486=CARTESIAN_POINT('',(14.4305329766294,-46.975063500081,-130.749260245167));
#50487=CARTESIAN_POINT('Origin',(57.75,-46.4162674639966,-129.99913892906));
#50488=CARTESIAN_POINT('',(58.,-46.6415166711983,-129.890682510832));
#50489=CARTESIAN_POINT('',(57.5,-46.1910182567949,-130.107595347289));
#50490=CARTESIAN_POINT('Origin',(57.5,-48.0106462326609,-130.446264217578));
#50491=CARTESIAN_POINT('',(57.5,-48.3570826171013,-129.790723455271));
#50492=CARTESIAN_POINT('',(58.,-47.8842774043812,-129.960169823373));
#50493=CARTESIAN_POINT('',(57.5,-48.3570826171013,-129.790723455271));
#50494=CARTESIAN_POINT('',(57.5,-48.0106462326609,-130.446264217578));
#50495=CARTESIAN_POINT('',(57.5,-48.0106462326609,-130.446264217578));
#50496=CARTESIAN_POINT('',(58.,-47.8842774043812,-129.960169823373));
#50497=CARTESIAN_POINT('Origin',(14.,-48.1838644248811,-130.118493836425));
#50498=CARTESIAN_POINT('',(14.2512407024475,-48.1838644248811,-130.118493836425));
#50499=CARTESIAN_POINT('',(14.5,-48.0106462326609,-130.446264217578));
#50500=CARTESIAN_POINT('',(14.2590041943422,-48.1784584841,-130.128723173468));
#50501=CARTESIAN_POINT('',(14.,-48.0106462326609,-130.446264217578));
#50502=CARTESIAN_POINT('',(14.5,-48.3570826171013,-129.790723455271));
#50503=CARTESIAN_POINT('',(14.,-48.3570826171013,-129.790723455271));
#50504=CARTESIAN_POINT('',(14.6801520303733,-48.4825276128585,-129.553351424388));
#50505=CARTESIAN_POINT('Origin',(57.75,-47.9251411968295,-130.211341062382));
#50506=CARTESIAN_POINT('',(58.,-47.8396361609981,-129.976417907185));
#50507=CARTESIAN_POINT('',(57.5,-48.0106462326609,-130.446264217578));
#50508=CARTESIAN_POINT('Origin',(57.75,-47.5088102499061,-127.473130330375));
#50509=CARTESIAN_POINT('',(57.5,-47.7510755952283,-127.411425367399));
#50510=CARTESIAN_POINT('',(58.,-47.2665449045839,-127.534835293351));
#50511=CARTESIAN_POINT('Origin',(14.25,-46.4162674639966,-129.99913892906));
#50512=CARTESIAN_POINT('',(14.,-46.8553022968291,-130.334686134323));
#50513=CARTESIAN_POINT('',(14.5,-46.6011073014821,-130.959294432567));
#50514=CARTESIAN_POINT('',(14.,-46.6415166711983,-129.890682510832));
#50515=CARTESIAN_POINT('',(14.5,-46.1910182567949,-130.107595347289));
#50516=CARTESIAN_POINT('Origin',(14.,-48.4804925430539,-130.275254145916));
#50517=CARTESIAN_POINT('',(14.5,-48.0106462326609,-130.446264217578));
#50518=CARTESIAN_POINT('Origin',(14.25,-47.9251411968295,-130.211341062382));
#50519=CARTESIAN_POINT('',(14.,-47.8842774043812,-129.960169823373));
#50520=CARTESIAN_POINT('',(14.,-47.8842774043812,-129.960169823373));
#50521=CARTESIAN_POINT('',(14.,-47.8396361609981,-129.976417907185));
#50522=CARTESIAN_POINT('Origin',(14.25,-47.5088102499061,-127.473130330375));
#50523=CARTESIAN_POINT('',(14.5,-47.7510755952283,-127.411425367399));
#50524=CARTESIAN_POINT('',(14.,-47.2665449045839,-127.534835293351));
#50525=CARTESIAN_POINT('Origin',(14.,-47.4882890180656,-126.379675605442));
#50526=CARTESIAN_POINT('Origin',(14.,-46.6011073014821,-130.959294432567));
#50527=CARTESIAN_POINT('Origin',(57.5,-36.458810182395,-134.134280331629));
#50528=CARTESIAN_POINT('',(57.5,-36.8610624138408,-133.511428020236));
#50529=CARTESIAN_POINT('',(58.,-36.375288143631,-133.639021904261));
#50530=CARTESIAN_POINT('',(57.5,-36.8610624138408,-133.511428020236));
#50531=CARTESIAN_POINT('',(57.5,-36.458810182395,-134.134280331629));
#50532=CARTESIAN_POINT('',(57.5,-36.458810182395,-134.134280331629));
#50533=CARTESIAN_POINT('',(58.,-36.375288143631,-133.639021904261));
#50534=CARTESIAN_POINT('Origin',(57.5,-34.8330975492484,-134.054819567983));
#50535=CARTESIAN_POINT('',(57.5,-35.4928843561059,-134.393099376732));
#50536=CARTESIAN_POINT('',(58.,-35.3175873497673,-133.922431977811));
#50537=CARTESIAN_POINT('',(57.5,-35.4928843561059,-134.393099376732));
#50538=CARTESIAN_POINT('',(57.5,-34.8330975492484,-134.054819567983));
#50539=CARTESIAN_POINT('',(57.5,-34.8330975492484,-134.054819567983));
#50540=CARTESIAN_POINT('',(58.,-35.3175873497673,-133.922431977811));
#50541=CARTESIAN_POINT('Origin',(14.,-36.375288143631,-133.639021904261));
#50542=CARTESIAN_POINT('',(14.5,-36.8610624138408,-133.511428020236));
#50543=CARTESIAN_POINT('',(14.5,-36.458810182395,-134.134280331629));
#50544=CARTESIAN_POINT('',(14.5,-36.8610624138408,-133.511428020236));
#50545=CARTESIAN_POINT('',(14.,-36.375288143631,-133.639021904261));
#50546=CARTESIAN_POINT('',(14.,-36.375288143631,-133.639021904261));
#50547=CARTESIAN_POINT('',(14.5,-36.458810182395,-134.134280331629));
#50548=CARTESIAN_POINT('Origin',(14.25,-36.2180095292904,-131.128722228666));
#50549=CARTESIAN_POINT('',(14.,-35.9712881348696,-131.169077569515));
#50550=CARTESIAN_POINT('',(14.5,-36.4647309237111,-131.088366887817));
#50551=CARTESIAN_POINT('Origin',(14.5,-34.8330975492484,-134.054819567983));
#50552=CARTESIAN_POINT('',(14.,-35.3175873497673,-133.922431977811));
#50553=CARTESIAN_POINT('',(14.5,-35.4928843561059,-134.393099376732));
#50554=CARTESIAN_POINT('',(14.,-35.3175873497673,-133.922431977811));
#50555=CARTESIAN_POINT('',(14.5,-34.8330975492484,-134.054819567983));
#50556=CARTESIAN_POINT('',(14.5,-34.8330975492484,-134.054819567983));
#50557=CARTESIAN_POINT('',(14.5,-35.4928843561059,-134.393099376732));
#50558=CARTESIAN_POINT('Origin',(14.25,-34.9094680429236,-133.549897224021));
#50559=CARTESIAN_POINT('',(14.5,-34.6756233772734,-133.638309170877));
#50560=CARTESIAN_POINT('',(14.,-35.1433127085738,-133.461485277164));
#50561=CARTESIAN_POINT('Origin',(14.,-35.1629909526772,-134.223959472357));
#50562=CARTESIAN_POINT('',(14.,-35.4928843561059,-134.393099376732));
#50563=CARTESIAN_POINT('',(14.,-34.8330975492484,-134.054819567983));
#50564=CARTESIAN_POINT('Origin',(14.25,-36.3941054211193,-133.892798875057));
#50565=CARTESIAN_POINT('',(14.5,-36.458810182395,-134.134280331629));
#50566=CARTESIAN_POINT('',(14.,-36.3294006598437,-133.651317418485));
#50567=CARTESIAN_POINT('Origin',(14.,-36.6599362981179,-133.822854175933));
#50568=CARTESIAN_POINT('',(14.,-36.8610624138408,-133.511428020236));
#50569=CARTESIAN_POINT('',(14.,-36.458810182395,-134.134280331629));
#50570=CARTESIAN_POINT('Origin',(57.75,-34.9094680429236,-133.549897224021));
#50571=CARTESIAN_POINT('',(58.,-35.1433127085738,-133.461485277164));
#50572=CARTESIAN_POINT('',(57.5,-34.6756233772734,-133.638309170877));
#50573=CARTESIAN_POINT('Origin',(57.75,-36.3941054211193,-133.892798875057));
#50574=CARTESIAN_POINT('',(58.,-36.3294006598437,-133.651317418485));
#50575=CARTESIAN_POINT('',(57.5,-36.458810182395,-134.134280331629));
#50576=CARTESIAN_POINT('Origin',(57.75,-36.2180095292904,-131.128722228666));
#50577=CARTESIAN_POINT('',(57.5,-36.4647309237111,-131.088366887817));
#50578=CARTESIAN_POINT('',(58.,-35.9712881348696,-131.169077569515));
#50579=CARTESIAN_POINT('Origin',(14.,-35.4582091790454,-132.331838201602));
#50580=CARTESIAN_POINT('Origin',(14.,-36.292867245645,-130.037639885881));
#50581=CARTESIAN_POINT('Origin',(14.,-36.9417730955395,-134.004870809078));
#50582=CARTESIAN_POINT('Origin',(57.5,-24.6295005722095,-136.801453579863));
#50583=CARTESIAN_POINT('',(57.5,-25.0845072682929,-136.216030001563));
#50584=CARTESIAN_POINT('',(58.,-24.5894609761083,-136.30080033501));
#50585=CARTESIAN_POINT('',(57.5,-25.0845072682929,-136.216030001563));
#50586=CARTESIAN_POINT('',(57.5,-24.6295005722095,-136.801453579863));
#50587=CARTESIAN_POINT('',(57.5,-24.6295005722095,-136.801453579863));
#50588=CARTESIAN_POINT('',(58.,-24.5894609761083,-136.30080033501));
#50589=CARTESIAN_POINT('Origin',(57.5,-23.016899728323,-136.580604996376));
#50590=CARTESIAN_POINT('',(57.5,-23.6446928191973,-136.97510175753));
#50591=CARTESIAN_POINT('',(58.,-23.5110842376315,-136.490947249372));
#50592=CARTESIAN_POINT('',(57.5,-23.6446928191973,-136.97510175753));
#50593=CARTESIAN_POINT('',(57.5,-23.016899728323,-136.580604996376));
#50594=CARTESIAN_POINT('',(57.5,-23.016899728323,-136.580604996376));
#50595=CARTESIAN_POINT('',(58.,-23.5110842376315,-136.490947249372));
#50596=CARTESIAN_POINT('Origin',(14.,-24.5894609761083,-136.30080033501));
#50597=CARTESIAN_POINT('',(14.5,-25.0845072682929,-136.216030001563));
#50598=CARTESIAN_POINT('',(14.5,-24.6295005722095,-136.801453579863));
#50599=CARTESIAN_POINT('',(14.5,-25.0845072682929,-136.216030001563));
#50600=CARTESIAN_POINT('',(14.,-24.5894609761083,-136.30080033501));
#50601=CARTESIAN_POINT('',(14.,-24.5894609761083,-136.30080033501));
#50602=CARTESIAN_POINT('',(14.5,-24.6295005722095,-136.801453579863));
#50603=CARTESIAN_POINT('Origin',(14.25,-24.6515678871247,-133.786345373109));
#50604=CARTESIAN_POINT('',(14.,-24.4022681423913,-133.805043963321));
#50605=CARTESIAN_POINT('',(14.5,-24.900867631858,-133.767646782898));
#50606=CARTESIAN_POINT('Origin',(14.5,-23.016899728323,-136.580604996376));
#50607=CARTESIAN_POINT('',(14.,-23.5110842376315,-136.490947249372));
#50608=CARTESIAN_POINT('',(14.5,-23.6446928191973,-136.97510175753));
#50609=CARTESIAN_POINT('',(14.,-23.5110842376315,-136.490947249372));
#50610=CARTESIAN_POINT('',(14.5,-23.016899728323,-136.580604996376));
#50611=CARTESIAN_POINT('',(14.5,-23.016899728323,-136.580604996376));
#50612=CARTESIAN_POINT('',(14.5,-23.6446928191973,-136.97510175753));
#50613=CARTESIAN_POINT('Origin',(14.25,-23.1369864911308,-136.084260161474));
#50614=CARTESIAN_POINT('',(14.5,-22.896326066137,-136.151954768658));
#50615=CARTESIAN_POINT('',(14.,-23.3776469161246,-136.01656555429));
#50616=CARTESIAN_POINT('Origin',(14.,-23.3307962737602,-136.777853376953));
#50617=CARTESIAN_POINT('',(14.,-23.6446928191973,-136.97510175753));
#50618=CARTESIAN_POINT('',(14.,-23.016899728323,-136.580604996376));
#50619=CARTESIAN_POINT('Origin',(14.25,-24.5860885277927,-136.55525164161));
#50620=CARTESIAN_POINT('',(14.5,-24.6295005722095,-136.801453579863));
#50621=CARTESIAN_POINT('',(14.,-24.542676483376,-136.309049703357));
#50622=CARTESIAN_POINT('Origin',(14.,-24.8570039202512,-136.508741790713));
#50623=CARTESIAN_POINT('',(14.,-25.0845072682929,-136.216030001563));
#50624=CARTESIAN_POINT('',(14.,-24.6295005722095,-136.801453579863));
#50625=CARTESIAN_POINT('Origin',(57.75,-23.1369864911308,-136.084260161474));
#50626=CARTESIAN_POINT('',(58.,-23.3776469161246,-136.01656555429));
#50627=CARTESIAN_POINT('',(57.5,-22.896326066137,-136.151954768658));
#50628=CARTESIAN_POINT('Origin',(57.75,-24.5860885277927,-136.55525164161));
#50629=CARTESIAN_POINT('',(58.,-24.542676483376,-136.309049703357));
#50630=CARTESIAN_POINT('',(57.5,-24.6295005722095,-136.801453579863));
#50631=CARTESIAN_POINT('Origin',(57.75,-24.6515678871247,-133.786345373109));
#50632=CARTESIAN_POINT('',(57.5,-24.900867631858,-133.767646782898));
#50633=CARTESIAN_POINT('',(58.,-24.4022681423913,-133.805043963321));
#50634=CARTESIAN_POINT('Origin',(14.,-23.7898003403695,-134.918662162672));
#50635=CARTESIAN_POINT('Origin',(14.,-24.8212348392527,-132.705939207914));
#50636=CARTESIAN_POINT('Origin',(14.,-25.1219044487156,-136.71462949103));
#50637=CARTESIAN_POINT('Origin',(57.75,-12.8975129283142,-135.425773646859));
#50638=CARTESIAN_POINT('',(57.7487592975525,-12.864894733482,-138.155715454235));
#50639=CARTESIAN_POINT('',(58.,-12.6164931630349,-137.925247374536));
#50640=CARTESIAN_POINT('',(58.2319907935076,-12.3871239689705,-137.712437618128));
#50641=CARTESIAN_POINT('',(58.,-12.647532154857,-135.422673178871));
#50642=CARTESIAN_POINT('',(57.5,-13.1170438759937,-137.883945745091));
#50643=CARTESIAN_POINT('',(57.5,-13.1474937017714,-135.428874114848));
#50644=CARTESIAN_POINT('',(50.4896657310027,-20.2229080267582,-130.225150580314));
#50645=CARTESIAN_POINT('Origin',(58.,-11.9403367564292,-136.478673638569));
#50646=CARTESIAN_POINT('',(58.,-11.5256475780664,-138.020683996878));
#50647=CARTESIAN_POINT('',(58.,-12.5691677195965,-137.929387814333));
#50648=CARTESIAN_POINT('',(58.,-11.4340631148344,-137.536477638499));
#50649=CARTESIAN_POINT('Origin',(57.75,-12.5909566552834,-138.178436488856));
#50650=CARTESIAN_POINT('',(57.5,-12.6127455909704,-138.427485163379));
#50651=CARTESIAN_POINT('',(57.5,-12.6127455909704,-138.427485163379));
#50652=CARTESIAN_POINT('',(57.5,-11.6165508928786,-138.514640906126));
#50653=CARTESIAN_POINT('',(57.5,-12.6127455909704,-138.427485163379));
#50654=CARTESIAN_POINT('',(57.5,-11.6165508928786,-138.514640906126));
#50655=CARTESIAN_POINT('Origin',(14.,-12.864894733482,-138.155715454235));
#50656=CARTESIAN_POINT('',(14.5,-13.1170438759937,-137.883945745091));
#50657=CARTESIAN_POINT('',(14.,-13.1170438759937,-137.883945745091));
#50658=CARTESIAN_POINT('',(14.5,-12.6127455909704,-138.427485163379));
#50659=CARTESIAN_POINT('',(14.5,-13.1170438759937,-137.883945745091));
#50660=CARTESIAN_POINT('',(14.,-12.6127455909704,-138.427485163379));
#50661=CARTESIAN_POINT('Origin',(57.5,-11.025529402481,-138.066929551123));
#50662=CARTESIAN_POINT('',(57.5,-11.025529402481,-138.066929551123));
#50663=CARTESIAN_POINT('',(57.5,-11.025529402481,-138.066929551123));
#50664=CARTESIAN_POINT('',(58.,-11.5256475780664,-138.020683996878));
#50665=CARTESIAN_POINT('Origin',(14.,-12.6164931630349,-137.925247374536));
#50666=CARTESIAN_POINT('',(14.,-12.6164931630349,-137.925247374536));
#50667=CARTESIAN_POINT('',(14.,-12.6164931630349,-137.925247374536));
#50668=CARTESIAN_POINT('',(14.5,-12.6127455909704,-138.427485163379));
#50669=CARTESIAN_POINT('Origin',(14.25,-12.8975129283142,-135.425773646859));
#50670=CARTESIAN_POINT('',(14.,-12.647532154857,-135.422673178871));
#50671=CARTESIAN_POINT('',(14.5,-13.1474937017714,-135.428874114848));
#50672=CARTESIAN_POINT('Origin',(14.5,-11.025529402481,-138.066929551123));
#50673=CARTESIAN_POINT('',(14.,-11.5256475780664,-138.020683996878));
#50674=CARTESIAN_POINT('',(14.5,-11.6165508928786,-138.514640906126));
#50675=CARTESIAN_POINT('',(14.,-11.5256475780664,-138.020683996878));
#50676=CARTESIAN_POINT('',(14.5,-11.025529402481,-138.066929551123));
#50677=CARTESIAN_POINT('',(14.5,-11.025529402481,-138.066929551123));
#50678=CARTESIAN_POINT('',(14.5,-11.6165508928786,-138.514640906126));
#50679=CARTESIAN_POINT('Origin',(14.25,-11.188418501646,-137.582939709175));
#50680=CARTESIAN_POINT('',(14.5,-10.9427738884575,-137.629401779851));
#50681=CARTESIAN_POINT('',(14.,-11.4340631148344,-137.536477638499));
#50682=CARTESIAN_POINT('Origin',(14.,-11.3210401476798,-138.290785228625));
#50683=CARTESIAN_POINT('',(14.,-11.6165508928786,-138.514640906126));
#50684=CARTESIAN_POINT('',(14.,-11.025529402481,-138.066929551123));
#50685=CARTESIAN_POINT('Origin',(14.25,-12.5909566552834,-138.178436488856));
#50686=CARTESIAN_POINT('',(14.5,-12.6127455909704,-138.427485163379));
#50687=CARTESIAN_POINT('',(14.,-12.5691677195965,-137.929387814333));
#50688=CARTESIAN_POINT('Origin',(57.75,-11.188418501646,-137.582939709175));
#50689=CARTESIAN_POINT('',(57.5,-10.9427738884575,-137.629401779851));
#50690=CARTESIAN_POINT('Origin',(14.,-13.1606978482623,-134.364266202539));
#50691=CARTESIAN_POINT('Origin',(14.,-13.1108429400162,-138.383907292005));
#50692=CARTESIAN_POINT('Origin',(57.5,-0.500000000000016,-139.));
#50693=CARTESIAN_POINT('',(57.5,-1.04975185951052,-138.502481404895));
#50694=CARTESIAN_POINT('',(58.,-0.547506218943973,-138.5));
#50695=CARTESIAN_POINT('',(57.5,-1.04975185951052,-138.502481404895));
#50696=CARTESIAN_POINT('',(57.5,-0.500000000000016,-139.));
#50697=CARTESIAN_POINT('',(57.5,-0.500000000000016,-139.));
#50698=CARTESIAN_POINT('',(58.,-0.547506218943973,-138.5));
#50699=CARTESIAN_POINT('Origin',(57.5,1.04975185951048,-138.502481404895));
#50700=CARTESIAN_POINT('',(57.5,0.499999999999983,-139.));
#50701=CARTESIAN_POINT('',(58.,0.54750621894394,-138.5));
#50702=CARTESIAN_POINT('',(57.5,0.499999999999983,-139.));
#50703=CARTESIAN_POINT('',(57.5,1.04975185951048,-138.502481404895));
#50704=CARTESIAN_POINT('',(57.5,1.04975185951048,-138.502481404895));
#50705=CARTESIAN_POINT('',(58.,0.54750621894394,-138.5));
#50706=CARTESIAN_POINT('Origin',(14.,-0.547506218943975,-138.5));
#50707=CARTESIAN_POINT('',(14.5,-1.04975185951052,-138.502481404895));
#50708=CARTESIAN_POINT('',(14.5,-0.500000000000016,-139.));
#50709=CARTESIAN_POINT('',(14.5,-1.04975185951052,-138.502481404895));
#50710=CARTESIAN_POINT('',(14.,-0.547506218943975,-138.5));
#50711=CARTESIAN_POINT('',(14.,-0.547506218943975,-138.5));
#50712=CARTESIAN_POINT('',(14.5,-0.500000000000016,-139.));
#50713=CARTESIAN_POINT('Origin',(14.25,-1.04530010838811,-136.034530010839));
#50714=CARTESIAN_POINT('',(14.,-0.796540810835615,-136.009654081084));
#50715=CARTESIAN_POINT('',(14.5,-1.29405940594061,-136.059405940594));
#50716=CARTESIAN_POINT('Origin',(14.5,1.04975185951048,-138.502481404895));
#50717=CARTESIAN_POINT('',(14.,0.54750621894394,-138.5));
#50718=CARTESIAN_POINT('',(14.5,0.499999999999983,-139.));
#50719=CARTESIAN_POINT('',(14.,0.547506218943941,-138.5));
#50720=CARTESIAN_POINT('',(14.5,1.04975185951048,-138.502481404895));
#50721=CARTESIAN_POINT('',(14.5,1.04975185951048,-138.502481404895));
#50722=CARTESIAN_POINT('',(14.5,0.499999999999983,-139.));
#50723=CARTESIAN_POINT('Origin',(14.25,0.84530010838808,-138.034530010839));
#50724=CARTESIAN_POINT('',(14.5,1.09405940594058,-138.059405940594));
#50725=CARTESIAN_POINT('',(14.,0.596540810835583,-138.009654081084));
#50726=CARTESIAN_POINT('Origin',(14.,0.774875929755232,-138.751240702448));
#50727=CARTESIAN_POINT('',(14.,0.499999999999983,-139.));
#50728=CARTESIAN_POINT('',(14.,1.04975185951048,-138.502481404895));
#50729=CARTESIAN_POINT('Origin',(14.25,-0.500000000000017,-138.75));
#50730=CARTESIAN_POINT('',(14.5,-0.500000000000017,-139.));
#50731=CARTESIAN_POINT('',(14.,-0.500000000000017,-138.5));
#50732=CARTESIAN_POINT('Origin',(14.,-0.774875929755266,-138.751240702448));
#50733=CARTESIAN_POINT('',(14.,-1.04975185951052,-138.502481404895));
#50734=CARTESIAN_POINT('',(14.,-0.500000000000016,-139.));
#50735=CARTESIAN_POINT('Origin',(57.75,0.845300108388081,-138.034530010839));
#50736=CARTESIAN_POINT('',(58.,0.596540810835584,-138.009654081084));
#50737=CARTESIAN_POINT('',(57.5,1.09405940594058,-138.059405940594));
#50738=CARTESIAN_POINT('Origin',(57.75,-0.500000000000017,-138.75));
#50739=CARTESIAN_POINT('',(58.,-0.500000000000017,-138.5));
#50740=CARTESIAN_POINT('',(57.5,-0.500000000000017,-139.));
#50741=CARTESIAN_POINT('Origin',(57.75,-1.04530010838811,-136.034530010839));
#50742=CARTESIAN_POINT('',(57.5,-1.29405940594061,-136.059405940594));
#50743=CARTESIAN_POINT('',(58.,-0.796540810835615,-136.009654081084));
#50744=CARTESIAN_POINT('Origin',(14.,-1.67776611483187E-14,-137.));
#50745=CARTESIAN_POINT('Origin',(14.,-1.40000000000002,-135.));
#50746=CARTESIAN_POINT('Origin',(14.,-1.00000000000002,-139.));
#50747=CARTESIAN_POINT('Origin',(57.5,13.1170438759936,-137.883945745091));
#50748=CARTESIAN_POINT('',(57.5,12.6127455909703,-138.427485163379));
#50749=CARTESIAN_POINT('',(58.,12.6164931630349,-137.925247374536));
#50750=CARTESIAN_POINT('',(57.5,12.6127455909703,-138.427485163379));
#50751=CARTESIAN_POINT('',(57.5,13.1170438759936,-137.883945745091));
#50752=CARTESIAN_POINT('',(57.5,13.1170438759936,-137.883945745091));
#50753=CARTESIAN_POINT('',(58.,12.6164931630349,-137.925247374536));
#50754=CARTESIAN_POINT('Origin',(14.,12.864894733482,-138.155715454235));
#50755=CARTESIAN_POINT('',(14.2512407024475,12.864894733482,-138.155715454235));
#50756=CARTESIAN_POINT('',(14.5,13.1170438759936,-137.883945745091));
#50757=CARTESIAN_POINT('',(14.3353834448875,12.9501840897535,-138.063789448395));
#50758=CARTESIAN_POINT('',(14.,13.1170438759936,-137.883945745091));
#50759=CARTESIAN_POINT('',(14.5,12.6127455909703,-138.427485163379));
#50760=CARTESIAN_POINT('',(14.,12.6127455909703,-138.427485163379));
#50761=CARTESIAN_POINT('',(14.4305329766294,12.6831592420301,-138.351592391039));
#50762=CARTESIAN_POINT('Origin',(57.75,12.8725854741911,-137.435594191592));
#50763=CARTESIAN_POINT('',(58.,12.622604700734,-137.432493723604));
#50764=CARTESIAN_POINT('',(57.5,13.1225662476483,-137.438694659581));
#50765=CARTESIAN_POINT('Origin',(57.5,11.6165508928786,-138.514640906126));
#50766=CARTESIAN_POINT('',(57.5,11.025529402481,-138.066929551123));
#50767=CARTESIAN_POINT('',(58.,11.5256475780664,-138.020683996878));
#50768=CARTESIAN_POINT('',(57.5,11.025529402481,-138.066929551123));
#50769=CARTESIAN_POINT('',(57.5,11.6165508928786,-138.514640906126));
#50770=CARTESIAN_POINT('',(57.5,11.6165508928786,-138.514640906126));
#50771=CARTESIAN_POINT('',(58.,11.5256475780664,-138.020683996878));
#50772=CARTESIAN_POINT('Origin',(14.,11.3210401476798,-138.290785228625));
#50773=CARTESIAN_POINT('',(14.2512407024475,11.3210401476798,-138.290785228625));
#50774=CARTESIAN_POINT('',(14.5,11.6165508928786,-138.514640906126));
#50775=CARTESIAN_POINT('',(14.2590041943422,11.3302626985461,-138.297771507148));
#50776=CARTESIAN_POINT('',(14.,11.6165508928786,-138.514640906126));
#50777=CARTESIAN_POINT('',(14.5,11.025529402481,-138.066929551123));
#50778=CARTESIAN_POINT('',(14.,11.025529402481,-138.066929551123));
#50779=CARTESIAN_POINT('',(14.6801520303733,10.8115198709038,-137.90481277716));
#50780=CARTESIAN_POINT('Origin',(57.75,11.5947619571917,-138.265592231604));
#50781=CARTESIAN_POINT('',(58.,11.5729730215048,-138.016543557081));
#50782=CARTESIAN_POINT('',(57.5,11.6165508928786,-138.514640906126));
#50783=CARTESIAN_POINT('Origin',(57.75,10.8148680765323,-135.607981461541));
#50784=CARTESIAN_POINT('',(57.5,10.5692234633438,-135.654443532217));
#50785=CARTESIAN_POINT('',(58.,11.0605126897207,-135.561519390865));
#50786=CARTESIAN_POINT('Origin',(14.25,12.8725854741911,-137.435594191592));
#50787=CARTESIAN_POINT('',(14.,12.6164931630349,-137.925247374536));
#50788=CARTESIAN_POINT('',(14.5,13.1108429400162,-138.383907292005));
#50789=CARTESIAN_POINT('',(14.,12.622604700734,-137.432493723604));
#50790=CARTESIAN_POINT('',(14.5,13.1225662476483,-137.438694659581));
#50791=CARTESIAN_POINT('Origin',(14.,11.1184535438327,-138.5582187775));
#50792=CARTESIAN_POINT('',(14.5,11.6165508928786,-138.514640906126));
#50793=CARTESIAN_POINT('Origin',(14.25,11.5947619571917,-138.265592231604));
#50794=CARTESIAN_POINT('',(14.,11.5256475780664,-138.020683996878));
#50795=CARTESIAN_POINT('',(14.,11.5256475780664,-138.020683996878));
#50796=CARTESIAN_POINT('',(14.,11.5729730215048,-138.016543557081));
#50797=CARTESIAN_POINT('Origin',(14.25,10.8148680765323,-135.607981461541));
#50798=CARTESIAN_POINT('',(14.5,10.5692234633438,-135.654443532217));
#50799=CARTESIAN_POINT('',(14.,11.0605126897207,-135.561519390865));
#50800=CARTESIAN_POINT('Origin',(14.,10.3713526936054,-134.608302282232));
#50801=CARTESIAN_POINT('Origin',(14.,13.1108429400162,-138.383907292005));
#50802=CARTESIAN_POINT('Origin',(57.5,23.6446928191972,-136.97510175753));
#50803=CARTESIAN_POINT('',(57.5,23.016899728323,-136.580604996376));
#50804=CARTESIAN_POINT('',(58.,23.5110842376314,-136.490947249372));
#50805=CARTESIAN_POINT('',(57.5,23.016899728323,-136.580604996376));
#50806=CARTESIAN_POINT('',(57.5,23.6446928191972,-136.97510175753));
#50807=CARTESIAN_POINT('',(57.5,23.6446928191972,-136.97510175753));
#50808=CARTESIAN_POINT('',(58.,23.5110842376314,-136.490947249372));
#50809=CARTESIAN_POINT('Origin',(57.5,25.0845072682928,-136.216030001563));
#50810=CARTESIAN_POINT('',(57.5,24.6295005722094,-136.801453579863));
#50811=CARTESIAN_POINT('',(58.,24.5894609761082,-136.30080033501));
#50812=CARTESIAN_POINT('',(57.5,24.6295005722094,-136.801453579863));
#50813=CARTESIAN_POINT('',(57.5,25.0845072682928,-136.216030001563));
#50814=CARTESIAN_POINT('',(57.5,25.0845072682928,-136.216030001563));
#50815=CARTESIAN_POINT('',(58.,24.5894609761082,-136.30080033501));
#50816=CARTESIAN_POINT('Origin',(14.,23.5110842376314,-136.490947249372));
#50817=CARTESIAN_POINT('',(14.5,23.016899728323,-136.580604996376));
#50818=CARTESIAN_POINT('',(14.5,23.6446928191972,-136.97510175753));
#50819=CARTESIAN_POINT('',(14.5,23.016899728323,-136.580604996376));
#50820=CARTESIAN_POINT('',(14.,23.5110842376314,-136.490947249372));
#50821=CARTESIAN_POINT('',(14.,23.5110842376314,-136.490947249372));
#50822=CARTESIAN_POINT('',(14.5,23.6446928191972,-136.97510175753));
#50823=CARTESIAN_POINT('Origin',(14.25,22.5927285851944,-134.149374290983));
#50824=CARTESIAN_POINT('',(14.,22.8333890101882,-134.081679683799));
#50825=CARTESIAN_POINT('',(14.5,22.3520681602006,-134.217068898167));
#50826=CARTESIAN_POINT('Origin',(14.5,25.0845072682928,-136.216030001563));
#50827=CARTESIAN_POINT('',(14.,24.5894609761082,-136.30080033501));
#50828=CARTESIAN_POINT('',(14.5,24.6295005722094,-136.801453579863));
#50829=CARTESIAN_POINT('',(14.,24.5894609761082,-136.30080033501));
#50830=CARTESIAN_POINT('',(14.5,25.0845072682928,-136.216030001563));
#50831=CARTESIAN_POINT('',(14.5,25.0845072682928,-136.216030001563));
#50832=CARTESIAN_POINT('',(14.5,24.6295005722094,-136.801453579863));
#50833=CARTESIAN_POINT('Origin',(14.25,24.801902691856,-135.790690514667));
#50834=CARTESIAN_POINT('',(14.5,25.0512024365893,-135.771991924456));
#50835=CARTESIAN_POINT('',(14.,24.5526029471226,-135.809389104878));
#50836=CARTESIAN_POINT('Origin',(14.,24.8570039202511,-136.508741790713));
#50837=CARTESIAN_POINT('',(14.,24.6295005722094,-136.801453579863));
#50838=CARTESIAN_POINT('',(14.,25.0845072682928,-136.216030001563));
#50839=CARTESIAN_POINT('Origin',(14.25,23.6012807747804,-136.728899819277));
#50840=CARTESIAN_POINT('',(14.5,23.6446928191972,-136.97510175753));
#50841=CARTESIAN_POINT('',(14.,23.5578687303637,-136.482697881024));
#50842=CARTESIAN_POINT('Origin',(14.,23.3307962737601,-136.777853376953));
#50843=CARTESIAN_POINT('',(14.,23.016899728323,-136.580604996376));
#50844=CARTESIAN_POINT('',(14.,23.6446928191972,-136.97510175753));
#50845=CARTESIAN_POINT('Origin',(57.75,24.801902691856,-135.790690514667));
#50846=CARTESIAN_POINT('',(58.,24.5526029471226,-135.809389104878));
#50847=CARTESIAN_POINT('',(57.5,25.0512024365893,-135.771991924456));
#50848=CARTESIAN_POINT('Origin',(57.75,23.6012807747804,-136.728899819277));
#50849=CARTESIAN_POINT('',(58.,23.5578687303637,-136.482697881024));
#50850=CARTESIAN_POINT('',(57.5,23.6446928191972,-136.97510175753));
#50851=CARTESIAN_POINT('Origin',(57.75,22.5927285851944,-134.149374290983));
#50852=CARTESIAN_POINT('',(57.5,22.3520681602006,-134.217068898167));
#50853=CARTESIAN_POINT('',(58.,22.8333890101882,-134.081679683799));
#50854=CARTESIAN_POINT('Origin',(14.,23.7898003403694,-134.918662162673));
#50855=CARTESIAN_POINT('Origin',(14.,22.0637731308185,-133.192154105382));
#50856=CARTESIAN_POINT('Origin',(14.,23.1522889426911,-137.061925846364));
#50857=CARTESIAN_POINT('Origin',(57.5,35.4928843561059,-134.393099376732));
#50858=CARTESIAN_POINT('',(57.5,34.8330975492484,-134.054819567983));
#50859=CARTESIAN_POINT('',(58.,35.3175873497673,-133.922431977811));
#50860=CARTESIAN_POINT('',(57.5,34.8330975492484,-134.054819567983));
#50861=CARTESIAN_POINT('',(57.5,35.4928843561059,-134.393099376732));
#50862=CARTESIAN_POINT('',(57.5,35.4928843561059,-134.393099376732));
#50863=CARTESIAN_POINT('',(58.,35.3175873497673,-133.922431977811));
#50864=CARTESIAN_POINT('Origin',(57.5,36.8610624138407,-133.511428020236));
#50865=CARTESIAN_POINT('',(57.5,36.4588101823949,-134.134280331629));
#50866=CARTESIAN_POINT('',(58.,36.375288143631,-133.639021904261));
#50867=CARTESIAN_POINT('',(57.5,36.4588101823949,-134.134280331629));
#50868=CARTESIAN_POINT('',(57.5,36.8610624138407,-133.511428020236));
#50869=CARTESIAN_POINT('',(57.5,36.8610624138407,-133.511428020236));
#50870=CARTESIAN_POINT('',(58.,36.375288143631,-133.639021904261));
#50871=CARTESIAN_POINT('Origin',(14.,35.3175873497673,-133.922431977811));
#50872=CARTESIAN_POINT('',(14.5,34.8330975492484,-134.054819567983));
#50873=CARTESIAN_POINT('',(14.5,35.4928843561059,-134.393099376732));
#50874=CARTESIAN_POINT('',(14.5,34.8330975492484,-134.054819567983));
#50875=CARTESIAN_POINT('',(14.,35.3175873497673,-133.922431977811));
#50876=CARTESIAN_POINT('',(14.,35.3175873497673,-133.922431977811));
#50877=CARTESIAN_POINT('',(14.5,35.4928843561059,-134.393099376732));
#50878=CARTESIAN_POINT('Origin',(14.25,34.1986447874607,-131.669809380463));
#50879=CARTESIAN_POINT('',(14.,34.4324894531109,-131.581397433607));
#50880=CARTESIAN_POINT('',(14.5,33.9648001218105,-131.75822132732));
#50881=CARTESIAN_POINT('Origin',(14.5,36.8610624138407,-133.511428020236));
#50882=CARTESIAN_POINT('',(14.,36.375288143631,-133.639021904261));
#50883=CARTESIAN_POINT('',(14.5,36.4588101823949,-134.134280331629));
#50884=CARTESIAN_POINT('',(14.,36.375288143631,-133.639021904261));
#50885=CARTESIAN_POINT('',(14.5,36.8610624138407,-133.511428020236));
#50886=CARTESIAN_POINT('',(14.5,36.8610624138407,-133.511428020236));
#50887=CARTESIAN_POINT('',(14.5,36.4588101823949,-134.134280331629));
#50888=CARTESIAN_POINT('Origin',(14.25,36.5424624542376,-133.112337690265));
#50889=CARTESIAN_POINT('',(14.5,36.7891838486583,-133.071982349415));
#50890=CARTESIAN_POINT('',(14.,36.2957410598168,-133.152693031114));
#50891=CARTESIAN_POINT('Origin',(14.,36.6599362981178,-133.822854175933));
#50892=CARTESIAN_POINT('',(14.,36.4588101823949,-134.134280331629));
#50893=CARTESIAN_POINT('',(14.,36.8610624138407,-133.511428020236));
#50894=CARTESIAN_POINT('Origin',(14.25,35.4281795948302,-134.151617920159));
#50895=CARTESIAN_POINT('',(14.5,35.4928843561059,-134.393099376732));
#50896=CARTESIAN_POINT('',(14.,35.3634748335546,-133.910136463587));
#50897=CARTESIAN_POINT('Origin',(14.,35.1629909526771,-134.223959472357));
#50898=CARTESIAN_POINT('',(14.,34.8330975492484,-134.054819567983));
#50899=CARTESIAN_POINT('',(14.,35.4928843561059,-134.393099376732));
#50900=CARTESIAN_POINT('Origin',(57.75,36.5424624542376,-133.112337690265));
#50901=CARTESIAN_POINT('',(58.,36.2957410598168,-133.152693031114));
#50902=CARTESIAN_POINT('',(57.5,36.7891838486583,-133.071982349415));
#50903=CARTESIAN_POINT('Origin',(57.75,35.4281795948302,-134.151617920159));
#50904=CARTESIAN_POINT('',(58.,35.3634748335546,-133.910136463587));
#50905=CARTESIAN_POINT('',(57.5,35.4928843561059,-134.393099376732));
#50906=CARTESIAN_POINT('Origin',(57.75,34.1986447874607,-131.669809380463));
#50907=CARTESIAN_POINT('',(57.5,33.9648001218105,-131.75822132732));
#50908=CARTESIAN_POINT('',(58.,34.4324894531109,-131.581397433607));
#50909=CARTESIAN_POINT('Origin',(14.,35.4582091790453,-132.331838201602));
#50910=CARTESIAN_POINT('Origin',(14.,33.5882749320356,-130.762333212168));
#50911=CARTESIAN_POINT('Origin',(14.,35.0099214429613,-134.522508899283));
#50912=CARTESIAN_POINT('Origin',(57.75,45.5442886531881,-128.188157716154));
#50913=CARTESIAN_POINT('',(57.7487592975525,46.7275740384498,-130.648540189534));
#50914=CARTESIAN_POINT('',(58.,46.8553022968291,-130.334686134323));
#50915=CARTESIAN_POINT('',(58.2319907935076,46.9732440941815,-130.044879384841));
#50916=CARTESIAN_POINT('',(58.,45.7695378603898,-128.079701297925));
#50917=CARTESIAN_POINT('',(57.5,46.3841944650246,-130.508796018164));
#50918=CARTESIAN_POINT('',(57.5,45.3190394459863,-128.296614134382));
#50919=CARTESIAN_POINT('',(50.4896657310026,36.7073477519961,-126.570638276569));
#50920=CARTESIAN_POINT('Origin',(58.,46.8567596356166,-128.737889047669));
#50921=CARTESIAN_POINT('',(58.,47.8842774043812,-129.960169823373));
#50922=CARTESIAN_POINT('',(58.,46.8999435402121,-130.318438050511));
#50923=CARTESIAN_POINT('',(58.,47.762646667078,-129.482624563588));
#50924=CARTESIAN_POINT('Origin',(57.75,46.9854485760436,-130.553361205708));
#50925=CARTESIAN_POINT('',(57.5,47.070953611875,-130.788284360904));
#50926=CARTESIAN_POINT('',(57.5,47.070953611875,-130.788284360904));
#50927=CARTESIAN_POINT('',(57.5,48.0106462326609,-130.446264217578));
#50928=CARTESIAN_POINT('',(57.5,47.070953611875,-130.788284360904));
#50929=CARTESIAN_POINT('',(57.5,48.0106462326609,-130.446264217578));
#50930=CARTESIAN_POINT('Origin',(14.,46.7275740384498,-130.648540189534));
#50931=CARTESIAN_POINT('',(14.5,46.3841944650246,-130.508796018164));
#50932=CARTESIAN_POINT('',(14.,46.3841944650246,-130.508796018164));
#50933=CARTESIAN_POINT('',(14.5,47.070953611875,-130.788284360904));
#50934=CARTESIAN_POINT('',(14.5,46.3841944650246,-130.508796018164));
#50935=CARTESIAN_POINT('',(14.,47.070953611875,-130.788284360904));
#50936=CARTESIAN_POINT('Origin',(57.5,48.3570826171013,-129.790723455271));
#50937=CARTESIAN_POINT('',(57.5,48.3570826171013,-129.790723455271));
#50938=CARTESIAN_POINT('',(57.5,48.3570826171013,-129.790723455271));
#50939=CARTESIAN_POINT('',(58.,47.8842774043812,-129.960169823373));
#50940=CARTESIAN_POINT('Origin',(14.,46.8553022968291,-130.334686134323));
#50941=CARTESIAN_POINT('',(14.,46.8553022968291,-130.334686134323));
#50942=CARTESIAN_POINT('',(14.,46.8553022968291,-130.334686134323));
#50943=CARTESIAN_POINT('',(14.5,47.070953611875,-130.788284360904));
#50944=CARTESIAN_POINT('Origin',(14.25,45.544288653188,-128.188157716154));
#50945=CARTESIAN_POINT('',(14.,45.7695378603898,-128.079701297925));
#50946=CARTESIAN_POINT('',(14.5,45.3190394459863,-128.296614134382));
#50947=CARTESIAN_POINT('Origin',(14.5,48.3570826171013,-129.790723455271));
#50948=CARTESIAN_POINT('',(14.,47.8842774043812,-129.960169823373));
#50949=CARTESIAN_POINT('',(14.5,48.0106462326609,-130.446264217578));
#50950=CARTESIAN_POINT('',(14.,47.8842774043812,-129.960169823373));
#50951=CARTESIAN_POINT('',(14.5,48.3570826171013,-129.790723455271));
#50952=CARTESIAN_POINT('',(14.5,48.3570826171013,-129.790723455271));
#50953=CARTESIAN_POINT('',(14.5,48.0106462326609,-130.446264217578));
#50954=CARTESIAN_POINT('Origin',(14.25,48.0049120124002,-129.420919600612));
#50955=CARTESIAN_POINT('',(14.5,48.2471773577224,-129.359214637636));
#50956=CARTESIAN_POINT('',(14.,47.762646667078,-129.482624563588));
#50957=CARTESIAN_POINT('Origin',(14.,48.1838644248811,-130.118493836425));
#50958=CARTESIAN_POINT('',(14.,48.0106462326609,-130.446264217578));
#50959=CARTESIAN_POINT('',(14.,48.3570826171013,-129.790723455271));
#50960=CARTESIAN_POINT('Origin',(14.25,46.9854485760436,-130.553361205708));
#50961=CARTESIAN_POINT('',(14.5,47.070953611875,-130.788284360904));
#50962=CARTESIAN_POINT('',(14.,46.8999435402122,-130.318438050511));
#50963=CARTESIAN_POINT('Origin',(57.75,48.0049120124002,-129.420919600612));
#50964=CARTESIAN_POINT('',(57.5,48.2471773577224,-129.359214637636));
#50965=CARTESIAN_POINT('Origin',(14.,44.857149679865,-127.337332006754));
#50966=CARTESIAN_POINT('Origin',(14.,46.601107301482,-130.959294432567));
#50967=CARTESIAN_POINT('Origin',(57.5,58.2907844884389,-126.188091528965));
#50968=CARTESIAN_POINT('',(57.5,57.5822796533797,-125.969521727281));
#50969=CARTESIAN_POINT('',(58.,58.036420101407,-125.755014631118));
#50970=CARTESIAN_POINT('',(57.5,57.5822796533797,-125.969521727281));
#50971=CARTESIAN_POINT('',(57.5,58.2907844884389,-126.188091528965));
#50972=CARTESIAN_POINT('',(57.5,58.2907844884389,-126.188091528965));
#50973=CARTESIAN_POINT('',(58.,58.036420101407,-125.755014631118));
#50974=CARTESIAN_POINT('Origin',(57.5,59.4850762228408,-125.08223311503));
#50975=CARTESIAN_POINT('',(57.5,59.1970922754755,-125.765473267224));
#50976=CARTESIAN_POINT('',(58.,59.0288384007667,-125.292242378034));
#50977=CARTESIAN_POINT('',(57.5,59.1970922754755,-125.765473267224));
#50978=CARTESIAN_POINT('',(57.5,59.4850762228408,-125.08223311503));
#50979=CARTESIAN_POINT('',(57.5,59.4850762228408,-125.08223311503));
#50980=CARTESIAN_POINT('',(58.,59.0288384007667,-125.292242378034));
#50981=CARTESIAN_POINT('Origin',(14.,58.0364201014069,-125.755014631118));
#50982=CARTESIAN_POINT('',(14.5,57.5822796533797,-125.969521727281));
#50983=CARTESIAN_POINT('',(14.5,58.2907844884389,-126.188091528965));
#50984=CARTESIAN_POINT('',(14.5,57.5822796533797,-125.969521727281));
#50985=CARTESIAN_POINT('',(14.,58.0364201014069,-125.755014631118));
#50986=CARTESIAN_POINT('',(14.,58.0364201014069,-125.755014631118));
#50987=CARTESIAN_POINT('',(14.5,58.2907844884389,-126.188091528965));
#50988=CARTESIAN_POINT('Origin',(14.25,56.5433129818713,-123.730916769498));
#50989=CARTESIAN_POINT('',(14.,56.7582524481486,-123.603241298728));
#50990=CARTESIAN_POINT('',(14.5,56.3283735155941,-123.858592240269));
#50991=CARTESIAN_POINT('Origin',(14.5,59.4850762228408,-125.08223311503));
#50992=CARTESIAN_POINT('',(14.,59.0288384007667,-125.292242378034));
#50993=CARTESIAN_POINT('',(14.5,59.1970922754755,-125.765473267224));
#50994=CARTESIAN_POINT('',(14.,59.0288384007667,-125.292242378034));
#50995=CARTESIAN_POINT('',(14.5,59.4850762228408,-125.08223311503));
#50996=CARTESIAN_POINT('',(14.5,59.4850762228408,-125.08223311503));
#50997=CARTESIAN_POINT('',(14.5,59.1970922754755,-125.765473267224));
#50998=CARTESIAN_POINT('Origin',(14.25,59.1020152039901,-124.744530166311));
#50999=CARTESIAN_POINT('',(14.5,59.3379807146521,-124.661945193235));
#51000=CARTESIAN_POINT('',(14.,58.8660496933282,-124.827115139388));
#51001=CARTESIAN_POINT('Origin',(14.,59.3410842491582,-125.423853191127));
#51002=CARTESIAN_POINT('',(14.,59.1970922754755,-125.765473267224));
#51003=CARTESIAN_POINT('',(14.,59.4850762228408,-125.08223311503));
#51004=CARTESIAN_POINT('Origin',(14.25,58.1851299230037,-125.961514582206));
#51005=CARTESIAN_POINT('',(14.5,58.2907844884389,-126.188091528965));
#51006=CARTESIAN_POINT('',(14.,58.0794753575685,-125.734937635446));
#51007=CARTESIAN_POINT('Origin',(14.,57.9365320709093,-126.078806628123));
#51008=CARTESIAN_POINT('',(14.,57.5822796533797,-125.969521727281));
#51009=CARTESIAN_POINT('',(14.,58.2907844884389,-126.188091528965));
#51010=CARTESIAN_POINT('Origin',(57.75,59.1020152039901,-124.744530166311));
#51011=CARTESIAN_POINT('',(58.,58.8660496933282,-124.827115139388));
#51012=CARTESIAN_POINT('',(57.5,59.3379807146521,-124.661945193235));
#51013=CARTESIAN_POINT('Origin',(57.75,58.1851299230037,-125.961514582206));
#51014=CARTESIAN_POINT('',(58.,58.0794753575685,-125.734937635446));
#51015=CARTESIAN_POINT('',(57.5,58.2907844884389,-126.188091528965));
#51016=CARTESIAN_POINT('Origin',(57.75,56.5433129818713,-123.730916769498));
#51017=CARTESIAN_POINT('',(57.5,56.3283735155941,-123.858592240269));
#51018=CARTESIAN_POINT('',(58.,56.7582524481486,-123.603241298728));
#51019=CARTESIAN_POINT('Origin',(14.,57.8987018584758,-124.164166824021));
#51020=CARTESIAN_POINT('Origin',(14.,55.7846344331431,-122.943216816385));
#51021=CARTESIAN_POINT('Origin',(14.,57.8376305949206,-126.399400659835));
#51022=CARTESIAN_POINT('Origin',(57.5,70.1603524804535,-119.421791454066));
#51023=CARTESIAN_POINT('',(57.5,69.9330127018922,-120.127531126037));
#51024=CARTESIAN_POINT('',(58.,69.7241542943354,-119.670765314673));
#51025=CARTESIAN_POINT('',(57.5,69.9330127018922,-120.127531126037));
#51026=CARTESIAN_POINT('',(57.5,70.1603524804535,-119.421791454066));
#51027=CARTESIAN_POINT('',(57.5,70.1603524804535,-119.421791454066));
#51028=CARTESIAN_POINT('',(58.,69.7241542943354,-119.670765314673));
#51029=CARTESIAN_POINT('Origin',(14.,70.0466825911729,-119.774661290051));
#51030=CARTESIAN_POINT('',(14.2512407024475,70.0466825911729,-119.774661290051));
#51031=CARTESIAN_POINT('',(14.5,70.1603524804535,-119.421791454066));
#51032=CARTESIAN_POINT('',(14.3353834448874,70.0851313901163,-119.655303195635));
#51033=CARTESIAN_POINT('',(14.,70.1603524804535,-119.421791454066));
#51034=CARTESIAN_POINT('',(14.5,69.9330127018922,-120.127531126037));
#51035=CARTESIAN_POINT('',(14.,69.9330127018922,-120.127531126037));
#51036=CARTESIAN_POINT('',(14.4305329766294,69.9647554706364,-120.028990820672));
#51037=CARTESIAN_POINT('Origin',(57.75,69.7493163731052,-119.118759534638));
#51038=CARTESIAN_POINT('',(58.,69.5214465371195,-119.221595996303));
#51039=CARTESIAN_POINT('',(57.5,69.9771862090909,-119.015923072972));
#51040=CARTESIAN_POINT('Origin',(57.5,69.0669872981077,-120.627531126037));
#51041=CARTESIAN_POINT('',(57.5,68.3421289244414,-120.471543313576));
#51042=CARTESIAN_POINT('',(58.,68.7758457056645,-120.218271533617));
#51043=CARTESIAN_POINT('',(57.5,68.3421289244414,-120.471543313576));
#51044=CARTESIAN_POINT('',(57.5,69.0669872981077,-120.627531126037));
#51045=CARTESIAN_POINT('',(57.5,69.0669872981077,-120.627531126037));
#51046=CARTESIAN_POINT('',(58.,68.7758457056645,-120.218271533617));
#51047=CARTESIAN_POINT('Origin',(14.,68.7045581112746,-120.549537219807));
#51048=CARTESIAN_POINT('',(14.2512407024475,68.7045581112746,-120.549537219807));
#51049=CARTESIAN_POINT('',(14.5,69.0669872981077,-120.627531126037));
#51050=CARTESIAN_POINT('',(14.2590041943422,68.7158691098264,-120.551971320018));
#51051=CARTESIAN_POINT('',(14.,69.0669872981077,-120.627531126037));
#51052=CARTESIAN_POINT('',(14.5,68.3421289244414,-120.471543313576));
#51053=CARTESIAN_POINT('',(14.,68.3421289244414,-120.471543313576));
#51054=CARTESIAN_POINT('',(14.6801520303733,68.0796569102617,-120.415059955155));
#51055=CARTESIAN_POINT('Origin',(57.75,68.9419872981077,-120.411024775091));
#51056=CARTESIAN_POINT('',(58.,68.8169872981077,-120.194518424145));
#51057=CARTESIAN_POINT('',(57.5,69.0669872981077,-120.627531126037));
#51058=CARTESIAN_POINT('Origin',(57.75,67.1120085569767,-118.332008835457));
#51059=CARTESIAN_POINT('',(57.5,66.9090146507462,-118.477931671344));
#51060=CARTESIAN_POINT('',(58.,67.3150024632071,-118.18608599957));
#51061=CARTESIAN_POINT('Origin',(14.25,69.7493163731052,-119.118759534638));
#51062=CARTESIAN_POINT('',(14.,69.7241542943354,-119.670765314673));
#51063=CARTESIAN_POINT('',(14.5,70.3660254037844,-119.877531126037));
#51064=CARTESIAN_POINT('',(14.,69.5214465371195,-119.221595996303));
#51065=CARTESIAN_POINT('',(14.5,69.9771862090909,-119.015923072972));
#51066=CARTESIAN_POINT('Origin',(14.,68.6339745962155,-120.877531126037));
#51067=CARTESIAN_POINT('',(14.5,69.0669872981077,-120.627531126037));
#51068=CARTESIAN_POINT('Origin',(14.25,68.9419872981077,-120.411024775091));
#51069=CARTESIAN_POINT('',(14.,68.7758457056645,-120.218271533617));
#51070=CARTESIAN_POINT('',(14.,68.7758457056645,-120.218271533617));
#51071=CARTESIAN_POINT('',(14.,68.8169872981077,-120.194518424145));
#51072=CARTESIAN_POINT('Origin',(14.25,67.1120085569767,-118.332008835457));
#51073=CARTESIAN_POINT('',(14.5,66.9090146507462,-118.477931671344));
#51074=CARTESIAN_POINT('',(14.,67.3150024632071,-118.18608599957));
#51075=CARTESIAN_POINT('Origin',(14.,66.2875644347017,-117.613429510899));
#51076=CARTESIAN_POINT('Origin',(14.,70.3660254037844,-119.877531126037));
#51077=CARTESIAN_POINT('Origin',(57.5,79.3175486306509,-114.148922374345));
#51078=CARTESIAN_POINT('',(57.5,78.5818533282824,-114.056703712549));
#51079=CARTESIAN_POINT('',(58.,78.9918455961109,-113.766594799967));
#51080=CARTESIAN_POINT('',(57.5,78.5818533282824,-114.056703712549));
#51081=CARTESIAN_POINT('',(57.5,79.3175486306509,-114.148922374345));
#51082=CARTESIAN_POINT('',(57.5,79.3175486306509,-114.148922374345));
#51083=CARTESIAN_POINT('',(58.,78.9918455961109,-113.766594799967));
#51084=CARTESIAN_POINT('Origin',(57.5,80.3016660917108,-112.852477851287));
#51085=CARTESIAN_POINT('',(57.5,80.1367006749398,-113.575345937994));
#51086=CARTESIAN_POINT('',(58.,79.8888272731287,-113.138521468083));
#51087=CARTESIAN_POINT('',(57.5,80.1367006749398,-113.575345937994));
#51088=CARTESIAN_POINT('',(57.5,80.3016660917108,-112.852477851287));
#51089=CARTESIAN_POINT('',(57.5,80.3016660917108,-112.852477851287));
#51090=CARTESIAN_POINT('',(58.,79.8888272731287,-113.138521468083));
#51091=CARTESIAN_POINT('Origin',(14.,78.9918455961109,-113.766594799967));
#51092=CARTESIAN_POINT('',(14.5,78.5818533282824,-114.056703712549));
#51093=CARTESIAN_POINT('',(14.5,79.3175486306509,-114.148922374345));
#51094=CARTESIAN_POINT('',(14.5,78.5818533282824,-114.056703712549));
#51095=CARTESIAN_POINT('',(14.,78.9918455961109,-113.766594799967));
#51096=CARTESIAN_POINT('',(14.,78.9918455961109,-113.766594799967));
#51097=CARTESIAN_POINT('',(14.5,79.3175486306509,-114.148922374345));
#51098=CARTESIAN_POINT('Origin',(14.25,77.1699412236247,-112.032522863357));
#51099=CARTESIAN_POINT('',(14.,77.3594446636108,-111.869463223246));
#51100=CARTESIAN_POINT('',(14.5,76.9804377836386,-112.195582503469));
#51101=CARTESIAN_POINT('Origin',(14.5,80.3016660917108,-112.852477851287));
#51102=CARTESIAN_POINT('',(14.,79.8888272731287,-113.138521468083));
#51103=CARTESIAN_POINT('',(14.5,80.1367006749398,-113.575345937994));
#51104=CARTESIAN_POINT('',(14.,79.8888272731287,-113.138521468083));
#51105=CARTESIAN_POINT('',(14.5,80.3016660917108,-112.852477851287));
#51106=CARTESIAN_POINT('',(14.5,80.3016660917108,-112.852477851287));
#51107=CARTESIAN_POINT('',(14.5,80.1367006749398,-113.575345937994));
#51108=CARTESIAN_POINT('Origin',(14.25,79.8657831288322,-112.586423217032));
#51109=CARTESIAN_POINT('',(14.5,80.0838230630982,-112.464117914346));
#51110=CARTESIAN_POINT('',(14.,79.6477431945662,-112.708728519719));
#51111=CARTESIAN_POINT('Origin',(14.,80.2191833833253,-113.213911894641));
#51112=CARTESIAN_POINT('',(14.,80.1367006749398,-113.575345937994));
#51113=CARTESIAN_POINT('',(14.,80.3016660917108,-112.852477851287));
#51114=CARTESIAN_POINT('Origin',(14.25,79.1741545215631,-113.944134363273));
#51115=CARTESIAN_POINT('',(14.5,79.3175486306509,-114.148922374345));
#51116=CARTESIAN_POINT('',(14.,79.0307604124753,-113.739346352201));
#51117=CARTESIAN_POINT('Origin',(14.,78.9497009794667,-114.102813043447));
#51118=CARTESIAN_POINT('',(14.,78.5818533282824,-114.056703712549));
#51119=CARTESIAN_POINT('',(14.,79.3175486306509,-114.148922374345));
#51120=CARTESIAN_POINT('Origin',(57.75,79.8657831288322,-112.586423217032));
#51121=CARTESIAN_POINT('',(58.,79.6477431945662,-112.708728519719));
#51122=CARTESIAN_POINT('',(57.5,80.0838230630982,-112.464117914346));
#51123=CARTESIAN_POINT('Origin',(57.75,79.1741545215631,-113.944134363273));
#51124=CARTESIAN_POINT('',(58.,79.0307604124753,-113.739346352201));
#51125=CARTESIAN_POINT('',(57.5,79.3175486306509,-114.148922374345));
#51126=CARTESIAN_POINT('Origin',(57.75,77.1699412236247,-112.032522863357));
#51127=CARTESIAN_POINT('',(57.5,76.9804377836386,-112.195582503469));
#51128=CARTESIAN_POINT('',(58.,77.3594446636108,-111.869463223246));
#51129=CARTESIAN_POINT('Origin',(14.,78.5799717800933,-112.223830067592));
#51130=CARTESIAN_POINT('Origin',(14.,76.2860060453866,-111.388532989905));
#51131=CARTESIAN_POINT('Origin',(14.,78.9079726085064,-114.435710592521));
#51132=CARTESIAN_POINT('Origin',(57.5,88.9644555248695,-106.801571398381));
#51133=CARTESIAN_POINT('',(57.5,88.223522379275,-106.773823726948));
#51134=CARTESIAN_POINT('',(58.,88.6066698449906,-106.449085585742));
#51135=CARTESIAN_POINT('',(57.5,88.223522379275,-106.773823726948));
#51136=CARTESIAN_POINT('',(57.5,88.9644555248695,-106.801571398381));
#51137=CARTESIAN_POINT('',(57.5,88.9644555248695,-106.801571398381));
#51138=CARTESIAN_POINT('',(58.,88.6066698449906,-106.449085585742));
#51139=CARTESIAN_POINT('Origin',(57.5,89.8318355365387,-105.424288749871));
#51140=CARTESIAN_POINT('',(57.5,89.7304999679885,-106.158783788695));
#51141=CARTESIAN_POINT('',(58.,89.4454980381808,-105.745225158215));
#51142=CARTESIAN_POINT('',(57.5,89.7304999679885,-106.158783788695));
#51143=CARTESIAN_POINT('',(57.5,89.8318355365387,-105.424288749871));
#51144=CARTESIAN_POINT('',(57.5,89.8318355365387,-105.424288749871));
#51145=CARTESIAN_POINT('',(58.,89.4454980381808,-105.745225158215));
#51146=CARTESIAN_POINT('Origin',(14.,88.6066698449906,-106.449085585742));
#51147=CARTESIAN_POINT('',(14.5,88.223522379275,-106.773823726948));
#51148=CARTESIAN_POINT('',(14.5,88.9644555248695,-106.801571398381));
#51149=CARTESIAN_POINT('',(14.5,88.223522379275,-106.773823726948));
#51150=CARTESIAN_POINT('',(14.,88.6066698449906,-106.449085585742));
#51151=CARTESIAN_POINT('',(14.,88.6066698449906,-106.449085585742));
#51152=CARTESIAN_POINT('',(14.5,88.9644555248695,-106.801571398381));
#51153=CARTESIAN_POINT('Origin',(14.25,86.6405640410765,-104.880401745181));
#51154=CARTESIAN_POINT('',(14.,86.8151347792147,-104.701446283163));
#51155=CARTESIAN_POINT('',(14.5,86.4659933029384,-105.059357207198));
#51156=CARTESIAN_POINT('Origin',(14.5,89.8318355365387,-105.424288749871));
#51157=CARTESIAN_POINT('',(14.,89.4454980381808,-105.745225158215));
#51158=CARTESIAN_POINT('',(14.5,89.7304999679885,-106.158783788695));
#51159=CARTESIAN_POINT('',(14.,89.4454980381808,-105.745225158215));
#51160=CARTESIAN_POINT('',(14.5,89.8318355365387,-105.424288749871));
#51161=CARTESIAN_POINT('',(14.5,89.8318355365387,-105.424288749871));
#51162=CARTESIAN_POINT('',(14.5,89.7304999679885,-106.158783788695));
#51163=CARTESIAN_POINT('Origin',(14.25,89.3744230506705,-105.197236237204));
#51164=CARTESIAN_POINT('',(14.5,89.5809736676609,-105.0563929107));
#51165=CARTESIAN_POINT('',(14.,89.1678724336801,-105.338079563709));
#51166=CARTESIAN_POINT('Origin',(14.,89.7811677522636,-105.791536269283));
#51167=CARTESIAN_POINT('',(14.,89.7304999679885,-106.158783788695));
#51168=CARTESIAN_POINT('',(14.,89.8318355365387,-105.424288749871));
#51169=CARTESIAN_POINT('Origin',(14.25,88.8037586224479,-106.610060287601));
#51170=CARTESIAN_POINT('',(14.5,88.9644555248695,-106.801571398381));
#51171=CARTESIAN_POINT('',(14.,88.6430617200262,-106.418549176822));
#51172=CARTESIAN_POINT('Origin',(14.,88.5939889520722,-106.787697562665));
#51173=CARTESIAN_POINT('',(14.,88.223522379275,-106.773823726948));
#51174=CARTESIAN_POINT('',(14.,88.9644555248695,-106.801571398381));
#51175=CARTESIAN_POINT('Origin',(57.75,89.3744230506705,-105.197236237204));
#51176=CARTESIAN_POINT('',(58.,89.1678724336801,-105.338079563709));
#51177=CARTESIAN_POINT('',(57.5,89.5809736676609,-105.0563929107));
#51178=CARTESIAN_POINT('Origin',(57.75,88.8037586224478,-106.610060287601));
#51179=CARTESIAN_POINT('',(58.,88.6430617200262,-106.418549176822));
#51180=CARTESIAN_POINT('',(57.5,88.9644555248695,-106.801571398381));
#51181=CARTESIAN_POINT('Origin',(57.75,86.6405640410765,-104.880401745181));
#51182=CARTESIAN_POINT('',(57.5,86.4659933029383,-105.059357207198));
#51183=CARTESIAN_POINT('',(58.,86.8151347792147,-104.701446283163));
#51184=CARTESIAN_POINT('Origin',(14.,88.0619025270559,-104.9480887073));
#51185=CARTESIAN_POINT('Origin',(14.,85.7038650873162,-104.315902474623));
#51186=CARTESIAN_POINT('Origin',(14.,88.58143330331,-107.122965203225));
#51187=CARTESIAN_POINT('Origin',(57.75,95.4517998511728,-96.9300774412053));
#51188=CARTESIAN_POINT('',(57.7487592975525,97.5640231742394,-98.6598632232557));
#51189=CARTESIAN_POINT('',(58.,97.5471438341798,-98.3214345544939));
#51190=CARTESIAN_POINT('',(58.2319907935076,97.5315577788306,-98.0089360833189));
#51191=CARTESIAN_POINT('',(58.,95.6101092987371,-96.7365881164045));
#51192=CARTESIAN_POINT('',(57.5,97.1937571541419,-98.6783304709881));
#51193=CARTESIAN_POINT('',(57.5,95.2934904036084,-97.1235667660061));
#51194=CARTESIAN_POINT('',(50.4896657310025,86.7592182449509,-99.1987595801943));
#51195=CARTESIAN_POINT('Origin',(58.,96.873629022557,-96.873629022557));
#51196=CARTESIAN_POINT('',(58.,98.3214345544939,-97.5471438341798));
#51197=CARTESIAN_POINT('',(58.,97.5807358037436,-98.2878425849301));
#51198=CARTESIAN_POINT('',(58.,98.0093803225402,-97.1657442173475));
#51199=CARTESIAN_POINT('Origin',(57.75,97.7575124990402,-98.4646192802268));
#51200=CARTESIAN_POINT('',(57.5,97.9342891943369,-98.6413959755234));
#51201=CARTESIAN_POINT('',(57.5,97.9342891943369,-98.6413959755234));
#51202=CARTESIAN_POINT('',(57.5,98.6413959755234,-97.9342891943369));
#51203=CARTESIAN_POINT('',(57.5,97.9342891943368,-98.6413959755234));
#51204=CARTESIAN_POINT('',(57.5,98.6413959755234,-97.9342891943369));
#51205=CARTESIAN_POINT('Origin',(14.,97.5640231742394,-98.6598632232557));
#51206=CARTESIAN_POINT('',(14.5,97.1937571541419,-98.6783304709881));
#51207=CARTESIAN_POINT('',(14.,97.1937571541419,-98.6783304709881));
#51208=CARTESIAN_POINT('',(14.5,97.9342891943368,-98.6413959755234));
#51209=CARTESIAN_POINT('',(14.5,97.1937571541419,-98.6783304709881));
#51210=CARTESIAN_POINT('',(14.,97.9342891943368,-98.6413959755234));
#51211=CARTESIAN_POINT('Origin',(57.5,98.678330470988,-97.1937571541419));
#51212=CARTESIAN_POINT('',(57.5,98.678330470988,-97.1937571541419));
#51213=CARTESIAN_POINT('',(57.5,98.678330470988,-97.1937571541419));
#51214=CARTESIAN_POINT('',(58.,98.3214345544939,-97.5471438341798));
#51215=CARTESIAN_POINT('Origin',(14.,97.5471438341798,-98.3214345544939));
#51216=CARTESIAN_POINT('',(14.,97.5471438341798,-98.3214345544939));
#51217=CARTESIAN_POINT('',(14.,97.5471438341798,-98.3214345544939));
#51218=CARTESIAN_POINT('',(14.5,97.9342891943369,-98.6413959755234));
#51219=CARTESIAN_POINT('Origin',(14.25,95.4517998511728,-96.9300774412053));
#51220=CARTESIAN_POINT('',(14.,95.6101092987371,-96.7365881164045));
#51221=CARTESIAN_POINT('',(14.5,95.2934904036084,-97.1235667660061));
#51222=CARTESIAN_POINT('Origin',(14.5,98.678330470988,-97.1937571541419));
#51223=CARTESIAN_POINT('',(14.,98.3214345544939,-97.5471438341798));
#51224=CARTESIAN_POINT('',(14.5,98.6413959755234,-97.9342891943369));
#51225=CARTESIAN_POINT('',(14.,98.3214345544939,-97.5471438341798));
#51226=CARTESIAN_POINT('',(14.5,98.678330470988,-97.1937571541419));
#51227=CARTESIAN_POINT('',(14.5,98.678330470988,-97.1937571541419));
#51228=CARTESIAN_POINT('',(14.5,98.6413959755234,-97.9342891943369));
#51229=CARTESIAN_POINT('Origin',(14.25,98.2028696473411,-97.0074347697832));
#51230=CARTESIAN_POINT('',(14.5,98.3963589721419,-96.8491253222189));
#51231=CARTESIAN_POINT('',(14.,98.0093803225402,-97.1657442173475));
#51232=CARTESIAN_POINT('Origin',(14.,98.6598632232557,-97.5640231742394));
#51233=CARTESIAN_POINT('',(14.,98.6413959755234,-97.9342891943369));
#51234=CARTESIAN_POINT('',(14.,98.678330470988,-97.1937571541419));
#51235=CARTESIAN_POINT('Origin',(14.25,97.7575124990402,-98.4646192802268));
#51236=CARTESIAN_POINT('',(14.5,97.9342891943368,-98.6413959755234));
#51237=CARTESIAN_POINT('',(14.,97.5807358037436,-98.2878425849301));
#51238=CARTESIAN_POINT('Origin',(57.75,98.2028696473411,-97.0074347697832));
#51239=CARTESIAN_POINT('',(57.5,98.3963589721419,-96.8491253222189));
#51240=CARTESIAN_POINT('Origin',(14.,94.4694659665227,-96.4493649538451));
#51241=CARTESIAN_POINT('Origin',(14.,97.5807358037436,-98.9949493661167));
#51242=CARTESIAN_POINT('Origin',(57.5,106.158783788695,-89.7304999679885));
#51243=CARTESIAN_POINT('',(57.5,105.424288749871,-89.8318355365387));
#51244=CARTESIAN_POINT('',(58.,105.745225158215,-89.4454980381808));
#51245=CARTESIAN_POINT('',(57.5,105.424288749871,-89.8318355365387));
#51246=CARTESIAN_POINT('',(57.5,106.158783788695,-89.7304999679885));
#51247=CARTESIAN_POINT('',(57.5,106.158783788695,-89.7304999679885));
#51248=CARTESIAN_POINT('',(58.,105.745225158215,-89.4454980381808));
#51249=CARTESIAN_POINT('Origin',(57.5,106.773823726948,-88.223522379275));
#51250=CARTESIAN_POINT('',(57.5,106.801571398381,-88.9644555248695));
#51251=CARTESIAN_POINT('',(58.,106.449085585742,-88.6066698449906));
#51252=CARTESIAN_POINT('',(57.5,106.801571398381,-88.9644555248695));
#51253=CARTESIAN_POINT('',(57.5,106.773823726948,-88.223522379275));
#51254=CARTESIAN_POINT('',(57.5,106.773823726948,-88.223522379275));
#51255=CARTESIAN_POINT('',(58.,106.449085585742,-88.6066698449906));
#51256=CARTESIAN_POINT('Origin',(14.,105.745225158215,-89.4454980381808));
#51257=CARTESIAN_POINT('',(14.5,105.424288749871,-89.8318355365387));
#51258=CARTESIAN_POINT('',(14.5,106.158783788695,-89.7304999679885));
#51259=CARTESIAN_POINT('',(14.5,105.424288749871,-89.8318355365387));
#51260=CARTESIAN_POINT('',(14.,105.745225158215,-89.4454980381808));
#51261=CARTESIAN_POINT('',(14.,105.745225158215,-89.4454980381808));
#51262=CARTESIAN_POINT('',(14.5,106.158783788695,-89.7304999679885));
#51263=CARTESIAN_POINT('Origin',(14.25,103.536589829029,-88.2420567199213));
#51264=CARTESIAN_POINT('',(14.,103.677433155534,-88.0355061029309));
#51265=CARTESIAN_POINT('',(14.5,103.395746502524,-88.4486073369116));
#51266=CARTESIAN_POINT('Origin',(14.5,106.773823726948,-88.223522379275));
#51267=CARTESIAN_POINT('',(14.,106.449085585742,-88.6066698449906));
#51268=CARTESIAN_POINT('',(14.5,106.801571398381,-88.9644555248695));
#51269=CARTESIAN_POINT('',(14.,106.449085585742,-88.6066698449906));
#51270=CARTESIAN_POINT('',(14.5,106.773823726948,-88.223522379275));
#51271=CARTESIAN_POINT('',(14.5,106.773823726948,-88.223522379275));
#51272=CARTESIAN_POINT('',(14.5,106.801571398381,-88.9644555248695));
#51273=CARTESIAN_POINT('Origin',(14.25,106.283933109481,-88.0793481490734));
#51274=CARTESIAN_POINT('',(14.5,106.462888571499,-87.9047774109353));
#51275=CARTESIAN_POINT('',(14.,106.104977647464,-88.2539188872116));
#51276=CARTESIAN_POINT('Origin',(14.,106.787697562665,-88.5939889520723));
#51277=CARTESIAN_POINT('',(14.,106.801571398381,-88.9644555248695));
#51278=CARTESIAN_POINT('',(14.,106.773823726948,-88.223522379275));
#51279=CARTESIAN_POINT('Origin',(14.25,105.967272677915,-89.5698030655668));
#51280=CARTESIAN_POINT('',(14.5,106.158783788695,-89.7304999679885));
#51281=CARTESIAN_POINT('',(14.,105.775761567135,-89.4091061631452));
#51282=CARTESIAN_POINT('Origin',(14.,105.791536269283,-89.7811677522636));
#51283=CARTESIAN_POINT('',(14.,105.424288749871,-89.8318355365387));
#51284=CARTESIAN_POINT('',(14.,106.158783788695,-89.7304999679885));
#51285=CARTESIAN_POINT('Origin',(57.75,106.283933109481,-88.0793481490734));
#51286=CARTESIAN_POINT('',(58.,106.104977647464,-88.2539188872116));
#51287=CARTESIAN_POINT('',(57.5,106.462888571499,-87.9047774109353));
#51288=CARTESIAN_POINT('Origin',(57.75,105.967272677915,-89.5698030655668));
#51289=CARTESIAN_POINT('',(58.,105.775761567135,-89.4091061631452));
#51290=CARTESIAN_POINT('',(57.5,106.158783788695,-89.7304999679885));
#51291=CARTESIAN_POINT('Origin',(57.75,103.536589829029,-88.2420567199213));
#51292=CARTESIAN_POINT('',(57.5,103.395746502524,-88.4486073369116));
#51293=CARTESIAN_POINT('',(58.,103.677433155534,-88.0355061029309));
#51294=CARTESIAN_POINT('Origin',(14.,104.9480887073,-88.0619025270559));
#51295=CARTESIAN_POINT('Origin',(14.,102.516097167501,-87.8487895280494));
#51296=CARTESIAN_POINT('Origin',(14.,105.837389983851,-90.113522189548));
#51297=CARTESIAN_POINT('Origin',(57.5,114.056703712549,-78.5818533282825));
#51298=CARTESIAN_POINT('',(57.5,114.148922374345,-79.317548630651));
#51299=CARTESIAN_POINT('',(58.,113.766594799967,-78.9918455961111));
#51300=CARTESIAN_POINT('',(57.5,114.148922374345,-79.317548630651));
#51301=CARTESIAN_POINT('',(57.5,114.056703712549,-78.5818533282825));
#51302=CARTESIAN_POINT('',(57.5,114.056703712549,-78.5818533282825));
#51303=CARTESIAN_POINT('',(58.,113.766594799967,-78.9918455961111));
#51304=CARTESIAN_POINT('Origin',(14.,114.102813043447,-78.9497009794668));
#51305=CARTESIAN_POINT('',(14.2512407024475,114.102813043447,-78.9497009794668));
#51306=CARTESIAN_POINT('',(14.5,114.056703712549,-78.5818533282825));
#51307=CARTESIAN_POINT('',(14.3353834448875,114.087216578945,-78.825276644476));
#51308=CARTESIAN_POINT('',(14.,114.056703712549,-78.5818533282825));
#51309=CARTESIAN_POINT('',(14.5,114.148922374345,-79.317548630651));
#51310=CARTESIAN_POINT('',(14.,114.148922374345,-79.317548630651));
#51311=CARTESIAN_POINT('',(14.4305329766294,114.136046160276,-79.2148257108122));
#51312=CARTESIAN_POINT('Origin',(57.75,113.556111664665,-78.4809245051847));
#51313=CARTESIAN_POINT('',(58.,113.393052024553,-78.6704279451708));
#51314=CARTESIAN_POINT('',(57.5,113.719171304777,-78.2914210651986));
#51315=CARTESIAN_POINT('Origin',(57.5,113.575345937994,-80.13670067494));
#51316=CARTESIAN_POINT('',(57.5,112.852477851287,-80.301666091711));
#51317=CARTESIAN_POINT('',(58.,113.138521468083,-79.8888272731288));
#51318=CARTESIAN_POINT('',(57.5,112.852477851287,-80.301666091711));
#51319=CARTESIAN_POINT('',(57.5,113.575345937994,-80.13670067494));
#51320=CARTESIAN_POINT('',(57.5,113.575345937994,-80.13670067494));
#51321=CARTESIAN_POINT('',(58.,113.138521468083,-79.8888272731288));
#51322=CARTESIAN_POINT('Origin',(14.,113.213911894641,-80.2191833833255));
#51323=CARTESIAN_POINT('',(14.2512407024475,113.213911894641,-80.2191833833255));
#51324=CARTESIAN_POINT('',(14.5,113.575345937994,-80.13670067494));
#51325=CARTESIAN_POINT('',(14.2590041943422,113.225191835908,-80.2166091927553));
#51326=CARTESIAN_POINT('',(14.,113.575345937994,-80.13670067494));
#51327=CARTESIAN_POINT('',(14.5,112.852477851287,-80.301666091711));
#51328=CARTESIAN_POINT('',(14.,112.852477851287,-80.301666091711));
#51329=CARTESIAN_POINT('',(14.6801520303733,112.590726522204,-80.3614002505245));
#51330=CARTESIAN_POINT('Origin',(57.75,113.370557926922,-79.9933065658522));
#51331=CARTESIAN_POINT('',(58.,113.16576991585,-79.8499124567644));
#51332=CARTESIAN_POINT('',(57.5,113.575345937994,-80.13670067494));
#51333=CARTESIAN_POINT('Origin',(57.75,110.833403841184,-78.882460664988));
#51334=CARTESIAN_POINT('',(57.5,110.711098538497,-79.100500599254));
#51335=CARTESIAN_POINT('',(58.,110.955709143871,-78.6644207307221));
#51336=CARTESIAN_POINT('Origin',(14.25,113.556111664665,-78.4809245051847));
#51337=CARTESIAN_POINT('',(14.,113.766594799967,-78.991845596111));
#51338=CARTESIAN_POINT('',(14.5,114.435710592521,-78.9079726085065));
#51339=CARTESIAN_POINT('',(14.,113.393052024553,-78.6704279451708));
#51340=CARTESIAN_POINT('',(14.5,113.719171304777,-78.2914210651986));
#51341=CARTESIAN_POINT('Origin',(14.,113.288557719819,-80.5462766970845));
#51342=CARTESIAN_POINT('',(14.5,113.575345937994,-80.13670067494));
#51343=CARTESIAN_POINT('Origin',(14.25,113.370557926922,-79.9933065658522));
#51344=CARTESIAN_POINT('',(14.,113.138521468083,-79.8888272731288));
#51345=CARTESIAN_POINT('',(14.,113.138521468083,-79.8888272731288));
#51346=CARTESIAN_POINT('',(14.,113.16576991585,-79.8499124567644));
#51347=CARTESIAN_POINT('Origin',(14.25,110.833403841184,-78.882460664988));
#51348=CARTESIAN_POINT('',(14.5,110.711098538497,-79.100500599254));
#51349=CARTESIAN_POINT('',(14.,110.955709143871,-78.6644207307221));
#51350=CARTESIAN_POINT('Origin',(14.,109.782518968122,-78.5796317693959));
#51351=CARTESIAN_POINT('Origin',(14.,114.435710592521,-78.9079726085065));
#51352=CARTESIAN_POINT('Origin',(57.5,120.127531126037,-69.9330127018923));
#51353=CARTESIAN_POINT('',(57.5,119.421791454066,-70.1603524804536));
#51354=CARTESIAN_POINT('',(58.,119.670765314673,-69.7241542943355));
#51355=CARTESIAN_POINT('',(57.5,119.421791454066,-70.1603524804536));
#51356=CARTESIAN_POINT('',(57.5,120.127531126037,-69.9330127018923));
#51357=CARTESIAN_POINT('',(57.5,120.127531126037,-69.9330127018923));
#51358=CARTESIAN_POINT('',(58.,119.670765314673,-69.7241542943355));
#51359=CARTESIAN_POINT('Origin',(57.5,120.471543313576,-68.3421289244415));
#51360=CARTESIAN_POINT('',(57.5,120.627531126037,-69.0669872981079));
#51361=CARTESIAN_POINT('',(58.,120.218271533617,-68.7758457056646));
#51362=CARTESIAN_POINT('',(57.5,120.627531126037,-69.0669872981079));
#51363=CARTESIAN_POINT('',(57.5,120.471543313576,-68.3421289244415));
#51364=CARTESIAN_POINT('',(57.5,120.471543313576,-68.3421289244415));
#51365=CARTESIAN_POINT('',(58.,120.218271533617,-68.7758457056646));
#51366=CARTESIAN_POINT('Origin',(14.,119.670765314673,-69.7241542943355));
#51367=CARTESIAN_POINT('',(14.5,119.421791454066,-70.1603524804536));
#51368=CARTESIAN_POINT('',(14.5,120.127531126037,-69.9330127018923));
#51369=CARTESIAN_POINT('',(14.5,119.421791454066,-70.1603524804536));
#51370=CARTESIAN_POINT('',(14.,119.670765314673,-69.7241542943355));
#51371=CARTESIAN_POINT('',(14.,119.670765314673,-69.7241542943355));
#51372=CARTESIAN_POINT('',(14.5,120.127531126037,-69.9330127018923));
#51373=CARTESIAN_POINT('Origin',(14.25,117.286708727069,-68.9225214538622));
#51374=CARTESIAN_POINT('',(14.,117.389545188734,-68.6946516178765));
#51375=CARTESIAN_POINT('',(14.5,117.183872265403,-69.1503912898478));
#51376=CARTESIAN_POINT('Origin',(14.5,120.471543313576,-68.3421289244415));
#51377=CARTESIAN_POINT('',(14.,120.218271533617,-68.7758457056646));
#51378=CARTESIAN_POINT('',(14.5,120.627531126037,-69.0669872981079));
#51379=CARTESIAN_POINT('',(14.,120.218271533617,-68.7758457056646));
#51380=CARTESIAN_POINT('',(14.5,120.471543313576,-68.3421289244415));
#51381=CARTESIAN_POINT('',(14.5,120.471543313576,-68.3421289244415));
#51382=CARTESIAN_POINT('',(14.5,120.627531126037,-69.0669872981079));
#51383=CARTESIAN_POINT('Origin',(14.25,119.964059643026,-68.2852136377336));
#51384=CARTESIAN_POINT('',(14.5,120.109982478913,-68.0822197315032));
#51385=CARTESIAN_POINT('',(14.,119.818136807139,-68.488207543964));
#51386=CARTESIAN_POINT('Origin',(14.,120.549537219807,-68.7045581112747));
#51387=CARTESIAN_POINT('',(14.,120.627531126037,-69.0669872981079));
#51388=CARTESIAN_POINT('',(14.,120.471543313576,-68.3421289244415));
#51389=CARTESIAN_POINT('Origin',(14.25,119.911024775091,-69.8080127018923));
#51390=CARTESIAN_POINT('',(14.5,120.127531126037,-69.9330127018923));
#51391=CARTESIAN_POINT('',(14.,119.694518424145,-69.6830127018923));
#51392=CARTESIAN_POINT('Origin',(14.,119.774661290051,-70.0466825911729));
#51393=CARTESIAN_POINT('',(14.,119.421791454066,-70.1603524804536));
#51394=CARTESIAN_POINT('',(14.,120.127531126037,-69.9330127018923));
#51395=CARTESIAN_POINT('Origin',(57.75,119.964059643026,-68.2852136377336));
#51396=CARTESIAN_POINT('',(58.,119.818136807139,-68.4882075439641));
#51397=CARTESIAN_POINT('',(57.5,120.109982478913,-68.0822197315032));
#51398=CARTESIAN_POINT('Origin',(57.75,119.911024775091,-69.8080127018923));
#51399=CARTESIAN_POINT('',(58.,119.694518424145,-69.6830127018923));
#51400=CARTESIAN_POINT('',(57.5,120.127531126037,-69.9330127018923));
#51401=CARTESIAN_POINT('Origin',(57.75,117.286708727069,-68.9225214538622));
#51402=CARTESIAN_POINT('',(57.5,117.183872265403,-69.1503912898478));
#51403=CARTESIAN_POINT('',(58.,117.389545188734,-68.6946516178765));
#51404=CARTESIAN_POINT('Origin',(14.,118.645480318468,-68.5000000000001));
#51405=CARTESIAN_POINT('Origin',(14.,116.213429510899,-68.7124355652983));
#51406=CARTESIAN_POINT('Origin',(14.,119.877531126037,-70.3660254037845));
#51407=CARTESIAN_POINT('Origin',(57.5,125.765473267224,-59.1970922754756));
#51408=CARTESIAN_POINT('',(57.5,125.08223311503,-59.4850762228409));
#51409=CARTESIAN_POINT('',(58.,125.292242378034,-59.0288384007668));
#51410=CARTESIAN_POINT('',(57.5,125.08223311503,-59.4850762228409));
#51411=CARTESIAN_POINT('',(57.5,125.765473267224,-59.1970922754756));
#51412=CARTESIAN_POINT('',(57.5,125.765473267224,-59.1970922754756));
#51413=CARTESIAN_POINT('',(58.,125.292242378034,-59.0288384007668));
#51414=CARTESIAN_POINT('Origin',(57.5,125.969521727281,-57.5822796533798));
#51415=CARTESIAN_POINT('',(57.5,126.188091528965,-58.290784488439));
#51416=CARTESIAN_POINT('',(58.,125.755014631118,-58.036420101407));
#51417=CARTESIAN_POINT('',(57.5,126.188091528965,-58.290784488439));
#51418=CARTESIAN_POINT('',(57.5,125.969521727281,-57.5822796533798));
#51419=CARTESIAN_POINT('',(57.5,125.969521727281,-57.5822796533798));
#51420=CARTESIAN_POINT('',(58.,125.755014631118,-58.036420101407));
#51421=CARTESIAN_POINT('Origin',(14.,125.292242378034,-59.0288384007668));
#51422=CARTESIAN_POINT('',(14.5,125.08223311503,-59.4850762228409));
#51423=CARTESIAN_POINT('',(14.5,125.765473267224,-59.1970922754756));
#51424=CARTESIAN_POINT('',(14.5,125.08223311503,-59.4850762228409));
#51425=CARTESIAN_POINT('',(14.,125.292242378034,-59.0288384007668));
#51426=CARTESIAN_POINT('',(14.,125.292242378034,-59.0288384007668));
#51427=CARTESIAN_POINT('',(14.5,125.765473267224,-59.1970922754756));
#51428=CARTESIAN_POINT('Origin',(14.25,122.84739093989,-58.4380402379162));
#51429=CARTESIAN_POINT('',(14.,122.929975912966,-58.2020747272542));
#51430=CARTESIAN_POINT('',(14.5,122.764805966813,-58.6740057485781));
#51431=CARTESIAN_POINT('Origin',(14.5,125.969521727281,-57.5822796533798));
#51432=CARTESIAN_POINT('',(14.,125.755014631118,-58.036420101407));
#51433=CARTESIAN_POINT('',(14.5,126.188091528965,-58.290784488439));
#51434=CARTESIAN_POINT('',(14.,125.755014631118,-58.036420101407));
#51435=CARTESIAN_POINT('',(14.5,125.969521727281,-57.5822796533798));
#51436=CARTESIAN_POINT('',(14.5,125.969521727281,-57.5822796533798));
#51437=CARTESIAN_POINT('',(14.5,126.188091528965,-58.290784488439));
#51438=CARTESIAN_POINT('Origin',(14.25,125.459008691224,-57.5698110627601));
#51439=CARTESIAN_POINT('',(14.5,125.586684161994,-57.3548715964829));
#51440=CARTESIAN_POINT('',(14.,125.331333220453,-57.7847505290374));
#51441=CARTESIAN_POINT('Origin',(14.,126.078806628123,-57.9365320709094));
#51442=CARTESIAN_POINT('',(14.,126.188091528965,-58.290784488439));
#51443=CARTESIAN_POINT('',(14.,125.969521727281,-57.5822796533798));
#51444=CARTESIAN_POINT('Origin',(14.25,125.538896320465,-59.0914377100405));
#51445=CARTESIAN_POINT('',(14.5,125.765473267224,-59.1970922754756));
#51446=CARTESIAN_POINT('',(14.,125.312319373706,-58.9857831446053));
#51447=CARTESIAN_POINT('Origin',(14.,125.423853191127,-59.3410842491583));
#51448=CARTESIAN_POINT('',(14.,125.08223311503,-59.4850762228409));
#51449=CARTESIAN_POINT('',(14.,125.765473267224,-59.1970922754756));
#51450=CARTESIAN_POINT('Origin',(57.75,125.459008691224,-57.5698110627601));
#51451=CARTESIAN_POINT('',(58.,125.331333220453,-57.7847505290374));
#51452=CARTESIAN_POINT('',(57.5,125.586684161994,-57.3548715964829));
#51453=CARTESIAN_POINT('Origin',(57.75,125.538896320465,-59.0914377100405));
#51454=CARTESIAN_POINT('',(58.,125.312319373706,-58.9857831446053));
#51455=CARTESIAN_POINT('',(57.5,125.765473267224,-59.1970922754756));
#51456=CARTESIAN_POINT('Origin',(57.75,122.84739093989,-58.4380402379162));
#51457=CARTESIAN_POINT('',(57.5,122.764805966813,-58.6740057485781));
#51458=CARTESIAN_POINT('',(58.,122.929975912966,-58.2020747272542));
#51459=CARTESIAN_POINT('Origin',(14.,124.164166824021,-57.8987018584759));
#51460=CARTESIAN_POINT('Origin',(14.,121.759885683511,-58.3222962368458));
#51461=CARTESIAN_POINT('Origin',(14.,125.554164136354,-59.6502461689939));
#51462=CARTESIAN_POINT('Origin',(57.75,127.473130330375,-47.5088102499062));
#51463=CARTESIAN_POINT('',(57.7487592975525,130.118493836425,-48.1838644248812));
#51464=CARTESIAN_POINT('',(58.,129.960169823373,-47.8842774043812));
#51465=CARTESIAN_POINT('',(58.2319907935076,129.813976499357,-47.6076445581374));
#51466=CARTESIAN_POINT('',(58.,127.534835293351,-47.266544904584));
#51467=CARTESIAN_POINT('',(57.5,129.790723455271,-48.3570826171013));
#51468=CARTESIAN_POINT('',(57.5,127.411425367399,-47.7510755952284));
#51469=CARTESIAN_POINT('',(50.4896657310027,120.553762433226,-53.2385782672432));
#51470=CARTESIAN_POINT('Origin',(58.,128.737889047669,-46.8567596356167));
#51471=CARTESIAN_POINT('',(58.,130.334686134323,-46.8553022968292));
#51472=CARTESIAN_POINT('',(58.,129.976417907185,-47.8396361609982));
#51473=CARTESIAN_POINT('',(58.,129.890682510832,-46.6415166711984));
#51474=CARTESIAN_POINT('Origin',(57.75,130.211341062382,-47.9251411968296));
#51475=CARTESIAN_POINT('',(57.5,130.446264217578,-48.010646232661));
#51476=CARTESIAN_POINT('',(57.5,130.446264217578,-48.010646232661));
#51477=CARTESIAN_POINT('',(57.5,130.788284360904,-47.0709536118751));
#51478=CARTESIAN_POINT('',(57.5,130.446264217578,-48.010646232661));
#51479=CARTESIAN_POINT('',(57.5,130.788284360904,-47.0709536118751));
#51480=CARTESIAN_POINT('Origin',(14.,130.118493836425,-48.1838644248812));
#51481=CARTESIAN_POINT('',(14.5,129.790723455271,-48.3570826171013));
#51482=CARTESIAN_POINT('',(14.,129.790723455271,-48.3570826171013));
#51483=CARTESIAN_POINT('',(14.5,130.446264217578,-48.010646232661));
#51484=CARTESIAN_POINT('',(14.5,129.790723455271,-48.3570826171013));
#51485=CARTESIAN_POINT('',(14.,130.446264217578,-48.010646232661));
#51486=CARTESIAN_POINT('Origin',(57.5,130.508796018163,-46.3841944650247));
#51487=CARTESIAN_POINT('',(57.5,130.508796018163,-46.3841944650247));
#51488=CARTESIAN_POINT('',(57.5,130.508796018163,-46.3841944650247));
#51489=CARTESIAN_POINT('',(58.,130.334686134323,-46.8553022968292));
#51490=CARTESIAN_POINT('Origin',(14.,129.960169823373,-47.8842774043812));
#51491=CARTESIAN_POINT('',(14.,129.960169823373,-47.8842774043812));
#51492=CARTESIAN_POINT('',(14.,129.960169823373,-47.8842774043812));
#51493=CARTESIAN_POINT('',(14.5,130.446264217578,-48.010646232661));
#51494=CARTESIAN_POINT('Origin',(14.25,127.473130330375,-47.5088102499062));
#51495=CARTESIAN_POINT('',(14.,127.534835293351,-47.266544904584));
#51496=CARTESIAN_POINT('',(14.5,127.411425367399,-47.7510755952284));
#51497=CARTESIAN_POINT('Origin',(14.5,130.508796018163,-46.3841944650247));
#51498=CARTESIAN_POINT('',(14.,130.334686134323,-46.8553022968292));
#51499=CARTESIAN_POINT('',(14.5,130.788284360904,-47.0709536118751));
#51500=CARTESIAN_POINT('',(14.,130.334686134323,-46.8553022968292));
#51501=CARTESIAN_POINT('',(14.5,130.508796018163,-46.3841944650247));
#51502=CARTESIAN_POINT('',(14.5,130.508796018163,-46.3841944650247));
#51503=CARTESIAN_POINT('',(14.5,130.788284360904,-47.0709536118751));
#51504=CARTESIAN_POINT('Origin',(14.25,129.99913892906,-46.4162674639967));
#51505=CARTESIAN_POINT('',(14.5,130.107595347289,-46.191018256795));
#51506=CARTESIAN_POINT('',(14.,129.890682510832,-46.6415166711984));
#51507=CARTESIAN_POINT('Origin',(14.,130.648540189534,-46.7275740384499));
#51508=CARTESIAN_POINT('',(14.,130.788284360904,-47.0709536118751));
#51509=CARTESIAN_POINT('',(14.,130.508796018163,-46.3841944650247));
#51510=CARTESIAN_POINT('Origin',(14.25,130.211341062382,-47.9251411968296));
#51511=CARTESIAN_POINT('',(14.5,130.446264217578,-48.010646232661));
#51512=CARTESIAN_POINT('',(14.,129.976417907185,-47.8396361609982));
#51513=CARTESIAN_POINT('Origin',(57.75,129.99913892906,-46.4162674639967));
#51514=CARTESIAN_POINT('',(57.5,130.107595347289,-46.191018256795));
#51515=CARTESIAN_POINT('Origin',(14.,126.379675605442,-47.4882890180656));
#51516=CARTESIAN_POINT('Origin',(14.,130.275254145916,-48.480492543054));
#51517=CARTESIAN_POINT('Origin',(57.5,134.134280331629,-36.4588101823949));
#51518=CARTESIAN_POINT('',(57.5,133.511428020236,-36.8610624138407));
#51519=CARTESIAN_POINT('',(58.,133.639021904261,-36.375288143631));
#51520=CARTESIAN_POINT('',(57.5,133.511428020236,-36.8610624138407));
#51521=CARTESIAN_POINT('',(57.5,134.134280331629,-36.4588101823949));
#51522=CARTESIAN_POINT('',(57.5,134.134280331629,-36.4588101823949));
#51523=CARTESIAN_POINT('',(58.,133.639021904261,-36.375288143631));
#51524=CARTESIAN_POINT('Origin',(57.5,134.054819567983,-34.8330975492484));
#51525=CARTESIAN_POINT('',(57.5,134.393099376732,-35.4928843561058));
#51526=CARTESIAN_POINT('',(58.,133.922431977811,-35.3175873497673));
#51527=CARTESIAN_POINT('',(57.5,134.393099376732,-35.4928843561058));
#51528=CARTESIAN_POINT('',(57.5,134.054819567983,-34.8330975492484));
#51529=CARTESIAN_POINT('',(57.5,134.054819567983,-34.8330975492484));
#51530=CARTESIAN_POINT('',(58.,133.922431977811,-35.3175873497673));
#51531=CARTESIAN_POINT('Origin',(14.,133.639021904261,-36.375288143631));
#51532=CARTESIAN_POINT('',(14.5,133.511428020236,-36.8610624138407));
#51533=CARTESIAN_POINT('',(14.5,134.134280331629,-36.4588101823949));
#51534=CARTESIAN_POINT('',(14.5,133.511428020236,-36.8610624138407));
#51535=CARTESIAN_POINT('',(14.,133.639021904261,-36.3752881436309));
#51536=CARTESIAN_POINT('',(14.,133.639021904261,-36.375288143631));
#51537=CARTESIAN_POINT('',(14.5,134.134280331629,-36.4588101823949));
#51538=CARTESIAN_POINT('Origin',(14.25,131.128722228666,-36.2180095292903));
#51539=CARTESIAN_POINT('',(14.,131.169077569515,-35.9712881348695));
#51540=CARTESIAN_POINT('',(14.5,131.088366887817,-36.4647309237111));
#51541=CARTESIAN_POINT('Origin',(14.5,134.054819567983,-34.8330975492484));
#51542=CARTESIAN_POINT('',(14.,133.922431977811,-35.3175873497673));
#51543=CARTESIAN_POINT('',(14.5,134.393099376732,-35.4928843561058));
#51544=CARTESIAN_POINT('',(14.,133.922431977811,-35.3175873497673));
#51545=CARTESIAN_POINT('',(14.5,134.054819567983,-34.8330975492484));
#51546=CARTESIAN_POINT('',(14.5,134.054819567983,-34.8330975492484));
#51547=CARTESIAN_POINT('',(14.5,134.393099376732,-35.4928843561058));
#51548=CARTESIAN_POINT('Origin',(14.25,133.549897224021,-34.9094680429235));
#51549=CARTESIAN_POINT('',(14.5,133.638309170877,-34.6756233772733));
#51550=CARTESIAN_POINT('',(14.,133.461485277164,-35.1433127085737));
#51551=CARTESIAN_POINT('Origin',(14.,134.223959472357,-35.1629909526771));
#51552=CARTESIAN_POINT('',(14.,134.393099376732,-35.4928843561058));
#51553=CARTESIAN_POINT('',(14.,134.054819567983,-34.8330975492484));
#51554=CARTESIAN_POINT('Origin',(14.25,133.892798875057,-36.3941054211193));
#51555=CARTESIAN_POINT('',(14.5,134.134280331629,-36.4588101823949));
#51556=CARTESIAN_POINT('',(14.,133.651317418485,-36.3294006598436));
#51557=CARTESIAN_POINT('Origin',(14.,133.822854175933,-36.6599362981178));
#51558=CARTESIAN_POINT('',(14.,133.511428020236,-36.8610624138407));
#51559=CARTESIAN_POINT('',(14.,134.134280331629,-36.4588101823949));
#51560=CARTESIAN_POINT('Origin',(57.75,133.549897224021,-34.9094680429235));
#51561=CARTESIAN_POINT('',(58.,133.461485277164,-35.1433127085737));
#51562=CARTESIAN_POINT('',(57.5,133.638309170877,-34.6756233772733));
#51563=CARTESIAN_POINT('Origin',(57.75,133.892798875057,-36.3941054211193));
#51564=CARTESIAN_POINT('',(58.,133.651317418485,-36.3294006598436));
#51565=CARTESIAN_POINT('',(57.5,134.134280331629,-36.4588101823949));
#51566=CARTESIAN_POINT('Origin',(57.75,131.128722228666,-36.2180095292903));
#51567=CARTESIAN_POINT('',(57.5,131.088366887817,-36.4647309237111));
#51568=CARTESIAN_POINT('',(58.,131.169077569515,-35.9712881348695));
#51569=CARTESIAN_POINT('Origin',(14.,132.331838201602,-35.4582091790453));
#51570=CARTESIAN_POINT('Origin',(14.,130.037639885881,-36.292867245645));
#51571=CARTESIAN_POINT('Origin',(14.,134.004870809078,-36.9417730955394));
#51572=CARTESIAN_POINT('Origin',(57.5,136.580604996376,-23.016899728323));
#51573=CARTESIAN_POINT('',(57.5,136.97510175753,-23.6446928191972));
#51574=CARTESIAN_POINT('',(58.,136.490947249372,-23.5110842376315));
#51575=CARTESIAN_POINT('',(57.5,136.97510175753,-23.6446928191972));
#51576=CARTESIAN_POINT('',(57.5,136.580604996376,-23.016899728323));
#51577=CARTESIAN_POINT('',(57.5,136.580604996376,-23.016899728323));
#51578=CARTESIAN_POINT('',(58.,136.490947249372,-23.5110842376315));
#51579=CARTESIAN_POINT('Origin',(14.,136.777853376953,-23.3307962737601));
#51580=CARTESIAN_POINT('',(14.2512407024475,136.777853376953,-23.3307962737601));
#51581=CARTESIAN_POINT('',(14.5,136.580604996376,-23.016899728323));
#51582=CARTESIAN_POINT('',(14.3353834448875,136.711134183553,-23.2246208807783));
#51583=CARTESIAN_POINT('',(14.,136.580604996376,-23.016899728323));
#51584=CARTESIAN_POINT('',(14.5,136.97510175753,-23.6446928191972));
#51585=CARTESIAN_POINT('',(14.,136.97510175753,-23.6446928191972));
#51586=CARTESIAN_POINT('',(14.4305329766294,136.920019362628,-23.5570359602482));
#51587=CARTESIAN_POINT('Origin',(57.75,136.084260161474,-23.1369864911307));
#51588=CARTESIAN_POINT('',(58.,136.01656555429,-23.3776469161245));
#51589=CARTESIAN_POINT('',(57.5,136.151954768658,-22.8963260661369));
#51590=CARTESIAN_POINT('Origin',(57.5,136.801453579863,-24.6295005722094));
#51591=CARTESIAN_POINT('',(57.5,136.216030001563,-25.0845072682928));
#51592=CARTESIAN_POINT('',(58.,136.30080033501,-24.5894609761083));
#51593=CARTESIAN_POINT('',(57.5,136.216030001563,-25.0845072682928));
#51594=CARTESIAN_POINT('',(57.5,136.801453579863,-24.6295005722094));
#51595=CARTESIAN_POINT('',(57.5,136.801453579863,-24.6295005722094));
#51596=CARTESIAN_POINT('',(58.,136.30080033501,-24.5894609761083));
#51597=CARTESIAN_POINT('Origin',(14.,136.508741790713,-24.8570039202511));
#51598=CARTESIAN_POINT('',(14.2512407024475,136.508741790713,-24.8570039202511));
#51599=CARTESIAN_POINT('',(14.5,136.801453579863,-24.6295005722094));
#51600=CARTESIAN_POINT('',(14.2590041943422,136.517876989377,-24.8499038021212));
#51601=CARTESIAN_POINT('',(14.,136.801453579863,-24.6295005722094));
#51602=CARTESIAN_POINT('',(14.5,136.216030001563,-25.0845072682928));
#51603=CARTESIAN_POINT('',(14.,136.216030001563,-25.0845072682928));
#51604=CARTESIAN_POINT('',(14.6801520303733,136.004047480112,-25.2492656932831));
#51605=CARTESIAN_POINT('Origin',(57.75,136.55525164161,-24.5860885277927));
#51606=CARTESIAN_POINT('',(58.,136.309049703357,-24.542676483376));
#51607=CARTESIAN_POINT('',(57.5,136.801453579863,-24.6295005722094));
#51608=CARTESIAN_POINT('Origin',(57.75,133.786345373109,-24.6515678871246));
#51609=CARTESIAN_POINT('',(57.5,133.767646782898,-24.9008676318579));
#51610=CARTESIAN_POINT('',(58.,133.805043963321,-24.4022681423913));
#51611=CARTESIAN_POINT('Origin',(14.25,136.084260161474,-23.1369864911307));
#51612=CARTESIAN_POINT('',(14.,136.490947249372,-23.5110842376314));
#51613=CARTESIAN_POINT('',(14.5,137.061925846364,-23.1522889426911));
#51614=CARTESIAN_POINT('',(14.,136.01656555429,-23.3776469161245));
#51615=CARTESIAN_POINT('',(14.5,136.151954768658,-22.8963260661369));
#51616=CARTESIAN_POINT('Origin',(14.,136.71462949103,-25.1219044487155));
#51617=CARTESIAN_POINT('',(14.5,136.801453579863,-24.6295005722094));
#51618=CARTESIAN_POINT('Origin',(14.25,136.55525164161,-24.5860885277927));
#51619=CARTESIAN_POINT('',(14.,136.30080033501,-24.5894609761083));
#51620=CARTESIAN_POINT('',(14.,136.30080033501,-24.5894609761083));
#51621=CARTESIAN_POINT('',(14.,136.309049703357,-24.542676483376));
#51622=CARTESIAN_POINT('Origin',(14.25,133.786345373109,-24.6515678871246));
#51623=CARTESIAN_POINT('',(14.5,133.767646782898,-24.9008676318579));
#51624=CARTESIAN_POINT('',(14.,133.805043963321,-24.4022681423913));
#51625=CARTESIAN_POINT('Origin',(14.,132.705939207914,-24.8212348392527));
#51626=CARTESIAN_POINT('Origin',(14.,137.061925846364,-23.1522889426911));
#51627=CARTESIAN_POINT('Origin',(57.5,138.427485163379,-12.6127455909704));
#51628=CARTESIAN_POINT('',(57.5,137.883945745091,-13.1170438759937));
#51629=CARTESIAN_POINT('',(58.,137.925247374536,-12.6164931630349));
#51630=CARTESIAN_POINT('',(57.5,137.883945745091,-13.1170438759937));
#51631=CARTESIAN_POINT('',(57.5,138.427485163379,-12.6127455909704));
#51632=CARTESIAN_POINT('',(57.5,138.427485163379,-12.6127455909704));
#51633=CARTESIAN_POINT('',(58.,137.925247374536,-12.6164931630349));
#51634=CARTESIAN_POINT('Origin',(57.5,138.066929551123,-11.025529402481));
#51635=CARTESIAN_POINT('',(57.5,138.514640906126,-11.6165508928786));
#51636=CARTESIAN_POINT('',(58.,138.020683996878,-11.5256475780664));
#51637=CARTESIAN_POINT('',(57.5,138.514640906126,-11.6165508928786));
#51638=CARTESIAN_POINT('',(57.5,138.066929551123,-11.025529402481));
#51639=CARTESIAN_POINT('',(57.5,138.066929551123,-11.025529402481));
#51640=CARTESIAN_POINT('',(58.,138.020683996878,-11.5256475780664));
#51641=CARTESIAN_POINT('Origin',(14.,137.925247374536,-12.6164931630349));
#51642=CARTESIAN_POINT('',(14.5,137.883945745091,-13.1170438759937));
#51643=CARTESIAN_POINT('',(14.5,138.427485163379,-12.6127455909704));
#51644=CARTESIAN_POINT('',(14.5,137.883945745091,-13.1170438759937));
#51645=CARTESIAN_POINT('',(14.,137.925247374536,-12.6164931630349));
#51646=CARTESIAN_POINT('',(14.,137.925247374536,-12.6164931630349));
#51647=CARTESIAN_POINT('',(14.5,138.427485163379,-12.6127455909704));
#51648=CARTESIAN_POINT('Origin',(14.25,135.425773646859,-12.8975129283142));
#51649=CARTESIAN_POINT('',(14.,135.422673178871,-12.647532154857));
#51650=CARTESIAN_POINT('',(14.5,135.428874114848,-13.1474937017714));
#51651=CARTESIAN_POINT('Origin',(14.5,138.066929551123,-11.025529402481));
#51652=CARTESIAN_POINT('',(14.,138.020683996878,-11.5256475780664));
#51653=CARTESIAN_POINT('',(14.5,138.514640906126,-11.6165508928786));
#51654=CARTESIAN_POINT('',(14.,138.020683996878,-11.5256475780664));
#51655=CARTESIAN_POINT('',(14.5,138.066929551123,-11.025529402481));
#51656=CARTESIAN_POINT('',(14.5,138.066929551123,-11.025529402481));
#51657=CARTESIAN_POINT('',(14.5,138.514640906126,-11.6165508928786));
#51658=CARTESIAN_POINT('Origin',(14.25,137.582939709175,-11.188418501646));
#51659=CARTESIAN_POINT('',(14.5,137.629401779851,-10.9427738884575));
#51660=CARTESIAN_POINT('',(14.,137.536477638499,-11.4340631148344));
#51661=CARTESIAN_POINT('Origin',(14.,138.290785228625,-11.3210401476798));
#51662=CARTESIAN_POINT('',(14.,138.514640906126,-11.6165508928786));
#51663=CARTESIAN_POINT('',(14.,138.066929551123,-11.025529402481));
#51664=CARTESIAN_POINT('Origin',(14.25,138.178436488856,-12.5909566552835));
#51665=CARTESIAN_POINT('',(14.5,138.427485163379,-12.6127455909704));
#51666=CARTESIAN_POINT('',(14.,137.929387814333,-12.5691677195965));
#51667=CARTESIAN_POINT('Origin',(14.,138.155715454235,-12.864894733482));
#51668=CARTESIAN_POINT('',(14.,137.883945745091,-13.1170438759937));
#51669=CARTESIAN_POINT('',(14.,138.427485163379,-12.6127455909704));
#51670=CARTESIAN_POINT('Origin',(57.75,137.582939709175,-11.188418501646));
#51671=CARTESIAN_POINT('',(58.,137.536477638499,-11.4340631148344));
#51672=CARTESIAN_POINT('',(57.5,137.629401779851,-10.9427738884575));
#51673=CARTESIAN_POINT('Origin',(57.75,138.178436488856,-12.5909566552835));
#51674=CARTESIAN_POINT('',(58.,137.929387814333,-12.5691677195965));
#51675=CARTESIAN_POINT('',(57.5,138.427485163379,-12.6127455909704));
#51676=CARTESIAN_POINT('Origin',(57.75,135.425773646859,-12.8975129283142));
#51677=CARTESIAN_POINT('',(57.5,135.428874114848,-13.1474937017714));
#51678=CARTESIAN_POINT('',(58.,135.422673178871,-12.647532154857));
#51679=CARTESIAN_POINT('Origin',(14.,136.478673638569,-11.9403367564292));
#51680=CARTESIAN_POINT('Origin',(14.,134.364266202539,-13.1606978482623));
#51681=CARTESIAN_POINT('Origin',(14.,138.383907292005,-13.1108429400162));
#51682=CARTESIAN_POINT('Origin',(57.5,139.,-0.500000000000025));
#51683=CARTESIAN_POINT('',(57.5,138.502481404895,-1.04975185951052));
#51684=CARTESIAN_POINT('',(58.,138.5,-0.547506218943981));
#51685=CARTESIAN_POINT('',(57.5,138.502481404895,-1.04975185951052));
#51686=CARTESIAN_POINT('',(57.5,139.,-0.500000000000025));
#51687=CARTESIAN_POINT('',(57.5,139.,-0.500000000000025));
#51688=CARTESIAN_POINT('',(58.,138.5,-0.547506218943981));
#51689=CARTESIAN_POINT('Origin',(57.5,138.502481404895,1.04975185951047));
#51690=CARTESIAN_POINT('',(57.5,139.,0.499999999999975));
#51691=CARTESIAN_POINT('',(58.,138.5,0.547506218943931));
#51692=CARTESIAN_POINT('',(57.5,139.,0.499999999999975));
#51693=CARTESIAN_POINT('',(57.5,138.502481404895,1.04975185951047));
#51694=CARTESIAN_POINT('',(57.5,138.502481404895,1.04975185951047));
#51695=CARTESIAN_POINT('',(58.,138.5,0.547506218943931));
#51696=CARTESIAN_POINT('Origin',(14.,138.5,-0.547506218943981));
#51697=CARTESIAN_POINT('',(14.5,138.502481404895,-1.04975185951052));
#51698=CARTESIAN_POINT('',(14.5,139.,-0.500000000000025));
#51699=CARTESIAN_POINT('',(14.5,138.502481404895,-1.04975185951052));
#51700=CARTESIAN_POINT('',(14.,138.5,-0.547506218943981));
#51701=CARTESIAN_POINT('',(14.,138.5,-0.547506218943981));
#51702=CARTESIAN_POINT('',(14.5,139.,-0.500000000000025));
#51703=CARTESIAN_POINT('Origin',(14.25,136.034530010839,-1.04530010838812));
#51704=CARTESIAN_POINT('',(14.,136.009654081084,-0.796540810835624));
#51705=CARTESIAN_POINT('',(14.5,136.059405940594,-1.29405940594062));
#51706=CARTESIAN_POINT('Origin',(14.5,138.502481404895,1.04975185951047));
#51707=CARTESIAN_POINT('',(14.,138.5,0.54750621894393));
#51708=CARTESIAN_POINT('',(14.5,139.,0.499999999999975));
#51709=CARTESIAN_POINT('',(14.,138.5,0.54750621894393));
#51710=CARTESIAN_POINT('',(14.5,138.502481404895,1.04975185951047));
#51711=CARTESIAN_POINT('',(14.5,138.502481404895,1.04975185951047));
#51712=CARTESIAN_POINT('',(14.5,139.,0.499999999999975));
#51713=CARTESIAN_POINT('Origin',(14.25,138.034530010839,0.845300108388072));
#51714=CARTESIAN_POINT('',(14.5,138.059405940594,1.09405940594057));
#51715=CARTESIAN_POINT('',(14.,138.009654081084,0.596540810835574));
#51716=CARTESIAN_POINT('Origin',(14.,138.751240702448,0.774875929755224));
#51717=CARTESIAN_POINT('',(14.,139.,0.499999999999975));
#51718=CARTESIAN_POINT('',(14.,138.502481404895,1.04975185951047));
#51719=CARTESIAN_POINT('Origin',(14.25,138.75,-0.500000000000025));
#51720=CARTESIAN_POINT('',(14.5,139.,-0.500000000000026));
#51721=CARTESIAN_POINT('',(14.,138.5,-0.500000000000025));
#51722=CARTESIAN_POINT('Origin',(14.,138.751240702448,-0.774875929755274));
#51723=CARTESIAN_POINT('',(14.,138.502481404895,-1.04975185951052));
#51724=CARTESIAN_POINT('',(14.,139.,-0.500000000000025));
#51725=CARTESIAN_POINT('Origin',(57.75,138.034530010839,0.845300108388072));
#51726=CARTESIAN_POINT('',(58.,138.009654081084,0.596540810835575));
#51727=CARTESIAN_POINT('',(57.5,138.059405940594,1.09405940594057));
#51728=CARTESIAN_POINT('Origin',(57.75,138.75,-0.500000000000025));
#51729=CARTESIAN_POINT('',(58.,138.5,-0.500000000000025));
#51730=CARTESIAN_POINT('',(57.5,139.,-0.500000000000026));
#51731=CARTESIAN_POINT('Origin',(57.75,136.034530010839,-1.04530010838812));
#51732=CARTESIAN_POINT('',(57.5,136.059405940594,-1.29405940594062));
#51733=CARTESIAN_POINT('',(58.,136.009654081084,-0.796540810835624));
#51734=CARTESIAN_POINT('Origin',(14.,137.,-2.51664917224781E-14));
#51735=CARTESIAN_POINT('Origin',(14.,135.,-1.40000000000002));
#51736=CARTESIAN_POINT('Origin',(14.,139.,-1.00000000000003));
#51737=CARTESIAN_POINT('Origin',(57.75,135.607981461541,10.8148680765323));
#51738=CARTESIAN_POINT('',(57.7487592975525,138.290785228625,11.3210401476798));
#51739=CARTESIAN_POINT('',(58.,138.020683996878,11.5256475780664));
#51740=CARTESIAN_POINT('',(58.2319907935076,137.771277756289,11.7145781122933));
#51741=CARTESIAN_POINT('',(58.,135.561519390865,11.0605126897207));
#51742=CARTESIAN_POINT('',(57.5,138.066929551123,11.025529402481));
#51743=CARTESIAN_POINT('',(57.5,135.654443532217,10.5692234633438));
#51744=CARTESIAN_POINT('',(50.4896657310026,131.758409054648,2.69768347146864));
#51745=CARTESIAN_POINT('Origin',(58.,136.478673638569,11.9403367564291));
#51746=CARTESIAN_POINT('',(58.,137.925247374536,12.6164931630348));
#51747=CARTESIAN_POINT('',(58.,138.016543557081,11.5729730215047));
#51748=CARTESIAN_POINT('',(58.,137.432493723604,12.6226047007339));
#51749=CARTESIAN_POINT('Origin',(57.75,138.265592231604,11.5947619571917));
#51750=CARTESIAN_POINT('',(57.5,138.514640906126,11.6165508928786));
#51751=CARTESIAN_POINT('',(57.5,138.514640906126,11.6165508928786));
#51752=CARTESIAN_POINT('',(57.5,138.427485163379,12.6127455909703));
#51753=CARTESIAN_POINT('',(57.5,138.514640906126,11.6165508928786));
#51754=CARTESIAN_POINT('',(57.5,138.427485163379,12.6127455909703));
#51755=CARTESIAN_POINT('Origin',(14.,138.290785228625,11.3210401476798));
#51756=CARTESIAN_POINT('',(14.5,138.066929551123,11.025529402481));
#51757=CARTESIAN_POINT('',(14.,138.066929551123,11.025529402481));
#51758=CARTESIAN_POINT('',(14.5,138.514640906126,11.6165508928786));
#51759=CARTESIAN_POINT('',(14.5,138.066929551123,11.025529402481));
#51760=CARTESIAN_POINT('',(14.,138.514640906126,11.6165508928786));
#51761=CARTESIAN_POINT('Origin',(57.5,137.883945745091,13.1170438759936));
#51762=CARTESIAN_POINT('',(57.5,137.883945745091,13.1170438759936));
#51763=CARTESIAN_POINT('',(57.5,137.883945745091,13.1170438759936));
#51764=CARTESIAN_POINT('',(58.,137.925247374536,12.6164931630348));
#51765=CARTESIAN_POINT('Origin',(14.,138.020683996878,11.5256475780664));
#51766=CARTESIAN_POINT('',(14.,138.020683996878,11.5256475780664));
#51767=CARTESIAN_POINT('',(14.,138.020683996878,11.5256475780664));
#51768=CARTESIAN_POINT('',(14.5,138.514640906126,11.6165508928786));
#51769=CARTESIAN_POINT('Origin',(14.25,135.607981461541,10.8148680765323));
#51770=CARTESIAN_POINT('',(14.,135.561519390865,11.0605126897207));
#51771=CARTESIAN_POINT('',(14.5,135.654443532217,10.5692234633438));
#51772=CARTESIAN_POINT('Origin',(14.5,137.883945745091,13.1170438759936));
#51773=CARTESIAN_POINT('',(14.,137.925247374536,12.6164931630348));
#51774=CARTESIAN_POINT('',(14.5,138.427485163379,12.6127455909703));
#51775=CARTESIAN_POINT('',(14.,137.925247374536,12.6164931630348));
#51776=CARTESIAN_POINT('',(14.5,137.883945745091,13.1170438759936));
#51777=CARTESIAN_POINT('',(14.5,137.883945745091,13.1170438759936));
#51778=CARTESIAN_POINT('',(14.5,138.427485163379,12.6127455909703));
#51779=CARTESIAN_POINT('Origin',(14.25,137.435594191592,12.8725854741911));
#51780=CARTESIAN_POINT('',(14.5,137.438694659581,13.1225662476483));
#51781=CARTESIAN_POINT('',(14.,137.432493723604,12.6226047007339));
#51782=CARTESIAN_POINT('Origin',(14.,138.155715454235,12.864894733482));
#51783=CARTESIAN_POINT('',(14.,138.427485163379,12.6127455909703));
#51784=CARTESIAN_POINT('',(14.,137.883945745091,13.1170438759936));
#51785=CARTESIAN_POINT('Origin',(14.25,138.265592231604,11.5947619571917));
#51786=CARTESIAN_POINT('',(14.5,138.514640906126,11.6165508928786));
#51787=CARTESIAN_POINT('',(14.,138.016543557081,11.5729730215047));
#51788=CARTESIAN_POINT('Origin',(57.75,137.435594191592,12.8725854741911));
#51789=CARTESIAN_POINT('',(57.5,137.438694659581,13.1225662476483));
#51790=CARTESIAN_POINT('Origin',(14.,134.608302282232,10.3713526936054));
#51791=CARTESIAN_POINT('Origin',(14.,138.5582187775,11.1184535438327));
#51792=CARTESIAN_POINT('Origin',(57.5,136.97510175753,23.6446928191972));
#51793=CARTESIAN_POINT('',(57.5,136.580604996376,23.016899728323));
#51794=CARTESIAN_POINT('',(58.,136.490947249372,23.5110842376314));
#51795=CARTESIAN_POINT('',(57.5,136.580604996376,23.0168997283229));
#51796=CARTESIAN_POINT('',(57.5,136.97510175753,23.6446928191972));
#51797=CARTESIAN_POINT('',(57.5,136.97510175753,23.6446928191972));
#51798=CARTESIAN_POINT('',(58.,136.490947249372,23.5110842376314));
#51799=CARTESIAN_POINT('Origin',(57.5,136.216030001563,25.0845072682928));
#51800=CARTESIAN_POINT('',(57.5,136.801453579863,24.6295005722094));
#51801=CARTESIAN_POINT('',(58.,136.30080033501,24.5894609761082));
#51802=CARTESIAN_POINT('',(57.5,136.801453579863,24.6295005722094));
#51803=CARTESIAN_POINT('',(57.5,136.216030001563,25.0845072682928));
#51804=CARTESIAN_POINT('',(57.5,136.216030001563,25.0845072682928));
#51805=CARTESIAN_POINT('',(58.,136.30080033501,24.5894609761082));
#51806=CARTESIAN_POINT('Origin',(14.,136.490947249372,23.5110842376314));
#51807=CARTESIAN_POINT('',(14.5,136.580604996376,23.0168997283229));
#51808=CARTESIAN_POINT('',(14.5,136.97510175753,23.6446928191972));
#51809=CARTESIAN_POINT('',(14.5,136.580604996376,23.016899728323));
#51810=CARTESIAN_POINT('',(14.,136.490947249372,23.5110842376314));
#51811=CARTESIAN_POINT('',(14.,136.490947249372,23.5110842376314));
#51812=CARTESIAN_POINT('',(14.5,136.97510175753,23.6446928191972));
#51813=CARTESIAN_POINT('Origin',(14.25,134.149374290983,22.5927285851944));
#51814=CARTESIAN_POINT('',(14.,134.081679683799,22.8333890101882));
#51815=CARTESIAN_POINT('',(14.5,134.217068898167,22.3520681602006));
#51816=CARTESIAN_POINT('Origin',(14.5,136.216030001563,25.0845072682928));
#51817=CARTESIAN_POINT('',(14.,136.30080033501,24.5894609761082));
#51818=CARTESIAN_POINT('',(14.5,136.801453579863,24.6295005722094));
#51819=CARTESIAN_POINT('',(14.,136.30080033501,24.5894609761082));
#51820=CARTESIAN_POINT('',(14.5,136.216030001563,25.0845072682928));
#51821=CARTESIAN_POINT('',(14.5,136.216030001563,25.0845072682928));
#51822=CARTESIAN_POINT('',(14.5,136.801453579863,24.6295005722094));
#51823=CARTESIAN_POINT('Origin',(14.25,135.790690514667,24.801902691856));
#51824=CARTESIAN_POINT('',(14.5,135.771991924456,25.0512024365893));
#51825=CARTESIAN_POINT('',(14.,135.809389104878,24.5526029471226));
#51826=CARTESIAN_POINT('Origin',(14.,136.508741790713,24.8570039202511));
#51827=CARTESIAN_POINT('',(14.,136.801453579863,24.6295005722094));
#51828=CARTESIAN_POINT('',(14.,136.216030001563,25.0845072682928));
#51829=CARTESIAN_POINT('Origin',(14.25,136.728899819277,23.6012807747804));
#51830=CARTESIAN_POINT('',(14.5,136.97510175753,23.6446928191972));
#51831=CARTESIAN_POINT('',(14.,136.482697881024,23.5578687303637));
#51832=CARTESIAN_POINT('Origin',(14.,136.777853376953,23.3307962737601));
#51833=CARTESIAN_POINT('',(14.,136.580604996376,23.016899728323));
#51834=CARTESIAN_POINT('',(14.,136.97510175753,23.6446928191972));
#51835=CARTESIAN_POINT('Origin',(57.75,135.790690514667,24.801902691856));
#51836=CARTESIAN_POINT('',(58.,135.809389104878,24.5526029471226));
#51837=CARTESIAN_POINT('',(57.5,135.771991924456,25.0512024365893));
#51838=CARTESIAN_POINT('Origin',(57.75,136.728899819277,23.6012807747804));
#51839=CARTESIAN_POINT('',(58.,136.482697881024,23.5578687303637));
#51840=CARTESIAN_POINT('',(57.5,136.97510175753,23.6446928191972));
#51841=CARTESIAN_POINT('Origin',(57.75,134.149374290983,22.5927285851944));
#51842=CARTESIAN_POINT('',(57.5,134.217068898167,22.3520681602006));
#51843=CARTESIAN_POINT('',(58.,134.081679683799,22.8333890101882));
#51844=CARTESIAN_POINT('Origin',(14.,134.918662162673,23.7898003403694));
#51845=CARTESIAN_POINT('Origin',(14.,133.192154105382,22.0637731308185));
#51846=CARTESIAN_POINT('Origin',(14.,137.061925846364,23.1522889426911));
#51847=CARTESIAN_POINT('Origin',(57.5,133.511428020236,36.8610624138407));
#51848=CARTESIAN_POINT('',(57.5,134.134280331629,36.4588101823948));
#51849=CARTESIAN_POINT('',(58.,133.639021904261,36.3752881436309));
#51850=CARTESIAN_POINT('',(57.5,134.134280331629,36.4588101823948));
#51851=CARTESIAN_POINT('',(57.5,133.511428020236,36.8610624138407));
#51852=CARTESIAN_POINT('',(57.5,133.511428020236,36.8610624138407));
#51853=CARTESIAN_POINT('',(58.,133.639021904261,36.3752881436309));
#51854=CARTESIAN_POINT('Origin',(14.,133.822854175933,36.6599362981178));
#51855=CARTESIAN_POINT('',(14.2512407024475,133.822854175933,36.6599362981178));
#51856=CARTESIAN_POINT('',(14.5,133.511428020236,36.8610624138407));
#51857=CARTESIAN_POINT('',(14.3353834448874,133.717514391388,36.7279671340291));
#51858=CARTESIAN_POINT('',(14.,133.511428020236,36.8610624138407));
#51859=CARTESIAN_POINT('',(14.5,134.134280331629,36.4588101823948));
#51860=CARTESIAN_POINT('',(14.,134.134280331629,36.4588101823948));
#51861=CARTESIAN_POINT('',(14.4305329766294,134.047313338842,36.5149754502615));
#51862=CARTESIAN_POINT('Origin',(57.75,133.112337690265,36.5424624542375));
#51863=CARTESIAN_POINT('',(58.,133.152693031114,36.2957410598167));
#51864=CARTESIAN_POINT('',(57.5,133.071982349415,36.7891838486583));
#51865=CARTESIAN_POINT('Origin',(57.5,134.393099376732,35.4928843561058));
#51866=CARTESIAN_POINT('',(57.5,134.054819567983,34.8330975492483));
#51867=CARTESIAN_POINT('',(58.,133.922431977811,35.3175873497672));
#51868=CARTESIAN_POINT('',(57.5,134.054819567983,34.8330975492483));
#51869=CARTESIAN_POINT('',(57.5,134.393099376732,35.4928843561058));
#51870=CARTESIAN_POINT('',(57.5,134.393099376732,35.4928843561058));
#51871=CARTESIAN_POINT('',(58.,133.922431977811,35.3175873497672));
#51872=CARTESIAN_POINT('Origin',(14.,134.223959472357,35.1629909526771));
#51873=CARTESIAN_POINT('',(14.2512407024475,134.223959472357,35.1629909526771));
#51874=CARTESIAN_POINT('',(14.5,134.393099376732,35.4928843561058));
#51875=CARTESIAN_POINT('',(14.2590041943422,134.22923813446,35.1732865468069));
#51876=CARTESIAN_POINT('',(14.,134.393099376732,35.4928843561058));
#51877=CARTESIAN_POINT('',(14.5,134.054819567983,34.8330975492483));
#51878=CARTESIAN_POINT('',(14.,134.054819567983,34.8330975492483));
#51879=CARTESIAN_POINT('',(14.6801520303733,133.932328077252,34.5941880209647));
#51880=CARTESIAN_POINT('Origin',(57.75,134.151617920159,35.4281795948302));
#51881=CARTESIAN_POINT('',(58.,133.910136463587,35.3634748335545));
#51882=CARTESIAN_POINT('',(57.5,134.393099376732,35.4928843561058));
#51883=CARTESIAN_POINT('Origin',(57.75,131.669809380463,34.1986447874606));
#51884=CARTESIAN_POINT('',(57.5,131.75822132732,33.9648001218104));
#51885=CARTESIAN_POINT('',(58.,131.581397433607,34.4324894531108));
#51886=CARTESIAN_POINT('Origin',(14.25,133.112337690265,36.5424624542375));
#51887=CARTESIAN_POINT('',(14.,133.639021904261,36.3752881436309));
#51888=CARTESIAN_POINT('',(14.5,134.004870809078,36.9417730955394));
#51889=CARTESIAN_POINT('',(14.,133.152693031114,36.2957410598167));
#51890=CARTESIAN_POINT('',(14.5,133.071982349415,36.7891838486583));
#51891=CARTESIAN_POINT('Origin',(14.,134.522508899283,35.0099214429613));
#51892=CARTESIAN_POINT('',(14.5,134.393099376732,35.4928843561058));
#51893=CARTESIAN_POINT('Origin',(14.25,134.151617920159,35.4281795948302));
#51894=CARTESIAN_POINT('',(14.,133.922431977811,35.3175873497672));
#51895=CARTESIAN_POINT('',(14.,133.922431977811,35.3175873497672));
#51896=CARTESIAN_POINT('',(14.,133.910136463587,35.3634748335545));
#51897=CARTESIAN_POINT('Origin',(14.25,131.669809380463,34.1986447874606));
#51898=CARTESIAN_POINT('',(14.5,131.75822132732,33.9648001218104));
#51899=CARTESIAN_POINT('',(14.,131.581397433607,34.4324894531108));
#51900=CARTESIAN_POINT('Origin',(14.,130.762333212168,33.5882749320355));
#51901=CARTESIAN_POINT('Origin',(14.,134.004870809078,36.9417730955394));
#51902=CARTESIAN_POINT('Origin',(57.5,130.788284360904,47.0709536118749));
#51903=CARTESIAN_POINT('',(57.5,130.508796018164,46.3841944650246));
#51904=CARTESIAN_POINT('',(58.,130.334686134323,46.855302296829));
#51905=CARTESIAN_POINT('',(57.5,130.508796018164,46.3841944650246));
#51906=CARTESIAN_POINT('',(57.5,130.788284360904,47.0709536118749));
#51907=CARTESIAN_POINT('',(57.5,130.788284360904,47.0709536118749));
#51908=CARTESIAN_POINT('',(58.,130.334686134323,46.855302296829));
#51909=CARTESIAN_POINT('Origin',(57.5,129.790723455271,48.3570826171012));
#51910=CARTESIAN_POINT('',(57.5,130.446264217578,48.0106462326609));
#51911=CARTESIAN_POINT('',(58.,129.960169823373,47.8842774043811));
#51912=CARTESIAN_POINT('',(57.5,130.446264217578,48.0106462326609));
#51913=CARTESIAN_POINT('',(57.5,129.790723455271,48.3570826171012));
#51914=CARTESIAN_POINT('',(57.5,129.790723455271,48.3570826171012));
#51915=CARTESIAN_POINT('',(58.,129.960169823373,47.8842774043811));
#51916=CARTESIAN_POINT('Origin',(14.,130.334686134323,46.855302296829));
#51917=CARTESIAN_POINT('',(14.5,130.508796018164,46.3841944650246));
#51918=CARTESIAN_POINT('',(14.5,130.788284360904,47.0709536118749));
#51919=CARTESIAN_POINT('',(14.5,130.508796018164,46.3841944650246));
#51920=CARTESIAN_POINT('',(14.,130.334686134323,46.855302296829));
#51921=CARTESIAN_POINT('',(14.,130.334686134323,46.855302296829));
#51922=CARTESIAN_POINT('',(14.5,130.788284360904,47.0709536118749));
#51923=CARTESIAN_POINT('Origin',(14.25,128.188157716154,45.544288653188));
#51924=CARTESIAN_POINT('',(14.,128.079701297925,45.7695378603897));
#51925=CARTESIAN_POINT('',(14.5,128.296614134382,45.3190394459863));
#51926=CARTESIAN_POINT('Origin',(14.5,129.790723455271,48.3570826171012));
#51927=CARTESIAN_POINT('',(14.,129.960169823373,47.8842774043811));
#51928=CARTESIAN_POINT('',(14.5,130.446264217578,48.0106462326609));
#51929=CARTESIAN_POINT('',(14.,129.960169823373,47.8842774043811));
#51930=CARTESIAN_POINT('',(14.5,129.790723455271,48.3570826171012));
#51931=CARTESIAN_POINT('',(14.5,129.790723455271,48.3570826171012));
#51932=CARTESIAN_POINT('',(14.5,130.446264217578,48.0106462326609));
#51933=CARTESIAN_POINT('Origin',(14.25,129.420919600612,48.0049120124002));
#51934=CARTESIAN_POINT('',(14.5,129.359214637636,48.2471773577224));
#51935=CARTESIAN_POINT('',(14.,129.482624563588,47.762646667078));
#51936=CARTESIAN_POINT('Origin',(14.,130.118493836425,48.183864424881));
#51937=CARTESIAN_POINT('',(14.,130.446264217578,48.0106462326609));
#51938=CARTESIAN_POINT('',(14.,129.790723455271,48.3570826171012));
#51939=CARTESIAN_POINT('Origin',(14.25,130.553361205708,46.9854485760435));
#51940=CARTESIAN_POINT('',(14.5,130.788284360904,47.0709536118749));
#51941=CARTESIAN_POINT('',(14.,130.318438050511,46.8999435402121));
#51942=CARTESIAN_POINT('Origin',(14.,130.648540189534,46.7275740384498));
#51943=CARTESIAN_POINT('',(14.,130.508796018164,46.3841944650246));
#51944=CARTESIAN_POINT('',(14.,130.788284360904,47.0709536118749));
#51945=CARTESIAN_POINT('Origin',(57.75,129.420919600612,48.0049120124002));
#51946=CARTESIAN_POINT('',(58.,129.482624563588,47.762646667078));
#51947=CARTESIAN_POINT('',(57.5,129.359214637636,48.2471773577224));
#51948=CARTESIAN_POINT('Origin',(57.75,130.553361205708,46.9854485760435));
#51949=CARTESIAN_POINT('',(58.,130.318438050511,46.8999435402121));
#51950=CARTESIAN_POINT('',(57.5,130.788284360904,47.0709536118749));
#51951=CARTESIAN_POINT('Origin',(57.75,128.188157716154,45.544288653188));
#51952=CARTESIAN_POINT('',(57.5,128.296614134382,45.3190394459863));
#51953=CARTESIAN_POINT('',(58.,128.079701297925,45.7695378603897));
#51954=CARTESIAN_POINT('Origin',(14.,128.737889047669,46.8567596356165));
#51955=CARTESIAN_POINT('Origin',(14.,127.337332006754,44.8571496798649));
#51956=CARTESIAN_POINT('Origin',(14.,130.959294432567,46.601107301482));
#51957=CARTESIAN_POINT('Origin',(57.5,126.188091528965,58.2907844884388));
#51958=CARTESIAN_POINT('',(57.5,125.969521727281,57.5822796533796));
#51959=CARTESIAN_POINT('',(58.,125.755014631118,58.0364201014069));
#51960=CARTESIAN_POINT('',(57.5,125.969521727281,57.5822796533796));
#51961=CARTESIAN_POINT('',(57.5,126.188091528965,58.2907844884388));
#51962=CARTESIAN_POINT('',(57.5,126.188091528965,58.2907844884388));
#51963=CARTESIAN_POINT('',(58.,125.755014631118,58.0364201014069));
#51964=CARTESIAN_POINT('Origin',(57.5,125.08223311503,59.4850762228408));
#51965=CARTESIAN_POINT('',(57.5,125.765473267224,59.1970922754755));
#51966=CARTESIAN_POINT('',(58.,125.292242378034,59.0288384007667));
#51967=CARTESIAN_POINT('',(57.5,125.765473267224,59.1970922754755));
#51968=CARTESIAN_POINT('',(57.5,125.08223311503,59.4850762228408));
#51969=CARTESIAN_POINT('',(57.5,125.08223311503,59.4850762228408));
#51970=CARTESIAN_POINT('',(58.,125.292242378034,59.0288384007667));
#51971=CARTESIAN_POINT('Origin',(14.,125.755014631118,58.0364201014069));
#51972=CARTESIAN_POINT('',(14.5,125.969521727281,57.5822796533796));
#51973=CARTESIAN_POINT('',(14.5,126.188091528965,58.2907844884388));
#51974=CARTESIAN_POINT('',(14.5,125.969521727281,57.5822796533796));
#51975=CARTESIAN_POINT('',(14.,125.755014631118,58.0364201014069));
#51976=CARTESIAN_POINT('',(14.,125.755014631118,58.0364201014069));
#51977=CARTESIAN_POINT('',(14.5,126.188091528965,58.2907844884388));
#51978=CARTESIAN_POINT('Origin',(14.25,123.730916769498,56.5433129818712));
#51979=CARTESIAN_POINT('',(14.,123.603241298728,56.7582524481485));
#51980=CARTESIAN_POINT('',(14.5,123.858592240269,56.328373515594));
#51981=CARTESIAN_POINT('Origin',(14.5,125.08223311503,59.4850762228408));
#51982=CARTESIAN_POINT('',(14.,125.292242378034,59.0288384007667));
#51983=CARTESIAN_POINT('',(14.5,125.765473267224,59.1970922754755));
#51984=CARTESIAN_POINT('',(14.,125.292242378034,59.0288384007667));
#51985=CARTESIAN_POINT('',(14.5,125.08223311503,59.4850762228408));
#51986=CARTESIAN_POINT('',(14.5,125.08223311503,59.4850762228408));
#51987=CARTESIAN_POINT('',(14.5,125.765473267224,59.1970922754755));
#51988=CARTESIAN_POINT('Origin',(14.25,124.744530166311,59.1020152039901));
#51989=CARTESIAN_POINT('',(14.5,124.661945193235,59.337980714652));
#51990=CARTESIAN_POINT('',(14.,124.827115139388,58.8660496933281));
#51991=CARTESIAN_POINT('Origin',(14.,125.423853191127,59.3410842491581));
#51992=CARTESIAN_POINT('',(14.,125.765473267224,59.1970922754755));
#51993=CARTESIAN_POINT('',(14.,125.08223311503,59.4850762228408));
#51994=CARTESIAN_POINT('Origin',(14.25,125.961514582206,58.1851299230036));
#51995=CARTESIAN_POINT('',(14.5,126.188091528965,58.2907844884388));
#51996=CARTESIAN_POINT('',(14.,125.734937635446,58.0794753575685));
#51997=CARTESIAN_POINT('Origin',(14.,126.078806628123,57.9365320709092));
#51998=CARTESIAN_POINT('',(14.,125.969521727281,57.5822796533796));
#51999=CARTESIAN_POINT('',(14.,126.188091528965,58.2907844884388));
#52000=CARTESIAN_POINT('Origin',(57.75,124.744530166311,59.1020152039901));
#52001=CARTESIAN_POINT('',(58.,124.827115139388,58.8660496933281));
#52002=CARTESIAN_POINT('',(57.5,124.661945193235,59.337980714652));
#52003=CARTESIAN_POINT('Origin',(57.75,125.961514582206,58.1851299230036));
#52004=CARTESIAN_POINT('',(58.,125.734937635446,58.0794753575685));
#52005=CARTESIAN_POINT('',(57.5,126.188091528965,58.2907844884388));
#52006=CARTESIAN_POINT('Origin',(57.75,123.730916769498,56.5433129818712));
#52007=CARTESIAN_POINT('',(57.5,123.858592240269,56.328373515594));
#52008=CARTESIAN_POINT('',(58.,123.603241298728,56.7582524481485));
#52009=CARTESIAN_POINT('Origin',(14.,124.164166824021,57.8987018584757));
#52010=CARTESIAN_POINT('Origin',(14.,122.943216816385,55.784634433143));
#52011=CARTESIAN_POINT('Origin',(14.,126.399400659835,57.8376305949205));
#52012=CARTESIAN_POINT('Origin',(57.75,118.332008835457,67.1120085569767));
#52013=CARTESIAN_POINT('',(57.7487592975525,120.549537219807,68.7045581112747));
#52014=CARTESIAN_POINT('',(58.,120.218271533617,68.7758457056646));
#52015=CARTESIAN_POINT('',(58.2319907935076,119.912387221671,68.8416712881784));
#52016=CARTESIAN_POINT('',(58.,118.18608599957,67.3150024632071));
#52017=CARTESIAN_POINT('',(57.5,120.471543313576,68.3421289244415));
#52018=CARTESIAN_POINT('',(57.5,118.477931671344,66.9090146507463));
#52019=CARTESIAN_POINT('',(50.4896657310029,118.273581834349,58.1284413415477));
#52020=CARTESIAN_POINT('Origin',(58.,118.645480318468,68.5));
#52021=CARTESIAN_POINT('',(58.,119.670765314673,69.7241542943354));
#52022=CARTESIAN_POINT('',(58.,120.194518424145,68.8169872981078));
#52023=CARTESIAN_POINT('',(58.,119.221595996303,69.5214465371196));
#52024=CARTESIAN_POINT('Origin',(57.75,120.411024775091,68.9419872981078));
#52025=CARTESIAN_POINT('',(57.5,120.627531126037,69.0669872981078));
#52026=CARTESIAN_POINT('',(57.5,120.627531126037,69.0669872981078));
#52027=CARTESIAN_POINT('',(57.5,120.127531126037,69.9330127018922));
#52028=CARTESIAN_POINT('',(57.5,120.627531126037,69.0669872981078));
#52029=CARTESIAN_POINT('',(57.5,120.127531126037,69.9330127018922));
#52030=CARTESIAN_POINT('Origin',(14.,120.549537219807,68.7045581112747));
#52031=CARTESIAN_POINT('',(14.5,120.471543313576,68.3421289244415));
#52032=CARTESIAN_POINT('',(14.,120.471543313576,68.3421289244415));
#52033=CARTESIAN_POINT('',(14.5,120.627531126037,69.0669872981078));
#52034=CARTESIAN_POINT('',(14.5,120.471543313576,68.3421289244415));
#52035=CARTESIAN_POINT('',(14.,120.627531126037,69.0669872981078));
#52036=CARTESIAN_POINT('Origin',(57.5,119.421791454066,70.1603524804536));
#52037=CARTESIAN_POINT('',(57.5,119.421791454066,70.1603524804536));
#52038=CARTESIAN_POINT('',(57.5,119.421791454066,70.1603524804536));
#52039=CARTESIAN_POINT('',(58.,119.670765314673,69.7241542943354));
#52040=CARTESIAN_POINT('Origin',(14.,120.218271533617,68.7758457056646));
#52041=CARTESIAN_POINT('',(14.,120.218271533617,68.7758457056646));
#52042=CARTESIAN_POINT('',(14.,120.218271533617,68.7758457056646));
#52043=CARTESIAN_POINT('',(14.5,120.627531126037,69.0669872981078));
#52044=CARTESIAN_POINT('Origin',(14.25,118.332008835457,67.1120085569767));
#52045=CARTESIAN_POINT('',(14.,118.18608599957,67.3150024632071));
#52046=CARTESIAN_POINT('',(14.5,118.477931671344,66.9090146507463));
#52047=CARTESIAN_POINT('Origin',(14.5,119.421791454066,70.1603524804536));
#52048=CARTESIAN_POINT('',(14.,119.670765314673,69.7241542943354));
#52049=CARTESIAN_POINT('',(14.5,120.127531126037,69.9330127018922));
#52050=CARTESIAN_POINT('',(14.,119.670765314673,69.7241542943354));
#52051=CARTESIAN_POINT('',(14.5,119.421791454066,70.1603524804536));
#52052=CARTESIAN_POINT('',(14.5,119.421791454066,70.1603524804536));
#52053=CARTESIAN_POINT('',(14.5,120.127531126037,69.9330127018922));
#52054=CARTESIAN_POINT('Origin',(14.25,119.118759534638,69.7493163731053));
#52055=CARTESIAN_POINT('',(14.5,119.015923072972,69.9771862090909));
#52056=CARTESIAN_POINT('',(14.,119.221595996303,69.5214465371196));
#52057=CARTESIAN_POINT('Origin',(14.,119.774661290051,70.0466825911729));
#52058=CARTESIAN_POINT('',(14.,120.127531126037,69.9330127018922));
#52059=CARTESIAN_POINT('',(14.,119.421791454066,70.1603524804536));
#52060=CARTESIAN_POINT('Origin',(14.25,120.411024775091,68.9419872981078));
#52061=CARTESIAN_POINT('',(14.5,120.627531126037,69.0669872981078));
#52062=CARTESIAN_POINT('',(14.,120.194518424145,68.8169872981078));
#52063=CARTESIAN_POINT('Origin',(57.75,119.118759534638,69.7493163731053));
#52064=CARTESIAN_POINT('',(57.5,119.015923072972,69.9771862090909));
#52065=CARTESIAN_POINT('Origin',(14.,117.613429510899,66.2875644347018));
#52066=CARTESIAN_POINT('Origin',(14.,120.877531126037,68.6339745962156));
#52067=CARTESIAN_POINT('Origin',(57.5,114.148922374345,79.3175486306509));
#52068=CARTESIAN_POINT('',(57.5,114.056703712549,78.5818533282825));
#52069=CARTESIAN_POINT('',(58.,113.766594799967,78.991845596111));
#52070=CARTESIAN_POINT('',(57.5,114.056703712549,78.5818533282825));
#52071=CARTESIAN_POINT('',(57.5,114.148922374345,79.3175486306509));
#52072=CARTESIAN_POINT('',(57.5,114.148922374345,79.3175486306509));
#52073=CARTESIAN_POINT('',(58.,113.766594799967,78.991845596111));
#52074=CARTESIAN_POINT('Origin',(57.5,112.852477851287,80.3016660917109));
#52075=CARTESIAN_POINT('',(57.5,113.575345937994,80.1367006749399));
#52076=CARTESIAN_POINT('',(58.,113.138521468083,79.8888272731288));
#52077=CARTESIAN_POINT('',(57.5,113.575345937994,80.1367006749399));
#52078=CARTESIAN_POINT('',(57.5,112.852477851287,80.3016660917109));
#52079=CARTESIAN_POINT('',(57.5,112.852477851287,80.3016660917109));
#52080=CARTESIAN_POINT('',(58.,113.138521468083,79.8888272731288));
#52081=CARTESIAN_POINT('Origin',(14.,113.766594799967,78.991845596111));
#52082=CARTESIAN_POINT('',(14.5,114.056703712549,78.5818533282825));
#52083=CARTESIAN_POINT('',(14.5,114.148922374345,79.3175486306509));
#52084=CARTESIAN_POINT('',(14.5,114.056703712549,78.5818533282825));
#52085=CARTESIAN_POINT('',(14.,113.766594799967,78.991845596111));
#52086=CARTESIAN_POINT('',(14.,113.766594799967,78.991845596111));
#52087=CARTESIAN_POINT('',(14.5,114.148922374345,79.3175486306509));
#52088=CARTESIAN_POINT('Origin',(14.25,112.032522863357,77.1699412236247));
#52089=CARTESIAN_POINT('',(14.,111.869463223246,77.3594446636108));
#52090=CARTESIAN_POINT('',(14.5,112.195582503469,76.9804377836387));
#52091=CARTESIAN_POINT('Origin',(14.5,112.852477851287,80.3016660917109));
#52092=CARTESIAN_POINT('',(14.,113.138521468083,79.8888272731288));
#52093=CARTESIAN_POINT('',(14.5,113.575345937994,80.1367006749399));
#52094=CARTESIAN_POINT('',(14.,113.138521468083,79.8888272731288));
#52095=CARTESIAN_POINT('',(14.5,112.852477851287,80.3016660917109));
#52096=CARTESIAN_POINT('',(14.5,112.852477851287,80.3016660917109));
#52097=CARTESIAN_POINT('',(14.5,113.575345937994,80.1367006749399));
#52098=CARTESIAN_POINT('Origin',(14.25,112.586423217032,79.8657831288323));
#52099=CARTESIAN_POINT('',(14.5,112.464117914346,80.0838230630982));
#52100=CARTESIAN_POINT('',(14.,112.708728519719,79.6477431945663));
#52101=CARTESIAN_POINT('Origin',(14.,113.213911894641,80.2191833833254));
#52102=CARTESIAN_POINT('',(14.,113.575345937994,80.1367006749399));
#52103=CARTESIAN_POINT('',(14.,112.852477851287,80.3016660917109));
#52104=CARTESIAN_POINT('Origin',(14.25,113.944134363273,79.1741545215632));
#52105=CARTESIAN_POINT('',(14.5,114.148922374345,79.3175486306509));
#52106=CARTESIAN_POINT('',(14.,113.739346352201,79.0307604124754));
#52107=CARTESIAN_POINT('Origin',(14.,114.102813043447,78.9497009794667));
#52108=CARTESIAN_POINT('',(14.,114.056703712549,78.5818533282825));
#52109=CARTESIAN_POINT('',(14.,114.148922374345,79.3175486306509));
#52110=CARTESIAN_POINT('Origin',(57.75,112.586423217032,79.8657831288323));
#52111=CARTESIAN_POINT('',(58.,112.708728519719,79.6477431945663));
#52112=CARTESIAN_POINT('',(57.5,112.464117914346,80.0838230630982));
#52113=CARTESIAN_POINT('Origin',(57.75,113.944134363273,79.1741545215632));
#52114=CARTESIAN_POINT('',(58.,113.739346352201,79.0307604124754));
#52115=CARTESIAN_POINT('',(57.5,114.148922374345,79.3175486306509));
#52116=CARTESIAN_POINT('Origin',(57.75,112.032522863357,77.1699412236247));
#52117=CARTESIAN_POINT('',(57.5,112.195582503469,76.9804377836387));
#52118=CARTESIAN_POINT('',(58.,111.869463223246,77.3594446636108));
#52119=CARTESIAN_POINT('Origin',(14.,112.223830067592,78.5799717800933));
#52120=CARTESIAN_POINT('Origin',(14.,111.388532989905,76.2860060453866));
#52121=CARTESIAN_POINT('Origin',(14.,114.435710592521,78.9079726085064));
#52122=CARTESIAN_POINT('Origin',(57.5,105.424288749871,89.8318355365386));
#52123=CARTESIAN_POINT('',(57.5,106.158783788695,89.7304999679884));
#52124=CARTESIAN_POINT('',(58.,105.745225158215,89.4454980381808));
#52125=CARTESIAN_POINT('',(57.5,106.158783788695,89.7304999679884));
#52126=CARTESIAN_POINT('',(57.5,105.424288749871,89.8318355365386));
#52127=CARTESIAN_POINT('',(57.5,105.424288749871,89.8318355365386));
#52128=CARTESIAN_POINT('',(58.,105.745225158215,89.4454980381808));
#52129=CARTESIAN_POINT('Origin',(14.,105.791536269283,89.7811677522635));
#52130=CARTESIAN_POINT('',(14.2512407024475,105.791536269283,89.7811677522635));
#52131=CARTESIAN_POINT('',(14.5,105.424288749871,89.8318355365386));
#52132=CARTESIAN_POINT('',(14.3353834448875,105.667314928647,89.7983061119719));
#52133=CARTESIAN_POINT('',(14.,105.424288749871,89.8318355365386));
#52134=CARTESIAN_POINT('',(14.5,106.158783788695,89.7304999679884));
#52135=CARTESIAN_POINT('',(14.,106.158783788695,89.7304999679884));
#52136=CARTESIAN_POINT('',(14.4305329766294,106.056228458041,89.7446491482965));
#52137=CARTESIAN_POINT('Origin',(57.75,105.197236237204,89.3744230506705));
#52138=CARTESIAN_POINT('',(58.,105.338079563709,89.1678724336801));
#52139=CARTESIAN_POINT('',(57.5,105.0563929107,89.5809736676609));
#52140=CARTESIAN_POINT('Origin',(57.5,106.801571398381,88.9644555248695));
#52141=CARTESIAN_POINT('',(57.5,106.773823726948,88.223522379275));
#52142=CARTESIAN_POINT('',(58.,106.449085585742,88.6066698449906));
#52143=CARTESIAN_POINT('',(57.5,106.773823726948,88.223522379275));
#52144=CARTESIAN_POINT('',(57.5,106.801571398381,88.9644555248695));
#52145=CARTESIAN_POINT('',(57.5,106.801571398381,88.9644555248695));
#52146=CARTESIAN_POINT('',(58.,106.449085585742,88.6066698449906));
#52147=CARTESIAN_POINT('Origin',(14.,106.787697562665,88.5939889520722));
#52148=CARTESIAN_POINT('',(14.2512407024475,106.787697562665,88.5939889520722));
#52149=CARTESIAN_POINT('',(14.5,106.801571398381,88.9644555248695));
#52150=CARTESIAN_POINT('',(14.2590041943422,106.788130549139,88.6055507882064));
#52151=CARTESIAN_POINT('',(14.,106.801571398381,88.9644555248695));
#52152=CARTESIAN_POINT('',(14.5,106.773823726948,88.223522379275));
#52153=CARTESIAN_POINT('',(14.,106.773823726948,88.223522379275));
#52154=CARTESIAN_POINT('',(14.6801520303733,106.76377626461,87.9552296725038));
#52155=CARTESIAN_POINT('Origin',(57.75,106.610060287601,88.8037586224478));
#52156=CARTESIAN_POINT('',(58.,106.418549176822,88.6430617200262));
#52157=CARTESIAN_POINT('',(57.5,106.801571398381,88.9644555248695));
#52158=CARTESIAN_POINT('Origin',(57.75,104.880401745181,86.6405640410765));
#52159=CARTESIAN_POINT('',(57.5,105.059357207198,86.4659933029383));
#52160=CARTESIAN_POINT('',(58.,104.701446283163,86.8151347792147));
#52161=CARTESIAN_POINT('Origin',(14.25,105.197236237204,89.3744230506705));
#52162=CARTESIAN_POINT('',(14.,105.745225158215,89.4454980381808));
#52163=CARTESIAN_POINT('',(14.5,105.837389983851,90.1135221895479));
#52164=CARTESIAN_POINT('',(14.,105.338079563709,89.1678724336801));
#52165=CARTESIAN_POINT('',(14.5,105.0563929107,89.5809736676609));
#52166=CARTESIAN_POINT('Origin',(14.,107.122965203225,88.58143330331));
#52167=CARTESIAN_POINT('',(14.5,106.801571398381,88.9644555248695));
#52168=CARTESIAN_POINT('Origin',(14.25,106.610060287601,88.8037586224478));
#52169=CARTESIAN_POINT('',(14.,106.449085585742,88.6066698449906));
#52170=CARTESIAN_POINT('',(14.,106.449085585742,88.6066698449906));
#52171=CARTESIAN_POINT('',(14.,106.418549176822,88.6430617200262));
#52172=CARTESIAN_POINT('Origin',(14.25,104.880401745181,86.6405640410765));
#52173=CARTESIAN_POINT('',(14.5,105.059357207198,86.4659933029383));
#52174=CARTESIAN_POINT('',(14.,104.701446283163,86.8151347792147));
#52175=CARTESIAN_POINT('Origin',(14.,104.315902474623,85.7038650873162));
#52176=CARTESIAN_POINT('Origin',(14.,105.837389983851,90.1135221895479));
#52177=CARTESIAN_POINT('Origin',(57.5,98.6413959755234,97.9342891943368));
#52178=CARTESIAN_POINT('',(57.5,98.6783304709881,97.1937571541419));
#52179=CARTESIAN_POINT('',(58.,98.3214345544939,97.5471438341797));
#52180=CARTESIAN_POINT('',(57.5,98.6783304709881,97.1937571541419));
#52181=CARTESIAN_POINT('',(57.5,98.6413959755234,97.9342891943368));
#52182=CARTESIAN_POINT('',(57.5,98.6413959755234,97.9342891943368));
#52183=CARTESIAN_POINT('',(58.,98.3214345544939,97.5471438341797));
#52184=CARTESIAN_POINT('Origin',(57.5,97.1937571541419,98.678330470988));
#52185=CARTESIAN_POINT('',(57.5,97.9342891943369,98.6413959755234));
#52186=CARTESIAN_POINT('',(58.,97.5471438341798,98.3214345544939));
#52187=CARTESIAN_POINT('',(57.5,97.9342891943369,98.6413959755234));
#52188=CARTESIAN_POINT('',(57.5,97.1937571541419,98.678330470988));
#52189=CARTESIAN_POINT('',(57.5,97.1937571541419,98.678330470988));
#52190=CARTESIAN_POINT('',(58.,97.5471438341798,98.3214345544939));
#52191=CARTESIAN_POINT('Origin',(14.,98.3214345544939,97.5471438341797));
#52192=CARTESIAN_POINT('',(14.5,98.6783304709881,97.1937571541419));
#52193=CARTESIAN_POINT('',(14.5,98.6413959755234,97.9342891943368));
#52194=CARTESIAN_POINT('',(14.5,98.6783304709881,97.1937571541419));
#52195=CARTESIAN_POINT('',(14.,98.3214345544939,97.5471438341797));
#52196=CARTESIAN_POINT('',(14.,98.3214345544939,97.5471438341797));
#52197=CARTESIAN_POINT('',(14.5,98.6413959755234,97.9342891943368));
#52198=CARTESIAN_POINT('Origin',(14.25,96.9300774412053,95.4517998511728));
#52199=CARTESIAN_POINT('',(14.,96.7365881164045,95.6101092987371));
#52200=CARTESIAN_POINT('',(14.5,97.1235667660061,95.2934904036084));
#52201=CARTESIAN_POINT('Origin',(14.5,97.1937571541419,98.678330470988));
#52202=CARTESIAN_POINT('',(14.,97.5471438341798,98.3214345544939));
#52203=CARTESIAN_POINT('',(14.5,97.9342891943369,98.6413959755234));
#52204=CARTESIAN_POINT('',(14.,97.5471438341798,98.3214345544939));
#52205=CARTESIAN_POINT('',(14.5,97.1937571541419,98.678330470988));
#52206=CARTESIAN_POINT('',(14.5,97.1937571541419,98.678330470988));
#52207=CARTESIAN_POINT('',(14.5,97.9342891943369,98.6413959755234));
#52208=CARTESIAN_POINT('Origin',(14.25,97.0074347697832,98.2028696473411));
#52209=CARTESIAN_POINT('',(14.5,96.8491253222189,98.3963589721419));
#52210=CARTESIAN_POINT('',(14.,97.1657442173475,98.0093803225402));
#52211=CARTESIAN_POINT('Origin',(14.,97.5640231742394,98.6598632232557));
#52212=CARTESIAN_POINT('',(14.,97.9342891943369,98.6413959755234));
#52213=CARTESIAN_POINT('',(14.,97.1937571541419,98.678330470988));
#52214=CARTESIAN_POINT('Origin',(14.25,98.4646192802268,97.7575124990402));
#52215=CARTESIAN_POINT('',(14.5,98.6413959755234,97.9342891943368));
#52216=CARTESIAN_POINT('',(14.,98.2878425849301,97.5807358037436));
#52217=CARTESIAN_POINT('Origin',(14.,98.6598632232557,97.5640231742393));
#52218=CARTESIAN_POINT('',(14.,98.6783304709881,97.1937571541419));
#52219=CARTESIAN_POINT('',(14.,98.6413959755234,97.9342891943368));
#52220=CARTESIAN_POINT('Origin',(57.75,97.0074347697832,98.2028696473411));
#52221=CARTESIAN_POINT('',(58.,97.1657442173475,98.0093803225402));
#52222=CARTESIAN_POINT('',(57.5,96.8491253222189,98.3963589721419));
#52223=CARTESIAN_POINT('Origin',(57.75,98.4646192802268,97.7575124990402));
#52224=CARTESIAN_POINT('',(58.,98.2878425849301,97.5807358037436));
#52225=CARTESIAN_POINT('',(57.5,98.6413959755234,97.9342891943368));
#52226=CARTESIAN_POINT('Origin',(57.75,96.9300774412053,95.4517998511728));
#52227=CARTESIAN_POINT('',(57.5,97.1235667660061,95.2934904036084));
#52228=CARTESIAN_POINT('',(58.,96.7365881164045,95.6101092987371));
#52229=CARTESIAN_POINT('Origin',(14.,96.873629022557,96.873629022557));
#52230=CARTESIAN_POINT('Origin',(14.,96.4493649538451,94.4694659665227));
#52231=CARTESIAN_POINT('Origin',(14.,98.9949493661167,97.5807358037436));
#52232=CARTESIAN_POINT('Origin',(57.5,89.7304999679885,106.158783788695));
#52233=CARTESIAN_POINT('',(57.5,89.8318355365387,105.424288749871));
#52234=CARTESIAN_POINT('',(58.,89.4454980381808,105.745225158215));
#52235=CARTESIAN_POINT('',(57.5,89.8318355365387,105.424288749871));
#52236=CARTESIAN_POINT('',(57.5,89.7304999679885,106.158783788695));
#52237=CARTESIAN_POINT('',(57.5,89.7304999679885,106.158783788695));
#52238=CARTESIAN_POINT('',(58.,89.4454980381808,105.745225158215));
#52239=CARTESIAN_POINT('Origin',(57.5,88.223522379275,106.773823726948));
#52240=CARTESIAN_POINT('',(57.5,88.9644555248695,106.801571398381));
#52241=CARTESIAN_POINT('',(58.,88.6066698449906,106.449085585742));
#52242=CARTESIAN_POINT('',(57.5,88.9644555248695,106.801571398381));
#52243=CARTESIAN_POINT('',(57.5,88.223522379275,106.773823726948));
#52244=CARTESIAN_POINT('',(57.5,88.223522379275,106.773823726948));
#52245=CARTESIAN_POINT('',(58.,88.6066698449906,106.449085585742));
#52246=CARTESIAN_POINT('Origin',(14.,89.4454980381808,105.745225158215));
#52247=CARTESIAN_POINT('',(14.5,89.8318355365387,105.424288749871));
#52248=CARTESIAN_POINT('',(14.5,89.7304999679885,106.158783788695));
#52249=CARTESIAN_POINT('',(14.5,89.8318355365387,105.424288749871));
#52250=CARTESIAN_POINT('',(14.,89.4454980381808,105.745225158215));
#52251=CARTESIAN_POINT('',(14.,89.4454980381808,105.745225158215));
#52252=CARTESIAN_POINT('',(14.5,89.7304999679885,106.158783788695));
#52253=CARTESIAN_POINT('Origin',(14.25,88.2420567199213,103.536589829029));
#52254=CARTESIAN_POINT('',(14.,88.0355061029309,103.677433155534));
#52255=CARTESIAN_POINT('',(14.5,88.4486073369117,103.395746502524));
#52256=CARTESIAN_POINT('Origin',(14.5,88.223522379275,106.773823726948));
#52257=CARTESIAN_POINT('',(14.,88.6066698449906,106.449085585742));
#52258=CARTESIAN_POINT('',(14.5,88.9644555248695,106.801571398381));
#52259=CARTESIAN_POINT('',(14.,88.6066698449906,106.449085585742));
#52260=CARTESIAN_POINT('',(14.5,88.223522379275,106.773823726948));
#52261=CARTESIAN_POINT('',(14.5,88.223522379275,106.773823726948));
#52262=CARTESIAN_POINT('',(14.5,88.9644555248695,106.801571398381));
#52263=CARTESIAN_POINT('Origin',(14.25,88.0793481490734,106.283933109481));
#52264=CARTESIAN_POINT('',(14.5,87.9047774109353,106.462888571499));
#52265=CARTESIAN_POINT('',(14.,88.2539188872116,106.104977647464));
#52266=CARTESIAN_POINT('Origin',(14.,88.5939889520723,106.787697562665));
#52267=CARTESIAN_POINT('',(14.,88.9644555248695,106.801571398381));
#52268=CARTESIAN_POINT('',(14.,88.223522379275,106.773823726948));
#52269=CARTESIAN_POINT('Origin',(14.25,89.5698030655669,105.967272677915));
#52270=CARTESIAN_POINT('',(14.5,89.7304999679885,106.158783788695));
#52271=CARTESIAN_POINT('',(14.,89.4091061631452,105.775761567135));
#52272=CARTESIAN_POINT('Origin',(14.,89.7811677522636,105.791536269283));
#52273=CARTESIAN_POINT('',(14.,89.8318355365387,105.424288749871));
#52274=CARTESIAN_POINT('',(14.,89.7304999679885,106.158783788695));
#52275=CARTESIAN_POINT('Origin',(57.75,88.0793481490734,106.283933109481));
#52276=CARTESIAN_POINT('',(58.,88.2539188872116,106.104977647464));
#52277=CARTESIAN_POINT('',(57.5,87.9047774109353,106.462888571499));
#52278=CARTESIAN_POINT('Origin',(57.75,89.5698030655669,105.967272677915));
#52279=CARTESIAN_POINT('',(58.,89.4091061631452,105.775761567135));
#52280=CARTESIAN_POINT('',(57.5,89.7304999679885,106.158783788695));
#52281=CARTESIAN_POINT('Origin',(57.75,88.2420567199213,103.536589829029));
#52282=CARTESIAN_POINT('',(57.5,88.4486073369117,103.395746502524));
#52283=CARTESIAN_POINT('',(58.,88.0355061029309,103.677433155534));
#52284=CARTESIAN_POINT('Origin',(14.,88.0619025270559,104.9480887073));
#52285=CARTESIAN_POINT('Origin',(14.,87.8487895280494,102.516097167501));
#52286=CARTESIAN_POINT('Origin',(14.,90.113522189548,105.837389983851));
#52287=CARTESIAN_POINT('Origin',(57.75,78.882460664988,110.833403841184));
#52288=CARTESIAN_POINT('',(57.7487592975525,80.2191833833255,113.213911894641));
#52289=CARTESIAN_POINT('',(58.,79.8888272731288,113.138521468083));
#52290=CARTESIAN_POINT('',(58.2319907935076,79.5837828460196,113.068907409893));
#52291=CARTESIAN_POINT('',(58.,78.6644207307221,110.955709143871));
#52292=CARTESIAN_POINT('',(57.5,80.301666091711,112.852477851287));
#52293=CARTESIAN_POINT('',(57.5,79.100500599254,110.711098538497));
#52294=CARTESIAN_POINT('',(50.4896657310026,82.6261273797262,102.666834600827));
#52295=CARTESIAN_POINT('Origin',(58.,78.5799717800934,112.223830067592));
#52296=CARTESIAN_POINT('',(58.,78.9918455961111,113.766594799967));
#52297=CARTESIAN_POINT('',(58.,79.8499124567644,113.16576991585));
#52298=CARTESIAN_POINT('',(58.,78.6704279451708,113.393052024553));
#52299=CARTESIAN_POINT('Origin',(57.75,79.9933065658522,113.370557926922));
#52300=CARTESIAN_POINT('',(57.5,80.13670067494,113.575345937994));
#52301=CARTESIAN_POINT('',(57.5,80.13670067494,113.575345937994));
#52302=CARTESIAN_POINT('',(57.5,79.317548630651,114.148922374345));
#52303=CARTESIAN_POINT('',(57.5,80.13670067494,113.575345937994));
#52304=CARTESIAN_POINT('',(57.5,79.317548630651,114.148922374345));
#52305=CARTESIAN_POINT('Origin',(14.,80.2191833833255,113.213911894641));
#52306=CARTESIAN_POINT('',(14.5,80.301666091711,112.852477851287));
#52307=CARTESIAN_POINT('',(14.,80.301666091711,112.852477851287));
#52308=CARTESIAN_POINT('',(14.5,80.13670067494,113.575345937994));
#52309=CARTESIAN_POINT('',(14.5,80.301666091711,112.852477851287));
#52310=CARTESIAN_POINT('',(14.,80.13670067494,113.575345937994));
#52311=CARTESIAN_POINT('Origin',(57.5,78.5818533282826,114.056703712549));
#52312=CARTESIAN_POINT('',(57.5,78.5818533282826,114.056703712549));
#52313=CARTESIAN_POINT('',(57.5,78.5818533282826,114.056703712549));
#52314=CARTESIAN_POINT('',(58.,78.9918455961111,113.766594799967));
#52315=CARTESIAN_POINT('Origin',(14.,79.8888272731288,113.138521468083));
#52316=CARTESIAN_POINT('',(14.,79.8888272731288,113.138521468083));
#52317=CARTESIAN_POINT('',(14.,79.8888272731288,113.138521468083));
#52318=CARTESIAN_POINT('',(14.5,80.13670067494,113.575345937994));
#52319=CARTESIAN_POINT('Origin',(14.25,78.882460664988,110.833403841184));
#52320=CARTESIAN_POINT('',(14.,78.6644207307221,110.955709143871));
#52321=CARTESIAN_POINT('',(14.5,79.100500599254,110.711098538497));
#52322=CARTESIAN_POINT('Origin',(14.5,78.5818533282826,114.056703712549));
#52323=CARTESIAN_POINT('',(14.,78.9918455961111,113.766594799967));
#52324=CARTESIAN_POINT('',(14.5,79.317548630651,114.148922374345));
#52325=CARTESIAN_POINT('',(14.,78.9918455961111,113.766594799967));
#52326=CARTESIAN_POINT('',(14.5,78.5818533282826,114.056703712549));
#52327=CARTESIAN_POINT('',(14.5,78.5818533282826,114.056703712549));
#52328=CARTESIAN_POINT('',(14.5,79.317548630651,114.148922374345));
#52329=CARTESIAN_POINT('Origin',(14.25,78.4809245051847,113.556111664665));
#52330=CARTESIAN_POINT('',(14.5,78.2914210651986,113.719171304777));
#52331=CARTESIAN_POINT('',(14.,78.6704279451708,113.393052024553));
#52332=CARTESIAN_POINT('Origin',(14.,78.9497009794668,114.102813043447));
#52333=CARTESIAN_POINT('',(14.,79.317548630651,114.148922374345));
#52334=CARTESIAN_POINT('',(14.,78.5818533282826,114.056703712549));
#52335=CARTESIAN_POINT('Origin',(14.25,79.9933065658522,113.370557926922));
#52336=CARTESIAN_POINT('',(14.5,80.13670067494,113.575345937994));
#52337=CARTESIAN_POINT('',(14.,79.8499124567644,113.16576991585));
#52338=CARTESIAN_POINT('Origin',(57.75,78.4809245051847,113.556111664665));
#52339=CARTESIAN_POINT('',(57.5,78.2914210651986,113.719171304777));
#52340=CARTESIAN_POINT('Origin',(14.,78.5796317693959,109.782518968122));
#52341=CARTESIAN_POINT('Origin',(14.,80.5462766970845,113.288557719819));
#52342=CARTESIAN_POINT('Origin',(57.5,69.9330127018923,120.127531126037));
#52343=CARTESIAN_POINT('',(57.5,70.1603524804536,119.421791454066));
#52344=CARTESIAN_POINT('',(58.,69.7241542943355,119.670765314673));
#52345=CARTESIAN_POINT('',(57.5,70.1603524804536,119.421791454066));
#52346=CARTESIAN_POINT('',(57.5,69.9330127018923,120.127531126037));
#52347=CARTESIAN_POINT('',(57.5,69.9330127018923,120.127531126037));
#52348=CARTESIAN_POINT('',(58.,69.7241542943355,119.670765314673));
#52349=CARTESIAN_POINT('Origin',(57.5,68.3421289244415,120.471543313576));
#52350=CARTESIAN_POINT('',(57.5,69.0669872981079,120.627531126037));
#52351=CARTESIAN_POINT('',(58.,68.7758457056646,120.218271533617));
#52352=CARTESIAN_POINT('',(57.5,69.0669872981079,120.627531126037));
#52353=CARTESIAN_POINT('',(57.5,68.3421289244415,120.471543313576));
#52354=CARTESIAN_POINT('',(57.5,68.3421289244415,120.471543313576));
#52355=CARTESIAN_POINT('',(58.,68.7758457056646,120.218271533617));
#52356=CARTESIAN_POINT('Origin',(14.,69.7241542943355,119.670765314673));
#52357=CARTESIAN_POINT('',(14.5,70.1603524804536,119.421791454066));
#52358=CARTESIAN_POINT('',(14.5,69.9330127018923,120.127531126037));
#52359=CARTESIAN_POINT('',(14.5,70.1603524804536,119.421791454066));
#52360=CARTESIAN_POINT('',(14.,69.7241542943355,119.670765314673));
#52361=CARTESIAN_POINT('',(14.,69.7241542943355,119.670765314673));
#52362=CARTESIAN_POINT('',(14.5,69.9330127018923,120.127531126037));
#52363=CARTESIAN_POINT('Origin',(14.25,68.9225214538622,117.286708727069));
#52364=CARTESIAN_POINT('',(14.,68.6946516178765,117.389545188734));
#52365=CARTESIAN_POINT('',(14.5,69.1503912898478,117.183872265403));
#52366=CARTESIAN_POINT('Origin',(14.5,68.3421289244415,120.471543313576));
#52367=CARTESIAN_POINT('',(14.,68.7758457056646,120.218271533617));
#52368=CARTESIAN_POINT('',(14.5,69.0669872981079,120.627531126037));
#52369=CARTESIAN_POINT('',(14.,68.7758457056646,120.218271533617));
#52370=CARTESIAN_POINT('',(14.5,68.3421289244415,120.471543313576));
#52371=CARTESIAN_POINT('',(14.5,68.3421289244415,120.471543313576));
#52372=CARTESIAN_POINT('',(14.5,69.0669872981079,120.627531126037));
#52373=CARTESIAN_POINT('Origin',(14.25,68.2852136377336,119.964059643026));
#52374=CARTESIAN_POINT('',(14.5,68.0822197315032,120.109982478913));
#52375=CARTESIAN_POINT('',(14.,68.488207543964,119.818136807139));
#52376=CARTESIAN_POINT('Origin',(14.,68.7045581112747,120.549537219807));
#52377=CARTESIAN_POINT('',(14.,69.0669872981079,120.627531126037));
#52378=CARTESIAN_POINT('',(14.,68.3421289244415,120.471543313576));
#52379=CARTESIAN_POINT('Origin',(14.25,69.8080127018923,119.911024775091));
#52380=CARTESIAN_POINT('',(14.5,69.9330127018923,120.127531126037));
#52381=CARTESIAN_POINT('',(14.,69.6830127018923,119.694518424145));
#52382=CARTESIAN_POINT('Origin',(14.,70.0466825911729,119.774661290051));
#52383=CARTESIAN_POINT('',(14.,70.1603524804536,119.421791454066));
#52384=CARTESIAN_POINT('',(14.,69.9330127018923,120.127531126037));
#52385=CARTESIAN_POINT('Origin',(57.75,68.2852136377336,119.964059643026));
#52386=CARTESIAN_POINT('',(58.,68.4882075439641,119.818136807139));
#52387=CARTESIAN_POINT('',(57.5,68.0822197315032,120.109982478913));
#52388=CARTESIAN_POINT('Origin',(57.75,69.8080127018923,119.911024775091));
#52389=CARTESIAN_POINT('',(58.,69.6830127018923,119.694518424145));
#52390=CARTESIAN_POINT('',(57.5,69.9330127018923,120.127531126037));
#52391=CARTESIAN_POINT('Origin',(57.75,68.9225214538622,117.286708727069));
#52392=CARTESIAN_POINT('',(57.5,69.1503912898478,117.183872265403));
#52393=CARTESIAN_POINT('',(58.,68.6946516178765,117.389545188734));
#52394=CARTESIAN_POINT('Origin',(14.,68.5000000000001,118.645480318468));
#52395=CARTESIAN_POINT('Origin',(14.,68.7124355652983,116.213429510899));
#52396=CARTESIAN_POINT('Origin',(14.,70.3660254037845,119.877531126037));
#52397=CARTESIAN_POINT('Origin',(57.5,57.5822796533798,125.969521727281));
#52398=CARTESIAN_POINT('',(57.5,58.290784488439,126.188091528965));
#52399=CARTESIAN_POINT('',(58.,58.0364201014071,125.755014631118));
#52400=CARTESIAN_POINT('',(57.5,58.290784488439,126.188091528965));
#52401=CARTESIAN_POINT('',(57.5,57.5822796533798,125.969521727281));
#52402=CARTESIAN_POINT('',(57.5,57.5822796533798,125.969521727281));
#52403=CARTESIAN_POINT('',(58.,58.0364201014071,125.755014631118));
#52404=CARTESIAN_POINT('Origin',(14.,57.9365320709094,126.078806628123));
#52405=CARTESIAN_POINT('',(14.2512407024475,57.9365320709094,126.078806628123));
#52406=CARTESIAN_POINT('',(14.5,57.5822796533798,125.969521727281));
#52407=CARTESIAN_POINT('',(14.3353834448874,57.816706318786,126.041841049933));
#52408=CARTESIAN_POINT('',(14.,57.5822796533798,125.969521727281));
#52409=CARTESIAN_POINT('',(14.5,58.290784488439,126.188091528965));
#52410=CARTESIAN_POINT('',(14.,58.290784488439,126.188091528965));
#52411=CARTESIAN_POINT('',(14.4305329766294,58.1918580916782,126.157573285685));
#52412=CARTESIAN_POINT('Origin',(57.75,57.5698110627601,125.459008691224));
#52413=CARTESIAN_POINT('',(58.,57.7847505290374,125.331333220453));
#52414=CARTESIAN_POINT('',(57.5,57.3548715964829,125.586684161994));
#52415=CARTESIAN_POINT('Origin',(57.5,59.1970922754756,125.765473267224));
#52416=CARTESIAN_POINT('',(57.5,59.4850762228409,125.08223311503));
#52417=CARTESIAN_POINT('',(58.,59.0288384007668,125.292242378034));
#52418=CARTESIAN_POINT('',(57.5,59.4850762228409,125.08223311503));
#52419=CARTESIAN_POINT('',(57.5,59.1970922754756,125.765473267224));
#52420=CARTESIAN_POINT('',(57.5,59.1970922754756,125.765473267224));
#52421=CARTESIAN_POINT('',(58.,59.0288384007668,125.292242378034));
#52422=CARTESIAN_POINT('Origin',(14.,59.3410842491583,125.423853191127));
#52423=CARTESIAN_POINT('',(14.2512407024475,59.3410842491583,125.423853191127));
#52424=CARTESIAN_POINT('',(14.5,59.1970922754756,125.765473267224));
#52425=CARTESIAN_POINT('',(14.2590041943422,59.3365904250818,125.434514761239));
#52426=CARTESIAN_POINT('',(14.,59.1970922754756,125.765473267224));
#52427=CARTESIAN_POINT('',(14.5,59.4850762228409,125.08223311503));
#52428=CARTESIAN_POINT('',(14.,59.4850762228409,125.08223311503));
#52429=CARTESIAN_POINT('',(14.6801520303733,59.5893555268573,124.83483110461));
#52430=CARTESIAN_POINT('Origin',(57.75,59.0914377100405,125.538896320465));
#52431=CARTESIAN_POINT('',(58.,58.9857831446053,125.312319373706));
#52432=CARTESIAN_POINT('',(57.5,59.1970922754756,125.765473267224));
#52433=CARTESIAN_POINT('Origin',(57.75,58.4380402379162,122.84739093989));
#52434=CARTESIAN_POINT('',(57.5,58.6740057485781,122.764805966813));
#52435=CARTESIAN_POINT('',(58.,58.2020747272542,122.929975912966));
#52436=CARTESIAN_POINT('Origin',(14.25,57.5698110627601,125.459008691224));
#52437=CARTESIAN_POINT('',(14.,58.0364201014071,125.755014631118));
#52438=CARTESIAN_POINT('',(14.5,57.8376305949207,126.399400659835));
#52439=CARTESIAN_POINT('',(14.,57.7847505290374,125.331333220453));
#52440=CARTESIAN_POINT('',(14.5,57.3548715964829,125.586684161994));
#52441=CARTESIAN_POINT('Origin',(14.,59.650246168994,125.554164136354));
#52442=CARTESIAN_POINT('',(14.5,59.1970922754756,125.765473267224));
#52443=CARTESIAN_POINT('Origin',(14.25,59.0914377100405,125.538896320465));
#52444=CARTESIAN_POINT('',(14.,59.0288384007668,125.292242378034));
#52445=CARTESIAN_POINT('',(14.,59.0288384007668,125.292242378034));
#52446=CARTESIAN_POINT('',(14.,58.9857831446053,125.312319373706));
#52447=CARTESIAN_POINT('Origin',(14.25,58.4380402379162,122.84739093989));
#52448=CARTESIAN_POINT('',(14.5,58.6740057485781,122.764805966813));
#52449=CARTESIAN_POINT('',(14.,58.2020747272542,122.929975912966));
#52450=CARTESIAN_POINT('Origin',(14.,58.3222962368458,121.759885683511));
#52451=CARTESIAN_POINT('Origin',(14.,57.8376305949207,126.399400659835));
#52452=CARTESIAN_POINT('Origin',(57.5,48.010646232661,130.446264217578));
#52453=CARTESIAN_POINT('',(57.5,48.3570826171014,129.790723455271));
#52454=CARTESIAN_POINT('',(58.,47.8842774043812,129.960169823373));
#52455=CARTESIAN_POINT('',(57.5,48.3570826171014,129.790723455271));
#52456=CARTESIAN_POINT('',(57.5,48.010646232661,130.446264217578));
#52457=CARTESIAN_POINT('',(57.5,48.010646232661,130.446264217578));
#52458=CARTESIAN_POINT('',(58.,47.8842774043812,129.960169823373));
#52459=CARTESIAN_POINT('Origin',(57.5,46.3841944650248,130.508796018163));
#52460=CARTESIAN_POINT('',(57.5,47.0709536118751,130.788284360904));
#52461=CARTESIAN_POINT('',(58.,46.8553022968292,130.334686134323));
#52462=CARTESIAN_POINT('',(57.5,47.0709536118751,130.788284360904));
#52463=CARTESIAN_POINT('',(57.5,46.3841944650248,130.508796018163));
#52464=CARTESIAN_POINT('',(57.5,46.3841944650248,130.508796018163));
#52465=CARTESIAN_POINT('',(58.,46.8553022968292,130.334686134323));
#52466=CARTESIAN_POINT('Origin',(14.,47.8842774043813,129.960169823373));
#52467=CARTESIAN_POINT('',(14.5,48.3570826171014,129.790723455271));
#52468=CARTESIAN_POINT('',(14.5,48.010646232661,130.446264217578));
#52469=CARTESIAN_POINT('',(14.5,48.3570826171014,129.790723455271));
#52470=CARTESIAN_POINT('',(14.,47.8842774043813,129.960169823373));
#52471=CARTESIAN_POINT('',(14.,47.8842774043813,129.960169823373));
#52472=CARTESIAN_POINT('',(14.5,48.010646232661,130.446264217578));
#52473=CARTESIAN_POINT('Origin',(14.25,47.5088102499062,127.473130330375));
#52474=CARTESIAN_POINT('',(14.,47.266544904584,127.534835293351));
#52475=CARTESIAN_POINT('',(14.5,47.7510755952284,127.411425367399));
#52476=CARTESIAN_POINT('Origin',(14.5,46.3841944650248,130.508796018163));
#52477=CARTESIAN_POINT('',(14.,46.8553022968292,130.334686134323));
#52478=CARTESIAN_POINT('',(14.5,47.0709536118751,130.788284360904));
#52479=CARTESIAN_POINT('',(14.,46.8553022968292,130.334686134323));
#52480=CARTESIAN_POINT('',(14.5,46.3841944650248,130.508796018163));
#52481=CARTESIAN_POINT('',(14.5,46.3841944650248,130.508796018163));
#52482=CARTESIAN_POINT('',(14.5,47.0709536118751,130.788284360904));
#52483=CARTESIAN_POINT('Origin',(14.25,46.4162674639967,129.99913892906));
#52484=CARTESIAN_POINT('',(14.5,46.191018256795,130.107595347289));
#52485=CARTESIAN_POINT('',(14.,46.6415166711984,129.890682510832));
#52486=CARTESIAN_POINT('Origin',(14.,46.7275740384499,130.648540189534));
#52487=CARTESIAN_POINT('',(14.,47.0709536118751,130.788284360904));
#52488=CARTESIAN_POINT('',(14.,46.3841944650248,130.508796018163));
#52489=CARTESIAN_POINT('Origin',(14.25,47.9251411968296,130.211341062382));
#52490=CARTESIAN_POINT('',(14.5,48.010646232661,130.446264217578));
#52491=CARTESIAN_POINT('',(14.,47.8396361609982,129.976417907185));
#52492=CARTESIAN_POINT('Origin',(14.,48.1838644248812,130.118493836425));
#52493=CARTESIAN_POINT('',(14.,48.3570826171014,129.790723455271));
#52494=CARTESIAN_POINT('',(14.,48.010646232661,130.446264217578));
#52495=CARTESIAN_POINT('Origin',(57.75,46.4162674639967,129.99913892906));
#52496=CARTESIAN_POINT('',(58.,46.6415166711984,129.890682510832));
#52497=CARTESIAN_POINT('',(57.5,46.191018256795,130.107595347289));
#52498=CARTESIAN_POINT('Origin',(57.75,47.9251411968296,130.211341062382));
#52499=CARTESIAN_POINT('',(58.,47.8396361609982,129.976417907185));
#52500=CARTESIAN_POINT('',(57.5,48.010646232661,130.446264217578));
#52501=CARTESIAN_POINT('Origin',(57.75,47.5088102499062,127.473130330375));
#52502=CARTESIAN_POINT('',(57.5,47.7510755952284,127.411425367399));
#52503=CARTESIAN_POINT('',(58.,47.266544904584,127.534835293351));
#52504=CARTESIAN_POINT('Origin',(14.,46.8567596356167,128.737889047669));
#52505=CARTESIAN_POINT('Origin',(14.,47.4882890180657,126.379675605442));
#52506=CARTESIAN_POINT('Origin',(14.,48.480492543054,130.275254145916));
#52507=CARTESIAN_POINT('Origin',(57.5,36.4588101823949,134.134280331629));
#52508=CARTESIAN_POINT('',(57.5,36.8610624138407,133.511428020236));
#52509=CARTESIAN_POINT('',(58.,36.375288143631,133.639021904261));
#52510=CARTESIAN_POINT('',(57.5,36.8610624138407,133.511428020236));
#52511=CARTESIAN_POINT('',(57.5,36.4588101823949,134.134280331629));
#52512=CARTESIAN_POINT('',(57.5,36.4588101823949,134.134280331629));
#52513=CARTESIAN_POINT('',(58.,36.375288143631,133.639021904261));
#52514=CARTESIAN_POINT('Origin',(57.5,34.8330975492484,134.054819567983));
#52515=CARTESIAN_POINT('',(57.5,35.4928843561058,134.393099376732));
#52516=CARTESIAN_POINT('',(58.,35.3175873497673,133.922431977811));
#52517=CARTESIAN_POINT('',(57.5,35.4928843561058,134.393099376732));
#52518=CARTESIAN_POINT('',(57.5,34.8330975492484,134.054819567983));
#52519=CARTESIAN_POINT('',(57.5,34.8330975492484,134.054819567983));
#52520=CARTESIAN_POINT('',(58.,35.3175873497673,133.922431977811));
#52521=CARTESIAN_POINT('Origin',(14.,36.375288143631,133.639021904261));
#52522=CARTESIAN_POINT('',(14.5,36.8610624138407,133.511428020236));
#52523=CARTESIAN_POINT('',(14.5,36.4588101823949,134.134280331629));
#52524=CARTESIAN_POINT('',(14.5,36.8610624138407,133.511428020236));
#52525=CARTESIAN_POINT('',(14.,36.375288143631,133.639021904261));
#52526=CARTESIAN_POINT('',(14.,36.375288143631,133.639021904261));
#52527=CARTESIAN_POINT('',(14.5,36.4588101823949,134.134280331629));
#52528=CARTESIAN_POINT('Origin',(14.25,36.2180095292903,131.128722228666));
#52529=CARTESIAN_POINT('',(14.,35.9712881348695,131.169077569515));
#52530=CARTESIAN_POINT('',(14.5,36.4647309237111,131.088366887817));
#52531=CARTESIAN_POINT('Origin',(14.5,34.8330975492484,134.054819567983));
#52532=CARTESIAN_POINT('',(14.,35.3175873497673,133.922431977811));
#52533=CARTESIAN_POINT('',(14.5,35.4928843561058,134.393099376732));
#52534=CARTESIAN_POINT('',(14.,35.3175873497673,133.922431977811));
#52535=CARTESIAN_POINT('',(14.5,34.8330975492484,134.054819567983));
#52536=CARTESIAN_POINT('',(14.5,34.8330975492484,134.054819567983));
#52537=CARTESIAN_POINT('',(14.5,35.4928843561058,134.393099376732));
#52538=CARTESIAN_POINT('Origin',(14.25,34.9094680429235,133.549897224021));
#52539=CARTESIAN_POINT('',(14.5,34.6756233772733,133.638309170877));
#52540=CARTESIAN_POINT('',(14.,35.1433127085737,133.461485277164));
#52541=CARTESIAN_POINT('Origin',(14.,35.1629909526771,134.223959472357));
#52542=CARTESIAN_POINT('',(14.,35.4928843561058,134.393099376732));
#52543=CARTESIAN_POINT('',(14.,34.8330975492484,134.054819567983));
#52544=CARTESIAN_POINT('Origin',(14.25,36.3941054211193,133.892798875057));
#52545=CARTESIAN_POINT('',(14.5,36.4588101823949,134.134280331629));
#52546=CARTESIAN_POINT('',(14.,36.3294006598436,133.651317418485));
#52547=CARTESIAN_POINT('Origin',(14.,36.6599362981178,133.822854175933));
#52548=CARTESIAN_POINT('',(14.,36.8610624138407,133.511428020236));
#52549=CARTESIAN_POINT('',(14.,36.4588101823949,134.134280331629));
#52550=CARTESIAN_POINT('Origin',(57.75,34.9094680429235,133.549897224021));
#52551=CARTESIAN_POINT('',(58.,35.1433127085737,133.461485277164));
#52552=CARTESIAN_POINT('',(57.5,34.6756233772733,133.638309170877));
#52553=CARTESIAN_POINT('Origin',(57.75,36.3941054211193,133.892798875057));
#52554=CARTESIAN_POINT('',(58.,36.3294006598436,133.651317418485));
#52555=CARTESIAN_POINT('',(57.5,36.4588101823949,134.134280331629));
#52556=CARTESIAN_POINT('Origin',(57.75,36.2180095292903,131.128722228666));
#52557=CARTESIAN_POINT('',(57.5,36.4647309237111,131.088366887817));
#52558=CARTESIAN_POINT('',(58.,35.9712881348695,131.169077569515));
#52559=CARTESIAN_POINT('Origin',(14.,35.4582091790453,132.331838201602));
#52560=CARTESIAN_POINT('Origin',(14.,36.292867245645,130.037639885881));
#52561=CARTESIAN_POINT('Origin',(14.,36.9417730955394,134.004870809078));
#52562=CARTESIAN_POINT('Origin',(1.88275881709439,0.,-3.89963199725568E-15));
#52563=CARTESIAN_POINT('',(1.46551763418878,127.371647073124,-1.55985279890227E-14));
#52564=CARTESIAN_POINT('',(1.46551763418879,-127.371647073124,-1.55985279890227E-14));
#52565=CARTESIAN_POINT('Origin',(1.46551763418878,0.,-7.79926399451136E-15));
#52566=CARTESIAN_POINT('Origin',(1.46551763418878,0.,-7.79926399451136E-15));
#52567=CARTESIAN_POINT('',(2.3,127.,1.55530143491714E-14));
#52568=CARTESIAN_POINT('',(1.88275881709439,127.185823536562,-1.5575771169097E-14));
#52569=CARTESIAN_POINT('',(2.3,-127.,-1.55530143491714E-14));
#52570=CARTESIAN_POINT('Origin',(2.3,0.,0.));
#52571=CARTESIAN_POINT('Origin',(2.3,0.,0.));
#52572=CARTESIAN_POINT('Origin',(0.9,0.,0.));
#52573=CARTESIAN_POINT('',(0.334482365811226,-128.628352926876,-1.57524300691495E-14));
#52574=CARTESIAN_POINT('',(0.9,-128.,-1.56754790290861E-14));
#52575=CARTESIAN_POINT('',(0.334482365811233,128.628352926876,1.57524300691495E-14));
#52576=CARTESIAN_POINT('Origin',(0.334482365811233,0.,-7.87621503457476E-15));
#52577=CARTESIAN_POINT('Origin',(0.334482365811233,0.,-7.87621503457476E-15));
#52578=CARTESIAN_POINT('Origin',(30.775,0.,0.));
#52579=CARTESIAN_POINT('',(59.75,-127.,-1.55530143491714E-14));
#52580=CARTESIAN_POINT('Origin',(59.75,0.,0.));
#52581=CARTESIAN_POINT('',(30.775,-127.,-1.55530143491714E-14));
#52582=CARTESIAN_POINT('Origin',(57.5,24.6295005722094,136.801453579863));
#52583=CARTESIAN_POINT('',(57.5,25.0845072682929,136.216030001563));
#52584=CARTESIAN_POINT('',(58.,24.5894609761083,136.30080033501));
#52585=CARTESIAN_POINT('',(57.5,25.0845072682929,136.216030001563));
#52586=CARTESIAN_POINT('',(57.5,24.6295005722094,136.801453579863));
#52587=CARTESIAN_POINT('',(57.5,24.6295005722094,136.801453579863));
#52588=CARTESIAN_POINT('',(58.,24.5894609761083,136.30080033501));
#52589=CARTESIAN_POINT('Origin',(57.5,23.016899728323,136.580604996376));
#52590=CARTESIAN_POINT('',(57.5,23.6446928191972,136.97510175753));
#52591=CARTESIAN_POINT('',(58.,23.5110842376315,136.490947249372));
#52592=CARTESIAN_POINT('',(57.5,23.6446928191972,136.97510175753));
#52593=CARTESIAN_POINT('',(57.5,23.016899728323,136.580604996376));
#52594=CARTESIAN_POINT('',(57.5,23.016899728323,136.580604996376));
#52595=CARTESIAN_POINT('',(58.,23.5110842376315,136.490947249372));
#52596=CARTESIAN_POINT('Origin',(14.,24.5894609761083,136.30080033501));
#52597=CARTESIAN_POINT('',(14.5,25.0845072682929,136.216030001563));
#52598=CARTESIAN_POINT('',(14.5,24.6295005722094,136.801453579863));
#52599=CARTESIAN_POINT('',(14.5,25.0845072682929,136.216030001563));
#52600=CARTESIAN_POINT('',(14.,24.5894609761083,136.30080033501));
#52601=CARTESIAN_POINT('',(14.,24.5894609761083,136.30080033501));
#52602=CARTESIAN_POINT('',(14.5,24.6295005722094,136.801453579863));
#52603=CARTESIAN_POINT('Origin',(14.25,24.6515678871246,133.786345373109));
#52604=CARTESIAN_POINT('',(14.,24.4022681423913,133.805043963321));
#52605=CARTESIAN_POINT('',(14.5,24.900867631858,133.767646782898));
#52606=CARTESIAN_POINT('Origin',(14.5,23.016899728323,136.580604996376));
#52607=CARTESIAN_POINT('',(14.,23.5110842376315,136.490947249372));
#52608=CARTESIAN_POINT('',(14.5,23.6446928191972,136.97510175753));
#52609=CARTESIAN_POINT('',(14.,23.5110842376315,136.490947249372));
#52610=CARTESIAN_POINT('',(14.5,23.016899728323,136.580604996376));
#52611=CARTESIAN_POINT('',(14.5,23.016899728323,136.580604996376));
#52612=CARTESIAN_POINT('',(14.5,23.6446928191972,136.97510175753));
#52613=CARTESIAN_POINT('Origin',(14.25,23.1369864911307,136.084260161474));
#52614=CARTESIAN_POINT('',(14.5,22.8963260661369,136.151954768658));
#52615=CARTESIAN_POINT('',(14.,23.3776469161245,136.01656555429));
#52616=CARTESIAN_POINT('Origin',(14.,23.3307962737601,136.777853376953));
#52617=CARTESIAN_POINT('',(14.,23.6446928191972,136.97510175753));
#52618=CARTESIAN_POINT('',(14.,23.016899728323,136.580604996376));
#52619=CARTESIAN_POINT('Origin',(14.25,24.5860885277927,136.55525164161));
#52620=CARTESIAN_POINT('',(14.5,24.6295005722094,136.801453579863));
#52621=CARTESIAN_POINT('',(14.,24.542676483376,136.309049703357));
#52622=CARTESIAN_POINT('Origin',(14.,24.8570039202511,136.508741790713));
#52623=CARTESIAN_POINT('',(14.,25.0845072682929,136.216030001563));
#52624=CARTESIAN_POINT('',(14.,24.6295005722094,136.801453579863));
#52625=CARTESIAN_POINT('Origin',(57.75,23.1369864911307,136.084260161474));
#52626=CARTESIAN_POINT('',(58.,23.3776469161245,136.01656555429));
#52627=CARTESIAN_POINT('',(57.5,22.8963260661369,136.151954768658));
#52628=CARTESIAN_POINT('Origin',(57.75,24.5860885277927,136.55525164161));
#52629=CARTESIAN_POINT('',(58.,24.542676483376,136.309049703357));
#52630=CARTESIAN_POINT('',(57.5,24.6295005722094,136.801453579863));
#52631=CARTESIAN_POINT('Origin',(57.75,24.6515678871246,133.786345373109));
#52632=CARTESIAN_POINT('',(57.5,24.900867631858,133.767646782898));
#52633=CARTESIAN_POINT('',(58.,24.4022681423913,133.805043963321));
#52634=CARTESIAN_POINT('Origin',(14.,23.7898003403695,134.918662162673));
#52635=CARTESIAN_POINT('Origin',(14.,24.8212348392527,132.705939207914));
#52636=CARTESIAN_POINT('Origin',(14.,25.1219044487155,136.71462949103));
#52637=CARTESIAN_POINT('Origin',(57.5,12.6127455909704,138.427485163379));
#52638=CARTESIAN_POINT('',(57.5,13.1170438759937,137.883945745091));
#52639=CARTESIAN_POINT('',(58.,12.6164931630349,137.925247374536));
#52640=CARTESIAN_POINT('',(57.5,13.1170438759937,137.883945745091));
#52641=CARTESIAN_POINT('',(57.5,12.6127455909704,138.427485163379));
#52642=CARTESIAN_POINT('',(57.5,12.6127455909704,138.427485163379));
#52643=CARTESIAN_POINT('',(58.,12.6164931630349,137.925247374536));
#52644=CARTESIAN_POINT('Origin',(57.5,11.025529402481,138.066929551123));
#52645=CARTESIAN_POINT('',(57.5,11.6165508928786,138.514640906126));
#52646=CARTESIAN_POINT('',(58.,11.5256475780665,138.020683996878));
#52647=CARTESIAN_POINT('',(57.5,11.6165508928786,138.514640906126));
#52648=CARTESIAN_POINT('',(57.5,11.0255294024811,138.066929551123));
#52649=CARTESIAN_POINT('',(57.5,11.025529402481,138.066929551123));
#52650=CARTESIAN_POINT('',(58.,11.5256475780665,138.020683996878));
#52651=CARTESIAN_POINT('Origin',(14.,12.6164931630349,137.925247374536));
#52652=CARTESIAN_POINT('',(14.5,13.1170438759937,137.883945745091));
#52653=CARTESIAN_POINT('',(14.5,12.6127455909704,138.427485163379));
#52654=CARTESIAN_POINT('',(14.5,13.1170438759937,137.883945745091));
#52655=CARTESIAN_POINT('',(14.,12.6164931630349,137.925247374536));
#52656=CARTESIAN_POINT('',(14.,12.6164931630349,137.925247374536));
#52657=CARTESIAN_POINT('',(14.5,12.6127455909704,138.427485163379));
#52658=CARTESIAN_POINT('Origin',(14.25,12.8975129283142,135.425773646859));
#52659=CARTESIAN_POINT('',(14.,12.647532154857,135.422673178871));
#52660=CARTESIAN_POINT('',(14.5,13.1474937017714,135.428874114848));
#52661=CARTESIAN_POINT('Origin',(14.5,11.0255294024811,138.066929551123));
#52662=CARTESIAN_POINT('',(14.,11.5256475780664,138.020683996878));
#52663=CARTESIAN_POINT('',(14.5,11.6165508928786,138.514640906126));
#52664=CARTESIAN_POINT('',(14.,11.5256475780664,138.020683996878));
#52665=CARTESIAN_POINT('',(14.5,11.025529402481,138.066929551123));
#52666=CARTESIAN_POINT('',(14.5,11.0255294024811,138.066929551123));
#52667=CARTESIAN_POINT('',(14.5,11.6165508928786,138.514640906126));
#52668=CARTESIAN_POINT('Origin',(14.25,11.188418501646,137.582939709175));
#52669=CARTESIAN_POINT('',(14.5,10.9427738884575,137.629401779851));
#52670=CARTESIAN_POINT('',(14.,11.4340631148345,137.536477638499));
#52671=CARTESIAN_POINT('Origin',(14.,11.3210401476798,138.290785228625));
#52672=CARTESIAN_POINT('',(14.,11.6165508928786,138.514640906126));
#52673=CARTESIAN_POINT('',(14.,11.025529402481,138.066929551123));
#52674=CARTESIAN_POINT('Origin',(14.25,12.5909566552835,138.178436488856));
#52675=CARTESIAN_POINT('',(14.5,12.6127455909704,138.427485163379));
#52676=CARTESIAN_POINT('',(14.,12.5691677195965,137.929387814333));
#52677=CARTESIAN_POINT('Origin',(14.,12.864894733482,138.155715454235));
#52678=CARTESIAN_POINT('',(14.,13.1170438759937,137.883945745091));
#52679=CARTESIAN_POINT('',(14.,12.6127455909704,138.427485163379));
#52680=CARTESIAN_POINT('Origin',(57.75,11.188418501646,137.582939709175));
#52681=CARTESIAN_POINT('',(58.,11.4340631148345,137.536477638499));
#52682=CARTESIAN_POINT('',(57.5,10.9427738884575,137.629401779851));
#52683=CARTESIAN_POINT('Origin',(57.75,12.5909566552835,138.178436488856));
#52684=CARTESIAN_POINT('',(58.,12.5691677195965,137.929387814333));
#52685=CARTESIAN_POINT('',(57.5,12.6127455909704,138.427485163379));
#52686=CARTESIAN_POINT('Origin',(57.75,12.8975129283142,135.425773646859));
#52687=CARTESIAN_POINT('',(57.5,13.1474937017714,135.428874114848));
#52688=CARTESIAN_POINT('',(58.,12.647532154857,135.422673178871));
#52689=CARTESIAN_POINT('Origin',(14.,11.9403367564292,136.478673638569));
#52690=CARTESIAN_POINT('Origin',(14.,13.1606978482623,134.364266202539));
#52691=CARTESIAN_POINT('Origin',(14.,13.1108429400163,138.383907292005));
#52692=CARTESIAN_POINT('Origin',(11.2910997468263,0.,-4.24054782501806E-15));
#52693=CARTESIAN_POINT('',(11.5821994936527,138.506803038084,-1.69621913000722E-14));
#52694=CARTESIAN_POINT('',(11.5821994936527,-138.506803038084,-1.69621913000722E-14));
#52695=CARTESIAN_POINT('Origin',(11.5821994936527,0.,-8.48109565003612E-15));
#52696=CARTESIAN_POINT('Origin',(11.5821994936527,0.,-8.48109565003612E-15));
#52697=CARTESIAN_POINT('',(11.,139.,1.70225905081482E-14));
#52698=CARTESIAN_POINT('',(11.2910997468263,138.753401519042,1.69923909041102E-14));
#52699=CARTESIAN_POINT('',(11.,-139.,-1.70225905081482E-14));
#52700=CARTESIAN_POINT('Origin',(11.,0.,0.));
#52701=CARTESIAN_POINT('Origin',(11.,0.,0.));
#52702=CARTESIAN_POINT('Origin',(5.75,0.,0.));
#52703=CARTESIAN_POINT('',(1.5,-139.,-1.70225905081482E-14));
#52704=CARTESIAN_POINT('',(5.75,-139.,-1.70225905081482E-14));
#52705=CARTESIAN_POINT('',(1.5,139.,-1.70225905081482E-14));
#52706=CARTESIAN_POINT('Origin',(1.5,0.,0.));
#52707=CARTESIAN_POINT('Origin',(1.5,0.,0.));
#52708=CARTESIAN_POINT('Origin',(11.75,0.,0.));
#52709=CARTESIAN_POINT('',(11.75,-137.5,-1.68388934882761E-14));
#52710=CARTESIAN_POINT('Origin',(0.167241182905616,0.,-3.93810751728738E-15));
#52711=CARTESIAN_POINT('',(0.,129.5,-1.58591760489582E-14));
#52712=CARTESIAN_POINT('Origin',(0.,0.,0.));
#52713=CARTESIAN_POINT('',(0.167241182905616,129.064176463438,-1.58058030590539E-14));
#52714=CARTESIAN_POINT('Origin',(0.,139.,0.));
#52715=CARTESIAN_POINT('',(0.,137.5,1.68388934882761E-14));
#52716=CARTESIAN_POINT('Origin',(0.,0.,0.));
#52717=CARTESIAN_POINT('Origin',(1.07322330470336,0.,4.24482317633411E-15));
#52718=CARTESIAN_POINT('',(0.646446609406718,138.646446609407,3.39585854106729E-14));
#52719=CARTESIAN_POINT('Origin',(0.646446609406718,0.,8.48964635266822E-15));
#52720=CARTESIAN_POINT('',(1.07322330470336,138.823223304703,-8.51129525407411E-15));
#52721=CARTESIAN_POINT('Origin',(0.5,0.,0.));
#52722=CARTESIAN_POINT('',(0.353553390593267,138.353553390593,0.));
#52723=CARTESIAN_POINT('',(0.5,138.5,1.69613581681908E-14));
#52724=CARTESIAN_POINT('Origin',(0.353553390593267,0.,8.47171181552262E-15));
#52725=CARTESIAN_POINT('Origin',(0.176776695296634,0.,4.23585590776131E-15));
#52726=CARTESIAN_POINT('',(0.176776695296634,137.926776695297,2.53628703751833E-14));
#52727=CARTESIAN_POINT('Origin',(14.,11.1184535438328,138.5582187775));
#52728=CARTESIAN_POINT('Origin',(58.,11.9403367564292,136.478673638569));
#52729=CARTESIAN_POINT('Origin',(14.,23.1522889426911,137.061925846364));
#52730=CARTESIAN_POINT('Origin',(58.,23.7898003403695,134.918662162673));
#52731=CARTESIAN_POINT('Origin',(14.,35.0099214429613,134.522508899283));
#52732=CARTESIAN_POINT('Origin',(58.,35.4582091790453,132.331838201602));
#52733=CARTESIAN_POINT('Origin',(14.,46.6011073014821,130.959294432567));
#52734=CARTESIAN_POINT('Origin',(58.,46.8567596356167,128.737889047669));
#52735=CARTESIAN_POINT('Origin',(14.,57.8987018584759,124.164166824021));
#52736=CARTESIAN_POINT('Origin',(58.,57.8987018584759,124.164166824021));
#52737=CARTESIAN_POINT('Origin',(14.,68.6339745962156,120.877531126037));
#52738=CARTESIAN_POINT('Origin',(58.,68.5000000000001,118.645480318468));
#52739=CARTESIAN_POINT('Origin',(14.,78.5799717800934,112.223830067592));
#52740=CARTESIAN_POINT('Origin',(14.,78.9079726085065,114.435710592521));
#52741=CARTESIAN_POINT('Origin',(14.,88.58143330331,107.122965203224));
#52742=CARTESIAN_POINT('Origin',(58.,88.0619025270559,104.9480887073));
#52743=CARTESIAN_POINT('Origin',(14.,97.5807358037436,98.9949493661166));
#52744=CARTESIAN_POINT('Origin',(58.,96.873629022557,96.873629022557));
#52745=CARTESIAN_POINT('Origin',(14.,104.9480887073,88.0619025270559));
#52746=CARTESIAN_POINT('Origin',(58.,104.9480887073,88.0619025270559));
#52747=CARTESIAN_POINT('Origin',(14.,113.288557719819,80.5462766970844));
#52748=CARTESIAN_POINT('Origin',(58.,112.223830067592,78.5799717800933));
#52749=CARTESIAN_POINT('Origin',(14.,118.645480318468,68.5));
#52750=CARTESIAN_POINT('Origin',(14.,119.877531126037,70.3660254037845));
#52751=CARTESIAN_POINT('Origin',(14.,125.554164136354,59.6502461689938));
#52752=CARTESIAN_POINT('Origin',(58.,124.164166824021,57.8987018584757));
#52753=CARTESIAN_POINT('Origin',(14.,130.275254145916,48.4804925430538));
#52754=CARTESIAN_POINT('Origin',(58.,128.737889047669,46.8567596356165));
#52755=CARTESIAN_POINT('Origin',(14.,132.331838201602,35.4582091790453));
#52756=CARTESIAN_POINT('Origin',(58.,132.331838201602,35.4582091790453));
#52757=CARTESIAN_POINT('Origin',(14.,136.71462949103,25.1219044487155));
#52758=CARTESIAN_POINT('Origin',(58.,134.918662162673,23.7898003403694));
#52759=CARTESIAN_POINT('Origin',(14.,136.478673638569,11.9403367564291));
#52760=CARTESIAN_POINT('Origin',(14.,138.383907292005,13.1108429400162));
#52761=CARTESIAN_POINT('Origin',(14.,139.,0.999999999999974));
#52762=CARTESIAN_POINT('Origin',(58.,137.,-2.51664917224781E-14));
#52763=CARTESIAN_POINT('Origin',(14.,138.5582187775,-11.1184535438328));
#52764=CARTESIAN_POINT('Origin',(58.,136.478673638569,-11.9403367564292));
#52765=CARTESIAN_POINT('Origin',(14.,134.918662162673,-23.7898003403695));
#52766=CARTESIAN_POINT('Origin',(58.,134.918662162673,-23.7898003403695));
#52767=CARTESIAN_POINT('Origin',(14.,134.522508899283,-35.0099214429613));
#52768=CARTESIAN_POINT('Origin',(58.,132.331838201602,-35.4582091790453));
#52769=CARTESIAN_POINT('Origin',(14.,128.737889047669,-46.8567596356167));
#52770=CARTESIAN_POINT('Origin',(14.,130.959294432567,-46.6011073014821));
#52771=CARTESIAN_POINT('Origin',(14.,126.399400659835,-57.8376305949206));
#52772=CARTESIAN_POINT('Origin',(58.,124.164166824021,-57.8987018584759));
#52773=CARTESIAN_POINT('Origin',(14.,120.877531126037,-68.6339745962156));
#52774=CARTESIAN_POINT('Origin',(58.,118.645480318468,-68.5000000000001));
#52775=CARTESIAN_POINT('Origin',(14.,112.223830067592,-78.5799717800934));
#52776=CARTESIAN_POINT('Origin',(58.,112.223830067592,-78.5799717800934));
#52777=CARTESIAN_POINT('Origin',(14.,107.122965203224,-88.58143330331));
#52778=CARTESIAN_POINT('Origin',(58.,104.9480887073,-88.0619025270559));
#52779=CARTESIAN_POINT('Origin',(14.,96.873629022557,-96.873629022557));
#52780=CARTESIAN_POINT('Origin',(14.,98.9949493661167,-97.5807358037436));
#52781=CARTESIAN_POINT('Origin',(14.,90.113522189548,-105.837389983851));
#52782=CARTESIAN_POINT('Origin',(58.,88.0619025270559,-104.9480887073));
#52783=CARTESIAN_POINT('Origin',(14.,80.5462766970844,-113.288557719819));
#52784=CARTESIAN_POINT('Origin',(58.,78.5799717800933,-112.223830067592));
#52785=CARTESIAN_POINT('Origin',(14.,68.5,-118.645480318468));
#52786=CARTESIAN_POINT('Origin',(58.,68.5,-118.645480318468));
#52787=CARTESIAN_POINT('Origin',(14.,59.6502461689939,-125.554164136354));
#52788=CARTESIAN_POINT('Origin',(58.,57.8987018584758,-124.164166824021));
#52789=CARTESIAN_POINT('Origin',(14.,46.8567596356166,-128.737889047669));
#52790=CARTESIAN_POINT('Origin',(14.,48.4804925430539,-130.275254145916));
#52791=CARTESIAN_POINT('Origin',(14.,36.9417730955395,-134.004870809078));
#52792=CARTESIAN_POINT('Origin',(58.,35.4582091790453,-132.331838201602));
#52793=CARTESIAN_POINT('Origin',(14.,25.1219044487155,-136.71462949103));
#52794=CARTESIAN_POINT('Origin',(58.,23.7898003403694,-134.918662162673));
#52795=CARTESIAN_POINT('Origin',(14.,11.9403367564291,-136.478673638569));
#52796=CARTESIAN_POINT('Origin',(58.,11.9403367564291,-136.478673638569));
#52797=CARTESIAN_POINT('Origin',(14.,0.999999999999983,-139.));
#52798=CARTESIAN_POINT('Origin',(58.,-1.67776611483187E-14,-137.));
#52799=CARTESIAN_POINT('Origin',(14.,-11.9403367564292,-136.478673638569));
#52800=CARTESIAN_POINT('Origin',(14.,-11.1184535438327,-138.5582187775));
#52801=CARTESIAN_POINT('Origin',(14.,-23.1522889426912,-137.061925846364));
#52802=CARTESIAN_POINT('Origin',(58.,-23.7898003403695,-134.918662162672));
#52803=CARTESIAN_POINT('Origin',(14.,-35.0099214429614,-134.522508899283));
#52804=CARTESIAN_POINT('Origin',(58.,-35.4582091790454,-132.331838201602));
#52805=CARTESIAN_POINT('Origin',(14.,-46.8567596356166,-128.737889047669));
#52806=CARTESIAN_POINT('Origin',(58.,-46.8567596356166,-128.737889047669));
#52807=CARTESIAN_POINT('Origin',(14.,-57.8376305949206,-126.399400659835));
#52808=CARTESIAN_POINT('Origin',(58.,-57.8987018584758,-124.164166824021));
#52809=CARTESIAN_POINT('Origin',(14.,-68.5,-118.645480318468));
#52810=CARTESIAN_POINT('Origin',(14.,-68.6339745962156,-120.877531126037));
#52811=CARTESIAN_POINT('Origin',(14.,-78.9079726085065,-114.435710592521));
#52812=CARTESIAN_POINT('Origin',(58.,-78.5799717800934,-112.223830067592));
#52813=CARTESIAN_POINT('Origin',(14.,-88.58143330331,-107.122965203224));
#52814=CARTESIAN_POINT('Origin',(58.,-88.0619025270559,-104.9480887073));
#52815=CARTESIAN_POINT('Origin',(14.,-96.873629022557,-96.873629022557));
#52816=CARTESIAN_POINT('Origin',(58.,-96.873629022557,-96.873629022557));
#52817=CARTESIAN_POINT('Origin',(14.,-105.837389983851,-90.113522189548));
#52818=CARTESIAN_POINT('Origin',(58.,-104.9480887073,-88.0619025270559));
#52819=CARTESIAN_POINT('Origin',(14.,-112.223830067592,-78.5799717800933));
#52820=CARTESIAN_POINT('Origin',(14.,-113.288557719819,-80.5462766970844));
#52821=CARTESIAN_POINT('Origin',(14.,-119.877531126037,-70.3660254037844));
#52822=CARTESIAN_POINT('Origin',(58.,-118.645480318468,-68.5));
#52823=CARTESIAN_POINT('Origin',(14.,-125.554164136354,-59.6502461689939));
#52824=CARTESIAN_POINT('Origin',(58.,-124.164166824021,-57.8987018584758));
#52825=CARTESIAN_POINT('Origin',(14.,-128.737889047669,-46.8567596356166));
#52826=CARTESIAN_POINT('Origin',(58.,-128.737889047669,-46.8567596356166));
#52827=CARTESIAN_POINT('Origin',(14.,-134.004870809078,-36.9417730955394));
#52828=CARTESIAN_POINT('Origin',(58.,-132.331838201602,-35.4582091790453));
#52829=CARTESIAN_POINT('Origin',(14.,-134.918662162673,-23.7898003403695));
#52830=CARTESIAN_POINT('Origin',(14.,-136.71462949103,-25.1219044487155));
#52831=CARTESIAN_POINT('Origin',(14.,-138.383907292005,-13.1108429400162));
#52832=CARTESIAN_POINT('Origin',(58.,-136.478673638569,-11.9403367564291));
#52833=CARTESIAN_POINT('Origin',(14.,-139.,-0.999999999999992));
#52834=CARTESIAN_POINT('Origin',(58.,-137.,8.38883057415937E-15));
#52835=CARTESIAN_POINT('Origin',(14.,-136.478673638569,11.9403367564292));
#52836=CARTESIAN_POINT('Origin',(58.,-136.478673638569,11.9403367564292));
#52837=CARTESIAN_POINT('Origin',(14.,-137.061925846364,23.1522889426911));
#52838=CARTESIAN_POINT('Origin',(58.,-134.918662162673,23.7898003403695));
#52839=CARTESIAN_POINT('Origin',(14.,-132.331838201602,35.4582091790453));
#52840=CARTESIAN_POINT('Origin',(14.,-134.522508899283,35.0099214429613));
#52841=CARTESIAN_POINT('Origin',(14.,-130.959294432567,46.6011073014821));
#52842=CARTESIAN_POINT('Origin',(58.,-128.737889047669,46.8567596356166));
#52843=CARTESIAN_POINT('Origin',(14.,-126.399400659835,57.8376305949206));
#52844=CARTESIAN_POINT('Origin',(58.,-124.164166824021,57.8987018584758));
#52845=CARTESIAN_POINT('Origin',(14.,-118.645480318468,68.5));
#52846=CARTESIAN_POINT('Origin',(58.,-118.645480318468,68.5));
#52847=CARTESIAN_POINT('Origin',(14.,-114.435710592521,78.9079726085064));
#52848=CARTESIAN_POINT('Origin',(58.,-112.223830067592,78.5799717800933));
#52849=CARTESIAN_POINT('Origin',(14.,-104.9480887073,88.0619025270559));
#52850=CARTESIAN_POINT('Origin',(14.,-107.122965203224,88.58143330331));
#52851=CARTESIAN_POINT('Origin',(14.,-98.9949493661167,97.5807358037436));
#52852=CARTESIAN_POINT('Origin',(58.,-96.873629022557,96.873629022557));
#52853=CARTESIAN_POINT('Origin',(14.,-90.113522189548,105.837389983851));
#52854=CARTESIAN_POINT('Origin',(58.,-88.0619025270559,104.9480887073));
#52855=CARTESIAN_POINT('Origin',(14.,-78.5799717800933,112.223830067592));
#52856=CARTESIAN_POINT('Origin',(58.,-78.5799717800933,112.223830067592));
#52857=CARTESIAN_POINT('Origin',(14.,-70.3660254037844,119.877531126037));
#52858=CARTESIAN_POINT('Origin',(58.,-68.5,118.645480318468));
#52859=CARTESIAN_POINT('Origin',(14.,-57.8987018584758,124.164166824021));
#52860=CARTESIAN_POINT('Origin',(14.,-59.6502461689939,125.554164136354));
#52861=CARTESIAN_POINT('Origin',(14.,-48.4804925430539,130.275254145916));
#52862=CARTESIAN_POINT('Origin',(58.,-46.8567596356166,128.737889047669));
#52863=CARTESIAN_POINT('Origin',(14.,-36.9417730955394,134.004870809078));
#52864=CARTESIAN_POINT('Origin',(58.,-35.4582091790453,132.331838201602));
#52865=CARTESIAN_POINT('Origin',(14.,-23.7898003403695,134.918662162673));
#52866=CARTESIAN_POINT('Origin',(58.,-23.7898003403695,134.918662162673));
#52867=CARTESIAN_POINT('Origin',(14.,-13.1108429400162,138.383907292005));
#52868=CARTESIAN_POINT('Origin',(58.,-11.9403367564292,136.478673638569));
#52869=CARTESIAN_POINT('Origin',(14.,0.,137.));
#52870=CARTESIAN_POINT('Origin',(14.,-1.,139.));
#52871=CARTESIAN_POINT('Origin',(80.,33.5919271685148,-46.2353212285282));
#52872=CARTESIAN_POINT('',(62.,33.5919271685148,-39.0553212285282));
#52873=CARTESIAN_POINT('',(80.,33.5919271685148,-39.0553212285282));
#52874=CARTESIAN_POINT('Origin',(62.,33.5919271685148,-46.2353212285282));
#52875=CARTESIAN_POINT('Origin',(80.,-33.5919271685148,-46.2353212285282));
#52876=CARTESIAN_POINT('',(62.,-33.5919271685148,-39.0553212285282));
#52877=CARTESIAN_POINT('',(80.,-33.5919271685148,-39.0553212285282));
#52878=CARTESIAN_POINT('Origin',(62.,-33.5919271685148,-46.2353212285282));
#52879=CARTESIAN_POINT('Origin',(80.,-54.352879906268,17.6603212285283));
#52880=CARTESIAN_POINT('',(62.,-54.352879906268,24.8403212285282));
#52881=CARTESIAN_POINT('',(80.,-54.352879906268,24.8403212285282));
#52882=CARTESIAN_POINT('Origin',(62.,-54.352879906268,17.6603212285283));
#52883=CARTESIAN_POINT('Origin',(80.,3.49942822856356E-15,57.15));
#52884=CARTESIAN_POINT('',(62.,2.62013182677576E-15,64.33));
#52885=CARTESIAN_POINT('',(80.,4.37872463035136E-15,64.33));
#52886=CARTESIAN_POINT('Origin',(62.,3.49942822856356E-15,57.15));
#52887=CARTESIAN_POINT('Origin',(80.,54.352879906268,17.6603212285282));
#52888=CARTESIAN_POINT('',(62.,54.352879906268,24.8403212285282));
#52889=CARTESIAN_POINT('',(80.,54.352879906268,24.8403212285282));
#52890=CARTESIAN_POINT('Origin',(62.,54.352879906268,17.6603212285282));
#52891=CARTESIAN_POINT('Origin',(76.,0.,0.));
#52892=CARTESIAN_POINT('',(75.,-27.,-3.30654635769785E-15));
#52893=CARTESIAN_POINT('Origin',(75.,0.,0.));
#52894=CARTESIAN_POINT('',(77.,-23.,-2.81668763803891E-15));
#52895=CARTESIAN_POINT('',(76.,-25.,-3.06161699786838E-15));
#52896=CARTESIAN_POINT('Origin',(77.,0.,0.));
#52897=CARTESIAN_POINT('Origin',(78.5,0.,0.));
#52898=CARTESIAN_POINT('',(80.,-23.,-2.81668763803891E-15));
#52899=CARTESIAN_POINT('',(78.5,-23.,-2.81668763803891E-15));
#52900=CARTESIAN_POINT('Origin',(80.,0.,0.));
#52901=CARTESIAN_POINT('Origin',(72.,-54.352879906268,17.6603212285283));
#52902=CARTESIAN_POINT('',(72.,-43.6855709521459,28.205866244188));
#52903=CARTESIAN_POINT('',(72.,-43.6855709521459,28.205866244188));
#52904=CARTESIAN_POINT('Origin',(72.,-54.352879906268,17.6603212285283));
#52905=CARTESIAN_POINT('Origin',(72.,0.,0.));
#52906=CARTESIAN_POINT('',(72.,-13.3257890560989,50.2635389326334));
#52907=CARTESIAN_POINT('',(72.,-13.3257890560989,50.2635389326334));
#52908=CARTESIAN_POINT('Origin',(72.,0.,0.));
#52909=CARTESIAN_POINT('Origin',(72.,3.49942822856356E-15,57.15));
#52910=CARTESIAN_POINT('',(72.,13.3257890560989,50.2635389326334));
#52911=CARTESIAN_POINT('',(72.,13.3257890560989,50.2635389326334));
#52912=CARTESIAN_POINT('Origin',(72.,3.49942822856356E-15,57.15));
#52913=CARTESIAN_POINT('Origin',(72.,0.,0.));
#52914=CARTESIAN_POINT('Origin',(72.,0.,0.));
#52915=CARTESIAN_POINT('Origin',(72.,50.,0.));
#52916=CARTESIAN_POINT('Origin',(92.5,0.,0.));
#52917=CARTESIAN_POINT('',(80.,-25.16,-3.08121134665474E-15));
#52918=CARTESIAN_POINT('',(92.5,-25.16,-3.08121134665474E-15));
#52919=CARTESIAN_POINT('Origin',(80.,0.,0.));
#52920=CARTESIAN_POINT('Origin',(80.,23.,0.));
#52921=CARTESIAN_POINT('Origin',(54.5,0.,0.));
#52922=CARTESIAN_POINT('',(34.,-27.,-3.30654635769785E-15));
#52923=CARTESIAN_POINT('',(54.5,-27.,-3.30654635769785E-15));
#52924=CARTESIAN_POINT('Origin',(34.,0.,0.));
#52925=CARTESIAN_POINT('Origin',(34.,26.,0.));
#52926=CARTESIAN_POINT('Origin',(23.47,0.,0.));
#52927=CARTESIAN_POINT('',(15.,-29.58,-3.62250523187787E-15));
#52928=CARTESIAN_POINT('',(23.47,-29.58,-3.62250523187787E-15));
#52929=CARTESIAN_POINT('Origin',(15.,0.,0.));
#52930=CARTESIAN_POINT('Origin',(15.,32.6,0.));
#52931=CARTESIAN_POINT('',(15.,-32.6,-3.99234856522037E-15));
#52932=CARTESIAN_POINT('Origin',(15.,0.,0.));
#52933=CARTESIAN_POINT('Origin',(10.3,0.,0.));
#52934=CARTESIAN_POINT('',(5.6,-32.6,-3.99234856522037E-15));
#52935=CARTESIAN_POINT('',(10.3,-32.6,-3.99234856522037E-15));
#52936=CARTESIAN_POINT('Origin',(5.6,0.,0.));
#52937=CARTESIAN_POINT('Origin',(5.3,0.,0.));
#52938=CARTESIAN_POINT('',(5.3,-32.9,-4.02908796919479E-15));
#52939=CARTESIAN_POINT('Origin',(59.,0.,0.));
#52940=CARTESIAN_POINT('',(62.,-46.,-5.63337527607782E-15));
#52941=CARTESIAN_POINT('Origin',(62.,0.,0.));
#52942=CARTESIAN_POINT('',(59.,-43.,-5.26598123633362E-15));
#52943=CARTESIAN_POINT('Origin',(62.,123.,0.));
#52944=CARTESIAN_POINT('',(62.,-123.,-1.50631556295124E-14));
#52945=CARTESIAN_POINT('Origin',(62.,0.,0.));
#52946=CARTESIAN_POINT('Origin',(61.,0.,0.));
#52947=CARTESIAN_POINT('',(60.,-126.5,-1.5491782009214E-14));
#52948=CARTESIAN_POINT('',(61.,-124.75,-1.52774688193632E-14));
#52949=CARTESIAN_POINT('Origin',(60.,0.,0.));
#52950=CARTESIAN_POINT('Origin',(59.875,0.,0.));
#52951=CARTESIAN_POINT('',(59.875,-126.75,-1.55223981791927E-14));
#71600=UNCERTAINTY_MEASURE_WITH_UNIT(LENGTH_MEASURE(0.01),#71629,
'DISTANCE_ACCURACY_VALUE',
'Maximum model space distance between geometric entities at asserted c
onnectivities');
#71613=UNCERTAINTY_MEASURE_WITH_UNIT(LENGTH_MEASURE(0.01),#71629,
'DISTANCE_ACCURACY_VALUE',
'Maximum model space distance between geometric entities at asserted c
onnectivities');
#71615=(
GEOMETRIC_REPRESENTATION_CONTEXT(3)
GLOBAL_UNCERTAINTY_ASSIGNED_CONTEXT((#71600))
GLOBAL_UNIT_ASSIGNED_CONTEXT((#71629,#71631,#71632))
REPRESENTATION_CONTEXT('','3D')
);
#71628=(
GEOMETRIC_REPRESENTATION_CONTEXT(3)
GLOBAL_UNCERTAINTY_ASSIGNED_CONTEXT((#71613))
GLOBAL_UNIT_ASSIGNED_CONTEXT((#71629,#71631,#71632))
REPRESENTATION_CONTEXT('','3D')
);
#71629=(
LENGTH_UNIT()
NAMED_UNIT(*)
SI_UNIT(.MILLI.,.METRE.)
);
#71631=(
NAMED_UNIT(*)
PLANE_ANGLE_UNIT()
SI_UNIT($,.RADIAN.)
);
#71632=(
NAMED_UNIT(*)
SI_UNIT($,.STERADIAN.)
SOLID_ANGLE_UNIT()
);
#71634=SHAPE_DEFINITION_REPRESENTATION(#71648,#71683);
#71648=PRODUCT_DEFINITION_SHAPE('',$,#71698);
#71683=SHAPE_REPRESENTATION('',(#34366),#71615);
#71696=PRODUCT_DEFINITION_CONTEXT('part definition',#71740,'design');
#71698=PRODUCT_DEFINITION('2026-10-25-00-23-47-869',
'01_Hub_Drum_10x2.25_5on4.5_3500lb',#71712,#71696);
#71712=PRODUCT_DEFINITION_FORMATION('',$,#71743);
#71740=APPLICATION_CONTEXT(
'Core Data for Automotive Mechanical Design Process');
#71741=PRODUCT_CONTEXT('part definition',#71740,'mechanical');
#71743=PRODUCT('2026-10-25-00-23-47-869',
'01_Hub_Drum_10x2.25_5on4.5_3500lb',$,(#71741));
#71798=COLOUR_RGB('Light Blue',0.38,0.62,0.78);
#71799=FILL_AREA_STYLE_COLOUR('',#71798);
#71800=FILL_AREA_STYLE('',(#71799));
#71801=SURFACE_STYLE_FILL_AREA(#71800);
#71802=SURFACE_SIDE_STYLE('',(#71801));
#71803=SURFACE_STYLE_USAGE(.BOTH.,#71802);
#71804=PRESENTATION_STYLE_ASSIGNMENT((#71803));
ENDSEC;
END-ISO-10303-21;
